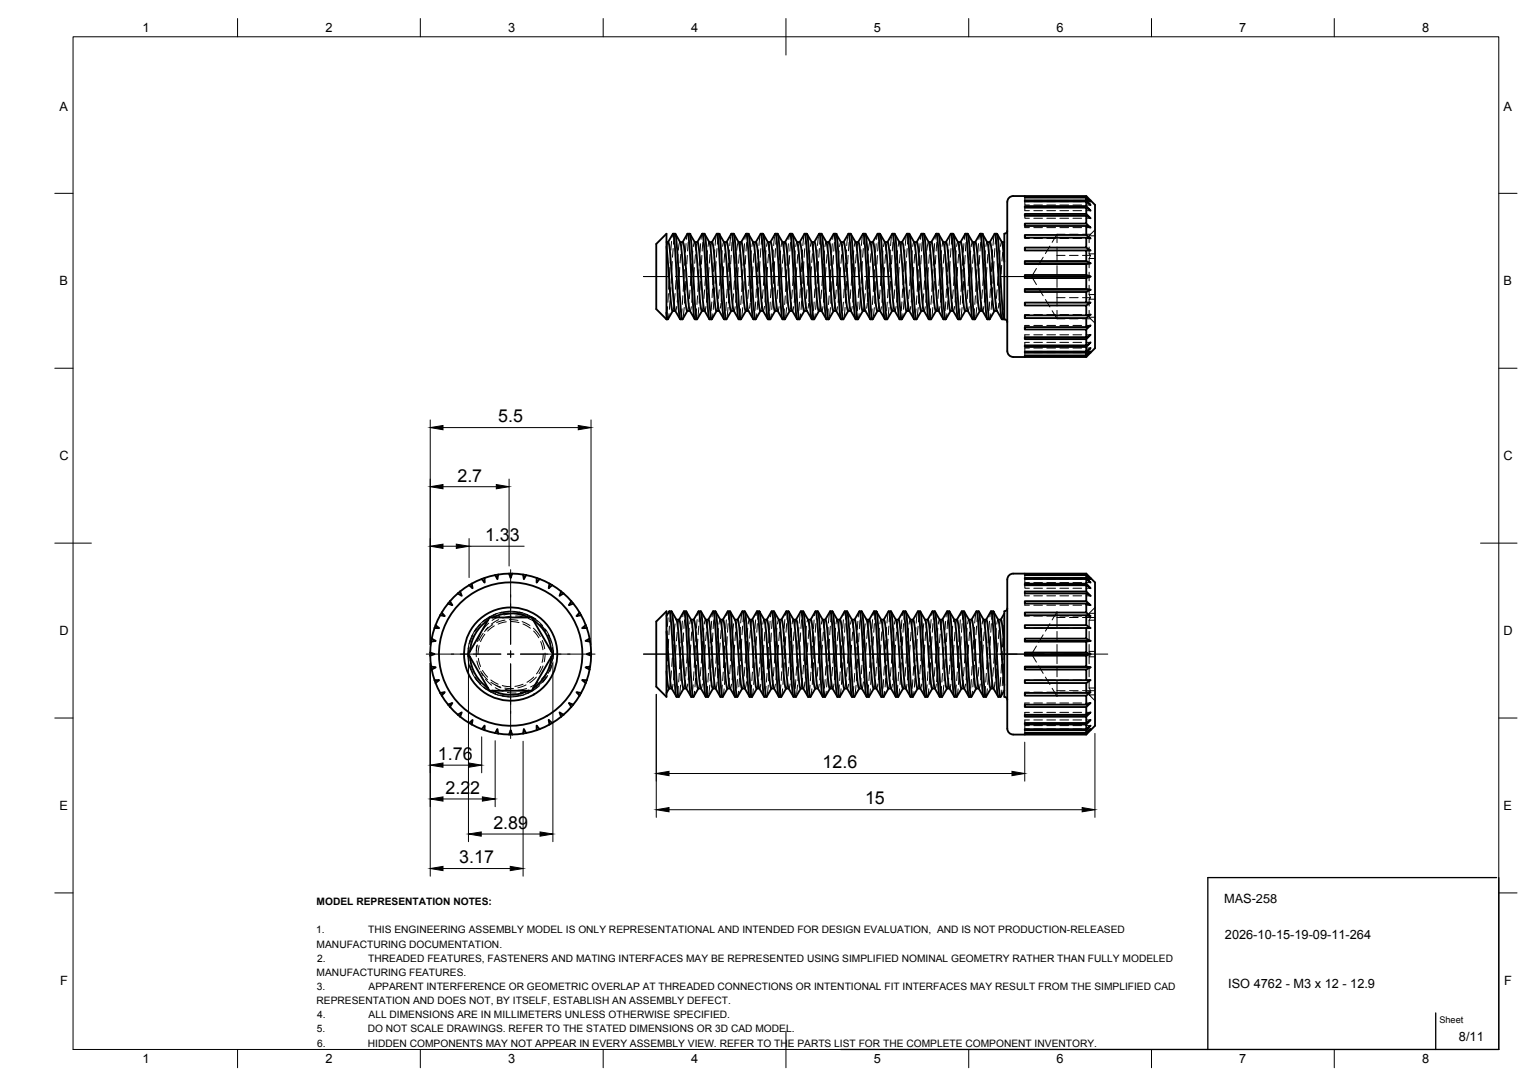
ISO-10303-21;
HEADER;
/* Generated by software containing ST-Developer
 * from STEP Tools, Inc. (www.steptools.com) 
 */

FILE_DESCRIPTION(
/* description */ (''),
/* implementation_level */ '2;1');

FILE_NAME(
/* name */ 'ISO 4762 - M3 x 12 - 12.9.step',
/* time_stamp */ '2026-10-15T12:29:06-07:00',
/* author */ (''),
/* organization */ (''),
/* preprocessor_version */ 'ST-DEVELOPER v20.2',
/* originating_system */ 'Autodesk Translation Framework v15.15.0.0',
/* authorisation */ '');

FILE_SCHEMA (('AUTOMOTIVE_DESIGN { 1 0 10303 214 3 1 1 }'));
ENDSEC;

DATA;
#10=MECHANICAL_DESIGN_GEOMETRIC_PRESENTATION_REPRESENTATION('',(#1749),#135282);
#95=TOROIDAL_SURFACE('',#33614,1.5635,0.1);
#96=TOROIDAL_SURFACE('',#33808,2.55,0.2);
#116=(
BOUNDED_CURVE()
B_SPLINE_CURVE(2,(#106679,#106680,#106681),.UNSPECIFIED.,.F.,.F.)
B_SPLINE_CURVE_WITH_KNOTS((3,3),(0.,0.0211644268265385),.UNSPECIFIED.)
CURVE()
GEOMETRIC_REPRESENTATION_ITEM()
RATIONAL_B_SPLINE_CURVE((1.,1.0009097917251,1.00093939181347))
REPRESENTATION_ITEM('')
);
#117=(
BOUNDED_CURVE()
B_SPLINE_CURVE(2,(#106685,#106686,#106687),.UNSPECIFIED.,.F.,.F.)
B_SPLINE_CURVE_WITH_KNOTS((3,3),(0.022587909800554,0.0437523366271111),
 .UNSPECIFIED.)
CURVE()
GEOMETRIC_REPRESENTATION_ITEM()
RATIONAL_B_SPLINE_CURVE((1.00093939181258,1.00090979172423,1.))
REPRESENTATION_ITEM('')
);
#118=(
BOUNDED_CURVE()
B_SPLINE_CURVE(2,(#106982,#106983,#106984),.UNSPECIFIED.,.F.,.F.)
B_SPLINE_CURVE_WITH_KNOTS((3,3),(0.,0.0211644268265826),.UNSPECIFIED.)
CURVE()
GEOMETRIC_REPRESENTATION_ITEM()
RATIONAL_B_SPLINE_CURVE((1.,1.00090979172134,1.00093939180958))
REPRESENTATION_ITEM('')
);
#119=(
BOUNDED_CURVE()
B_SPLINE_CURVE(2,(#106986,#106987,#106988),.UNSPECIFIED.,.F.,.F.)
B_SPLINE_CURVE_WITH_KNOTS((3,3),(0.0225879098005743,0.043752336627111),
 .UNSPECIFIED.)
CURVE()
GEOMETRIC_REPRESENTATION_ITEM()
RATIONAL_B_SPLINE_CURVE((1.00093939181478,1.00090979172637,1.))
REPRESENTATION_ITEM('')
);
#120=(
BOUNDED_CURVE()
B_SPLINE_CURVE(2,(#106993,#106994,#106995),.UNSPECIFIED.,.F.,.F.)
B_SPLINE_CURVE_WITH_KNOTS((3,3),(0.0225879098005881,0.043752336627111),
 .UNSPECIFIED.)
CURVE()
GEOMETRIC_REPRESENTATION_ITEM()
RATIONAL_B_SPLINE_CURVE((1.00093939180782,1.00090979171963,1.))
REPRESENTATION_ITEM('')
);
#121=(
BOUNDED_CURVE()
B_SPLINE_CURVE(2,(#106997,#106998,#106999),.UNSPECIFIED.,.F.,.F.)
B_SPLINE_CURVE_WITH_KNOTS((3,3),(0.,0.021164426826593),.UNSPECIFIED.)
CURVE()
GEOMETRIC_REPRESENTATION_ITEM()
RATIONAL_B_SPLINE_CURVE((1.,1.0009097917242,1.00093939181253))
REPRESENTATION_ITEM('')
);
#122=(
BOUNDED_CURVE()
B_SPLINE_CURVE(2,(#107000,#107001,#107002),.UNSPECIFIED.,.F.,.F.)
B_SPLINE_CURVE_WITH_KNOTS((3,3),(0.0225879098005839,0.0437523366271112),
 .UNSPECIFIED.)
CURVE()
GEOMETRIC_REPRESENTATION_ITEM()
RATIONAL_B_SPLINE_CURVE((1.00093939180822,1.00090979172002,1.))
REPRESENTATION_ITEM('')
);
#123=(
BOUNDED_CURVE()
B_SPLINE_CURVE(2,(#107004,#107005,#107006),.UNSPECIFIED.,.F.,.F.)
B_SPLINE_CURVE_WITH_KNOTS((3,3),(0.,0.0211644268265428),.UNSPECIFIED.)
CURVE()
GEOMETRIC_REPRESENTATION_ITEM()
RATIONAL_B_SPLINE_CURVE((1.,1.00090979172612,1.00093939181452))
REPRESENTATION_ITEM('')
);
#124=(
BOUNDED_CURVE()
B_SPLINE_CURVE(2,(#107007,#107008,#107009),.UNSPECIFIED.,.F.,.F.)
B_SPLINE_CURVE_WITH_KNOTS((3,3),(0.0225879098005574,0.0437523366271111),
 .UNSPECIFIED.)
CURVE()
GEOMETRIC_REPRESENTATION_ITEM()
RATIONAL_B_SPLINE_CURVE((1.00093939181255,1.00090979172421,1.))
REPRESENTATION_ITEM('')
);
#125=(
BOUNDED_CURVE()
B_SPLINE_CURVE(2,(#107011,#107012,#107013),.UNSPECIFIED.,.F.,.F.)
B_SPLINE_CURVE_WITH_KNOTS((3,3),(0.,0.0211644268266003),.UNSPECIFIED.)
CURVE()
GEOMETRIC_REPRESENTATION_ITEM()
RATIONAL_B_SPLINE_CURVE((1.,1.0009097917207,1.00093939180893))
REPRESENTATION_ITEM('')
);
#126=(
BOUNDED_CURVE()
B_SPLINE_CURVE(2,(#107014,#107015,#107016),.UNSPECIFIED.,.F.,.F.)
B_SPLINE_CURVE_WITH_KNOTS((3,3),(0.022587909800539,0.0437523366271111),
 .UNSPECIFIED.)
CURVE()
GEOMETRIC_REPRESENTATION_ITEM()
RATIONAL_B_SPLINE_CURVE((1.00093939181091,1.00090979172262,1.))
REPRESENTATION_ITEM('')
);
#127=(
BOUNDED_CURVE()
B_SPLINE_CURVE(2,(#107018,#107019,#107020),.UNSPECIFIED.,.F.,.F.)
B_SPLINE_CURVE_WITH_KNOTS((3,3),(0.,0.0211644268266019),.UNSPECIFIED.)
CURVE()
GEOMETRIC_REPRESENTATION_ITEM()
RATIONAL_B_SPLINE_CURVE((1.,1.0009097917251,1.00093939181347))
REPRESENTATION_ITEM('')
);
#128=(
BOUNDED_CURVE()
B_SPLINE_CURVE(2,(#107021,#107022,#107023),.UNSPECIFIED.,.F.,.F.)
B_SPLINE_CURVE_WITH_KNOTS((3,3),(0.0225879098005394,0.0437523366271111),
 .UNSPECIFIED.)
CURVE()
GEOMETRIC_REPRESENTATION_ITEM()
RATIONAL_B_SPLINE_CURVE((1.00093939181174,1.00090979172342,1.))
REPRESENTATION_ITEM('')
);
#129=(
BOUNDED_CURVE()
B_SPLINE_CURVE(2,(#107025,#107026,#107027),.UNSPECIFIED.,.F.,.F.)
B_SPLINE_CURVE_WITH_KNOTS((3,3),(0.,0.0211644268265645),.UNSPECIFIED.)
CURVE()
GEOMETRIC_REPRESENTATION_ITEM()
RATIONAL_B_SPLINE_CURVE((1.,1.00090979172128,1.00093939180953))
REPRESENTATION_ITEM('')
);
#130=(
BOUNDED_CURVE()
B_SPLINE_CURVE(2,(#107028,#107029,#107030),.UNSPECIFIED.,.F.,.F.)
B_SPLINE_CURVE_WITH_KNOTS((3,3),(0.0225879098005151,0.0437523366271111),
 .UNSPECIFIED.)
CURVE()
GEOMETRIC_REPRESENTATION_ITEM()
RATIONAL_B_SPLINE_CURVE((1.00093939181449,1.00090979172609,1.))
REPRESENTATION_ITEM('')
);
#131=(
BOUNDED_CURVE()
B_SPLINE_CURVE(2,(#107032,#107033,#107034),.UNSPECIFIED.,.F.,.F.)
B_SPLINE_CURVE_WITH_KNOTS((3,3),(0.,0.0211644268266015),.UNSPECIFIED.)
CURVE()
GEOMETRIC_REPRESENTATION_ITEM()
RATIONAL_B_SPLINE_CURVE((1.,1.00090979172521,1.00093939181358))
REPRESENTATION_ITEM('')
);
#132=(
BOUNDED_CURVE()
B_SPLINE_CURVE(2,(#107035,#107036,#107037),.UNSPECIFIED.,.F.,.F.)
B_SPLINE_CURVE_WITH_KNOTS((3,3),(0.0225879098005801,0.043752336627111),
 .UNSPECIFIED.)
CURVE()
GEOMETRIC_REPRESENTATION_ITEM()
RATIONAL_B_SPLINE_CURVE((1.00093939181248,1.00090979172414,1.))
REPRESENTATION_ITEM('')
);
#133=(
BOUNDED_CURVE()
B_SPLINE_CURVE(2,(#107039,#107040,#107041),.UNSPECIFIED.,.F.,.F.)
B_SPLINE_CURVE_WITH_KNOTS((3,3),(0.,0.0211644268265639),.UNSPECIFIED.)
CURVE()
GEOMETRIC_REPRESENTATION_ITEM()
RATIONAL_B_SPLINE_CURVE((1.,1.0009097917241,1.00093939181243))
REPRESENTATION_ITEM('')
);
#134=(
BOUNDED_CURVE()
B_SPLINE_CURVE(2,(#107042,#107043,#107044),.UNSPECIFIED.,.F.,.F.)
B_SPLINE_CURVE_WITH_KNOTS((3,3),(0.0225879098005415,0.043752336627111),
 .UNSPECIFIED.)
CURVE()
GEOMETRIC_REPRESENTATION_ITEM()
RATIONAL_B_SPLINE_CURVE((1.00093939181382,1.00090979172544,1.))
REPRESENTATION_ITEM('')
);
#135=(
BOUNDED_CURVE()
B_SPLINE_CURVE(2,(#107046,#107047,#107048),.UNSPECIFIED.,.F.,.F.)
B_SPLINE_CURVE_WITH_KNOTS((3,3),(0.,0.0211644268265226),.UNSPECIFIED.)
CURVE()
GEOMETRIC_REPRESENTATION_ITEM()
RATIONAL_B_SPLINE_CURVE((1.,1.00090979172353,1.00093939181185))
REPRESENTATION_ITEM('')
);
#136=(
BOUNDED_CURVE()
B_SPLINE_CURVE(2,(#107049,#107050,#107051),.UNSPECIFIED.,.F.,.F.)
B_SPLINE_CURVE_WITH_KNOTS((3,3),(0.0225879098005697,0.0437523366271111),
 .UNSPECIFIED.)
CURVE()
GEOMETRIC_REPRESENTATION_ITEM()
RATIONAL_B_SPLINE_CURVE((1.00093939181054,1.00090979172226,1.))
REPRESENTATION_ITEM('')
);
#137=(
BOUNDED_CURVE()
B_SPLINE_CURVE(2,(#107053,#107054,#107055),.UNSPECIFIED.,.F.,.F.)
B_SPLINE_CURVE_WITH_KNOTS((3,3),(0.,0.0211644268265259),.UNSPECIFIED.)
CURVE()
GEOMETRIC_REPRESENTATION_ITEM()
RATIONAL_B_SPLINE_CURVE((1.,1.00090979172262,1.00093939181091))
REPRESENTATION_ITEM('')
);
#138=(
BOUNDED_CURVE()
B_SPLINE_CURVE(2,(#107056,#107057,#107058),.UNSPECIFIED.,.F.,.F.)
B_SPLINE_CURVE_WITH_KNOTS((3,3),(0.0225879098005805,0.0437523366271111),
 .UNSPECIFIED.)
CURVE()
GEOMETRIC_REPRESENTATION_ITEM()
RATIONAL_B_SPLINE_CURVE((1.00093939181205,1.00090979172372,1.))
REPRESENTATION_ITEM('')
);
#139=(
BOUNDED_CURVE()
B_SPLINE_CURVE(2,(#107060,#107061,#107062),.UNSPECIFIED.,.F.,.F.)
B_SPLINE_CURVE_WITH_KNOTS((3,3),(0.,0.0211644268265664),.UNSPECIFIED.)
CURVE()
GEOMETRIC_REPRESENTATION_ITEM()
RATIONAL_B_SPLINE_CURVE((1.,1.0009097917218,1.00093939181006))
REPRESENTATION_ITEM('')
);
#140=(
BOUNDED_CURVE()
B_SPLINE_CURVE(2,(#107063,#107064,#107065),.UNSPECIFIED.,.F.,.F.)
B_SPLINE_CURVE_WITH_KNOTS((3,3),(0.0225879098005396,0.0437523366271112),
 .UNSPECIFIED.)
CURVE()
GEOMETRIC_REPRESENTATION_ITEM()
RATIONAL_B_SPLINE_CURVE((1.00093939181164,1.00090979172332,1.))
REPRESENTATION_ITEM('')
);
#141=(
BOUNDED_CURVE()
B_SPLINE_CURVE(2,(#107067,#107068,#107069),.UNSPECIFIED.,.F.,.F.)
B_SPLINE_CURVE_WITH_KNOTS((3,3),(0.,0.0211644268266089),.UNSPECIFIED.)
CURVE()
GEOMETRIC_REPRESENTATION_ITEM()
RATIONAL_B_SPLINE_CURVE((1.,1.0009097917234,1.00093939181171))
REPRESENTATION_ITEM('')
);
#142=(
BOUNDED_CURVE()
B_SPLINE_CURVE(2,(#107070,#107071,#107072),.UNSPECIFIED.,.F.,.F.)
B_SPLINE_CURVE_WITH_KNOTS((3,3),(0.0225879098005792,0.0437523366271112),
 .UNSPECIFIED.)
CURVE()
GEOMETRIC_REPRESENTATION_ITEM()
RATIONAL_B_SPLINE_CURVE((1.00093939181186,1.00090979172354,1.))
REPRESENTATION_ITEM('')
);
#143=(
BOUNDED_CURVE()
B_SPLINE_CURVE(2,(#107074,#107075,#107076),.UNSPECIFIED.,.F.,.F.)
B_SPLINE_CURVE_WITH_KNOTS((3,3),(0.,0.0211644268265289),.UNSPECIFIED.)
CURVE()
GEOMETRIC_REPRESENTATION_ITEM()
RATIONAL_B_SPLINE_CURVE((1.,1.00090979172507,1.00093939181344))
REPRESENTATION_ITEM('')
);
#144=(
BOUNDED_CURVE()
B_SPLINE_CURVE(2,(#107077,#107078,#107079),.UNSPECIFIED.,.F.,.F.)
B_SPLINE_CURVE_WITH_KNOTS((3,3),(0.0225879098005381,0.0437523366271112),
 .UNSPECIFIED.)
CURVE()
GEOMETRIC_REPRESENTATION_ITEM()
RATIONAL_B_SPLINE_CURVE((1.00093939181048,1.0009097917222,1.))
REPRESENTATION_ITEM('')
);
#145=(
BOUNDED_CURVE()
B_SPLINE_CURVE(2,(#107081,#107082,#107083),.UNSPECIFIED.,.F.,.F.)
B_SPLINE_CURVE_WITH_KNOTS((3,3),(0.,0.0211644268266039),.UNSPECIFIED.)
CURVE()
GEOMETRIC_REPRESENTATION_ITEM()
RATIONAL_B_SPLINE_CURVE((1.,1.00090979172139,1.00093939180963))
REPRESENTATION_ITEM('')
);
#146=(
BOUNDED_CURVE()
B_SPLINE_CURVE(2,(#107084,#107085,#107086),.UNSPECIFIED.,.F.,.F.)
B_SPLINE_CURVE_WITH_KNOTS((3,3),(0.0225879098005447,0.043752336627111),
 .UNSPECIFIED.)
CURVE()
GEOMETRIC_REPRESENTATION_ITEM()
RATIONAL_B_SPLINE_CURVE((1.00093939180967,1.00090979172142,1.))
REPRESENTATION_ITEM('')
);
#147=(
BOUNDED_CURVE()
B_SPLINE_CURVE(2,(#107088,#107089,#107090),.UNSPECIFIED.,.F.,.F.)
B_SPLINE_CURVE_WITH_KNOTS((3,3),(0.,0.021164426826594),.UNSPECIFIED.)
CURVE()
GEOMETRIC_REPRESENTATION_ITEM()
RATIONAL_B_SPLINE_CURVE((1.,1.00090979172174,1.00093939181))
REPRESENTATION_ITEM('')
);
#148=(
BOUNDED_CURVE()
B_SPLINE_CURVE(2,(#107091,#107092,#107093),.UNSPECIFIED.,.F.,.F.)
B_SPLINE_CURVE_WITH_KNOTS((3,3),(0.0225879098005432,0.043752336627111),
 .UNSPECIFIED.)
CURVE()
GEOMETRIC_REPRESENTATION_ITEM()
RATIONAL_B_SPLINE_CURVE((1.00093939180984,1.00090979172158,1.))
REPRESENTATION_ITEM('')
);
#149=(
BOUNDED_CURVE()
B_SPLINE_CURVE(2,(#107095,#107096,#107097),.UNSPECIFIED.,.F.,.F.)
B_SPLINE_CURVE_WITH_KNOTS((3,3),(0.,0.0211644268265628),.UNSPECIFIED.)
CURVE()
GEOMETRIC_REPRESENTATION_ITEM()
RATIONAL_B_SPLINE_CURVE((1.,1.00090979172392,1.00093939181225))
REPRESENTATION_ITEM('')
);
#150=(
BOUNDED_CURVE()
B_SPLINE_CURVE(2,(#107098,#107099,#107100),.UNSPECIFIED.,.F.,.F.)
B_SPLINE_CURVE_WITH_KNOTS((3,3),(0.0225879098005512,0.043752336627111),
 .UNSPECIFIED.)
CURVE()
GEOMETRIC_REPRESENTATION_ITEM()
RATIONAL_B_SPLINE_CURVE((1.00093939181024,1.00090979172197,1.))
REPRESENTATION_ITEM('')
);
#151=(
BOUNDED_CURVE()
B_SPLINE_CURVE(2,(#107102,#107103,#107104),.UNSPECIFIED.,.F.,.F.)
B_SPLINE_CURVE_WITH_KNOTS((3,3),(0.,0.0211644268265179),.UNSPECIFIED.)
CURVE()
GEOMETRIC_REPRESENTATION_ITEM()
RATIONAL_B_SPLINE_CURVE((1.,1.00090979172158,1.00093939180984))
REPRESENTATION_ITEM('')
);
#152=(
BOUNDED_CURVE()
B_SPLINE_CURVE(2,(#107105,#107106,#107107),.UNSPECIFIED.,.F.,.F.)
B_SPLINE_CURVE_WITH_KNOTS((3,3),(0.0225879098005361,0.043752336627111),
 .UNSPECIFIED.)
CURVE()
GEOMETRIC_REPRESENTATION_ITEM()
RATIONAL_B_SPLINE_CURVE((1.00093939181327,1.00090979172491,1.))
REPRESENTATION_ITEM('')
);
#153=(
BOUNDED_CURVE()
B_SPLINE_CURVE(2,(#107109,#107110,#107111),.UNSPECIFIED.,.F.,.F.)
B_SPLINE_CURVE_WITH_KNOTS((3,3),(0.,0.0211644268265286),.UNSPECIFIED.)
CURVE()
GEOMETRIC_REPRESENTATION_ITEM()
RATIONAL_B_SPLINE_CURVE((1.,1.00090979172298,1.00093939181129))
REPRESENTATION_ITEM('')
);
#154=(
BOUNDED_CURVE()
B_SPLINE_CURVE(2,(#107112,#107113,#107114),.UNSPECIFIED.,.F.,.F.)
B_SPLINE_CURVE_WITH_KNOTS((3,3),(0.0225879098005504,0.043752336627111),
 .UNSPECIFIED.)
CURVE()
GEOMETRIC_REPRESENTATION_ITEM()
RATIONAL_B_SPLINE_CURVE((1.00093939181167,1.00090979172335,1.))
REPRESENTATION_ITEM('')
);
#155=(
BOUNDED_CURVE()
B_SPLINE_CURVE(2,(#107116,#107117,#107118),.UNSPECIFIED.,.F.,.F.)
B_SPLINE_CURVE_WITH_KNOTS((3,3),(0.,0.0211644268266161),.UNSPECIFIED.)
CURVE()
GEOMETRIC_REPRESENTATION_ITEM()
RATIONAL_B_SPLINE_CURVE((1.,1.00090979172455,1.0009393918129))
REPRESENTATION_ITEM('')
);
#156=(
BOUNDED_CURVE()
B_SPLINE_CURVE(2,(#107119,#107120,#107121),.UNSPECIFIED.,.F.,.F.)
B_SPLINE_CURVE_WITH_KNOTS((3,3),(0.0225879098004947,0.0437523366271108),
 .UNSPECIFIED.)
CURVE()
GEOMETRIC_REPRESENTATION_ITEM()
RATIONAL_B_SPLINE_CURVE((1.0009393918129,1.00090979172455,1.))
REPRESENTATION_ITEM('')
);
#157=(
BOUNDED_CURVE()
B_SPLINE_CURVE(2,(#107123,#107124,#107125),.UNSPECIFIED.,.F.,.F.)
B_SPLINE_CURVE_WITH_KNOTS((3,3),(0.,0.0211644268265652),.UNSPECIFIED.)
CURVE()
GEOMETRIC_REPRESENTATION_ITEM()
RATIONAL_B_SPLINE_CURVE((1.,1.00090979172294,1.00093939181124))
REPRESENTATION_ITEM('')
);
#158=(
BOUNDED_CURVE()
B_SPLINE_CURVE(2,(#107126,#107127,#107128),.UNSPECIFIED.,.F.,.F.)
B_SPLINE_CURVE_WITH_KNOTS((3,3),(0.0225879098005252,0.043752336627111),
 .UNSPECIFIED.)
CURVE()
GEOMETRIC_REPRESENTATION_ITEM()
RATIONAL_B_SPLINE_CURVE((1.00093939181149,1.00090979172318,1.))
REPRESENTATION_ITEM('')
);
#159=(
BOUNDED_CURVE()
B_SPLINE_CURVE(2,(#107130,#107131,#107132),.UNSPECIFIED.,.F.,.F.)
B_SPLINE_CURVE_WITH_KNOTS((3,3),(0.,0.0211644268265705),.UNSPECIFIED.)
CURVE()
GEOMETRIC_REPRESENTATION_ITEM()
RATIONAL_B_SPLINE_CURVE((1.,1.00090979172216,1.00093939181044))
REPRESENTATION_ITEM('')
);
#160=(
BOUNDED_CURVE()
B_SPLINE_CURVE(2,(#107133,#107134,#107135),.UNSPECIFIED.,.F.,.F.)
B_SPLINE_CURVE_WITH_KNOTS((3,3),(0.0225879098005481,0.043752336627111),
 .UNSPECIFIED.)
CURVE()
GEOMETRIC_REPRESENTATION_ITEM()
RATIONAL_B_SPLINE_CURVE((1.00093939181285,1.0009097917245,1.))
REPRESENTATION_ITEM('')
);
#161=(
BOUNDED_CURVE()
B_SPLINE_CURVE(2,(#107137,#107138,#107139),.UNSPECIFIED.,.F.,.F.)
B_SPLINE_CURVE_WITH_KNOTS((3,3),(0.,0.0211644268265925),.UNSPECIFIED.)
CURVE()
GEOMETRIC_REPRESENTATION_ITEM()
RATIONAL_B_SPLINE_CURVE((1.,1.0009097917218,1.00093939181007))
REPRESENTATION_ITEM('')
);
#162=(
BOUNDED_CURVE()
B_SPLINE_CURVE(2,(#107140,#107141,#107142),.UNSPECIFIED.,.F.,.F.)
B_SPLINE_CURVE_WITH_KNOTS((3,3),(0.0225879098005822,0.0437523366271111),
 .UNSPECIFIED.)
CURVE()
GEOMETRIC_REPRESENTATION_ITEM()
RATIONAL_B_SPLINE_CURVE((1.00093939181221,1.00090979172388,1.))
REPRESENTATION_ITEM('')
);
#163=(
BOUNDED_CURVE()
B_SPLINE_CURVE(2,(#107144,#107145,#107146),.UNSPECIFIED.,.F.,.F.)
B_SPLINE_CURVE_WITH_KNOTS((3,3),(0.,0.0211644268265208),.UNSPECIFIED.)
CURVE()
GEOMETRIC_REPRESENTATION_ITEM()
RATIONAL_B_SPLINE_CURVE((1.,1.00090979172231,1.00093939181059))
REPRESENTATION_ITEM('')
);
#164=(
BOUNDED_CURVE()
B_SPLINE_CURVE(2,(#107147,#107148,#107149),.UNSPECIFIED.,.F.,.F.)
B_SPLINE_CURVE_WITH_KNOTS((3,3),(0.0225879098005163,0.043752336627111),
 .UNSPECIFIED.)
CURVE()
GEOMETRIC_REPRESENTATION_ITEM()
RATIONAL_B_SPLINE_CURVE((1.00093939181029,1.00090979172202,1.))
REPRESENTATION_ITEM('')
);
#165=(
BOUNDED_CURVE()
B_SPLINE_CURVE(2,(#107151,#107152,#107153),.UNSPECIFIED.,.F.,.F.)
B_SPLINE_CURVE_WITH_KNOTS((3,3),(0.,0.0211644268265845),.UNSPECIFIED.)
CURVE()
GEOMETRIC_REPRESENTATION_ITEM()
RATIONAL_B_SPLINE_CURVE((1.,1.00090979172432,1.00093939181266))
REPRESENTATION_ITEM('')
);
#166=(
BOUNDED_CURVE()
B_SPLINE_CURVE(2,(#107154,#107155,#107156),.UNSPECIFIED.,.F.,.F.)
B_SPLINE_CURVE_WITH_KNOTS((3,3),(0.0225879098005664,0.043752336627111),
 .UNSPECIFIED.)
CURVE()
GEOMETRIC_REPRESENTATION_ITEM()
RATIONAL_B_SPLINE_CURVE((1.0009393918107,1.00090979172242,1.))
REPRESENTATION_ITEM('')
);
#167=(
BOUNDED_CURVE()
B_SPLINE_CURVE(2,(#107158,#107159,#107160),.UNSPECIFIED.,.F.,.F.)
B_SPLINE_CURVE_WITH_KNOTS((3,3),(0.,0.0211644268265342),.UNSPECIFIED.)
CURVE()
GEOMETRIC_REPRESENTATION_ITEM()
RATIONAL_B_SPLINE_CURVE((1.,1.00090979172415,1.00093939181249))
REPRESENTATION_ITEM('')
);
#168=(
BOUNDED_CURVE()
B_SPLINE_CURVE(2,(#107161,#107162,#107163),.UNSPECIFIED.,.F.,.F.)
B_SPLINE_CURVE_WITH_KNOTS((3,3),(0.0225879098005407,0.043752336627111),
 .UNSPECIFIED.)
CURVE()
GEOMETRIC_REPRESENTATION_ITEM()
RATIONAL_B_SPLINE_CURVE((1.00093939181109,1.0009097917228,1.))
REPRESENTATION_ITEM('')
);
#169=(
BOUNDED_CURVE()
B_SPLINE_CURVE(2,(#107165,#107166,#107167),.UNSPECIFIED.,.F.,.F.)
B_SPLINE_CURVE_WITH_KNOTS((3,3),(0.,0.0211644268265271),.UNSPECIFIED.)
CURVE()
GEOMETRIC_REPRESENTATION_ITEM()
RATIONAL_B_SPLINE_CURVE((1.,1.00090979172368,1.00093939181201))
REPRESENTATION_ITEM('')
);
#170=(
BOUNDED_CURVE()
B_SPLINE_CURVE(2,(#107168,#107169,#107170),.UNSPECIFIED.,.F.,.F.)
B_SPLINE_CURVE_WITH_KNOTS((3,3),(0.0225879098005404,0.0437523366271111),
 .UNSPECIFIED.)
CURVE()
GEOMETRIC_REPRESENTATION_ITEM()
RATIONAL_B_SPLINE_CURVE((1.00093939181205,1.00090979172373,1.))
REPRESENTATION_ITEM('')
);
#171=(
BOUNDED_CURVE()
B_SPLINE_CURVE(2,(#107172,#107173,#107174),.UNSPECIFIED.,.F.,.F.)
B_SPLINE_CURVE_WITH_KNOTS((3,3),(0.,0.0211644268265742),.UNSPECIFIED.)
CURVE()
GEOMETRIC_REPRESENTATION_ITEM()
RATIONAL_B_SPLINE_CURVE((1.,1.00090979172235,1.00093939181063))
REPRESENTATION_ITEM('')
);
#172=(
BOUNDED_CURVE()
B_SPLINE_CURVE(2,(#107175,#107176,#107177),.UNSPECIFIED.,.F.,.F.)
B_SPLINE_CURVE_WITH_KNOTS((3,3),(0.0225879098005505,0.0437523366271111),
 .UNSPECIFIED.)
CURVE()
GEOMETRIC_REPRESENTATION_ITEM()
RATIONAL_B_SPLINE_CURVE((1.00093939181362,1.00090979172525,1.))
REPRESENTATION_ITEM('')
);
#173=(
BOUNDED_CURVE()
B_SPLINE_CURVE(2,(#107179,#107180,#107181),.UNSPECIFIED.,.F.,.F.)
B_SPLINE_CURVE_WITH_KNOTS((3,3),(0.,0.0211644268265471),.UNSPECIFIED.)
CURVE()
GEOMETRIC_REPRESENTATION_ITEM()
RATIONAL_B_SPLINE_CURVE((1.,1.00090979172441,1.00093939181276))
REPRESENTATION_ITEM('')
);
#174=(
BOUNDED_CURVE()
B_SPLINE_CURVE(2,(#107182,#107183,#107184),.UNSPECIFIED.,.F.,.F.)
B_SPLINE_CURVE_WITH_KNOTS((3,3),(0.0225879098005329,0.0437523366271112),
 .UNSPECIFIED.)
CURVE()
GEOMETRIC_REPRESENTATION_ITEM()
RATIONAL_B_SPLINE_CURVE((1.00093939181116,1.00090979172287,1.))
REPRESENTATION_ITEM('')
);
#175=(
BOUNDED_CURVE()
B_SPLINE_CURVE(2,(#107186,#107187,#107188),.UNSPECIFIED.,.F.,.F.)
B_SPLINE_CURVE_WITH_KNOTS((3,3),(0.,0.021164426826566),.UNSPECIFIED.)
CURVE()
GEOMETRIC_REPRESENTATION_ITEM()
RATIONAL_B_SPLINE_CURVE((1.,1.00090979172296,1.00093939181126))
REPRESENTATION_ITEM('')
);
#176=(
BOUNDED_CURVE()
B_SPLINE_CURVE(2,(#107189,#107190,#107191),.UNSPECIFIED.,.F.,.F.)
B_SPLINE_CURVE_WITH_KNOTS((3,3),(0.0225879098005499,0.0437523366271111),
 .UNSPECIFIED.)
CURVE()
GEOMETRIC_REPRESENTATION_ITEM()
RATIONAL_B_SPLINE_CURVE((1.0009393918127,1.00090979172436,1.))
REPRESENTATION_ITEM('')
);
#177=(
BOUNDED_CURVE()
B_SPLINE_CURVE(2,(#107193,#107194,#107195),.UNSPECIFIED.,.F.,.F.)
B_SPLINE_CURVE_WITH_KNOTS((3,3),(0.,0.0211644268265843),.UNSPECIFIED.)
CURVE()
GEOMETRIC_REPRESENTATION_ITEM()
RATIONAL_B_SPLINE_CURVE((1.,1.00090979172607,1.00093939181447))
REPRESENTATION_ITEM('')
);
#178=(
BOUNDED_CURVE()
B_SPLINE_CURVE(2,(#107196,#107197,#107198),.UNSPECIFIED.,.F.,.F.)
B_SPLINE_CURVE_WITH_KNOTS((3,3),(0.0225879098005132,0.0437523366271111),
 .UNSPECIFIED.)
CURVE()
GEOMETRIC_REPRESENTATION_ITEM()
RATIONAL_B_SPLINE_CURVE((1.00093939181137,1.00090979172306,1.))
REPRESENTATION_ITEM('')
);
#179=(
BOUNDED_CURVE()
B_SPLINE_CURVE(2,(#107200,#107201,#107202),.UNSPECIFIED.,.F.,.F.)
B_SPLINE_CURVE_WITH_KNOTS((3,3),(0.,0.0211644268266212),.UNSPECIFIED.)
CURVE()
GEOMETRIC_REPRESENTATION_ITEM()
RATIONAL_B_SPLINE_CURVE((1.,1.00090979172711,1.00093939181555))
REPRESENTATION_ITEM('')
);
#180=(
BOUNDED_CURVE()
B_SPLINE_CURVE(2,(#107203,#107204,#107205),.UNSPECIFIED.,.F.,.F.)
B_SPLINE_CURVE_WITH_KNOTS((3,3),(0.0225879098005048,0.0437523366271112),
 .UNSPECIFIED.)
CURVE()
GEOMETRIC_REPRESENTATION_ITEM()
RATIONAL_B_SPLINE_CURVE((1.00093939181225,1.00090979172392,1.))
REPRESENTATION_ITEM('')
);
#181=(
BOUNDED_CURVE()
B_SPLINE_CURVE(2,(#107207,#107208,#107209),.UNSPECIFIED.,.F.,.F.)
B_SPLINE_CURVE_WITH_KNOTS((3,3),(0.,0.0211644268265508),.UNSPECIFIED.)
CURVE()
GEOMETRIC_REPRESENTATION_ITEM()
RATIONAL_B_SPLINE_CURVE((1.,1.0009097917239,1.00093939181223))
REPRESENTATION_ITEM('')
);
#182=(
BOUNDED_CURVE()
B_SPLINE_CURVE(2,(#107210,#107211,#107212),.UNSPECIFIED.,.F.,.F.)
B_SPLINE_CURVE_WITH_KNOTS((3,3),(0.0225879098005375,0.0437523366271112),
 .UNSPECIFIED.)
CURVE()
GEOMETRIC_REPRESENTATION_ITEM()
RATIONAL_B_SPLINE_CURVE((1.00093939181233,1.000909791724,1.))
REPRESENTATION_ITEM('')
);
#183=(
BOUNDED_CURVE()
B_SPLINE_CURVE(2,(#107214,#107215,#107216),.UNSPECIFIED.,.F.,.F.)
B_SPLINE_CURVE_WITH_KNOTS((3,3),(0.,0.0211644268265515),.UNSPECIFIED.)
CURVE()
GEOMETRIC_REPRESENTATION_ITEM()
RATIONAL_B_SPLINE_CURVE((1.,1.00090979172704,1.00093939181547))
REPRESENTATION_ITEM('')
);
#184=(
BOUNDED_CURVE()
B_SPLINE_CURVE(2,(#107217,#107218,#107219),.UNSPECIFIED.,.F.,.F.)
B_SPLINE_CURVE_WITH_KNOTS((3,3),(0.022587909800513,0.043752336627111),
 .UNSPECIFIED.)
CURVE()
GEOMETRIC_REPRESENTATION_ITEM()
RATIONAL_B_SPLINE_CURVE((1.00093939181505,1.00090979172663,1.))
REPRESENTATION_ITEM('')
);
#185=(
BOUNDED_CURVE()
B_SPLINE_CURVE(2,(#107221,#107222,#107223),.UNSPECIFIED.,.F.,.F.)
B_SPLINE_CURVE_WITH_KNOTS((3,3),(0.,0.0211644268265743),.UNSPECIFIED.)
CURVE()
GEOMETRIC_REPRESENTATION_ITEM()
RATIONAL_B_SPLINE_CURVE((1.,1.00090979171876,1.00093939180693))
REPRESENTATION_ITEM('')
);
#186=(
BOUNDED_CURVE()
B_SPLINE_CURVE(2,(#107224,#107225,#107226),.UNSPECIFIED.,.F.,.F.)
B_SPLINE_CURVE_WITH_KNOTS((3,3),(0.0225879098005165,0.0437523366271111),
 .UNSPECIFIED.)
CURVE()
GEOMETRIC_REPRESENTATION_ITEM()
RATIONAL_B_SPLINE_CURVE((1.00093939181478,1.00090979172637,1.))
REPRESENTATION_ITEM('')
);
#187=(
BOUNDED_CURVE()
B_SPLINE_CURVE(2,(#107227,#107228,#107229),.UNSPECIFIED.,.F.,.F.)
B_SPLINE_CURVE_WITH_KNOTS((3,3),(0.,0.0211644268265909),.UNSPECIFIED.)
CURVE()
GEOMETRIC_REPRESENTATION_ITEM()
RATIONAL_B_SPLINE_CURVE((1.,1.00090979172334,1.00093939181166))
REPRESENTATION_ITEM('')
);
#188=(
BOUNDED_CURVE()
B_SPLINE_CURVE(2,(#107479,#107480,#107481),.UNSPECIFIED.,.F.,.F.)
B_SPLINE_CURVE_WITH_KNOTS((3,3),(0.,0.0126130588257607),.UNSPECIFIED.)
CURVE()
GEOMETRIC_REPRESENTATION_ITEM()
RATIONAL_B_SPLINE_CURVE((1.,1.00234596681281,1.00329298027609))
REPRESENTATION_ITEM('')
);
#189=(
BOUNDED_CURVE()
B_SPLINE_CURVE(2,(#107485,#107486,#107487),.UNSPECIFIED.,.F.,.F.)
B_SPLINE_CURVE_WITH_KNOTS((3,3),(0.0296897347922136,0.0423027936179772),
 .UNSPECIFIED.)
CURVE()
GEOMETRIC_REPRESENTATION_ITEM()
RATIONAL_B_SPLINE_CURVE((1.00329298027575,1.00234596681257,1.))
REPRESENTATION_ITEM('')
);
#190=(
BOUNDED_CURVE()
B_SPLINE_CURVE(2,(#107489,#107490,#107491),.UNSPECIFIED.,.F.,.F.)
B_SPLINE_CURVE_WITH_KNOTS((3,3),(0.,0.0126130588257611),.UNSPECIFIED.)
CURVE()
GEOMETRIC_REPRESENTATION_ITEM()
RATIONAL_B_SPLINE_CURVE((1.,1.00234596681276,1.00329298027602))
REPRESENTATION_ITEM('')
);
#191=(
BOUNDED_CURVE()
B_SPLINE_CURVE(2,(#107495,#107496,#107497),.UNSPECIFIED.,.F.,.F.)
B_SPLINE_CURVE_WITH_KNOTS((3,3),(0.0296897347922145,0.0423027936179771),
 .UNSPECIFIED.)
CURVE()
GEOMETRIC_REPRESENTATION_ITEM()
RATIONAL_B_SPLINE_CURVE((1.00329298027584,1.00234596681264,1.))
REPRESENTATION_ITEM('')
);
#192=(
BOUNDED_CURVE()
B_SPLINE_CURVE(2,(#107499,#107500,#107501),.UNSPECIFIED.,.F.,.F.)
B_SPLINE_CURVE_WITH_KNOTS((3,3),(0.,0.0126130588257613),.UNSPECIFIED.)
CURVE()
GEOMETRIC_REPRESENTATION_ITEM()
RATIONAL_B_SPLINE_CURVE((1.,1.00234596681274,1.00329298027598))
REPRESENTATION_ITEM('')
);
#193=(
BOUNDED_CURVE()
B_SPLINE_CURVE(2,(#107505,#107506,#107507),.UNSPECIFIED.,.F.,.F.)
B_SPLINE_CURVE_WITH_KNOTS((3,3),(0.0296897347922162,0.0423027936179772),
 .UNSPECIFIED.)
CURVE()
GEOMETRIC_REPRESENTATION_ITEM()
RATIONAL_B_SPLINE_CURVE((1.00329298027606,1.00234596681279,1.))
REPRESENTATION_ITEM('')
);
#194=(
BOUNDED_CURVE()
B_SPLINE_CURVE(2,(#107509,#107510,#107511),.UNSPECIFIED.,.F.,.F.)
B_SPLINE_CURVE_WITH_KNOTS((3,3),(0.,0.0126130588257623),.UNSPECIFIED.)
CURVE()
GEOMETRIC_REPRESENTATION_ITEM()
RATIONAL_B_SPLINE_CURVE((1.,1.00234596681267,1.00329298027589))
REPRESENTATION_ITEM('')
);
#195=(
BOUNDED_CURVE()
B_SPLINE_CURVE(2,(#107515,#107516,#107517),.UNSPECIFIED.,.F.,.F.)
B_SPLINE_CURVE_WITH_KNOTS((3,3),(0.0296897347922159,0.0423027936179772),
 .UNSPECIFIED.)
CURVE()
GEOMETRIC_REPRESENTATION_ITEM()
RATIONAL_B_SPLINE_CURVE((1.00329298027606,1.00234596681279,1.))
REPRESENTATION_ITEM('')
);
#196=(
BOUNDED_CURVE()
B_SPLINE_CURVE(2,(#107519,#107520,#107521),.UNSPECIFIED.,.F.,.F.)
B_SPLINE_CURVE_WITH_KNOTS((3,3),(0.,0.0126130588257623),.UNSPECIFIED.)
CURVE()
GEOMETRIC_REPRESENTATION_ITEM()
RATIONAL_B_SPLINE_CURVE((1.,1.00234596681271,1.00329298027594))
REPRESENTATION_ITEM('')
);
#197=(
BOUNDED_CURVE()
B_SPLINE_CURVE(2,(#107525,#107526,#107527),.UNSPECIFIED.,.F.,.F.)
B_SPLINE_CURVE_WITH_KNOTS((3,3),(0.0296897347922137,0.0423027936179772),
 .UNSPECIFIED.)
CURVE()
GEOMETRIC_REPRESENTATION_ITEM()
RATIONAL_B_SPLINE_CURVE((1.00329298027579,1.0023459668126,1.))
REPRESENTATION_ITEM('')
);
#198=(
BOUNDED_CURVE()
B_SPLINE_CURVE(2,(#107529,#107530,#107531),.UNSPECIFIED.,.F.,.F.)
B_SPLINE_CURVE_WITH_KNOTS((3,3),(0.,0.0126130588257624),.UNSPECIFIED.)
CURVE()
GEOMETRIC_REPRESENTATION_ITEM()
RATIONAL_B_SPLINE_CURVE((1.,1.00234596681265,1.00329298027586))
REPRESENTATION_ITEM('')
);
#199=(
BOUNDED_CURVE()
B_SPLINE_CURVE(2,(#107534,#107535,#107536),.UNSPECIFIED.,.F.,.F.)
B_SPLINE_CURVE_WITH_KNOTS((3,3),(0.0296897347922151,0.0423027936179771),
 .UNSPECIFIED.)
CURVE()
GEOMETRIC_REPRESENTATION_ITEM()
RATIONAL_B_SPLINE_CURVE((1.00329298027587,1.00234596681266,1.))
REPRESENTATION_ITEM('')
);
#611=B_SPLINE_SURFACE_WITH_KNOTS('',3,3,((#105337,#105338,#105339,#105340,
#105341,#105342,#105343,#105344,#105345,#105346,#105347,#105348,#105349,
#105350,#105351,#105352,#105353,#105354,#105355,#105356,#105357,#105358,
#105359,#105360,#105361,#105362,#105363,#105364,#105365,#105366,#105367,
#105368,#105369,#105370,#105371,#105372,#105373,#105374,#105375,#105376,
#105377,#105378,#105379,#105380,#105381,#105382,#105383,#105384,#105385,
#105386,#105387,#105388,#105389,#105390,#105391,#105392,#105393,#105394,
#105395,#105396,#105397,#105398,#105399,#105400,#105401,#105402,#105403,
#105404,#105405,#105406,#105407,#105408,#105409,#105410,#105411,#105412,
#105413,#105414,#105415,#105416,#105417,#105418,#105419,#105420,#105421,
#105422,#105423,#105424,#105425,#105426,#105427,#105428,#105429,#105430,
#105431,#105432,#105433,#105434,#105435,#105436,#105437,#105438,#105439,
#105440,#105441,#105442,#105443,#105444,#105445,#105446,#105447,#105448,
#105449,#105450,#105451,#105452,#105453,#105454,#105455,#105456,#105457,
#105458,#105459,#105460,#105461,#105462,#105463,#105464,#105465,#105466,
#105467,#105468,#105469,#105470,#105471,#105472,#105473,#105474,#105475,
#105476,#105477,#105478,#105479,#105480,#105481,#105482,#105483,#105484,
#105485,#105486,#105487),(#105488,#105489,#105490,#105491,#105492,#105493,
#105494,#105495,#105496,#105497,#105498,#105499,#105500,#105501,#105502,
#105503,#105504,#105505,#105506,#105507,#105508,#105509,#105510,#105511,
#105512,#105513,#105514,#105515,#105516,#105517,#105518,#105519,#105520,
#105521,#105522,#105523,#105524,#105525,#105526,#105527,#105528,#105529,
#105530,#105531,#105532,#105533,#105534,#105535,#105536,#105537,#105538,
#105539,#105540,#105541,#105542,#105543,#105544,#105545,#105546,#105547,
#105548,#105549,#105550,#105551,#105552,#105553,#105554,#105555,#105556,
#105557,#105558,#105559,#105560,#105561,#105562,#105563,#105564,#105565,
#105566,#105567,#105568,#105569,#105570,#105571,#105572,#105573,#105574,
#105575,#105576,#105577,#105578,#105579,#105580,#105581,#105582,#105583,
#105584,#105585,#105586,#105587,#105588,#105589,#105590,#105591,#105592,
#105593,#105594,#105595,#105596,#105597,#105598,#105599,#105600,#105601,
#105602,#105603,#105604,#105605,#105606,#105607,#105608,#105609,#105610,
#105611,#105612,#105613,#105614,#105615,#105616,#105617,#105618,#105619,
#105620,#105621,#105622,#105623,#105624,#105625,#105626,#105627,#105628,
#105629,#105630,#105631,#105632,#105633,#105634,#105635,#105636,#105637,
#105638),(#105639,#105640,#105641,#105642,#105643,#105644,#105645,#105646,
#105647,#105648,#105649,#105650,#105651,#105652,#105653,#105654,#105655,
#105656,#105657,#105658,#105659,#105660,#105661,#105662,#105663,#105664,
#105665,#105666,#105667,#105668,#105669,#105670,#105671,#105672,#105673,
#105674,#105675,#105676,#105677,#105678,#105679,#105680,#105681,#105682,
#105683,#105684,#105685,#105686,#105687,#105688,#105689,#105690,#105691,
#105692,#105693,#105694,#105695,#105696,#105697,#105698,#105699,#105700,
#105701,#105702,#105703,#105704,#105705,#105706,#105707,#105708,#105709,
#105710,#105711,#105712,#105713,#105714,#105715,#105716,#105717,#105718,
#105719,#105720,#105721,#105722,#105723,#105724,#105725,#105726,#105727,
#105728,#105729,#105730,#105731,#105732,#105733,#105734,#105735,#105736,
#105737,#105738,#105739,#105740,#105741,#105742,#105743,#105744,#105745,
#105746,#105747,#105748,#105749,#105750,#105751,#105752,#105753,#105754,
#105755,#105756,#105757,#105758,#105759,#105760,#105761,#105762,#105763,
#105764,#105765,#105766,#105767,#105768,#105769,#105770,#105771,#105772,
#105773,#105774,#105775,#105776,#105777,#105778,#105779,#105780,#105781,
#105782,#105783,#105784,#105785,#105786,#105787,#105788,#105789),(#105790,
#105791,#105792,#105793,#105794,#105795,#105796,#105797,#105798,#105799,
#105800,#105801,#105802,#105803,#105804,#105805,#105806,#105807,#105808,
#105809,#105810,#105811,#105812,#105813,#105814,#105815,#105816,#105817,
#105818,#105819,#105820,#105821,#105822,#105823,#105824,#105825,#105826,
#105827,#105828,#105829,#105830,#105831,#105832,#105833,#105834,#105835,
#105836,#105837,#105838,#105839,#105840,#105841,#105842,#105843,#105844,
#105845,#105846,#105847,#105848,#105849,#105850,#105851,#105852,#105853,
#105854,#105855,#105856,#105857,#105858,#105859,#105860,#105861,#105862,
#105863,#105864,#105865,#105866,#105867,#105868,#105869,#105870,#105871,
#105872,#105873,#105874,#105875,#105876,#105877,#105878,#105879,#105880,
#105881,#105882,#105883,#105884,#105885,#105886,#105887,#105888,#105889,
#105890,#105891,#105892,#105893,#105894,#105895,#105896,#105897,#105898,
#105899,#105900,#105901,#105902,#105903,#105904,#105905,#105906,#105907,
#105908,#105909,#105910,#105911,#105912,#105913,#105914,#105915,#105916,
#105917,#105918,#105919,#105920,#105921,#105922,#105923,#105924,#105925,
#105926,#105927,#105928,#105929,#105930,#105931,#105932,#105933,#105934,
#105935,#105936,#105937,#105938,#105939,#105940)),.UNSPECIFIED.,.F.,.F.,
 .F.,(4,4),(4,1,1,1,1,1,1,1,1,1,1,1,1,1,1,1,1,1,1,1,1,1,1,1,1,1,1,1,1,1,
1,1,1,1,1,1,1,1,1,1,1,1,1,1,1,1,1,1,1,1,1,1,1,1,1,1,1,1,1,1,1,1,1,1,1,1,
1,1,1,1,1,1,1,1,1,1,1,1,1,1,1,1,1,1,1,1,1,1,1,1,1,1,1,1,1,1,1,1,1,1,1,1,
1,1,1,1,1,1,1,1,1,1,1,1,1,1,1,1,1,1,1,1,1,1,1,1,1,1,1,1,1,1,1,1,1,1,1,1,
1,1,1,1,1,1,1,1,1,1,4),(-0.000239926289433817,0.0336233065451596),(8.30175083273572,
9.2967304331541,10.2914247119998,11.2861189908456,12.2808132696913,13.275507548537,
14.2702018273828,15.2648961062285,16.2595903850742,17.2542846639199,18.2489789427657,
19.2436732216114,20.2383675004571,21.2330617793029,22.2277560581486,23.2224503369943,
24.2171446158401,25.2118388946858,26.2065331735315,27.2012274523773,28.195921731223,
29.1906160100687,30.1853102889144,31.1800045677602,32.1746988466059,33.1693931254516,
34.1640874042974,35.1587816831431,36.1534759619888,37.1481702408346,38.1428645196803,
39.137558798526,40.1322530773718,41.1269473562175,42.1216416350632,43.1163359139089,
44.1110301927547,45.1057244716004,46.1004187504461,47.0951130292919,48.0898073081376,
49.0845015869833,50.0791958658291,51.0738901446748,52.0685844235205,53.0632787023663,
54.057972981212,55.0526672600577,56.0473615389035,57.0420558177492,58.0367500965949,
59.0314443754406,60.0261386542864,61.0208329331321,62.0155272119778,63.0102214908236,
64.0049157696693,64.999610048515,65.9943043273608,66.9889986062065,67.9836928850522,
68.978387163898,69.9730814427437,70.9677757215894,71.9624700004351,72.9571642792809,
73.9518585581266,74.9465528369723,75.9412471158181,76.9359413946638,77.9306356735095,
78.9253299523553,79.920024231201,80.9147185100467,81.9094127888925,82.9041070677382,
83.8988013465839,84.8934956254297,85.8881899042754,86.8828841831211,87.8775784619668,
88.8722727408126,89.8669670196583,90.861661298504,91.8563555773498,92.8510498561955,
93.8457441350412,94.840438413887,95.8351326927327,96.8298269715784,97.8245212504242,
98.8192155292699,99.8139098081156,100.808604086961,101.803298365807,102.797992644653,
103.792686923499,104.787381202344,105.78207548119,106.776769760036,107.771464038881,
108.766158317727,109.760852596573,110.755546875419,111.750241154264,112.74493543311,
113.739629711956,114.734323990802,115.729018269647,116.723712548493,117.718406827339,
118.713101106184,119.70779538503,120.702489663876,121.697183942722,122.691878221567,
123.686572500413,124.681266779259,125.675961058105,126.67065533695,127.665349615796,
128.660043894642,129.654738173488,130.649432452333,131.644126731179,132.638821010025,
133.63351528887,134.628209567716,135.622903846562,136.617598125408,137.612292404253,
138.606986683099,139.601680961945,140.596375240791,141.591069519636,142.585763798482,
143.580458077328,144.575152356173,145.569846635019,146.564540913865,147.559235192711,
148.553929471556,149.548623750402,150.543318029248,151.538012308094,152.532706586939,
153.527400865785,154.522095144631,155.517029349766),.UNSPECIFIED.);
#612=B_SPLINE_SURFACE_WITH_KNOTS('',3,3,((#106045,#106046,#106047,#106048,
#106049,#106050,#106051,#106052,#106053,#106054,#106055,#106056,#106057,
#106058,#106059,#106060,#106061,#106062,#106063,#106064,#106065,#106066,
#106067,#106068,#106069,#106070,#106071,#106072,#106073,#106074,#106075,
#106076,#106077,#106078,#106079,#106080,#106081,#106082,#106083,#106084,
#106085,#106086,#106087,#106088,#106089,#106090,#106091,#106092,#106093,
#106094,#106095,#106096,#106097,#106098,#106099,#106100,#106101,#106102,
#106103,#106104,#106105,#106106,#106107,#106108,#106109,#106110,#106111,
#106112,#106113,#106114,#106115,#106116,#106117,#106118,#106119,#106120,
#106121,#106122,#106123,#106124,#106125,#106126,#106127,#106128,#106129,
#106130,#106131,#106132,#106133,#106134,#106135,#106136,#106137,#106138,
#106139,#106140,#106141,#106142,#106143,#106144,#106145,#106146,#106147,
#106148,#106149,#106150,#106151,#106152,#106153,#106154,#106155,#106156,
#106157,#106158,#106159,#106160,#106161,#106162,#106163,#106164,#106165,
#106166,#106167,#106168,#106169,#106170,#106171,#106172,#106173,#106174,
#106175,#106176,#106177,#106178,#106179,#106180,#106181,#106182,#106183,
#106184,#106185,#106186,#106187,#106188,#106189,#106190,#106191,#106192,
#106193,#106194,#106195),(#106196,#106197,#106198,#106199,#106200,#106201,
#106202,#106203,#106204,#106205,#106206,#106207,#106208,#106209,#106210,
#106211,#106212,#106213,#106214,#106215,#106216,#106217,#106218,#106219,
#106220,#106221,#106222,#106223,#106224,#106225,#106226,#106227,#106228,
#106229,#106230,#106231,#106232,#106233,#106234,#106235,#106236,#106237,
#106238,#106239,#106240,#106241,#106242,#106243,#106244,#106245,#106246,
#106247,#106248,#106249,#106250,#106251,#106252,#106253,#106254,#106255,
#106256,#106257,#106258,#106259,#106260,#106261,#106262,#106263,#106264,
#106265,#106266,#106267,#106268,#106269,#106270,#106271,#106272,#106273,
#106274,#106275,#106276,#106277,#106278,#106279,#106280,#106281,#106282,
#106283,#106284,#106285,#106286,#106287,#106288,#106289,#106290,#106291,
#106292,#106293,#106294,#106295,#106296,#106297,#106298,#106299,#106300,
#106301,#106302,#106303,#106304,#106305,#106306,#106307,#106308,#106309,
#106310,#106311,#106312,#106313,#106314,#106315,#106316,#106317,#106318,
#106319,#106320,#106321,#106322,#106323,#106324,#106325,#106326,#106327,
#106328,#106329,#106330,#106331,#106332,#106333,#106334,#106335,#106336,
#106337,#106338,#106339,#106340,#106341,#106342,#106343,#106344,#106345,
#106346),(#106347,#106348,#106349,#106350,#106351,#106352,#106353,#106354,
#106355,#106356,#106357,#106358,#106359,#106360,#106361,#106362,#106363,
#106364,#106365,#106366,#106367,#106368,#106369,#106370,#106371,#106372,
#106373,#106374,#106375,#106376,#106377,#106378,#106379,#106380,#106381,
#106382,#106383,#106384,#106385,#106386,#106387,#106388,#106389,#106390,
#106391,#106392,#106393,#106394,#106395,#106396,#106397,#106398,#106399,
#106400,#106401,#106402,#106403,#106404,#106405,#106406,#106407,#106408,
#106409,#106410,#106411,#106412,#106413,#106414,#106415,#106416,#106417,
#106418,#106419,#106420,#106421,#106422,#106423,#106424,#106425,#106426,
#106427,#106428,#106429,#106430,#106431,#106432,#106433,#106434,#106435,
#106436,#106437,#106438,#106439,#106440,#106441,#106442,#106443,#106444,
#106445,#106446,#106447,#106448,#106449,#106450,#106451,#106452,#106453,
#106454,#106455,#106456,#106457,#106458,#106459,#106460,#106461,#106462,
#106463,#106464,#106465,#106466,#106467,#106468,#106469,#106470,#106471,
#106472,#106473,#106474,#106475,#106476,#106477,#106478,#106479,#106480,
#106481,#106482,#106483,#106484,#106485,#106486,#106487,#106488,#106489,
#106490,#106491,#106492,#106493,#106494,#106495,#106496,#106497),(#106498,
#106499,#106500,#106501,#106502,#106503,#106504,#106505,#106506,#106507,
#106508,#106509,#106510,#106511,#106512,#106513,#106514,#106515,#106516,
#106517,#106518,#106519,#106520,#106521,#106522,#106523,#106524,#106525,
#106526,#106527,#106528,#106529,#106530,#106531,#106532,#106533,#106534,
#106535,#106536,#106537,#106538,#106539,#106540,#106541,#106542,#106543,
#106544,#106545,#106546,#106547,#106548,#106549,#106550,#106551,#106552,
#106553,#106554,#106555,#106556,#106557,#106558,#106559,#106560,#106561,
#106562,#106563,#106564,#106565,#106566,#106567,#106568,#106569,#106570,
#106571,#106572,#106573,#106574,#106575,#106576,#106577,#106578,#106579,
#106580,#106581,#106582,#106583,#106584,#106585,#106586,#106587,#106588,
#106589,#106590,#106591,#106592,#106593,#106594,#106595,#106596,#106597,
#106598,#106599,#106600,#106601,#106602,#106603,#106604,#106605,#106606,
#106607,#106608,#106609,#106610,#106611,#106612,#106613,#106614,#106615,
#106616,#106617,#106618,#106619,#106620,#106621,#106622,#106623,#106624,
#106625,#106626,#106627,#106628,#106629,#106630,#106631,#106632,#106633,
#106634,#106635,#106636,#106637,#106638,#106639,#106640,#106641,#106642,
#106643,#106644,#106645,#106646,#106647,#106648)),.UNSPECIFIED.,.F.,.F.,
 .F.,(4,4),(4,1,1,1,1,1,1,1,1,1,1,1,1,1,1,1,1,1,1,1,1,1,1,1,1,1,1,1,1,1,
1,1,1,1,1,1,1,1,1,1,1,1,1,1,1,1,1,1,1,1,1,1,1,1,1,1,1,1,1,1,1,1,1,1,1,1,
1,1,1,1,1,1,1,1,1,1,1,1,1,1,1,1,1,1,1,1,1,1,1,1,1,1,1,1,1,1,1,1,1,1,1,1,
1,1,1,1,1,1,1,1,1,1,1,1,1,1,1,1,1,1,1,1,1,1,1,1,1,1,1,1,1,1,1,1,1,1,1,1,
1,1,1,1,1,1,1,1,1,1,4),(-0.000616092092482018,0.0332354813107788),(11.6156998340738,
12.6106340263461,13.6053283051919,14.6000225840376,15.5947168628833,16.589411141729,
17.5841054205748,18.5787996994205,19.5734939782662,20.568188257112,21.5628825359577,
22.5575768148034,23.5522710936492,24.5469653724949,25.5416596513406,26.5363539301864,
27.5310482090321,28.5257424878778,29.5204367667235,30.5151310455693,31.509825324415,
32.5045196032607,33.4992138821065,34.4939081609522,35.4886024397979,36.4832967186437,
37.4779909974894,38.4726852763351,39.4673795551809,40.4620738340266,41.4567681128723,
42.4514623917181,43.4461566705638,44.4408509494095,45.4355452282552,46.430239507101,
47.4249337859467,48.4196280647924,49.4143223436382,50.4090166224839,51.4037109013296,
52.3984051801754,53.3930994590211,54.3877937378668,55.3824880167126,56.3771822955583,
57.371876574404,58.3665708532497,59.3612651320955,60.3559594109412,61.3506536897869,
62.3453479686327,63.3400422474784,64.3347365263241,65.3294308051699,66.3241250840156,
67.3188193628613,68.3135136417071,69.3082079205528,70.3029021993985,71.2975964782443,
72.29229075709,73.2869850359357,74.2816793147815,75.2763735936272,76.2710678724729,
77.2657621513186,78.2604564301644,79.2551507090101,80.2498449878558,81.2445392667016,
82.2392335455473,83.233927824393,84.2286221032388,85.2233163820845,86.2180106609302,
87.2127049397759,88.2073992186217,89.2020934974674,90.1967877763131,91.1914820551589,
92.1861763340046,93.1808706128503,94.1755648916961,95.1702591705418,96.1649534493875,
97.1596477282333,98.154342007079,99.1490362859247,100.14373056477,101.138424843616,
102.133119122462,103.127813401308,104.122507680153,105.117201958999,106.111896237845,
107.106590516691,108.101284795536,109.095979074382,110.090673353228,111.085367632073,
112.080061910919,113.074756189765,114.069450468611,115.064144747456,116.058839026302,
117.053533305148,118.048227583994,119.042921862839,120.037616141685,121.032310420531,
122.027004699377,123.021698978222,124.016393257068,125.011087535914,126.005781814759,
127.000476093605,127.995170372451,128.989864651297,129.984558930142,130.979253208988,
131.973947487834,132.96864176668,133.963336045525,134.958030324371,135.952724603217,
136.947418882062,137.942113160908,138.936807439754,139.9315017186,140.926195997445,
141.920890276291,142.915584555137,143.910278833983,144.904973112828,145.899667391674,
146.89436167052,147.889055949366,148.883750228211,149.878444507057,150.873138785903,
151.867833064748,152.862527343594,153.85722162244,154.851915901286,155.846610180131,
156.841304458977,157.835998737823,158.831090341195),.UNSPECIFIED.);
#1429=B_SPLINE_CURVE_WITH_KNOTS('',3,(#84340,#84341,#84342,#84343,#84344,
#84345,#84346,#84347,#84348,#84349,#84350,#84351,#84352,#84353,#84354,#84355,
#84356,#84357,#84358,#84359,#84360,#84361,#84362,#84363,#84364,#84365,#84366,
#84367,#84368,#84369,#84370,#84371,#84372,#84373,#84374,#84375,#84376,#84377,
#84378,#84379,#84380,#84381,#84382,#84383,#84384,#84385,#84386,#84387,#84388,
#84389,#84390,#84391,#84392,#84393,#84394,#84395,#84396,#84397,#84398,#84399,
#84400,#84401,#84402,#84403,#84404,#84405,#84406,#84407,#84408,#84409),
 .UNSPECIFIED.,.F.,.F.,(4,2,2,2,2,2,2,2,2,2,2,2,2,2,2,2,2,2,2,2,2,2,2,2,
2,2,2,2,2,2,2,2,2,2,4),(2.76421125033917,2.77723201547172,2.77936414641811,
2.78041526769368,2.78124968604004,2.78223337735643,2.78402129528137,2.79321622328922,
2.83823089709693,2.84905302946592,2.85195012161635,2.85366978347659,2.85517171837985,
2.85702938956112,2.86065133867415,2.89285528030678,2.92143673575942,2.92472338498418,
2.92600594046501,2.92688020515189,2.92776295475109,2.92867181547554,2.9312066033969,
2.93465924463195,2.94366503037432,2.96357410075447,2.99173096918496,2.99493755243625,
2.99689366405073,2.99842510750741,3.00010057231402,3.0028156070367,3.01237607072373,
3.02909331213562,3.06016904789425),.UNSPECIFIED.);
#1430=B_SPLINE_CURVE_WITH_KNOTS('',3,(#84412,#84413,#84414,#84415,#84416,
#84417,#84418,#84419,#84420,#84421,#84422,#84423,#84424,#84425,#84426,#84427,
#84428,#84429,#84430,#84431,#84432,#84433,#84434,#84435,#84436,#84437,#84438,
#84439,#84440,#84441,#84442),.UNSPECIFIED.,.F.,.F.,(4,3,3,3,3,3,3,3,3,3,
4),(0.,0.116076982094954,0.232097056693097,0.348088955573432,0.464088864439995,
0.580132969108435,0.696353414548085,0.812667965282534,0.929223837127315,
0.994694278845732,1.12274180646094),.UNSPECIFIED.);
#1431=B_SPLINE_CURVE_WITH_KNOTS('',3,(#84447,#84448,#84449,#84450,#84451,
#84452,#84453,#84454,#84455,#84456,#84457,#84458,#84459,#84460,#84461,#84462,
#84463,#84464,#84465,#84466,#84467,#84468,#84469,#84470,#84471,#84472,#84473,
#84474,#84475,#84476,#84477,#84478,#84479,#84480,#84481,#84482,#84483,#84484,
#84485,#84486,#84487,#84488,#84489,#84490,#84491,#84492,#84493,#84494,#84495,
#84496,#84497,#84498,#84499,#84500,#84501,#84502,#84503,#84504,#84505,#84506,
#84507,#84508,#84509,#84510,#84511,#84512,#84513,#84514,#84515,#84516,#84517,
#84518,#84519,#84520,#84521,#84522,#84523,#84524,#84525,#84526,#84527,#84528,
#84529,#84530,#84531,#84532,#84533,#84534,#84535,#84536,#84537,#84538,#84539,
#84540,#84541,#84542,#84543,#84544,#84545,#84546,#84547,#84548,#84549,#84550,
#84551,#84552,#84553,#84554,#84555,#84556,#84557,#84558,#84559,#84560,#84561,
#84562,#84563,#84564,#84565,#84566,#84567,#84568,#84569,#84570,#84571,#84572,
#84573,#84574,#84575,#84576,#84577,#84578,#84579,#84580,#84581,#84582,#84583,
#84584,#84585,#84586,#84587,#84588,#84589,#84590,#84591,#84592,#84593,#84594,
#84595,#84596,#84597,#84598,#84599,#84600,#84601,#84602,#84603,#84604,#84605,
#84606,#84607,#84608,#84609,#84610,#84611,#84612,#84613,#84614,#84615,#84616,
#84617,#84618,#84619,#84620,#84621,#84622,#84623,#84624,#84625,#84626,#84627,
#84628,#84629,#84630,#84631,#84632,#84633,#84634,#84635,#84636,#84637,#84638,
#84639,#84640,#84641,#84642,#84643,#84644,#84645,#84646,#84647,#84648,#84649,
#84650,#84651,#84652,#84653,#84654,#84655,#84656,#84657,#84658,#84659,#84660),
 .UNSPECIFIED.,.F.,.F.,(4,2,2,2,2,2,2,2,2,2,2,2,2,2,2,2,2,2,2,2,2,2,2,2,
2,2,2,2,2,2,2,2,2,2,2,2,2,2,2,2,2,2,2,2,2,2,2,2,2,2,2,2,2,2,2,2,2,2,2,2,
2,2,2,2,2,2,2,2,2,2,2,2,2,2,2,2,2,2,2,2,2,2,2,2,2,2,2,2,2,2,2,2,2,2,2,2,
2,2,2,2,2,2,2,2,2,2,4),(1.84293212233226,1.84972675322102,1.89363004897352,
1.90253426724827,1.90421589751822,1.90527580132308,1.9061130180743,1.9070948894541,
1.90887607843526,1.91796374894772,1.96157588217745,1.9734275382624,1.97640543895408,
1.97813895591688,1.97963236349955,1.98145336963407,1.98492176112329,2.01127384547126,
2.03291890050351,2.03832564164711,2.048326749289,2.0500660438755,2.0511434476079,
2.05198233428802,2.05295244920587,2.05467801496651,2.06279629205082,2.08110985780627,
2.11599054523974,2.12097348378096,2.12292408285825,2.12434187368452,2.12586235332593,
2.12790854361059,2.13254366392763,2.15218614503713,2.17780798049297,2.19379892891233,
2.19594487901795,2.19700277548369,2.1978394715261,2.19882168401008,2.20060773195666,
2.20981355884135,2.25541638217924,2.26546442898909,2.26831135435854,2.26999727050283,
2.2713438929194,2.27315473618654,2.27658094594453,2.30095979807754,2.32755419651397,
2.33987540445844,2.34188814996879,2.34293155802555,2.34376710176236,2.34476042910123,
2.34659636222363,2.35679143941954,2.38524668656633,2.41008306395605,2.41330020671868,
2.41524359566025,2.41675309473676,2.418392185887,2.42102039518425,2.42997986942142,
2.4452871348725,2.47210216811407,2.47541844504838,2.48584383743905,2.48760480136674,
2.48868922252973,2.48953029356983,2.49050003240097,2.49221452784788,2.50009751299538,
2.51750384842348,2.5534564041636,2.5583405689607,2.56027666589274,2.56169249343251,
2.56321902214452,2.56528780056284,2.57003814006713,2.59059509311346,2.61634377357414,
2.62069829041445,2.6314517094385,2.63322921971431,2.63430640465496,2.635145025162,
2.63609429682987,2.63774973012023,2.64496969787454,2.66005364578665,2.69826158559999,
2.70411087848331,2.7064138930993,2.70781844494032,2.70932809953151,2.71136549642641,
2.71600495017063,2.73580471338088,2.7612174323221,2.76421125033917),
 .UNSPECIFIED.);
#1432=B_SPLINE_CURVE_WITH_KNOTS('',3,(#84661,#84662,#84663,#84664,#84665,
#84666,#84667,#84668,#84669,#84670,#84671,#84672,#84673,#84674,#84675,#84676,
#84677,#84678,#84679,#84680,#84681,#84682,#84683,#84684,#84685,#84686,#84687,
#84688,#84689,#84690,#84691,#84692,#84693,#84694,#84695,#84696,#84697,#84698,
#84699,#84700,#84701,#84702,#84703,#84704,#84705,#84706,#84707,#84708,#84709,
#84710,#84711,#84712,#84713,#84714,#84715,#84716,#84717,#84718,#84719,#84720,
#84721,#84722,#84723,#84724,#84725,#84726,#84727,#84728,#84729,#84730,#84731,
#84732,#84733,#84734,#84735,#84736,#84737,#84738,#84739,#84740,#84741,#84742,
#84743,#84744,#84745,#84746,#84747,#84748,#84749,#84750,#84751,#84752,#84753,
#84754,#84755,#84756,#84757,#84758,#84759,#84760,#84761,#84762,#84763,#84764,
#84765,#84766,#84767,#84768,#84769,#84770,#84771,#84772,#84773,#84774,#84775,
#84776,#84777,#84778,#84779,#84780,#84781,#84782,#84783,#84784,#84785,#84786,
#84787,#84788,#84789,#84790,#84791,#84792,#84793,#84794,#84795,#84796,#84797,
#84798,#84799,#84800,#84801,#84802,#84803,#84804,#84805,#84806,#84807,#84808,
#84809,#84810,#84811,#84812,#84813,#84814,#84815,#84816,#84817,#84818,#84819,
#84820,#84821,#84822,#84823,#84824,#84825,#84826,#84827,#84828,#84829,#84830,
#84831,#84832,#84833,#84834,#84835,#84836,#84837,#84838,#84839,#84840,#84841,
#84842,#84843,#84844,#84845,#84846,#84847,#84848,#84849,#84850,#84851,#84852,
#84853,#84854,#84855,#84856,#84857,#84858,#84859,#84860,#84861,#84862,#84863,
#84864,#84865,#84866,#84867,#84868),.UNSPECIFIED.,.F.,.F.,(4,3,3,3,3,3,
3,3,3,3,3,3,3,3,3,3,3,3,3,3,3,3,3,3,3,3,3,3,3,3,3,3,3,3,3,3,3,3,3,3,3,3,
3,3,3,3,3,3,3,3,3,3,3,3,3,3,3,3,3,3,3,3,3,3,3,3,3,3,3,4),(1.12274180646094,
1.23344303714648,1.34400474281886,1.45447521756778,1.5649025668582,1.675415346116,
1.78596714841024,1.89673028703231,1.98934601636245,1.98938855769146,2.09290450097165,
2.10300342145843,2.21641547630216,2.32971463245747,2.44294544481904,2.55615236718893,
2.66946071373613,2.78281897934694,2.89638843688897,2.98404626656238,2.98408283653719,
3.08824929947587,3.09772634541184,3.21117354665859,3.32451180574917,3.43778560999423,
3.5510393504477,3.66440012200753,3.77781400505187,3.89144367555841,3.9787386776113,
3.97877711538292,4.08250992410144,4.09207993213216,4.2051770493851,4.31815974498299,
4.43107315443572,4.5439623100504,4.6569549041463,4.76999804301306,4.88325740232231,
4.97343231611545,4.97347139422865,5.07727163318845,5.08695471027319,5.20023564231666,
5.31340404657688,5.42650472777391,5.53958238998565,5.65276390933596,5.76599650655475,
5.87944381868563,5.96812747436669,5.96816567307438,6.0720443952783,6.08163892013194,
6.19491039730512,6.30806973027035,6.42116174058675,6.53423114964273,6.64740513625744,
6.76063058862048,6.87407149018942,6.96282142730057,6.96285995192011,7.07055002716601,
7.08522649739166,7.20726927241575,7.32882665127003,7.40592683901607),
 .UNSPECIFIED.);
#1433=B_SPLINE_CURVE_WITH_KNOTS('',3,(#84873,#84874,#84875,#84876,#84877,
#84878,#84879,#84880,#84881,#84882,#84883,#84884,#84885,#84886,#84887,#84888,
#84889,#84890,#84891,#84892,#84893,#84894,#84895,#84896,#84897,#84898,#84899,
#84900,#84901,#84902,#84903,#84904,#84905,#84906,#84907,#84908,#84909,#84910,
#84911,#84912,#84913,#84914,#84915,#84916,#84917,#84918,#84919,#84920,#84921,
#84922,#84923,#84924,#84925,#84926,#84927,#84928,#84929,#84930,#84931,#84932,
#84933,#84934,#84935,#84936,#84937,#84938,#84939,#84940,#84941,#84942,#84943,
#84944,#84945,#84946,#84947,#84948,#84949,#84950,#84951,#84952,#84953,#84954,
#84955,#84956,#84957,#84958,#84959,#84960,#84961,#84962,#84963,#84964,#84965,
#84966,#84967,#84968,#84969,#84970,#84971,#84972,#84973,#84974,#84975,#84976,
#84977,#84978,#84979,#84980,#84981,#84982,#84983,#84984,#84985,#84986,#84987,
#84988,#84989,#84990,#84991,#84992,#84993,#84994,#84995,#84996,#84997,#84998,
#84999,#85000,#85001,#85002,#85003,#85004,#85005,#85006,#85007,#85008,#85009,
#85010,#85011,#85012,#85013,#85014,#85015,#85016,#85017,#85018,#85019,#85020,
#85021,#85022,#85023,#85024,#85025,#85026,#85027,#85028,#85029,#85030,#85031,
#85032,#85033,#85034,#85035,#85036,#85037,#85038,#85039,#85040,#85041,#85042,
#85043,#85044,#85045,#85046,#85047,#85048,#85049,#85050,#85051,#85052,#85053,
#85054,#85055,#85056,#85057,#85058,#85059,#85060,#85061,#85062,#85063,#85064,
#85065,#85066,#85067,#85068,#85069,#85070,#85071,#85072,#85073,#85074,#85075,
#85076,#85077,#85078,#85079,#85080,#85081,#85082,#85083,#85084,#85085,#85086,
#85087,#85088,#85089,#85090,#85091,#85092,#85093,#85094,#85095,#85096,#85097,
#85098),.UNSPECIFIED.,.F.,.F.,(4,2,2,2,2,2,2,2,2,2,2,2,2,2,2,2,2,2,2,2,
2,2,2,2,2,2,2,2,2,2,2,2,2,2,2,2,2,2,2,2,2,2,2,2,2,2,2,2,2,2,2,2,2,2,2,2,
2,2,2,2,2,2,2,2,2,2,2,2,2,2,2,2,2,2,2,2,2,2,2,2,2,2,2,2,2,2,2,2,2,2,2,2,
2,2,2,2,2,2,2,2,2,2,2,2,2,2,2,2,2,2,2,2,4),(0.921387803811605,0.926936758225414,
0.951373435828612,0.954804129395882,0.956617246048519,0.958110270005632,
0.959850259882243,0.962856479766152,0.975079366926509,0.979298190100335,
1.00936617713551,1.02525132937347,1.02835895414191,1.02958776700503,1.03044937020407,
1.03124081678934,1.03255472306991,1.03595728245377,1.05898895715911,1.07817757773221,
1.09572983648825,1.10009857587304,1.10209620322965,1.10360857411728,1.10523801182131,
1.10782317757969,1.1155528309422,1.16382109239489,1.17316224137613,1.17495699305652,
1.17594186589962,1.17677894771174,1.17783525422895,1.17997284248409,1.20478848107481,
1.22082347451628,1.2411536123937,1.24587177542103,1.24793238674917,1.24945505889899,
1.2508688142991,1.25280436776222,1.25769863891246,1.29382767544972,1.31129686844298,
1.31919614341598,1.32090736093341,1.3218740905318,1.32271329120114,1.32379516492506,
1.3255492457444,1.33585272962387,1.36377732188093,1.38901927785068,1.39246754258527,
1.39428454541659,1.39577801246737,1.39751538686612,1.40050929998135,1.41256425465499,
1.41678080299792,1.44711181859249,1.46294864718872,1.46605180321614,1.46728005483372,
1.46814167197881,1.46893344949856,1.47024853535171,1.47365750653068,1.49781380886419,
1.51969966924817,1.53009515824971,1.53676229020505,1.53920193144259,1.54064011778627,
1.54214955195102,1.54412539444957,1.54837552616952,1.56503137066043,1.5956648933522,
1.59975803175512,1.61049786588383,1.61227542886662,1.61335274298968,1.61419339272617,
1.61515160916936,1.61682389224284,1.62414366865277,1.63953154623754,1.6788830119811,
1.68346257349327,1.68534439024082,1.68674465313799,1.68827785157124,1.69039828910737,
1.69546656522473,1.70251767402919,1.73728983718405,1.75607952096858,1.7582557449891,
1.75931975099058,1.76015732887981,1.76113625723186,1.7629039629578,1.77174743009627,
1.81195911880053,1.82704847853715,1.82996837258339,1.83184298204354,1.83334004767241,
1.83503409198855,1.83791243905998,1.84293212233226),.UNSPECIFIED.);
#1434=B_SPLINE_CURVE_WITH_KNOTS('',3,(#85099,#85100,#85101,#85102,#85103,
#85104,#85105,#85106,#85107,#85108,#85109,#85110,#85111,#85112,#85113,#85114,
#85115,#85116,#85117,#85118,#85119,#85120,#85121,#85122,#85123,#85124,#85125,
#85126,#85127,#85128,#85129,#85130,#85131,#85132,#85133,#85134,#85135,#85136,
#85137,#85138,#85139,#85140,#85141,#85142,#85143,#85144,#85145,#85146,#85147,
#85148,#85149,#85150,#85151,#85152,#85153,#85154,#85155,#85156,#85157,#85158,
#85159,#85160,#85161,#85162,#85163,#85164,#85165,#85166,#85167,#85168,#85169,
#85170,#85171,#85172,#85173,#85174,#85175,#85176,#85177,#85178,#85179,#85180,
#85181,#85182,#85183,#85184,#85185,#85186,#85187,#85188,#85189,#85190,#85191,
#85192,#85193,#85194,#85195,#85196,#85197,#85198,#85199,#85200,#85201,#85202,
#85203,#85204,#85205,#85206,#85207,#85208,#85209,#85210,#85211,#85212,#85213,
#85214,#85215,#85216,#85217,#85218,#85219,#85220,#85221,#85222,#85223,#85224,
#85225,#85226,#85227,#85228,#85229,#85230,#85231,#85232,#85233,#85234,#85235,
#85236,#85237,#85238,#85239,#85240,#85241,#85242,#85243,#85244,#85245,#85246,
#85247,#85248,#85249,#85250,#85251,#85252,#85253,#85254,#85255,#85256,#85257,
#85258,#85259,#85260,#85261,#85262,#85263,#85264,#85265,#85266,#85267,#85268,
#85269,#85270,#85271,#85272,#85273,#85274,#85275,#85276,#85277,#85278,#85279,
#85280,#85281,#85282,#85283,#85284,#85285,#85286,#85287,#85288,#85289,#85290,
#85291,#85292,#85293,#85294,#85295,#85296,#85297,#85298,#85299,#85300,#85301,
#85302,#85303,#85304,#85305,#85306,#85307,#85308,#85309,#85310,#85311,#85312,
#85313,#85314,#85315,#85316,#85317,#85318,#85319,#85320,#85321,#85322,#85323,
#85324,#85325,#85326,#85327,#85328),.UNSPECIFIED.,.F.,.F.,(4,2,2,2,2,2,
2,2,2,2,2,2,2,2,2,2,2,2,2,2,2,2,2,2,2,2,2,2,2,2,2,2,2,2,2,2,2,2,2,2,2,2,
2,2,2,2,2,2,2,2,2,2,2,2,2,2,2,2,2,2,2,2,2,2,2,2,2,2,2,2,2,2,2,2,2,2,2,2,
2,2,2,2,2,2,2,2,2,2,2,2,2,2,2,2,2,2,2,2,2,2,2,2,2,2,2,2,2,2,2,2,2,2,2,2,
4),(0.000426663060224215,0.00334372776168892,0.00580548779923299,0.00727670778860057,
0.00871198391145891,0.0103315383843915,0.0128741686173557,0.0203085926939853,
0.0570868697109929,0.0714978925426921,0.0785257927530299,0.0801760904562657,
0.0811289542299877,0.0819704945671239,0.0830555745788977,0.0848588062267121,
0.0962351159769923,0.124063785064045,0.144501615681988,0.148544548354182,
0.150879174383388,0.152958208756853,0.154465811855288,0.155862769167813,
0.157728227317054,0.162314579956924,0.201686626305909,0.217047735981436,
0.224361138723218,0.226033975478501,0.226992862053752,0.227834109826924,
0.228912417961401,0.230692415220932,0.241510509066355,0.244482135005218,
0.271276682493469,0.29205639712943,0.296828998085613,0.298899590976447,
0.300424423771155,0.301836496266812,0.303764032652648,0.308608390476885,
0.345338042413753,0.362412884989664,0.370207396717381,0.371912159294307,
0.372877647242888,0.37371731505439,0.374801833290118,0.376564235549385,
0.387031484103116,0.40087227956388,0.438028661835564,0.44277751871448,0.444843806690825,
0.446367740496281,0.447780588628643,0.449711675069913,0.454577974334288,
0.491047669072744,0.50829002406265,0.51612937759542,0.517837022891107,0.518803123761574,
0.519642776758211,0.52072649754364,0.522485930166044,0.532888793509432,
0.537685758523827,0.565364551675045,0.584238306850816,0.588778130912684,
0.590807702261349,0.592325859451261,0.593748738852321,0.595717826580927,
0.600812133804884,0.633552216646864,0.65343742337661,0.661944835688176,
0.663694087838166,0.664669428112848,0.665507959022381,0.666578467197476,
0.668293955913746,0.677810385494339,0.681259025973914,0.708955282841503,
0.724322315414994,0.733307540591152,0.735939228265369,0.737579590421914,
0.739089652993197,0.741032922774273,0.744248044375697,0.768803454566392,
0.787489297391622,0.805480861800272,0.808788876760162,0.810048993630402,
0.810917125895629,0.811702758296273,0.812984199204998,0.816186915099057,
0.847096413183407,0.873857696524386,0.879947728043436,0.882227479436006,
0.883792101937034,0.88532504005613,0.887523684488924,0.892682153255465,
0.922069490131181),.UNSPECIFIED.);
#1435=B_SPLINE_CURVE_WITH_KNOTS('',3,(#85334,#85335,#85336,#85337),
 .UNSPECIFIED.,.F.,.F.,(4,4),(1.84334373110974,1.8434049874987),
 .UNSPECIFIED.);
#1436=B_SPLINE_CURVE_WITH_KNOTS('',3,(#85338,#85339,#85340,#85341,#85342,
#85343,#85344,#85345,#85346,#85347,#85348,#85349,#85350,#85351,#85352,#85353,
#85354,#85355,#85356,#85357,#85358,#85359,#85360,#85361,#85362,#85363,#85364,
#85365,#85366,#85367,#85368,#85369,#85370,#85371,#85372,#85373,#85374,#85375,
#85376,#85377,#85378,#85379,#85380,#85381,#85382,#85383,#85384,#85385,#85386,
#85387,#85388,#85389,#85390,#85391,#85392,#85393,#85394,#85395,#85396,#85397,
#85398,#85399,#85400,#85401,#85402,#85403,#85404,#85405,#85406,#85407,#85408,
#85409,#85410,#85411,#85412,#85413,#85414,#85415,#85416,#85417,#85418,#85419,
#85420,#85421,#85422,#85423,#85424,#85425,#85426,#85427,#85428,#85429,#85430,
#85431,#85432,#85433,#85434,#85435,#85436,#85437,#85438,#85439,#85440,#85441,
#85442,#85443,#85444,#85445,#85446,#85447,#85448,#85449,#85450,#85451,#85452,
#85453,#85454,#85455,#85456,#85457,#85458,#85459,#85460,#85461,#85462,#85463,
#85464,#85465,#85466,#85467,#85468,#85469,#85470,#85471,#85472,#85473,#85474,
#85475,#85476,#85477,#85478,#85479,#85480,#85481,#85482,#85483,#85484,#85485,
#85486,#85487,#85488,#85489,#85490,#85491,#85492,#85493,#85494,#85495,#85496,
#85497,#85498,#85499,#85500,#85501,#85502,#85503,#85504,#85505,#85506,#85507,
#85508,#85509,#85510,#85511,#85512,#85513,#85514,#85515,#85516,#85517,#85518,
#85519,#85520,#85521,#85522,#85523,#85524,#85525,#85526,#85527,#85528,#85529,
#85530,#85531,#85532,#85533,#85534,#85535,#85536,#85537,#85538,#85539,#85540,
#85541,#85542,#85543,#85544,#85545,#85546,#85547,#85548,#85549,#85550,#85551,
#85552,#85553,#85554,#85555,#85556,#85557,#85558,#85559,#85560,#85561,#85562,
#85563),.UNSPECIFIED.,.F.,.F.,(4,2,2,2,2,2,2,2,2,2,2,2,2,2,2,2,2,2,2,2,
2,2,2,2,2,2,2,2,2,2,2,2,2,2,2,2,2,2,2,2,2,2,2,2,2,2,2,2,2,2,2,2,2,2,2,2,
2,2,2,2,2,2,2,2,2,2,2,2,2,2,2,2,2,2,2,2,2,2,2,2,2,2,2,2,2,2,2,2,2,2,2,2,
2,2,2,2,2,2,2,2,2,2,2,2,2,2,2,2,2,2,2,2,4),(4.54905144340028E-6,0.0041094722612925,
0.00657049432095091,0.00771703352774657,0.00856563552563301,0.00935905819477919,
0.0101513018477034,0.0112525102515206,0.0140957116269979,0.0202980545450212,
0.0571463629281216,0.0746692716473391,0.0790340547558608,0.0810308935860163,
0.0825430852926223,0.0841727321326731,0.0867590920214259,0.0944986618932328,
0.130569489967454,0.145182799602654,0.149899830617738,0.152085823271165,
0.15335599822209,0.154482544528838,0.155315474323859,0.156238600428662,
0.157753602802971,0.162619840773681,0.210861806819959,0.222996281103226,
0.225898028138964,0.227597040939179,0.229093154496347,0.230959537339959,
0.233853109776184,0.248458457689565,0.289122425916873,0.297998275161044,
0.299767493740607,0.300746630223574,0.301583914535132,0.302646990995203,
0.304819680187474,0.322878272352124,0.324540037977519,0.358531980468752,
0.36909426516359,0.371871770213025,0.37354343423058,0.37504400973174,0.376954647423715,
0.379993338243799,0.397512267815056,0.425638329177515,0.441759870436782,
0.444890375655771,0.446122625691342,0.446984755870316,0.447775216055932,
0.449084579933711,0.452460116085028,0.478883733400005,0.509681405675604,
0.515906323967581,0.518204308451354,0.519771780931139,0.521300044481074,
0.523138237493501,0.527755482070769,0.567363111941259,0.582588715178668,
0.58986023005568,0.591528517627079,0.592485562766307,0.593325964847073,
0.594403933394872,0.59618451519723,0.606963369452004,0.611006890031077,
0.641645532284795,0.658301289750189,0.662550377430304,0.664525545119753,
0.6660343825478,0.667673146911211,0.670301678615058,0.678378247575453,0.726218018928619,
0.735537722002927,0.737331071839674,0.738315513007524,0.73915242755395,
0.740208778752125,0.742347299492102,0.757929978258259,0.782837246365346,
0.798045982360694,0.80696640652479,0.809590353565831,0.811228301061834,
0.812737764605744,0.814682524675043,0.817905007259305,0.844149739035602,
0.879397424834421,0.882512753585785,0.883742791169759,0.884604639141543,
0.885395829428673,0.886708359948769,0.890102331529588,0.915669479233778,
0.921387803811605),.UNSPECIFIED.);
#1437=B_SPLINE_CURVE_WITH_KNOTS('',3,(#85565,#85566,#85567,#85568,#85569,
#85570,#85571,#85572,#85573,#85574,#85575,#85576,#85577,#85578,#85579,#85580,
#85581,#85582,#85583,#85584,#85585,#85586,#85587,#85588,#85589,#85590,#85591,
#85592,#85593,#85594,#85595,#85596,#85597,#85598,#85599,#85600,#85601,#85602,
#85603,#85604,#85605,#85606,#85607,#85608,#85609,#85610,#85611,#85612,#85613,
#85614,#85615,#85616,#85617,#85618,#85619,#85620,#85621,#85622,#85623,#85624,
#85625,#85626,#85627,#85628,#85629,#85630,#85631,#85632,#85633,#85634,#85635,
#85636,#85637,#85638,#85639,#85640,#85641,#85642,#85643,#85644,#85645,#85646,
#85647,#85648,#85649,#85650,#85651,#85652,#85653,#85654,#85655,#85656,#85657,
#85658,#85659,#85660,#85661,#85662,#85663,#85664,#85665,#85666,#85667,#85668,
#85669,#85670,#85671,#85672,#85673,#85674,#85675,#85676,#85677,#85678,#85679,
#85680,#85681,#85682,#85683,#85684,#85685,#85686,#85687,#85688,#85689,#85690,
#85691,#85692,#85693,#85694,#85695,#85696,#85697,#85698,#85699,#85700,#85701,
#85702,#85703,#85704,#85705,#85706,#85707,#85708,#85709,#85710,#85711,#85712,
#85713,#85714,#85715,#85716,#85717,#85718,#85719,#85720,#85721,#85722,#85723,
#85724,#85725,#85726,#85727,#85728,#85729,#85730,#85731,#85732,#85733,#85734,
#85735,#85736,#85737,#85738,#85739,#85740,#85741,#85742,#85743,#85744,#85745,
#85746,#85747,#85748,#85749,#85750,#85751,#85752,#85753,#85754,#85755,#85756,
#85757,#85758,#85759,#85760,#85761,#85762,#85763,#85764,#85765,#85766,#85767,
#85768,#85769,#85770,#85771,#85772,#85773,#85774,#85775,#85776,#85777,#85778,
#85779,#85780,#85781,#85782,#85783,#85784,#85785,#85786,#85787,#85788,#85789,
#85790,#85791,#85792,#85793,#85794,#85795,#85796,#85797,#85798,#85799,#85800,
#85801,#85802,#85803,#85804,#85805,#85806,#85807,#85808,#85809,#85810,#85811,
#85812,#85813,#85814),.UNSPECIFIED.,.F.,.F.,(4,2,2,2,2,2,2,2,2,2,2,2,2,
2,2,2,2,2,2,2,2,2,2,2,2,2,2,2,2,2,2,2,2,2,2,2,2,2,2,2,2,2,2,2,2,2,2,2,2,
2,2,2,2,2,2,2,2,2,2,2,2,2,2,2,2,2,2,2,2,2,2,2,2,2,2,2,2,2,2,2,2,2,2,2,2,
2,2,2,2,2,2,2,2,2,2,2,2,2,2,2,2,2,2,2,2,2,2,2,2,2,2,2,2,2,2,2,2,2,2,2,2,
2,2,2,4),(0.922069490131181,0.92220125174563,0.951353304736987,0.954625118117278,
0.955918284162328,0.956706101202181,0.957571992931478,0.958820890154348,
0.962054932510227,0.979247484172206,1.00036945292123,1.02345131949731,1.02664415263097,
1.0285808536907,1.03008993408803,1.03173338397707,1.03437917454588,1.04350453637844,
1.05922352184658,1.08007867971714,1.09888348680942,1.10106046688351,1.10212487690641,
1.10296284130973,1.1039423551793,1.10571125425586,1.11456408315627,1.15488282919892,
1.16986590015639,1.17278119368915,1.17465492521696,1.17615263670132,1.17784886041334,
1.18073449162112,1.19263221391073,1.23748888475154,1.24545914765856,1.24708532537392,
1.24812860072792,1.24896527332474,1.24996139839117,1.25180738041548,1.26219220371598,
1.29185987101013,1.31527353737618,1.31847267636831,1.32041115918665,1.32192041053508,
1.32356281958281,1.32620423043858,1.33528718868746,1.35089906839215,1.38267770403834,
1.3912721222959,1.39293640903918,1.39399132599825,1.39482861099182,1.3958152612933,
1.39761719545511,1.40708742309575,1.45851884214338,1.46378698568197,1.46600360995306,
1.46740011670142,1.46893709676678,1.47107743577679,1.47626536388673,1.48353248270139,
1.50458633090199,1.53510174824096,1.53830950661935,1.53959157107798,1.5403771548807,
1.54124482781781,1.5425035857501,1.54580408246349,1.5637206453313,1.58310976211004,
1.60706307088978,1.61027039268239,1.61221104274299,1.61372032223805,1.61536109321222,
1.61799620218171,1.62702076197512,1.64248692143862,1.67446271177295,1.68306009096076,
1.68472427982311,1.6857790387771,1.68656908530414,1.68657222812386,1.68657530886022,
1.68657812929896,1.68658093692676,1.68658373179912,1.68658651403093,1.68658928366336,
1.6865920407385,1.68659478537549,1.68659751764687,1.68755659423814,1.68925853591206,
1.69138130109429,1.69590718357968,1.70958926057312,1.72872751629385,1.75289560636979,
1.75610588003528,1.75804742952256,1.75955688190076,1.76119731173892,1.76383071174866,
1.77283784978246,1.78825994119835,1.81850986985775,1.82477561214273,1.82952459293217,
1.8310257783573,1.83194604873785,1.83274910090807,1.83358616232252,1.83470060027602,
1.83785306587972,1.84354018446068),.UNSPECIFIED.);
#1438=B_SPLINE_CURVE_WITH_KNOTS('',3,(#85815,#85816,#85817,#85818),
 .UNSPECIFIED.,.F.,.F.,(4,4),(0.000539378737039987,0.000599447974599068),
 .UNSPECIFIED.);
#1439=B_SPLINE_CURVE_WITH_KNOTS('',3,(#85823,#85824,#85825,#85826,#85827,
#85828,#85829,#85830,#85831,#85832,#85833,#85834,#85835,#85836,#85837,#85838,
#85839,#85840,#85841,#85842,#85843,#85844,#85845,#85846,#85847,#85848,#85849,
#85850,#85851,#85852,#85853,#85854,#85855,#85856,#85857,#85858,#85859,#85860,
#85861,#85862,#85863,#85864,#85865,#85866,#85867,#85868,#85869,#85870,#85871,
#85872,#85873,#85874,#85875,#85876,#85877,#85878,#85879,#85880,#85881,#85882,
#85883,#85884,#85885,#85886,#85887,#85888,#85889,#85890,#85891,#85892,#85893,
#85894,#85895,#85896,#85897,#85898,#85899,#85900,#85901,#85902,#85903,#85904,
#85905,#85906,#85907,#85908,#85909,#85910,#85911,#85912,#85913,#85914,#85915,
#85916,#85917,#85918,#85919,#85920,#85921,#85922,#85923,#85924,#85925,#85926,
#85927,#85928,#85929,#85930,#85931,#85932,#85933,#85934,#85935,#85936,#85937,
#85938,#85939,#85940,#85941,#85942,#85943,#85944,#85945,#85946,#85947,#85948,
#85949,#85950,#85951,#85952,#85953,#85954,#85955,#85956,#85957,#85958,#85959,
#85960,#85961,#85962,#85963,#85964,#85965,#85966,#85967,#85968,#85969,#85970,
#85971,#85972,#85973,#85974,#85975,#85976,#85977,#85978,#85979,#85980,#85981,
#85982,#85983,#85984,#85985,#85986,#85987,#85988,#85989,#85990,#85991,#85992,
#85993,#85994,#85995,#85996,#85997,#85998,#85999,#86000,#86001,#86002,#86003,
#86004,#86005,#86006,#86007,#86008,#86009,#86010,#86011,#86012,#86013,#86014,
#86015,#86016,#86017,#86018,#86019,#86020,#86021,#86022,#86023,#86024,#86025,
#86026,#86027,#86028,#86029,#86030,#86031,#86032,#86033,#86034,#86035,#86036,
#86037,#86038,#86039,#86040,#86041,#86042,#86043,#86044,#86045,#86046,#86047,
#86048,#86049,#86050,#86051,#86052,#86053,#86054,#86055,#86056,#86057,#86058,
#86059,#86060,#86061,#86062),.UNSPECIFIED.,.F.,.F.,(4,2,2,2,2,2,2,2,2,2,
2,2,2,2,2,2,2,2,2,2,2,2,2,2,2,2,2,2,2,2,2,2,2,2,2,2,2,2,2,2,2,2,2,2,2,2,
2,2,2,2,2,2,2,2,2,2,2,2,2,2,2,2,2,2,2,2,2,2,2,2,2,2,2,2,2,2,2,2,2,2,2,2,
2,2,2,2,2,2,2,2,2,2,2,2,2,2,2,2,2,2,2,2,2,2,2,2,2,2,2,2,2,2,2,2,2,2,2,2,
2,4),(0.921708299814284,0.921789731266711,0.94590707435828,0.971652614281142,
0.975043877985191,0.976356194554188,0.977147502257003,0.978009700204245,
0.979240615055326,0.982360138460563,0.998362981766927,1.02774351448395,
1.0333326511807,1.04487915695327,1.04783400141833,1.0495625129385,1.05105668939971,
1.05288503461159,1.05638726784014,1.08491818002176,1.11813826540223,1.12111213088128,
1.12223220538517,1.12302961781011,1.12388701080135,1.1250921851985,1.1280509299624,
1.14246814861644,1.16168854550644,1.16954298334344,1.18994376038308,1.19307220768716,
1.19501045022373,1.19651505779055,1.19817327328402,1.20088713256837,1.2107232720813,
1.22831520302462,1.25335771752399,1.26550016535475,1.26733204145147,1.26842534373202,
1.26926803438747,1.27021676249985,1.27184596911428,1.27858159303533,1.29205337294686,
1.3129678169058,1.33571659974108,1.33890185416102,1.34083606715715,1.34234446318853,
1.34398843099019,1.34663783660143,1.35580368006252,1.37162666360741,1.40328457701521,
1.4117186746368,1.41337326519574,1.41442511900194,1.41526206444115,1.41625074633227,
1.41806265135896,1.42773493086101,1.45155602192279,1.48159686249775,1.48479702192268,
1.48673559873559,1.4882446057992,1.48988642553663,1.49252616713353,1.50159589293146,
1.5171748457098,1.54873879091301,1.55757950899064,1.559257930194,1.56031703561855,
1.56115443131396,1.56213745575501,1.56392319429677,1.5730889512963,1.61795557119905,
1.62865978357502,1.63157197593149,1.63327374429509,1.63475600232024,1.63661328644093,
1.6402569547735,1.67010809551642,1.68559854168956,1.70302311104751,1.70518502925304,
1.7062461782991,1.7070578572778,1.707062235329,1.70706655878106,1.70707082867284,
1.70707504605706,1.70707921191129,1.70708332714614,1.70708739269483,1.70709140946424,
1.7070953783664,1.7070993002579,1.70710317601657,1.7071070064775,1.70807797953287,
1.70912532094375,1.71076424036142,1.71390999278722,1.72183028100631,1.76418609796086,
1.7746137816538,1.77749980448296,1.77919566084649,1.78054296907062,1.7823454420134,
1.78572527668427,1.80810802194668,1.84334373110974),.UNSPECIFIED.);
#1440=B_SPLINE_CURVE_WITH_KNOTS('',3,(#86063,#86064,#86065,#86066,#86067,
#86068,#86069,#86070,#86071,#86072,#86073,#86074,#86075,#86076,#86077,#86078,
#86079,#86080,#86081,#86082,#86083,#86084,#86085,#86086,#86087,#86088,#86089,
#86090,#86091,#86092,#86093,#86094,#86095,#86096,#86097,#86098,#86099,#86100,
#86101,#86102,#86103,#86104,#86105,#86106,#86107,#86108,#86109,#86110,#86111,
#86112,#86113,#86114,#86115,#86116,#86117,#86118,#86119,#86120,#86121,#86122,
#86123,#86124,#86125,#86126,#86127,#86128,#86129,#86130,#86131,#86132,#86133,
#86134,#86135,#86136,#86137,#86138,#86139,#86140,#86141,#86142,#86143,#86144,
#86145,#86146,#86147,#86148,#86149,#86150,#86151,#86152,#86153,#86154,#86155,
#86156,#86157,#86158,#86159,#86160,#86161,#86162,#86163,#86164,#86165,#86166,
#86167,#86168,#86169,#86170,#86171,#86172,#86173,#86174,#86175,#86176,#86177,
#86178,#86179,#86180,#86181,#86182,#86183,#86184,#86185,#86186,#86187,#86188,
#86189,#86190,#86191,#86192,#86193,#86194,#86195,#86196,#86197,#86198,#86199,
#86200,#86201,#86202,#86203,#86204,#86205,#86206,#86207,#86208,#86209,#86210,
#86211,#86212,#86213,#86214,#86215,#86216,#86217,#86218,#86219,#86220,#86221,
#86222,#86223,#86224,#86225,#86226,#86227,#86228,#86229,#86230,#86231,#86232,
#86233,#86234,#86235,#86236,#86237,#86238,#86239,#86240,#86241,#86242,#86243,
#86244,#86245,#86246,#86247,#86248,#86249,#86250,#86251,#86252,#86253,#86254,
#86255,#86256,#86257,#86258,#86259,#86260,#86261,#86262,#86263,#86264,#86265,
#86266,#86267,#86268,#86269,#86270,#86271,#86272,#86273,#86274,#86275,#86276,
#86277,#86278,#86279,#86280,#86281,#86282,#86283,#86284),.UNSPECIFIED.,
 .F.,.F.,(4,2,2,2,2,2,2,2,2,2,2,2,2,2,2,2,2,2,2,2,2,2,2,2,2,2,2,2,2,2,2,
2,2,2,2,2,2,2,2,2,2,2,2,2,2,2,2,2,2,2,2,2,2,2,2,2,2,2,2,2,2,2,2,2,2,2,2,
2,2,2,2,2,2,2,2,2,2,2,2,2,2,2,2,2,2,2,2,2,2,2,2,2,2,2,2,2,2,2,2,2,2,2,2,
2,2,2,2,2,2,2,4),(0.000599447974599068,0.0316058343624691,0.0559765062106575,
0.0594065575766221,0.0612199114777653,0.0627134313290408,0.0644543456907345,
0.0674630407632168,0.0797103299225923,0.0838689340102289,0.113979531472804,
0.1259644542748,0.130121023356855,0.132119106774741,0.133722103550208,0.134667972504823,
0.135460246533888,0.136519301770196,0.138600674711707,0.153014955338879,
0.179757526025723,0.199859918933514,0.204550761093584,0.20660675735005,
0.208128831328901,0.209544038389503,0.211484713821694,0.216408393520337,
0.252154743076204,0.269874841602856,0.27784025270698,0.279555874845522,
0.280523658843792,0.281362871268922,0.282443592499416,0.284193516071882,
0.294407151238243,0.324622262655388,0.340095833821893,0.349122682942974,
0.351758123255411,0.353399020355675,0.35490836131806,0.356849013692629,
0.360056151691328,0.388757790755906,0.413625845140476,0.423508107512758,
0.425330280655839,0.426321179919503,0.427157984637327,0.428207136025029,
0.42985287271923,0.438140159811396,0.470089785829843,0.485828253098796,
0.494959683161271,0.497605616320123,0.49924880392347,0.500757407702729,
0.502693169520043,0.505883727193834,0.528897271108723,0.549423171677817,
0.562938892862379,0.569688593767652,0.57131884102101,0.572267789937073,
0.573110413999905,0.574203320701592,0.576033893173099,0.588140420692956,
0.618338736506903,0.637574875924401,0.642159239819632,0.644196328871069,
0.645715244828897,0.647135319990179,0.64909496239278,0.654133365625509,
0.688076099415013,0.713905071715865,0.716564481614196,0.717718906419336,
0.718567639260335,0.719379581544169,0.720797048959808,0.724900360469889,
0.732708270428822,0.735733864282571,0.760472217420362,0.777105431807572,
0.786582605608628,0.789262494582738,0.790913177848279,0.792419661684219,
0.794340356414039,0.797479780449177,0.818310957521071,0.825597637369747,
0.844690401519224,0.859273284321613,0.862249334135628,0.863457303400389,
0.864315189735906,0.865111883286627,0.866229333326279,0.869183841100843,
0.902580934070594,0.921827501307929,0.921911067911426),.UNSPECIFIED.);
#1441=B_SPLINE_CURVE_WITH_KNOTS('',3,(#86289,#86290,#86291,#86292,#86293,
#86294,#86295,#86296,#86297,#86298,#86299,#86300,#86301,#86302,#86303,#86304,
#86305,#86306,#86307,#86308,#86309,#86310,#86311,#86312,#86313,#86314,#86315,
#86316,#86317,#86318,#86319,#86320,#86321,#86322,#86323,#86324,#86325,#86326,
#86327,#86328,#86329,#86330,#86331,#86332,#86333,#86334,#86335,#86336,#86337,
#86338,#86339,#86340,#86341,#86342,#86343,#86344,#86345,#86346,#86347,#86348,
#86349,#86350,#86351,#86352,#86353,#86354,#86355,#86356,#86357,#86358,#86359,
#86360,#86361,#86362,#86363,#86364,#86365,#86366,#86367,#86368,#86369,#86370,
#86371,#86372,#86373,#86374,#86375,#86376,#86377,#86378,#86379,#86380,#86381,
#86382,#86383,#86384,#86385,#86386,#86387,#86388,#86389,#86390,#86391,#86392,
#86393,#86394,#86395,#86396,#86397,#86398,#86399,#86400,#86401,#86402,#86403,
#86404,#86405,#86406,#86407,#86408,#86409,#86410,#86411,#86412,#86413,#86414,
#86415,#86416,#86417,#86418,#86419,#86420,#86421,#86422,#86423,#86424,#86425,
#86426,#86427,#86428,#86429,#86430,#86431,#86432,#86433,#86434,#86435,#86436,
#86437,#86438,#86439,#86440,#86441,#86442,#86443,#86444,#86445,#86446,#86447,
#86448,#86449,#86450,#86451,#86452,#86453,#86454,#86455,#86456,#86457,#86458,
#86459,#86460,#86461,#86462,#86463,#86464,#86465,#86466,#86467,#86468,#86469,
#86470,#86471,#86472,#86473,#86474,#86475,#86476,#86477,#86478,#86479,#86480,
#86481,#86482,#86483,#86484,#86485,#86486,#86487,#86488,#86489,#86490,#86491,
#86492,#86493,#86494,#86495,#86496,#86497,#86498,#86499,#86500,#86501,#86502,
#86503,#86504,#86505,#86506,#86507,#86508,#86509,#86510,#86511,#86512,#86513,
#86514,#86515,#86516,#86517,#86518),.UNSPECIFIED.,.F.,.F.,(4,2,2,2,2,2,
2,2,2,2,2,2,2,2,2,2,2,2,2,2,2,2,2,2,2,2,2,2,2,2,2,2,2,2,2,2,2,2,2,2,2,2,
2,2,2,2,2,2,2,2,2,2,2,2,2,2,2,2,2,2,2,2,2,2,2,2,2,2,2,2,2,2,2,2,2,2,2,2,
2,2,2,2,2,2,2,2,2,2,2,2,2,2,2,2,2,2,2,2,2,2,2,2,2,2,2,2,2,2,2,2,2,2,2,2,
4),(0.000214697203212984,0.0160514925799108,0.0231282367207183,0.0254863851464672,
0.0271276107098235,0.0285295300915837,0.0300305745001698,0.0319418376304527,
0.0349815799780459,0.0525094072768143,0.064162534249541,0.0763414403195431,
0.0916808737339768,0.0989864539099635,0.100657443960427,0.101615233837524,
0.102455755710174,0.103533196016409,0.105311507480465,0.116063282985645,
0.116526333666239,0.144585197536107,0.16498866789945,0.169029260291844,
0.172259618593857,0.174023050365629,0.175501559721651,0.177248191605193,
0.18028319852455,0.192878898492621,0.224836677878989,0.242416819340641,
0.245686354163779,0.246940251979115,0.247806806685877,0.248593076365453,
0.24987951232973,0.253114206518393,0.283318632878354,0.290213340483236,
0.314615176939245,0.31804518230156,0.319858186682743,0.321351247099808,
0.323091426357392,0.326098340072308,0.338329663363518,0.34252944998083,
0.381802540076032,0.390568592898111,0.392331988507076,0.393310021502913,
0.394147673939351,0.395212904663296,0.397395599149604,0.41846926761471,
0.447989135166039,0.461283953489719,0.464266384567512,0.465983461799876,
0.467478195262668,0.469320549325389,0.472134979459764,0.485496686589406,
0.527479398662504,0.536454924390792,0.53823010447395,0.539210742250717,
0.540048203858205,0.541110087276293,0.543275660348879,0.560994786650693,
0.58180503566487,0.60408392751185,0.609030074556835,0.611129977332169,0.612659468916105,
0.614064059631685,0.616326109056425,0.621873214146587,0.660201877032794,
0.675306612768332,0.682543764088235,0.684210122161386,0.685167005928949,
0.686007895483813,0.687087293549919,0.688871888851967,0.699809609921197,
0.703508054607814,0.730498545966056,0.750391612974393,0.75505695456852,
0.757108358999092,0.758629564388107,0.76004577000708,0.762370145589266,
0.768289401515878,0.806216899890256,0.821239691086843,0.828452754316401,
0.830117461666343,0.831074018203979,0.831915033711835,0.832995122419306,
0.834781948020924,0.845770141194436,0.873154912323348,0.898203379129927,
0.901648020116273,0.903464388228047,0.904957984613752,0.906696248962834,
0.909693533631725,0.921708299814284),.UNSPECIFIED.);
#1442=B_SPLINE_CURVE_WITH_KNOTS('',3,(#86519,#86520,#86521,#86522,#86523,
#86524,#86525,#86526,#86527,#86528,#86529,#86530,#86531,#86532,#86533,#86534,
#86535,#86536,#86537,#86538,#86539,#86540,#86541,#86542,#86543,#86544,#86545,
#86546,#86547,#86548,#86549,#86550,#86551,#86552,#86553,#86554,#86555,#86556,
#86557,#86558,#86559,#86560,#86561,#86562,#86563,#86564,#86565,#86566,#86567,
#86568,#86569,#86570,#86571,#86572,#86573,#86574,#86575,#86576,#86577,#86578,
#86579,#86580,#86581,#86582,#86583,#86584,#86585,#86586,#86587,#86588,#86589,
#86590,#86591,#86592,#86593,#86594,#86595,#86596,#86597,#86598,#86599,#86600,
#86601,#86602,#86603,#86604,#86605,#86606,#86607,#86608,#86609,#86610,#86611,
#86612,#86613,#86614,#86615,#86616,#86617,#86618,#86619,#86620,#86621,#86622,
#86623,#86624,#86625,#86626,#86627,#86628,#86629,#86630,#86631,#86632,#86633,
#86634,#86635,#86636,#86637,#86638,#86639,#86640,#86641,#86642,#86643,#86644,
#86645,#86646,#86647,#86648,#86649,#86650,#86651,#86652,#86653,#86654,#86655,
#86656,#86657,#86658,#86659,#86660,#86661,#86662,#86663,#86664,#86665,#86666,
#86667,#86668,#86669,#86670,#86671,#86672,#86673,#86674,#86675,#86676,#86677,
#86678,#86679,#86680,#86681,#86682,#86683,#86684,#86685,#86686,#86687,#86688,
#86689,#86690,#86691,#86692,#86693,#86694,#86695,#86696,#86697,#86698,#86699,
#86700,#86701,#86702,#86703,#86704,#86705,#86706,#86707,#86708,#86709,#86710,
#86711,#86712,#86713,#86714,#86715,#86716,#86717,#86718,#86719,#86720,#86721,
#86722,#86723,#86724,#86725,#86726,#86727,#86728,#86729,#86730,#86731,#86732,
#86733,#86734,#86735,#86736,#86737,#86738,#86739,#86740,#86741,#86742,#86743,
#86744),.UNSPECIFIED.,.F.,.F.,(4,2,2,2,2,2,2,2,2,2,2,2,2,2,2,2,2,2,2,2,
2,2,2,2,2,2,2,2,2,2,2,2,2,2,2,2,2,2,2,2,2,2,2,2,2,2,2,2,2,2,2,2,2,2,2,2,
2,2,2,2,2,2,2,2,2,2,2,2,2,2,2,2,2,2,2,2,2,2,2,2,2,2,2,2,2,2,2,2,2,2,2,2,
2,2,2,2,2,2,2,2,2,2,2,2,2,2,2,2,2,2,2,2,4),(0.921911067911426,0.932057510574157,
0.934924512857622,0.936616411754293,0.937964562576898,0.939773288637249,
0.943181744868466,0.966647054738132,0.998596004945917,1.00688034467127,
1.00852574948545,1.0095747433567,1.01041145525951,1.01140227903129,1.01322441113245,
1.02310817570771,1.04798556341299,1.07669719648176,1.07990303696367,1.08184318333282,
1.08335230447239,1.08499313794199,1.08762886268935,1.09666067905984,1.11214562213073,
1.14268795106139,1.15255376393477,1.15428648229455,1.15536195955285,1.15620058621139,
1.15717166785449,1.15890274818593,1.1671175206504,1.18581259318349,1.22018566656015,
1.22520160674482,1.22715746888381,1.22857647307731,1.23009580462306,1.23213617402151,
1.23673963255853,1.2561292339163,1.28634040710973,1.29823263753587,1.30005521174384,
1.30114572279265,1.3019879577464,1.30293810587292,1.30457408750186,1.31140002537676,
1.32515913252836,1.34334903434381,1.3683395239452,1.37155708646108,1.3735006468175,
1.37501024103969,1.37664939910462,1.37927763419326,1.38823614880114,1.40353720091919,
1.42981948241854,1.4330803026184,1.44410327821361,1.44589133026969,1.44697171891923,
1.44781269366585,1.44876889839803,1.45043232239574,1.45762926841595,1.47260173335774,
1.51026920629644,1.51642618574486,1.51878717278402,1.52021018406596,1.52172698162709,
1.52375215328918,1.52827124515601,1.54698800140676,1.57234872007764,1.58965236270196,
1.59181295230498,1.59287380777954,1.59371115701819,1.59469248550477,1.59647101296352,
1.60550892465014,1.64840323755668,1.66089378565031,1.66392101937986,1.66566578872729,
1.66714425530211,1.66890948400089,1.67214302644645,1.67619197921456,1.69777064272047,
1.7179331817276,1.73547837295413,1.73764117613713,1.73870236080801,1.73953959930982,
1.74052036834784,1.74229679957767,1.75130046012535,1.76796782335889,1.78455164984034,
1.80590713024781,1.8090588792184,1.81098283232641,1.81248929892418,1.81413734079802,
1.81583126495222,1.81831832708071,1.84303969707496),.UNSPECIFIED.);
#1443=B_SPLINE_CURVE_WITH_KNOTS('',3,(#86750,#86751,#86752,#86753,#86754,
#86755,#86756,#86757,#86758,#86759,#86760,#86761,#86762,#86763,#86764,#86765,
#86766,#86767,#86768,#86769,#86770,#86771,#86772,#86773,#86774,#86775,#86776,
#86777,#86778,#86779,#86780,#86781,#86782,#86783,#86784,#86785,#86786,#86787,
#86788,#86789,#86790,#86791,#86792,#86793,#86794,#86795,#86796,#86797,#86798,
#86799,#86800,#86801,#86802,#86803,#86804,#86805,#86806,#86807,#86808,#86809,
#86810,#86811,#86812,#86813,#86814,#86815,#86816,#86817,#86818,#86819,#86820,
#86821,#86822,#86823,#86824,#86825,#86826,#86827,#86828,#86829,#86830,#86831,
#86832,#86833,#86834,#86835,#86836,#86837,#86838,#86839,#86840,#86841,#86842,
#86843,#86844,#86845,#86846,#86847,#86848,#86849,#86850,#86851,#86852,#86853,
#86854,#86855,#86856,#86857,#86858,#86859,#86860,#86861,#86862,#86863,#86864,
#86865,#86866,#86867,#86868,#86869,#86870,#86871,#86872,#86873,#86874,#86875,
#86876,#86877,#86878,#86879,#86880,#86881,#86882,#86883,#86884,#86885,#86886,
#86887,#86888,#86889,#86890,#86891,#86892,#86893,#86894,#86895,#86896,#86897,
#86898,#86899,#86900,#86901,#86902,#86903,#86904,#86905,#86906,#86907,#86908,
#86909,#86910,#86911,#86912,#86913,#86914,#86915,#86916,#86917,#86918,#86919,
#86920,#86921,#86922,#86923,#86924,#86925,#86926,#86927,#86928,#86929,#86930,
#86931,#86932,#86933,#86934,#86935,#86936,#86937,#86938,#86939,#86940,#86941,
#86942,#86943,#86944,#86945,#86946,#86947,#86948,#86949,#86950,#86951,#86952,
#86953,#86954,#86955,#86956,#86957,#86958,#86959,#86960,#86961,#86962,#86963,
#86964,#86965,#86966,#86967,#86968,#86969,#86970,#86971,#86972,#86973,#86974,
#86975,#86976,#86977,#86978,#86979),.UNSPECIFIED.,.F.,.F.,(4,2,2,2,2,2,
2,2,2,2,2,2,2,2,2,2,2,2,2,2,2,2,2,2,2,2,2,2,2,2,2,2,2,2,2,2,2,2,2,2,2,2,
2,2,2,2,2,2,2,2,2,2,2,2,2,2,2,2,2,2,2,2,2,2,2,2,2,2,2,2,2,2,2,2,2,2,2,2,
2,2,2,2,2,2,2,2,2,2,2,2,2,2,2,2,2,2,2,2,2,2,2,2,2,2,2,2,2,2,2,2,2,2,2,2,
4),(0.92195427717175,0.921973901496767,0.923091497504975,0.923888218207204,
0.924746030748282,0.925953709841547,0.928928085237592,0.943495821713098,
0.96262116175145,0.969950594700634,0.990774739088636,0.993914235461341,
0.995834912646202,0.997341347758119,0.998991938783069,1.00167158252704,
1.01114675507128,1.02777167317095,1.05232768032855,1.05543805573243,1.06642651098004,
1.06821325573149,1.06929330504395,1.0701342941729,1.07109081623147,1.07275546648672,
1.07996804917874,1.09499104306598,1.13290083688255,1.13885008560609,1.14117885649958,
1.14259585033082,1.1441164503858,1.14616449979271,1.15081115516655,1.1705500189747,
1.195821202368,1.19825117016901,1.20134648902897,1.21232065881903,1.21410668320771,
1.21518647274568,1.21602736955049,1.21698391217889,1.2186488865979,1.22586738079979,
1.24091111672634,1.27892362046886,1.28477171132582,1.28708490083993,1.28849888763765,
1.2900212475605,1.2920804506833,1.29679103739043,1.33300383179863,1.35607978761377,
1.35948236172438,1.36079641428702,1.36158799010225,1.36244976945527,1.36367889757174,
1.36678763657845,1.39641612445705,1.42578529984481,1.43094638411129,1.43314494150014,
1.4346773998433,1.4362411789582,1.43851904872315,1.44460008363608,1.47098728591634,
1.50229890416152,1.50546721600175,1.50674255959211,1.5075268164188,1.50839565409672,
1.50966062213922,1.51300325793552,1.53138701768706,1.5436707350812,1.57426990749613,
1.57745531446596,1.57938937668403,1.58089750971279,1.58254104393215,1.5851894259368,
1.59434841896075,1.61015540781746,1.64187006155175,1.65026317490606,1.65191508158618,
1.65296600885864,1.65380274865187,1.65479181097718,1.6566060277151,1.66633014598367,
1.69203812347397,1.72010097718476,1.72331179390172,1.72525330143445,1.72676249593133,
1.72816194572898,1.73041863275592,1.73677961569699,1.74635009680969,1.76338637087314,
1.79398356736075,1.79719820347499,1.79848131010894,1.79926700081203,1.80013428333466,
1.80139158082396,1.80468316854952,1.82250352462013,1.84334958263878),
 .UNSPECIFIED.);
#1444=B_SPLINE_CURVE_WITH_KNOTS('',3,(#86980,#86981,#86982,#86983),
 .UNSPECIFIED.,.F.,.F.,(4,4),(8.78772022666079E-5,0.000214697203212984),
 .UNSPECIFIED.);
#1445=B_SPLINE_CURVE_WITH_KNOTS('',3,(#86985,#86986,#86987,#86988),
 .UNSPECIFIED.,.F.,.F.,(4,4),(1.84303969707496,1.84316407965133),
 .UNSPECIFIED.);
#1446=B_SPLINE_CURVE_WITH_KNOTS('',3,(#86989,#86990,#86991,#86992,#86993,
#86994,#86995,#86996,#86997,#86998,#86999,#87000,#87001,#87002,#87003,#87004,
#87005,#87006,#87007,#87008,#87009,#87010,#87011,#87012,#87013,#87014,#87015,
#87016,#87017,#87018,#87019,#87020,#87021,#87022,#87023,#87024,#87025,#87026,
#87027,#87028,#87029,#87030,#87031,#87032,#87033,#87034,#87035,#87036,#87037,
#87038,#87039,#87040,#87041,#87042,#87043,#87044,#87045,#87046,#87047,#87048,
#87049,#87050,#87051,#87052,#87053,#87054,#87055,#87056,#87057,#87058,#87059,
#87060,#87061,#87062,#87063,#87064,#87065,#87066,#87067,#87068,#87069,#87070,
#87071,#87072,#87073,#87074,#87075,#87076,#87077,#87078,#87079,#87080,#87081,
#87082,#87083,#87084,#87085,#87086,#87087,#87088,#87089,#87090,#87091,#87092,
#87093,#87094,#87095,#87096,#87097,#87098,#87099,#87100,#87101,#87102,#87103,
#87104,#87105,#87106,#87107,#87108,#87109,#87110,#87111,#87112,#87113,#87114,
#87115,#87116,#87117,#87118,#87119,#87120,#87121,#87122,#87123,#87124,#87125,
#87126,#87127,#87128,#87129,#87130,#87131,#87132,#87133,#87134,#87135,#87136,
#87137,#87138,#87139,#87140,#87141,#87142,#87143,#87144,#87145,#87146,#87147,
#87148,#87149,#87150,#87151,#87152,#87153,#87154,#87155,#87156,#87157,#87158,
#87159,#87160,#87161,#87162,#87163,#87164,#87165,#87166,#87167,#87168,#87169,
#87170,#87171,#87172,#87173,#87174,#87175,#87176,#87177,#87178,#87179,#87180,
#87181,#87182,#87183,#87184,#87185,#87186,#87187,#87188,#87189,#87190,#87191,
#87192,#87193,#87194,#87195,#87196,#87197,#87198,#87199,#87200,#87201,#87202,
#87203,#87204,#87205,#87206,#87207,#87208,#87209,#87210,#87211,#87212,#87213,
#87214),.UNSPECIFIED.,.F.,.F.,(4,2,2,2,2,2,2,2,2,2,2,2,2,2,2,2,2,2,2,2,
2,2,2,2,2,2,2,2,2,2,2,2,2,2,2,2,2,2,2,2,2,2,2,2,2,2,2,2,2,2,2,2,2,2,2,2,
2,2,2,2,2,2,2,2,2,2,2,2,2,2,2,2,2,2,2,2,2,2,2,2,2,2,2,2,2,2,2,2,2,2,2,2,
2,2,2,2,2,2,2,2,2,2,2,2,2,2,2,2,2,2,2,2,4),(0.000470462646023128,0.0204922171035094,
0.0370988817818748,0.0402772102298867,0.0415173749253083,0.0423814292663502,
0.0431708564645063,0.0444730420352634,0.0478015357351266,0.0757274614132303,
0.0893807207704344,0.10267208687341,0.11076690917383,0.11324041277449,0.114880368170131,
0.116390052885393,0.118332831842172,0.121547132606634,0.149085445589273,
0.175197506194649,0.184994531675472,0.186812592023987,0.187802622633527,
0.188639510290839,0.189689798286327,0.191339207447399,0.199686462941816,
0.234798670915509,0.253357209902113,0.257856429728947,0.259878262423531,
0.261394773566892,0.262819126115341,0.265186139976812,0.271377543846967,
0.308997034944195,0.323961046158831,0.331156460148119,0.332819980688512,
0.33377632313522,0.334617468782666,0.335698151298732,0.337486847122686,
0.348517862090443,0.351878685779993,0.376163572466532,0.400891499282885,
0.404329534038799,0.406144629339743,0.407638314561696,0.409377977551032,
0.412380910472977,0.424549830877153,0.428668744361367,0.468081357076615,
0.476859626329267,0.478624173040981,0.479602680976926,0.480440644346913,
0.481506166891304,0.483689129389093,0.504980698994866,0.534325484471477,
0.547582551545762,0.550563270894803,0.552280375998838,0.553775735554607,
0.555619637621047,0.55843789193154,0.571848538021873,0.613779639160073,
0.622752158449686,0.62452763778718,0.625508565615243,0.626346357012073,
0.627408783422206,0.629575889756567,0.647381669012106,0.683023674088682,
0.690162597246958,0.695279564426719,0.697408478077412,0.698943578004517,
0.700342686913735,0.702572751506658,0.707922497214126,0.746463142660987,
0.761610871730347,0.768861159300485,0.770528798321554,0.771486147849491,
0.772327273494162,0.773406772434223,0.775191127926812,0.786069031016917,
0.789906217462343,0.815990244085093,0.83117387298874,0.840085558060999,
0.842709618298333,0.844348231087091,0.845858713681023,0.847805358567995,
0.851032222503032,0.878548247163884,0.912515951173339,0.915643813755194,
0.916876263137658,0.917738951430209,0.918530260935449,0.919626819211096,
0.921853710912926,0.921871960720837),.UNSPECIFIED.);
#1447=B_SPLINE_CURVE_WITH_KNOTS('',3,(#87220,#87221,#87222,#87223),
 .UNSPECIFIED.,.F.,.F.,(4,4),(1.84335924581655,1.84346799293763),
 .UNSPECIFIED.);
#1448=B_SPLINE_CURVE_WITH_KNOTS('',3,(#87224,#87225,#87226,#87227,#87228,
#87229,#87230,#87231,#87232,#87233,#87234,#87235,#87236,#87237,#87238,#87239,
#87240,#87241,#87242,#87243,#87244,#87245,#87246,#87247,#87248,#87249,#87250,
#87251,#87252,#87253,#87254,#87255,#87256,#87257,#87258,#87259,#87260,#87261,
#87262,#87263,#87264,#87265,#87266,#87267,#87268,#87269,#87270,#87271,#87272,
#87273,#87274,#87275,#87276,#87277,#87278,#87279,#87280,#87281,#87282,#87283,
#87284,#87285,#87286,#87287,#87288,#87289,#87290,#87291,#87292,#87293,#87294,
#87295,#87296,#87297,#87298,#87299,#87300,#87301,#87302,#87303,#87304,#87305,
#87306,#87307,#87308,#87309,#87310,#87311,#87312,#87313,#87314,#87315,#87316,
#87317,#87318,#87319,#87320,#87321,#87322,#87323,#87324,#87325,#87326,#87327,
#87328,#87329,#87330,#87331,#87332,#87333,#87334,#87335,#87336,#87337,#87338,
#87339,#87340,#87341,#87342,#87343,#87344,#87345,#87346,#87347,#87348,#87349,
#87350,#87351,#87352,#87353,#87354,#87355,#87356,#87357,#87358,#87359,#87360,
#87361,#87362,#87363,#87364,#87365,#87366,#87367,#87368,#87369,#87370,#87371,
#87372,#87373,#87374,#87375,#87376,#87377,#87378,#87379,#87380,#87381,#87382,
#87383,#87384,#87385,#87386,#87387,#87388,#87389,#87390,#87391,#87392,#87393,
#87394,#87395,#87396,#87397,#87398,#87399,#87400,#87401,#87402,#87403,#87404,
#87405,#87406,#87407,#87408,#87409,#87410,#87411,#87412,#87413,#87414,#87415,
#87416,#87417,#87418,#87419,#87420,#87421,#87422,#87423,#87424,#87425,#87426,
#87427,#87428,#87429,#87430,#87431,#87432,#87433,#87434,#87435,#87436,#87437,
#87438,#87439,#87440,#87441),.UNSPECIFIED.,.F.,.F.,(4,2,2,2,2,2,2,2,2,2,
2,2,2,2,2,2,2,2,2,2,2,2,2,2,2,2,2,2,2,2,2,2,2,2,2,2,2,2,2,2,2,2,2,2,2,2,
2,2,2,2,2,2,2,2,2,2,2,2,2,2,2,2,2,2,2,2,2,2,2,2,2,2,2,2,2,2,2,2,2,2,2,2,
2,2,2,2,2,2,2,2,2,2,2,2,2,2,2,2,2,2,2,2,2,2,2,2,2,2,4),(0.000501094062160151,
0.020376313225356,0.0377674182519577,0.0456454330718914,0.0473550889202536,
0.0483213823981442,0.0491605029236977,0.050242657749981,0.0519979328477672,
0.0623297296595978,0.0924281345294714,0.107896468141753,0.113871172024639,
0.118286036310736,0.120253520557417,0.121776926225932,0.123189123313575,
0.125119067206428,0.1299811675561,0.171020918051707,0.184829815969152,0.191672049711161,
0.193309194057752,0.194259561477828,0.195101668241075,0.196191588880556,
0.19801227919406,0.209853275385144,0.240238608264144,0.259566931752169,
0.264162484858407,0.266201349363525,0.267720332761023,0.269139562432046,
0.271480685232317,0.27751393626361,0.315309858531276,0.330310639796793,
0.337516802809565,0.339180862070359,0.340137196844317,0.340978117791995,
0.342058213536103,0.343845315306817,0.354844194203893,0.358356964904617,
0.384456646491752,0.405205415292156,0.409973673381514,0.41204302346883,
0.413567176170371,0.414978782742025,0.416905932910184,0.42175060921958,
0.458455869168049,0.475538961250223,0.483334938168772,0.485039458283113,
0.4860047231396,0.486844161090152,0.487928313168206,0.489689949193669,0.500147319720073,
0.530125159039801,0.551073509620668,0.555865492522148,0.55793899498697,
0.559463891338942,0.56087455297108,0.562797889452789,0.567619720314074,
0.604576424633933,0.621494178976928,0.629245445338757,0.630947065048312,
0.631911710767307,0.632751273135275,0.633836456256942,0.635601482843632,
0.646127313574301,0.676036838083129,0.691497983676949,0.700519949852961,
0.703154720605649,0.704795347685613,0.706304535108436,0.708245117099112,
0.71145239864302,0.740886310212513,0.765166140901391,0.774931614962136,
0.776747964858226,0.777737544172118,0.778574332254882,0.779624832536468,
0.781275183543627,0.78964021433028,0.821619046844376,0.842828702128301,
0.847651473401638,0.849730310823131,0.851256137888875,0.852665554840647,
0.8545839515487,0.85937647157219,0.896641722775173,0.902130835318364,0.918790577694836,
0.92195427717175),.UNSPECIFIED.);
#1449=B_SPLINE_CURVE_WITH_KNOTS('',3,(#87443,#87444,#87445,#87446,#87447,
#87448,#87449,#87450,#87451,#87452,#87453,#87454,#87455,#87456,#87457,#87458,
#87459,#87460,#87461,#87462,#87463,#87464,#87465,#87466,#87467,#87468,#87469,
#87470,#87471,#87472,#87473,#87474,#87475,#87476,#87477,#87478,#87479,#87480,
#87481,#87482,#87483,#87484,#87485,#87486,#87487,#87488,#87489,#87490,#87491,
#87492,#87493,#87494,#87495,#87496,#87497,#87498,#87499,#87500,#87501,#87502,
#87503,#87504,#87505,#87506,#87507,#87508,#87509,#87510,#87511,#87512,#87513,
#87514,#87515,#87516,#87517,#87518,#87519,#87520,#87521,#87522,#87523,#87524,
#87525,#87526,#87527,#87528,#87529,#87530,#87531,#87532,#87533,#87534,#87535,
#87536,#87537,#87538,#87539,#87540,#87541,#87542,#87543,#87544,#87545,#87546,
#87547,#87548,#87549,#87550,#87551,#87552,#87553,#87554,#87555,#87556,#87557,
#87558,#87559,#87560,#87561,#87562,#87563,#87564,#87565,#87566,#87567,#87568,
#87569,#87570,#87571,#87572,#87573,#87574,#87575,#87576,#87577,#87578,#87579,
#87580,#87581,#87582,#87583,#87584,#87585,#87586,#87587,#87588,#87589,#87590,
#87591,#87592,#87593,#87594,#87595,#87596,#87597,#87598,#87599,#87600,#87601,
#87602,#87603,#87604,#87605,#87606,#87607,#87608,#87609,#87610,#87611,#87612,
#87613,#87614,#87615,#87616,#87617,#87618,#87619,#87620,#87621,#87622,#87623,
#87624,#87625,#87626,#87627,#87628,#87629,#87630,#87631,#87632,#87633,#87634,
#87635,#87636,#87637,#87638,#87639,#87640,#87641,#87642,#87643,#87644,#87645,
#87646,#87647,#87648,#87649,#87650,#87651,#87652,#87653,#87654,#87655,#87656,
#87657,#87658,#87659,#87660,#87661,#87662,#87663,#87664,#87665,#87666,#87667,
#87668,#87669,#87670,#87671,#87672,#87673,#87674,#87675,#87676,#87677,#87678,
#87679,#87680,#87681,#87682,#87683,#87684,#87685,#87686,#87687,#87688,#87689,
#87690,#87691,#87692,#87693,#87694),.UNSPECIFIED.,.F.,.F.,(4,2,2,2,2,2,
2,2,2,2,2,2,2,2,2,2,2,2,2,2,2,2,2,2,2,2,2,2,2,2,2,2,2,2,2,2,2,2,2,2,2,2,
2,2,2,2,2,2,2,2,2,2,2,2,2,2,2,2,2,2,2,2,2,2,2,2,2,2,2,2,2,2,2,2,2,2,2,2,
2,2,2,2,2,2,2,2,2,2,2,2,2,2,2,2,2,2,2,2,2,2,2,2,2,2,2,2,2,2,2,2,2,2,2,2,
2,2,2,2,2,2,2,2,2,2,2,4),(0.921871960720837,0.949440270215207,0.981844760548665,
0.986952506252835,0.988923574561786,0.990346843202346,0.991864447701091,
0.99389161486827,0.998419030815228,1.0171946820494,1.04409920487034,1.0598501517797,
1.0619912342064,1.06304845733733,1.06388587399885,1.06487069916664,1.06666424384185,
1.07597318287055,1.12350908662567,1.13186598618005,1.13452943703573,1.13617647319092,
1.13768392914491,1.13964435589459,1.14381186007085,1.14930204889285,1.1629327539329,
1.18867677082547,1.19390841509642,1.20593926726569,1.20776703180699,1.20885910858364,
1.20970160953145,1.21065099282944,1.21228327831922,1.2190596204163,1.23266092093696,
1.25258459123235,1.27609284374246,1.2792930387934,1.28123159514816,1.2827405666013,
1.28438233156231,1.28702195934497,1.29609127492545,1.31167038566065,1.34326420112935,
1.35205414982,1.35372962784688,1.3547878219802,1.35562513678774,1.35660882851573,
1.35839773028544,1.36762397273887,1.41358743585898,1.4232923439455,1.42610590256454,
1.42778589124642,1.42913556913536,1.43096070576421,1.43444835877218,1.46197712635463,
1.49247184353942,1.49836368556698,1.49999114651512,1.50093938084243,1.50169750912244,
1.50276260327295,1.50494440575319,1.50781261548173,1.51723526435086,1.53831388440014,
1.56783276627006,1.57102968516615,1.57296712753593,1.57447575041889,1.57611765854942,
1.57875866690053,1.58784430150739,1.60346583626812,1.63530263667441,1.64380952792065,
1.64546820210787,1.64652119473949,1.64735805998754,1.64834551100934,1.65015224444485,
1.65972700100909,1.68463737325803,1.71364856568915,1.71685250923932,1.71879199860814,
1.72030090068092,1.72036734817925,1.72041439853904,1.72044803799979,1.72047225569849,
1.72050602193721,1.72053758851671,1.72056713939904,1.72059483925627,1.72062083588314,
1.72064526226447,1.72066823833742,1.72068987253635,1.72071026311724,1.72072949932219,
1.72074766235311,1.72076482625617,1.72078105871009,1.72079642165799,1.72081097189782,
1.72260456772777,1.7259599289535,1.73020406300406,1.73960705086323,1.75614464028749,
1.78758271474888,1.79073419597156,1.79200670526168,1.79279043246386,1.79365984490964,
1.7949276802637,1.79828966621556,1.81689221546138,1.84313766613365),
 .UNSPECIFIED.);
#1450=B_SPLINE_CURVE_WITH_KNOTS('',3,(#87695,#87696,#87697,#87698),
 .UNSPECIFIED.,.F.,.F.,(4,4),(0.000510341810198537,0.000621055971545034),
 .UNSPECIFIED.);
#1451=B_SPLINE_CURVE_WITH_KNOTS('',3,(#87703,#87704,#87705,#87706,#87707,
#87708,#87709,#87710,#87711,#87712,#87713,#87714,#87715,#87716,#87717,#87718,
#87719,#87720,#87721,#87722,#87723,#87724,#87725,#87726,#87727,#87728,#87729,
#87730,#87731,#87732,#87733,#87734,#87735,#87736,#87737,#87738,#87739,#87740,
#87741,#87742,#87743,#87744,#87745,#87746,#87747,#87748,#87749,#87750,#87751,
#87752,#87753,#87754,#87755,#87756,#87757,#87758,#87759,#87760,#87761,#87762,
#87763,#87764,#87765,#87766,#87767,#87768,#87769,#87770,#87771,#87772,#87773,
#87774,#87775,#87776,#87777,#87778,#87779,#87780,#87781,#87782,#87783,#87784,
#87785,#87786,#87787,#87788,#87789,#87790,#87791,#87792,#87793,#87794,#87795,
#87796,#87797,#87798,#87799,#87800,#87801,#87802,#87803,#87804,#87805,#87806,
#87807,#87808,#87809,#87810,#87811,#87812,#87813,#87814,#87815,#87816,#87817,
#87818,#87819,#87820,#87821,#87822,#87823,#87824,#87825,#87826,#87827,#87828,
#87829,#87830,#87831,#87832,#87833,#87834,#87835,#87836,#87837,#87838,#87839,
#87840,#87841,#87842,#87843,#87844,#87845,#87846,#87847,#87848,#87849,#87850,
#87851,#87852,#87853,#87854,#87855,#87856,#87857,#87858,#87859,#87860,#87861,
#87862,#87863,#87864,#87865,#87866,#87867,#87868,#87869,#87870,#87871,#87872,
#87873,#87874,#87875,#87876,#87877,#87878,#87879,#87880,#87881,#87882,#87883,
#87884,#87885,#87886,#87887,#87888,#87889,#87890,#87891,#87892,#87893,#87894,
#87895,#87896,#87897,#87898,#87899,#87900,#87901,#87902,#87903,#87904,#87905,
#87906,#87907,#87908,#87909,#87910,#87911,#87912,#87913,#87914,#87915,#87916,
#87917,#87918,#87919,#87920,#87921,#87922,#87923,#87924,#87925,#87926),
 .UNSPECIFIED.,.F.,.F.,(4,2,2,2,2,2,2,2,2,2,2,2,2,2,2,2,2,2,2,2,2,2,2,2,
2,2,2,2,2,2,2,2,2,2,2,2,2,2,2,2,2,2,2,2,2,2,2,2,2,2,2,2,2,2,2,2,2,2,2,2,
2,2,2,2,2,2,2,2,2,2,2,2,2,2,2,2,2,2,2,2,2,2,2,2,2,2,2,2,2,2,2,2,2,2,2,2,
2,2,2,2,2,2,2,2,2,2,2,2,2,2,2,4),(0.922109850357463,0.926364499330458,0.938252071945183,
0.941232922345019,0.942967199885786,0.944460690111436,0.946281080107383,
0.949746090750819,0.975891065241991,1.00038381370429,1.00451588356627,1.01329126410738,
1.01496793366453,1.01602636640117,1.01686352074859,1.01784659973918,1.01963329440533,
1.02882316078698,1.0741321101012,1.08442447138741,1.08729761044652,1.08899050727524,
1.09033800296037,1.09214398295239,1.09554109250375,1.11858613723642,1.14790794619228,
1.15898242127555,1.16077230856695,1.16185307932804,1.1626938941529,1.16364937824045,
1.16531029777561,1.17247680882564,1.18734837429602,1.22455924321813,1.23116209350491,
1.23359177536206,1.2350276994089,1.2365373818014,1.23851791453039,1.24279532185581,
1.25965907199514,1.28736898559233,1.30454171988466,1.30670444512319,1.30776555292121,
1.30860270835493,1.30958333616694,1.3113593851968,1.32035799399458,1.36267955028518,
1.37571905933657,1.37878488047906,1.38053817785746,1.38188102092444,1.38361697088017,
1.38668774526506,1.4014515929009,1.43929878506412,1.45067941081909,1.45248164966096,
1.45356595729397,1.45440708781459,1.45536016104177,1.45701058580612,1.464035749906,
1.47844050833185,1.50814651004822,1.52150880430896,1.52432265127615,1.52616449079028,
1.5276587262965,1.52937514250395,1.53235619951655,1.5456414545098,1.57512959381509,
1.59619729556426,1.59837898581387,1.59944379248093,1.60028114570728,1.60125886290403,
1.60302178303157,1.6117869241105,1.65106156349731,1.65523784576473,1.66748879079407,
1.67049639363684,1.67223631714902,1.67372877006225,1.67550444632073,1.67880087165689,
1.6829393562013,1.71244647747798,1.74029634877152,1.74362522015739,1.74492690475812,
1.74571583350044,1.74657915177492,1.74781792265938,1.75099081611581,1.76755352926108,
1.79100855696042,1.80084762855678,1.81326033949228,1.8162813771251,1.81802442210205,
1.81950250627412,1.8209278109473,1.82269097878976,1.82534575354189,1.84335924581655),
 .UNSPECIFIED.);
#1452=B_SPLINE_CURVE_WITH_KNOTS('',3,(#87927,#87928,#87929,#87930,#87931,
#87932,#87933,#87934,#87935,#87936,#87937,#87938,#87939,#87940,#87941,#87942,
#87943,#87944,#87945,#87946,#87947,#87948,#87949,#87950,#87951,#87952,#87953,
#87954,#87955,#87956,#87957,#87958,#87959,#87960,#87961,#87962,#87963,#87964,
#87965,#87966,#87967,#87968,#87969,#87970,#87971,#87972,#87973,#87974,#87975,
#87976,#87977,#87978,#87979,#87980,#87981,#87982,#87983,#87984,#87985,#87986,
#87987,#87988,#87989,#87990,#87991,#87992,#87993,#87994,#87995,#87996,#87997,
#87998,#87999,#88000,#88001,#88002,#88003,#88004,#88005,#88006,#88007,#88008,
#88009,#88010,#88011,#88012,#88013,#88014,#88015,#88016,#88017,#88018,#88019,
#88020,#88021,#88022,#88023,#88024,#88025,#88026,#88027,#88028,#88029,#88030,
#88031,#88032,#88033,#88034,#88035,#88036,#88037,#88038,#88039,#88040,#88041,
#88042,#88043,#88044,#88045,#88046,#88047,#88048,#88049,#88050,#88051,#88052,
#88053,#88054,#88055,#88056,#88057,#88058,#88059,#88060,#88061,#88062,#88063,
#88064,#88065,#88066,#88067,#88068,#88069,#88070,#88071,#88072,#88073,#88074,
#88075,#88076,#88077,#88078,#88079,#88080,#88081,#88082,#88083,#88084,#88085,
#88086,#88087,#88088,#88089,#88090,#88091,#88092,#88093,#88094,#88095,#88096,
#88097,#88098,#88099,#88100,#88101,#88102,#88103,#88104,#88105,#88106,#88107,
#88108,#88109,#88110,#88111,#88112,#88113,#88114,#88115,#88116,#88117,#88118,
#88119,#88120,#88121,#88122,#88123,#88124,#88125,#88126,#88127,#88128,#88129,
#88130,#88131,#88132,#88133,#88134,#88135,#88136,#88137,#88138,#88139,#88140,
#88141,#88142,#88143,#88144,#88145,#88146,#88147,#88148,#88149,#88150,#88151,
#88152,#88153,#88154,#88155,#88156,#88157,#88158,#88159,#88160,#88161,#88162),
 .UNSPECIFIED.,.F.,.F.,(4,2,2,2,2,2,2,2,2,2,2,2,2,2,2,2,2,2,2,2,2,2,2,2,
2,2,2,2,2,2,2,2,2,2,2,2,2,2,2,2,2,2,2,2,2,2,2,2,2,2,2,2,2,2,2,2,2,2,2,2,
2,2,2,2,2,2,2,2,2,2,2,2,2,2,2,2,2,2,2,2,2,2,2,2,2,2,2,2,2,2,2,2,2,2,2,2,
2,2,2,2,2,2,2,2,2,2,2,2,2,2,2,2,2,2,2,2,2,4),(0.000621055971545034,0.0164926796293739,
0.0191424794876196,0.0209040757166634,0.0223297365801582,0.0236773254295353,
0.0253762575001516,0.028274252475158,0.0388233649085059,0.0485458344049959,
0.0682550157821357,0.0852865890181955,0.0930686791312674,0.0947724834768994,
0.0957376949138948,0.0965773200645051,0.0976620404053763,0.0994252519311364,
0.109911090360743,0.114550976110018,0.126268455762736,0.148564967824195,
0.158404387555766,0.162786493138197,0.166240426924207,0.168049692651747,
0.169545187720327,0.17126067029907,0.174158237475727,0.18506807987538,0.191760653128429,
0.220146080575321,0.236670583682186,0.239841072468563,0.241080045847406,
0.241943888771945,0.242733603456548,0.244037204297219,0.247374245808302,
0.275159674935999,0.308505692472417,0.31208412791158,0.313928290823128,
0.315423554641253,0.317140210663372,0.320043200985554,0.331013388873103,
0.337597127611375,0.376013997553858,0.384707558979374,0.386467235801051,
0.387444661494943,0.388282703239985,0.389349619916852,0.391053647525328,
0.400357966284453,0.403997720132482,0.440250011500114,0.455242174118239,
0.45832721935937,0.46006698553238,0.461410802087836,0.463162567746466,0.466218578314965,
0.479100405068117,0.521582509197995,0.530593251180539,0.532370726160038,
0.533352040023926,0.534189720984912,0.535251443584593,0.536938258905477,
0.545927337685542,0.577357008136213,0.592922943615645,0.601986644574306,
0.604625954600122,0.606267793831014,0.607777015550761,0.609716145240351,
0.612917808843082,0.636497281597006,0.641289614579291,0.666172962314351,
0.676350172627506,0.678186413933024,0.679180370145092,0.680017039023202,
0.681062599921189,0.683080837211674,0.6954891002435,0.720222841308283,0.737839819218355,
0.747684069007246,0.750398810713735,0.752057305106886,0.753561999645563,
0.75550012606168,0.758627908359886,0.779009524883296,0.786951119708183,
0.806264450903208,0.820500464269846,0.82344031351037,0.824642442175337,
0.825499329162049,0.8262976042475,0.827420764790109,0.830416803026016,0.863430040095334,
0.882915239736762,0.893418385440269,0.896191831735704,0.897863197372455,
0.899364872648781,0.901278793526907,0.904326494053748,0.921990538769251),
 .UNSPECIFIED.);
#1453=B_SPLINE_CURVE_WITH_KNOTS('',3,(#88167,#88168,#88169,#88170,#88171,
#88172,#88173,#88174,#88175,#88176,#88177,#88178,#88179,#88180,#88181,#88182,
#88183,#88184,#88185,#88186,#88187,#88188,#88189,#88190,#88191,#88192,#88193,
#88194,#88195,#88196,#88197,#88198,#88199,#88200,#88201,#88202,#88203,#88204,
#88205,#88206,#88207,#88208,#88209,#88210,#88211,#88212,#88213,#88214,#88215,
#88216,#88217,#88218,#88219,#88220,#88221,#88222,#88223,#88224,#88225,#88226,
#88227,#88228,#88229,#88230,#88231,#88232,#88233,#88234,#88235,#88236,#88237,
#88238,#88239,#88240,#88241,#88242,#88243,#88244,#88245,#88246,#88247,#88248,
#88249,#88250,#88251,#88252,#88253,#88254,#88255,#88256,#88257,#88258,#88259,
#88260,#88261,#88262,#88263,#88264,#88265,#88266,#88267,#88268,#88269,#88270,
#88271,#88272,#88273,#88274,#88275,#88276,#88277,#88278,#88279,#88280,#88281,
#88282,#88283,#88284,#88285,#88286,#88287,#88288,#88289,#88290,#88291,#88292,
#88293,#88294,#88295,#88296,#88297,#88298,#88299,#88300,#88301,#88302,#88303,
#88304,#88305,#88306,#88307,#88308,#88309,#88310,#88311,#88312,#88313,#88314,
#88315,#88316,#88317,#88318,#88319,#88320,#88321,#88322,#88323,#88324,#88325,
#88326,#88327,#88328,#88329,#88330,#88331,#88332,#88333,#88334,#88335,#88336,
#88337,#88338,#88339,#88340,#88341,#88342,#88343,#88344,#88345,#88346,#88347,
#88348,#88349,#88350,#88351,#88352,#88353,#88354,#88355,#88356,#88357,#88358,
#88359,#88360,#88361,#88362,#88363,#88364,#88365,#88366,#88367,#88368,#88369,
#88370,#88371,#88372,#88373,#88374,#88375,#88376,#88377,#88378,#88379,#88380,
#88381,#88382,#88383,#88384,#88385,#88386,#88387,#88388,#88389,#88390,#88391,
#88392,#88393,#88394,#88395,#88396,#88397,#88398,#88399,#88400,#88401,#88402,
#88403,#88404,#88405,#88406,#88407,#88408,#88409,#88410,#88411,#88412,#88413,
#88414,#88415,#88416,#88417,#88418,#88419,#88420,#88421,#88422,#88423,#88424),
 .UNSPECIFIED.,.F.,.F.,(4,2,2,2,2,2,2,2,2,2,2,2,2,2,2,2,2,2,2,2,2,2,2,2,
2,2,2,2,2,2,2,2,2,2,2,2,2,2,2,2,2,2,2,2,2,2,2,2,2,2,2,2,2,2,2,2,2,2,2,2,
2,2,2,2,2,2,2,2,2,2,2,2,2,2,2,2,2,2,2,2,2,2,2,2,2,2,2,2,2,2,2,2,2,2,2,2,
2,2,2,2,2,2,2,2,2,2,2,2,2,2,2,2,2,2,2,2,2,2,2,2,2,2,2,2,2,2,2,2,4),(0.000580235344661419,
0.0225432725559789,0.0395195756805615,0.0547395813179001,0.0636647592289831,
0.0662893339773771,0.0679275068706122,0.0694370656605665,0.071381791396974,
0.0746038758623836,0.100692516496477,0.134022921254523,0.137186221434361,
0.138831619142547,0.139881618525447,0.140854475675506,0.14085845504871,
0.140862475382216,0.14086653747776,0.140870642194567,0.140874790346985,
0.140878982754138,0.140883220351244,0.140887504057328,0.140891834753636,
0.140896213392345,0.140900640982074,0.140905118533105,0.140909647062502,
0.140914227611597,0.140918861284402,0.140923549246386,0.14092829263095,
0.140933092597562,0.140937950393802,0.140942867296467,0.14094784458359,
0.141762958628665,0.142847246558218,0.144609616366993,0.155049145550168,
0.196770974110713,0.209027001387201,0.211938011948635,0.213639297782944,
0.21513550833927,0.216999514246637,0.219884630711234,0.234360152636289,
0.275172747046177,0.284061267213561,0.285831476204802,0.286810960669843,
0.287648418956745,0.288711557736351,0.290403810357839,0.299499540448613,
0.330229923266626,0.351800758571081,0.356665191279316,0.358750943959766,
0.360277740098149,0.361685174891756,0.363596460974486,0.368348380697992,
0.406003952948499,0.422457822563985,0.430081001629044,0.431773878741676,
0.432736493932439,0.433576193984735,0.434664063183912,0.436438424621314,
0.447137735160929,0.447666166110834,0.488570899497871,0.500829523502527,
0.503740726563205,0.505442057516021,0.506938267048643,0.508802218339132,
0.511687148474593,0.526159803908707,0.56697554561199,0.575864321203696,
0.577634547798976,0.578614037668986,0.579451497902992,0.580514635722414,
0.582686914796312,0.60106129134795,0.627512104316833,0.644443987980966,
0.648730689246205,0.650713189823178,0.652223398067841,0.653659090162944,
0.656086602020193,0.662672843991754,0.699893670327183,0.714764785291494,
0.721932128303132,0.723593308505528,0.724548963585063,0.725389937841757,
0.72647093567088,0.728261248933046,0.739338752603396,0.741691332518053,
0.768807938975371,0.791741189702345,0.795136080787728,0.796941804215888,
0.798420636620535,0.800161852764312,0.80317294626838,0.815457920507041,
0.819529757589767,0.849700462084764,0.865568663206356,0.868674777175894,
0.869903430230972,0.870765069343073,0.871556665839067,0.872871051160187,
0.876276076178247,0.899766057275845,0.922002574267844,0.922109850357463),
 .UNSPECIFIED.);
#1454=B_SPLINE_CURVE_WITH_KNOTS('',3,(#88425,#88426,#88427,#88428,#88429,
#88430,#88431,#88432,#88433,#88434,#88435,#88436,#88437,#88438,#88439,#88440,
#88441,#88442,#88443,#88444,#88445,#88446,#88447,#88448,#88449,#88450,#88451,
#88452,#88453,#88454,#88455,#88456,#88457,#88458,#88459,#88460,#88461,#88462,
#88463,#88464,#88465,#88466,#88467,#88468,#88469,#88470,#88471,#88472,#88473,
#88474,#88475,#88476,#88477,#88478,#88479,#88480,#88481,#88482,#88483,#88484,
#88485,#88486,#88487,#88488,#88489,#88490,#88491,#88492,#88493,#88494,#88495,
#88496,#88497,#88498,#88499,#88500,#88501,#88502,#88503,#88504,#88505,#88506,
#88507,#88508,#88509,#88510,#88511,#88512,#88513,#88514,#88515,#88516,#88517,
#88518,#88519,#88520,#88521,#88522,#88523,#88524,#88525,#88526,#88527,#88528,
#88529,#88530,#88531,#88532,#88533,#88534,#88535,#88536,#88537,#88538,#88539,
#88540,#88541,#88542,#88543,#88544,#88545,#88546,#88547,#88548,#88549,#88550,
#88551,#88552,#88553,#88554,#88555,#88556,#88557,#88558,#88559,#88560,#88561,
#88562,#88563,#88564,#88565,#88566,#88567,#88568,#88569,#88570,#88571,#88572,
#88573,#88574,#88575,#88576,#88577,#88578,#88579,#88580,#88581,#88582,#88583,
#88584,#88585,#88586,#88587,#88588,#88589,#88590,#88591,#88592,#88593,#88594,
#88595,#88596,#88597,#88598,#88599,#88600,#88601,#88602,#88603,#88604,#88605,
#88606,#88607,#88608,#88609,#88610,#88611,#88612,#88613,#88614,#88615,#88616,
#88617,#88618,#88619,#88620,#88621,#88622,#88623,#88624,#88625,#88626,#88627,
#88628,#88629,#88630,#88631,#88632,#88633,#88634,#88635,#88636),
 .UNSPECIFIED.,.F.,.F.,(4,2,2,2,2,2,2,2,2,2,2,2,2,2,2,2,2,2,2,2,2,2,2,2,
2,2,2,2,2,2,2,2,2,2,2,2,2,2,2,2,2,2,2,2,2,2,2,2,2,2,2,2,2,2,2,2,2,2,2,2,
2,2,2,2,2,2,2,2,2,2,2,2,2,2,2,2,2,2,2,2,2,2,2,2,2,2,2,2,2,2,2,2,2,2,2,2,
2,2,2,2,2,2,2,2,2,4),(0.921990538769251,0.922095714747312,0.954066959065241,
0.956951359949483,0.967811963590554,0.969592959807857,0.970671362648303,
0.971512220070758,0.972469925098997,0.974139718874511,0.981423336962385,
0.996687786089568,1.03626819204048,1.04089393363255,1.04273409733647,1.04426345407392,
1.04583149900183,1.0481293137838,1.05434765110521,1.08523431900078,1.11156122215719,
1.11493993802917,1.11625022294177,1.11704114865964,1.1179037117141,1.11913647685773,
1.12226774003668,1.138391386666,1.16660570962418,1.18407355713843,1.1871119728053,
1.18902303553471,1.19052433179077,1.19219720289691,1.1949776762486,1.20556384066999,
1.23969399347116,1.25922201751933,1.26140358689794,1.26246874595402,1.26330657907497,
1.26428510865692,1.2660501378811,1.2748395746389,1.31438580228374,1.31890257055696,
1.33060486333009,1.33357315738072,1.3353046884915,1.33679855930986,1.33862286541939,
1.34210601138453,1.36931958415441,1.39901068159224,1.40586936074096,1.40756671848025,
1.40854049621983,1.4093787857176,1.41045038567129,1.4126648696164,1.41558769301656,
1.42279167537777,1.45471099869009,1.4756146086433,1.47875571621069,1.48067677673975,
1.48218315387718,1.48383331875828,1.48651146728239,1.49597306370812,1.51256421488705,
1.53646255770429,1.55103584297068,1.55311760970949,1.55417665570773,1.55501393149779,
1.55599674841249,1.55778195653453,1.56694195061446,1.61175814102968,1.62248041990789,
1.62535976877521,1.62707059765008,1.62856583555445,1.63041648189668,1.63402848051207,
1.66610736196892,1.6951366279121,1.69840673501729,1.69970258802717,1.70056077746854,
1.70141992685552,1.70268965000434,1.70416224813143,1.7233984861634,1.74484585204786,
1.76723107794458,1.77040721009391,1.77233844050999,1.77384604614888,1.77549071054097,
1.77814469949125,1.78736208417325,1.80332027201119,1.83991647277704,1.84332409142739),
 .UNSPECIFIED.);
#1455=B_SPLINE_CURVE_WITH_KNOTS('',3,(#88642,#88643,#88644,#88645,#88646,
#88647,#88648,#88649,#88650,#88651,#88652,#88653,#88654,#88655,#88656,#88657,
#88658,#88659,#88660,#88661,#88662,#88663,#88664,#88665,#88666,#88667,#88668,
#88669,#88670,#88671,#88672,#88673,#88674,#88675,#88676,#88677,#88678,#88679,
#88680,#88681,#88682,#88683,#88684,#88685,#88686,#88687,#88688,#88689,#88690,
#88691,#88692,#88693,#88694,#88695,#88696,#88697,#88698,#88699,#88700,#88701,
#88702,#88703,#88704,#88705,#88706,#88707,#88708,#88709,#88710,#88711,#88712,
#88713,#88714,#88715,#88716,#88717,#88718,#88719,#88720,#88721,#88722,#88723,
#88724,#88725,#88726,#88727,#88728,#88729,#88730,#88731,#88732,#88733,#88734,
#88735,#88736,#88737,#88738,#88739,#88740,#88741,#88742,#88743,#88744,#88745,
#88746,#88747,#88748,#88749,#88750,#88751,#88752,#88753,#88754,#88755,#88756,
#88757,#88758,#88759,#88760,#88761,#88762,#88763,#88764,#88765,#88766,#88767,
#88768,#88769,#88770,#88771,#88772,#88773,#88774,#88775,#88776,#88777,#88778,
#88779,#88780,#88781,#88782,#88783,#88784,#88785,#88786,#88787,#88788,#88789,
#88790,#88791,#88792,#88793,#88794,#88795,#88796,#88797,#88798,#88799,#88800,
#88801,#88802,#88803,#88804,#88805,#88806,#88807,#88808,#88809,#88810,#88811,
#88812,#88813,#88814,#88815,#88816,#88817,#88818,#88819,#88820,#88821,#88822,
#88823,#88824,#88825,#88826,#88827,#88828,#88829,#88830,#88831,#88832,#88833,
#88834,#88835,#88836,#88837,#88838,#88839,#88840,#88841,#88842,#88843,#88844,
#88845,#88846,#88847,#88848,#88849,#88850,#88851,#88852,#88853,#88854,#88855,
#88856,#88857,#88858,#88859,#88860,#88861,#88862,#88863,#88864,#88865,#88866,
#88867,#88868,#88869),.UNSPECIFIED.,.F.,.F.,(4,2,2,2,2,2,2,2,2,2,2,2,2,
2,2,2,2,2,2,2,2,2,2,2,2,2,2,2,2,2,2,2,2,2,2,2,2,2,2,2,2,2,2,2,2,2,2,2,2,
2,2,2,2,2,2,2,2,2,2,2,2,2,2,2,2,2,2,2,2,2,2,2,2,2,2,2,2,2,2,2,2,2,2,2,2,
2,2,2,2,2,2,2,2,2,2,2,2,2,2,2,2,2,2,2,2,2,2,2,2,2,2,2,2,4),(0.922179861339329,
0.922305856265592,0.948358510328141,0.952471061589414,0.960057621900698,
0.961812599274569,0.962799615103655,0.963636667678953,0.964690587806809,
0.966815796791742,0.990242684552143,1.02785755058805,1.03261781327026,1.03453079875911,
1.03593889508962,1.03746584191979,1.03955078738963,1.04440870119828,1.06591590573847,
1.08588201402429,1.10529634706939,1.10747729341786,1.10854227211977,1.10938001991263,
1.11035849728518,1.11212353476405,1.12091481754642,1.16047210605452,1.16499180419956,
1.17669761125749,1.17966535219894,1.18139666135297,1.18289039691978,1.18471460416134,
1.18819774795401,1.21541593730762,1.2451114789543,1.25197835099754,1.2536763194092,
1.25465018452638,1.25548837095895,1.2565595886586,1.25877241890841,1.26169250881564,
1.26880617547408,1.30007185789791,1.32170910461652,1.32486827489585,1.32679458168917,
1.32830157689105,1.32994885606631,1.33261435486327,1.3419470979786,1.35820130365542,
1.38587320479266,1.39735432297528,1.39916106055838,1.40024688647809,1.40108845891231,
1.40204119731707,1.40368914947989,1.41067542785987,1.42495008116317,1.42943758368689,
1.46528075985601,1.47019886469861,1.47213831365025,1.47355296170009,1.4750747485341,
1.47713091099572,1.48182454587331,1.5019514764184,1.53197077249725,1.53459822760856,
1.54346465885915,1.54514421681024,1.5462035211316,1.54704072643429,1.54802312341557,
1.54980669905122,1.55893855784719,1.60327143654874,1.61444340938124,1.61736501374219,
1.61908547640894,1.62057964540784,1.62241681993276,1.62596378018616,1.6599767204213,
1.68708910933584,1.69044493580093,1.69175123085083,1.69254119999579,1.69338662910514,
1.69458300141436,1.69595131864392,1.69838545976789,1.71975572404526,1.75729822192961,
1.76206257494683,1.76397584026046,1.76538365933871,1.76690984135475,1.7689929087563,
1.77384262506732,1.79528699039251,1.83071308178169,1.83583772328696,1.8373827581069,
1.83831255036784,1.83912037044699,1.83995194488624,1.8410514131662,1.84370654451412),
 .UNSPECIFIED.);
#1456=B_SPLINE_CURVE_WITH_KNOTS('',3,(#88870,#88871,#88872,#88873),
 .UNSPECIFIED.,.F.,.F.,(4,4),(0.000555968474940145,0.000580235344661419),
 .UNSPECIFIED.);
#1457=B_SPLINE_CURVE_WITH_KNOTS('',3,(#88875,#88876,#88877,#88878),
 .UNSPECIFIED.,.F.,.F.,(4,4),(1.84332409142739,1.84334992990566),
 .UNSPECIFIED.);
#1458=B_SPLINE_CURVE_WITH_KNOTS('',3,(#88879,#88880,#88881,#88882,#88883,
#88884,#88885,#88886,#88887,#88888,#88889,#88890,#88891,#88892,#88893,#88894,
#88895,#88896,#88897,#88898,#88899,#88900,#88901,#88902,#88903,#88904,#88905,
#88906,#88907,#88908,#88909,#88910,#88911,#88912,#88913,#88914,#88915,#88916,
#88917,#88918,#88919,#88920,#88921,#88922,#88923,#88924,#88925,#88926,#88927,
#88928,#88929,#88930,#88931,#88932,#88933,#88934,#88935,#88936,#88937,#88938,
#88939,#88940,#88941,#88942,#88943,#88944,#88945,#88946,#88947,#88948,#88949,
#88950,#88951,#88952,#88953,#88954,#88955,#88956,#88957,#88958,#88959,#88960,
#88961,#88962,#88963,#88964,#88965,#88966,#88967,#88968,#88969,#88970,#88971,
#88972,#88973,#88974,#88975,#88976,#88977,#88978,#88979,#88980,#88981,#88982,
#88983,#88984,#88985,#88986,#88987,#88988,#88989,#88990,#88991,#88992,#88993,
#88994,#88995,#88996,#88997,#88998,#88999,#89000,#89001,#89002,#89003,#89004,
#89005,#89006,#89007,#89008,#89009,#89010,#89011,#89012,#89013,#89014,#89015,
#89016,#89017,#89018,#89019,#89020,#89021,#89022,#89023,#89024,#89025,#89026,
#89027,#89028,#89029,#89030,#89031,#89032,#89033,#89034,#89035,#89036,#89037,
#89038,#89039,#89040,#89041,#89042,#89043,#89044,#89045,#89046,#89047,#89048,
#89049,#89050,#89051,#89052,#89053,#89054,#89055,#89056,#89057,#89058,#89059,
#89060,#89061,#89062,#89063,#89064,#89065,#89066,#89067,#89068,#89069,#89070,
#89071,#89072,#89073,#89074,#89075,#89076,#89077,#89078,#89079,#89080,#89081,
#89082,#89083,#89084,#89085,#89086,#89087,#89088,#89089,#89090,#89091,#89092,
#89093,#89094,#89095,#89096,#89097,#89098,#89099,#89100,#89101,#89102,#89103,
#89104),.UNSPECIFIED.,.F.,.F.,(4,2,2,2,2,2,2,2,2,2,2,2,2,2,2,2,2,2,2,2,
2,2,2,2,2,2,2,2,2,2,2,2,2,2,2,2,2,2,2,2,2,2,2,2,2,2,2,2,2,2,2,2,2,2,2,2,
2,2,2,2,2,2,2,2,2,2,2,2,2,2,2,2,2,2,2,2,2,2,2,2,2,2,2,2,2,2,2,2,2,2,2,2,
2,2,2,2,2,2,2,2,2,2,2,2,2,2,2,2,2,2,2,2,4),(0.000558997173511017,0.00118482932324078,
0.00213421037112796,0.00296734761077362,0.00377422552920924,0.00458612664028208,
0.00600328572722705,0.0101047151419729,0.0499071472742641,0.0687509441811788,
0.0732860597346557,0.0753142545984871,0.0768316688740968,0.0782540592719929,
0.0802227984831767,0.0853180886060037,0.117978450357613,0.135225524452579,
0.142596710507808,0.145590045548383,0.147172427392033,0.148196450562901,
0.149149832051276,0.149957577827412,0.151012024863666,0.152675300869839,
0.161257720930523,0.192808992350366,0.216360670874264,0.219771331470604,
0.221580502378189,0.222928673605137,0.224620195985398,0.227485572994004,
0.237699113643811,0.28307311271274,0.292265224587159,0.294052346625034,
0.295035683625365,0.29587307375244,0.296931850412204,0.299011849248387,
0.313228411725894,0.32192560895474,0.339700225554792,0.360195866723772,
0.364934239562936,0.366998639521996,0.368522200395972,0.369935427239762,
0.371868157818852,0.376744432904364,0.413080927379175,0.430403285379708,
0.438263649441004,0.439972597159422,0.440938956990164,0.44177844179225,
0.44286148795803,0.444619045202413,0.454988911676274,0.468911596175963,
0.506079850619068,0.510828502862542,0.512894703262471,0.514418575931632,
0.515831371050421,0.517762392583832,0.522628581453398,0.559083053245657,
0.576326495362742,0.581545280923769,0.5850076798281,0.586290481428787,0.587163146112699,
0.587944538923776,0.589203378250332,0.592272158372798,0.624596620718649,
0.653883098486395,0.657394639692195,0.659225003737515,0.660575529111487,
0.662252712200261,0.665052391168854,0.674622328163887,0.720733300802602,
0.729967378695579,0.731756932043072,0.732740887696176,0.733578366533266,
0.734636696281846,0.736783353185639,0.752769023714274,0.779480604171151,
0.798235249906596,0.802759705631013,0.804786311058138,0.806303795753107,
0.807727167355917,0.80969872078133,0.814809762884154,0.847079575981986,
0.867316992227833,0.875907090064295,0.877660935188146,0.878637156507913,
0.879475434636893,0.880544289616095,0.882254529009274,0.891673459689964,
0.921986581853743,0.922114039327125),.UNSPECIFIED.);
#1459=B_SPLINE_CURVE_WITH_KNOTS('',3,(#89109,#89110,#89111,#89112,#89113,
#89114,#89115,#89116,#89117,#89118,#89119,#89120,#89121,#89122,#89123,#89124,
#89125,#89126,#89127,#89128,#89129,#89130,#89131,#89132,#89133,#89134,#89135,
#89136,#89137,#89138,#89139,#89140,#89141,#89142,#89143,#89144,#89145,#89146,
#89147,#89148,#89149,#89150,#89151,#89152,#89153,#89154,#89155,#89156,#89157,
#89158,#89159,#89160,#89161,#89162,#89163,#89164,#89165,#89166,#89167,#89168,
#89169,#89170,#89171,#89172,#89173,#89174,#89175,#89176,#89177,#89178,#89179,
#89180,#89181,#89182,#89183,#89184,#89185,#89186,#89187,#89188,#89189,#89190,
#89191,#89192,#89193,#89194,#89195,#89196,#89197,#89198,#89199,#89200,#89201,
#89202,#89203,#89204,#89205,#89206,#89207,#89208,#89209,#89210,#89211,#89212,
#89213,#89214,#89215,#89216,#89217,#89218,#89219,#89220,#89221,#89222,#89223,
#89224,#89225,#89226,#89227,#89228,#89229,#89230,#89231,#89232,#89233,#89234,
#89235,#89236,#89237,#89238,#89239,#89240,#89241,#89242,#89243,#89244,#89245,
#89246,#89247,#89248,#89249,#89250,#89251,#89252,#89253,#89254,#89255,#89256,
#89257,#89258,#89259,#89260,#89261,#89262,#89263,#89264,#89265,#89266,#89267,
#89268,#89269,#89270,#89271,#89272,#89273,#89274,#89275,#89276,#89277,#89278,
#89279,#89280,#89281,#89282,#89283,#89284,#89285,#89286,#89287,#89288,#89289,
#89290,#89291,#89292,#89293,#89294,#89295,#89296,#89297,#89298,#89299,#89300,
#89301,#89302,#89303,#89304,#89305,#89306,#89307,#89308,#89309,#89310,#89311,
#89312,#89313,#89314,#89315,#89316,#89317,#89318,#89319,#89320,#89321,#89322,
#89323,#89324,#89325,#89326,#89327,#89328,#89329,#89330,#89331,#89332,#89333,
#89334,#89335,#89336,#89337,#89338),.UNSPECIFIED.,.F.,.F.,(4,2,2,2,2,2,
2,2,2,2,2,2,2,2,2,2,2,2,2,2,2,2,2,2,2,2,2,2,2,2,2,2,2,2,2,2,2,2,2,2,2,2,
2,2,2,2,2,2,2,2,2,2,2,2,2,2,2,2,2,2,2,2,2,2,2,2,2,2,2,2,2,2,2,2,2,2,2,2,
2,2,2,2,2,2,2,2,2,2,2,2,2,2,2,2,2,2,2,2,2,2,2,2,2,2,2,2,2,2,2,2,2,2,2,2,
4),(0.000619400602369933,0.00919608380241888,0.0114757258341164,0.0130852337262251,
0.0144846605649322,0.0159937718795114,0.0179350564357408,0.022114236926196,
0.032031337510015,0.0624021120980362,0.0775989411366287,0.0848628546610285,
0.0865309563306177,0.0874881414695774,0.0883288305791964,0.0894073768571555,
0.0911893428924231,0.10206266955029,0.104991085741233,0.14435892336912,
0.151829607439505,0.155434572654819,0.157591370624042,0.159540601878171,
0.161024931277541,0.162451405275953,0.164831134417604,0.171102925614037,
0.208640876783377,0.223586868379027,0.230776472957122,0.232439230065579,
0.233395219437834,0.2342361054806,0.235316500447613,0.237104806172868,0.248135269445715,
0.251504598009287,0.277703873985716,0.300587409916543,0.303980957542119,
0.305786379850709,0.307265175533071,0.309006593252569,0.312018646113224,
0.324316932097665,0.328354201485825,0.367710139799065,0.376483397917154,
0.378247276673065,0.379225450016874,0.380063143578499,0.381128324899813,
0.383310579784424,0.404976144596082,0.434025501880801,0.447215797656127,
0.450191516252336,0.451907188438811,0.453402150641002,0.455246650255673,
0.458067838523388,0.471532547064675,0.513410537352359,0.522378940464121,
0.524153805453075,0.5251344104456,0.525971930927403,0.527034000333089,0.52920031942802,
0.546975894543856,0.572144314686801,0.590668106169812,0.595162823306987,
0.597183726938314,0.598699971185129,0.600124383781581,0.602100892286698,
0.607245577550293,0.638161720593932,0.647374159833474,0.661533690456628,
0.668485319846315,0.670130821667723,0.671083096507633,0.671924898523636,
0.673011854756539,0.674822217352027,0.686389561780758,0.713977024023634,
0.738224311746537,0.741651456337512,0.743464088741333,0.744812599207838,
0.746501622000406,0.749355633228877,0.759450426431562,0.764306768158382,
0.805280098387922,0.814182389041639,0.815953707955983,0.816933594006844,
0.817771264592479,0.818834504714592,0.821006448222701,0.839293883884213,
0.861414731154785,0.876657580204402,0.885592712470732,0.888218790759248,
0.889857595021026,0.891367528195395,0.893312446747319,0.896534221967008,
0.922179861339329),.UNSPECIFIED.);
#1460=B_SPLINE_CURVE_WITH_KNOTS('',3,(#89339,#89340,#89341,#89342,#89343,
#89344,#89345,#89346,#89347,#89348,#89349,#89350,#89351,#89352,#89353,#89354,
#89355,#89356,#89357,#89358,#89359,#89360,#89361,#89362,#89363,#89364,#89365,
#89366,#89367,#89368,#89369,#89370,#89371,#89372,#89373,#89374,#89375,#89376,
#89377,#89378,#89379,#89380,#89381,#89382,#89383,#89384,#89385,#89386,#89387,
#89388,#89389,#89390,#89391,#89392,#89393,#89394,#89395,#89396,#89397,#89398,
#89399,#89400,#89401,#89402,#89403,#89404,#89405,#89406,#89407,#89408,#89409,
#89410,#89411,#89412,#89413,#89414,#89415,#89416,#89417,#89418,#89419,#89420,
#89421,#89422,#89423,#89424,#89425,#89426,#89427,#89428,#89429,#89430,#89431,
#89432,#89433,#89434,#89435,#89436,#89437,#89438,#89439,#89440,#89441,#89442,
#89443,#89444,#89445,#89446,#89447,#89448,#89449,#89450,#89451,#89452,#89453,
#89454,#89455,#89456,#89457,#89458,#89459,#89460,#89461,#89462,#89463,#89464,
#89465,#89466,#89467,#89468,#89469,#89470,#89471,#89472,#89473,#89474,#89475,
#89476,#89477,#89478,#89479,#89480,#89481,#89482,#89483,#89484,#89485,#89486,
#89487,#89488,#89489,#89490,#89491,#89492,#89493,#89494,#89495,#89496,#89497,
#89498,#89499,#89500,#89501,#89502,#89503,#89504,#89505,#89506,#89507,#89508,
#89509,#89510,#89511,#89512,#89513,#89514,#89515,#89516,#89517,#89518,#89519,
#89520,#89521,#89522,#89523,#89524,#89525,#89526,#89527,#89528,#89529,#89530,
#89531,#89532,#89533,#89534,#89535,#89536,#89537,#89538,#89539,#89540,#89541,
#89542,#89543,#89544,#89545,#89546,#89547,#89548,#89549,#89550,#89551,#89552,
#89553,#89554,#89555,#89556,#89557,#89558,#89559,#89560,#89561,#89562),
 .UNSPECIFIED.,.F.,.F.,(4,2,2,2,2,2,2,2,2,2,2,2,2,2,2,2,2,2,2,2,2,2,2,2,
2,2,2,2,2,2,2,2,2,2,2,2,2,2,2,2,2,2,2,2,2,2,2,2,2,2,2,2,2,2,2,2,2,2,2,2,
2,2,2,2,2,2,2,2,2,2,2,2,2,2,2,2,2,2,2,2,2,2,2,2,2,2,2,2,2,2,2,2,2,2,2,2,
2,2,2,2,2,2,2,2,2,2,2,2,2,2,2,4),(0.922114039327125,0.945624226091696,0.948827213167595,
0.950766787910697,0.95227615166331,0.953917940417018,0.956556719896715,
0.965614224239166,0.98116202678807,1.01246585172647,1.02157084447469,1.02326409805016,
1.02432779940373,1.02516565711389,1.02614557025996,1.02791648355293,1.03680686138869,
1.07761456210416,1.09211817122803,1.09500593533567,1.09687116432286,1.09836805222302,
1.10006978317618,1.10298076015325,1.11522531876594,1.16043282024345,1.16774194722377,
1.16947654246819,1.17045901437327,1.17129662955524,1.17235692037406,1.17451339722148,
1.20075664048657,1.23511087100066,1.24012967632635,1.24208630216522,1.24350574076812,
1.24502542543749,1.24706607401043,1.25166932296381,1.2710526267236,1.30131640882227,
1.31318239624137,1.31500435576094,1.31609483207024,1.31693724471554,1.31788782455129,
1.31952506759398,1.32636376376929,1.34016140203455,1.35787370072324,1.38330156871137,
1.38652234062216,1.38846710080209,1.38997718922515,1.3916164452091,1.39424387758119,
1.4031901839883,1.41845886950231,1.43190817195468,1.45693337690098,1.46033498341433,
1.46164908933463,1.46244082570776,1.46330290638594,1.46453269474231,1.46764433395997,
1.49732463428851,1.52663891927665,1.5317955332396,1.53399368124589,1.53552637060039,
1.53709081954051,1.53937046727338,1.5454611581662,1.57234146806514,1.60308991959664,
1.60629536538627,1.60757714090552,1.60836274426424,1.60923062516734,1.61049000287245,
1.61379392792179,1.63174562065282,1.636085479537,1.67300778850469,1.67783363694066,
1.67975784583906,1.68116889339814,1.68266345697938,1.68466973481214,1.68690709750569,
1.69070946107611,1.71941683777152,1.74891025369856,1.75216760867964,1.7534581787459,
1.75424541769429,1.75511159462619,1.75636249846862,1.75961058599429,1.77695656433478,
1.80811934078148,1.81789037217457,1.82341798093191,1.82567704400571,1.82708129752298,
1.82850450734555,1.82999540875606,1.83196472933021,1.83647854077429,1.84364195192957),
 .UNSPECIFIED.);
#1461=B_SPLINE_CURVE_WITH_KNOTS('',3,(#89568,#89569,#89570,#89571,#89572,
#89573,#89574,#89575,#89576,#89577,#89578,#89579,#89580,#89581,#89582,#89583,
#89584,#89585,#89586,#89587,#89588,#89589,#89590,#89591,#89592,#89593,#89594,
#89595,#89596,#89597,#89598,#89599,#89600,#89601,#89602,#89603,#89604,#89605,
#89606,#89607,#89608,#89609,#89610,#89611,#89612,#89613,#89614,#89615,#89616,
#89617,#89618,#89619,#89620,#89621,#89622,#89623,#89624,#89625,#89626,#89627,
#89628,#89629,#89630,#89631,#89632,#89633,#89634,#89635,#89636,#89637,#89638,
#89639,#89640,#89641,#89642,#89643,#89644,#89645,#89646,#89647,#89648,#89649,
#89650,#89651,#89652,#89653,#89654,#89655,#89656,#89657,#89658,#89659,#89660,
#89661,#89662,#89663,#89664,#89665,#89666,#89667,#89668,#89669,#89670,#89671,
#89672,#89673,#89674,#89675,#89676,#89677,#89678,#89679,#89680,#89681,#89682,
#89683,#89684,#89685,#89686,#89687,#89688,#89689,#89690,#89691,#89692,#89693,
#89694,#89695,#89696,#89697,#89698,#89699,#89700,#89701,#89702,#89703,#89704,
#89705,#89706,#89707,#89708,#89709,#89710,#89711,#89712,#89713,#89714,#89715,
#89716,#89717,#89718,#89719,#89720,#89721,#89722,#89723,#89724,#89725,#89726,
#89727,#89728,#89729,#89730,#89731,#89732,#89733,#89734,#89735,#89736,#89737,
#89738,#89739,#89740,#89741,#89742,#89743,#89744,#89745,#89746,#89747,#89748,
#89749,#89750,#89751,#89752,#89753,#89754,#89755,#89756,#89757,#89758,#89759,
#89760,#89761,#89762,#89763,#89764,#89765,#89766,#89767,#89768,#89769,#89770,
#89771,#89772,#89773,#89774,#89775,#89776,#89777,#89778,#89779,#89780,#89781,
#89782,#89783),.UNSPECIFIED.,.F.,.F.,(4,2,2,2,2,2,2,2,2,2,2,2,2,2,2,2,2,
2,2,2,2,2,2,2,2,2,2,2,2,2,2,2,2,2,2,2,2,2,2,2,2,2,2,2,2,2,2,2,2,2,2,2,2,
2,2,2,2,2,2,2,2,2,2,2,2,2,2,2,2,2,2,2,2,2,2,2,2,2,2,2,2,2,2,2,2,2,2,2,2,
2,2,2,2,2,2,2,2,2,2,2,2,2,2,2,2,2,2,4),(0.921789712209714,0.969516972442617,
0.977663339138593,0.98030092688334,0.981941991943733,0.983450697723574,
0.985422434348305,0.989651431407274,1.00615278638608,1.03785913539119,1.04089646410054,
1.04775715836731,1.05261563440904,1.05412981322882,1.05505282476476,1.05590305395752,
1.0570678273355,1.05978746378977,1.07203033675686,1.10037080861799,1.12195989480259,
1.12511780720191,1.12704370160843,1.12855058745357,1.13019796401356,1.13286410403104,
1.14220414903906,1.15847764038684,1.18594699705429,1.19758809187558,1.19940103590949,
1.20048865537482,1.2013304224424,1.20228202611142,1.20392495737164,1.21084464147499,
1.22490386165016,1.23738994994271,1.26775655083843,1.27094342005437,1.27287782464316,
1.27438589890923,1.27602904006446,1.27867606162792,1.28782295291143,1.30359975283607,
1.33543111750219,1.34375461335686,1.34540221447486,1.34645177873384,1.34728837377195,
1.34827836932085,1.35009716687256,1.35991693227439,1.38447052606481,1.41357562985581,
1.41678799606442,1.41872987235136,1.42023901628632,1.42187854239438,1.42450923567496,
1.43349440273658,1.44886245267503,1.47682714120374,1.48925133127379,1.49126955204612,
1.49231487256587,1.49315122052713,1.49414462176963,1.49597937228689,1.50613467520886,
1.5343491410549,1.55943177379842,1.5626412378287,1.56458222624065,1.56609119464961,
1.56773104676413,1.57036339632274,1.57936548273834,1.59477627473829,1.62381683074958,
1.63517331849145,1.63697493135469,1.63805919866253,1.63890050656631,1.63985401801396,
1.64150574026862,1.64854454731483,1.66299183048334,1.69836402112731,1.70686349647,
1.70954327597369,1.7111935317762,1.71264536435632,1.71452935021861,1.71659050619125,
1.71996237934712,1.72676402910598,1.74567363976231,1.77712948827864,1.78191009300749,
1.78341478036209,1.78433560656666,1.78518656065515,1.78635622180276,1.78910466453662,
1.80160047464782,1.84316778997506),.UNSPECIFIED.);
#1462=B_SPLINE_CURVE_WITH_KNOTS('',3,(#89784,#89785,#89786,#89787),
 .UNSPECIFIED.,.F.,.F.,(4,4),(0.000539904033087321,0.000619400602369933),
 .UNSPECIFIED.);
#1463=B_SPLINE_CURVE_WITH_KNOTS('',3,(#89789,#89790,#89791,#89792),
 .UNSPECIFIED.,.F.,.F.,(4,4),(1.84364195192957,1.84371903373639),
 .UNSPECIFIED.);
#1464=B_SPLINE_CURVE_WITH_KNOTS('',3,(#89793,#89794,#89795,#89796,#89797,
#89798,#89799,#89800,#89801,#89802,#89803,#89804,#89805,#89806,#89807,#89808,
#89809,#89810,#89811,#89812,#89813,#89814,#89815,#89816,#89817,#89818,#89819,
#89820,#89821,#89822,#89823,#89824,#89825,#89826,#89827,#89828,#89829,#89830,
#89831,#89832,#89833,#89834,#89835,#89836,#89837,#89838,#89839,#89840,#89841,
#89842,#89843,#89844,#89845,#89846,#89847,#89848,#89849,#89850,#89851,#89852,
#89853,#89854,#89855,#89856,#89857,#89858,#89859,#89860,#89861,#89862,#89863,
#89864,#89865,#89866,#89867,#89868,#89869,#89870,#89871,#89872,#89873,#89874,
#89875,#89876,#89877,#89878,#89879,#89880,#89881,#89882,#89883,#89884,#89885,
#89886,#89887,#89888,#89889,#89890,#89891,#89892,#89893,#89894,#89895,#89896,
#89897,#89898,#89899,#89900,#89901,#89902,#89903,#89904,#89905,#89906,#89907,
#89908,#89909,#89910,#89911,#89912,#89913,#89914,#89915,#89916,#89917,#89918,
#89919,#89920,#89921,#89922,#89923,#89924,#89925,#89926,#89927,#89928,#89929,
#89930,#89931,#89932,#89933,#89934,#89935,#89936,#89937,#89938,#89939,#89940,
#89941,#89942,#89943,#89944,#89945,#89946,#89947,#89948,#89949,#89950,#89951,
#89952,#89953,#89954,#89955,#89956,#89957,#89958,#89959,#89960,#89961,#89962,
#89963,#89964,#89965,#89966,#89967,#89968,#89969,#89970,#89971,#89972,#89973,
#89974,#89975,#89976,#89977,#89978,#89979,#89980,#89981,#89982,#89983,#89984,
#89985,#89986,#89987,#89988,#89989,#89990,#89991,#89992,#89993,#89994,#89995,
#89996,#89997,#89998,#89999,#90000,#90001,#90002,#90003,#90004),
 .UNSPECIFIED.,.F.,.F.,(4,2,2,2,2,2,2,2,2,2,2,2,2,2,2,2,2,2,2,2,2,2,2,2,
2,2,2,2,2,2,2,2,2,2,2,2,2,2,2,2,2,2,2,2,2,2,2,2,2,2,2,2,2,2,2,2,2,2,2,2,
2,2,2,2,2,2,2,2,2,2,2,2,2,2,2,2,2,2,2,2,2,2,2,2,2,2,2,2,2,2,2,2,2,2,2,2,
2,2,2,2,2,2,2,2,2,4),(0.000533489402586898,0.00397323680534875,0.0450333008082084,
0.0539418411053825,0.0557137595300517,0.056693902620216,0.0575317523610931,
0.0585951874530287,0.0607674367854684,0.0830439982009745,0.111619081738958,
0.120239360693202,0.124230807004118,0.127429296934491,0.129169560833597,
0.130525137239771,0.132226947218926,0.135137666476426,0.145819993136191,
0.19068803890273,0.199852633535366,0.20163865270645,0.202621919678572,0.203459577841137,
0.204519111964732,0.206198411437829,0.215048351287394,0.24661592413807,
0.262200294062169,0.271271785411787,0.273912177051211,0.275554436616223,
0.277063875151419,0.27900304801765,0.282204274750429,0.311416513620761,
0.335887361997227,0.345692028790184,0.347510771624519,0.348501087103721,
0.34933816373541,0.350388623340007,0.352038181978138,0.360383549382576,
0.363199267196655,0.363475251828812,0.393650528935288,0.413775552405436,
0.418469745328183,0.420526662715693,0.422049208562541,0.423464704578996,
0.425783436093726,0.431662420042453,0.469630780813025,0.484662715424888,
0.491879054254956,0.493544390366178,0.494501294783121,0.49534261352143,
0.496423107518798,0.4982106451861,0.509205696583877,0.511730426493795,0.540834664335965,
0.559884502852041,0.564446383613359,0.566479881656849,0.567998637114707,
0.569420382840689,0.57177202267251,0.577868671527939,0.628203211064114,
0.637634008862099,0.639434289901172,0.640420768144195,0.641258348674152,
0.642314204333238,0.643981027453988,0.652612140878818,0.696826390533408,
0.708672631895328,0.711554932428218,0.713250689886008,0.714748899817381,
0.716624459510588,0.719544900341177,0.734616558799752,0.7748370878581,0.783682368437372,
0.785451084588931,0.786430684444065,0.787268828320787,0.788333610964954,
0.790511839375826,0.809397958946926,0.844119637683016,0.851167052438432,
0.856233481611442,0.858354303975419,0.859888198561486,0.861289382925383,
0.863172869886759,0.86775866705016,0.906923387391549,0.922374656735376),
 .UNSPECIFIED.);
#1465=B_SPLINE_CURVE_WITH_KNOTS('',3,(#90010,#90011,#90012,#90013),
 .UNSPECIFIED.,.F.,.F.,(4,4),(1.84368667532253,1.8438184773998),
 .UNSPECIFIED.);
#1466=B_SPLINE_CURVE_WITH_KNOTS('',3,(#90014,#90015,#90016,#90017,#90018,
#90019,#90020,#90021,#90022,#90023,#90024,#90025,#90026,#90027,#90028,#90029,
#90030,#90031,#90032,#90033,#90034,#90035,#90036,#90037,#90038,#90039,#90040,
#90041,#90042,#90043,#90044,#90045,#90046,#90047,#90048,#90049,#90050,#90051,
#90052,#90053,#90054,#90055,#90056,#90057,#90058,#90059,#90060,#90061,#90062,
#90063,#90064,#90065,#90066,#90067,#90068,#90069,#90070,#90071,#90072,#90073,
#90074,#90075,#90076,#90077,#90078,#90079,#90080,#90081,#90082,#90083,#90084,
#90085,#90086,#90087,#90088,#90089,#90090,#90091,#90092,#90093,#90094,#90095,
#90096,#90097,#90098,#90099,#90100,#90101,#90102,#90103,#90104,#90105,#90106,
#90107,#90108,#90109,#90110,#90111,#90112,#90113,#90114,#90115,#90116,#90117,
#90118,#90119,#90120,#90121,#90122,#90123,#90124,#90125,#90126,#90127,#90128,
#90129,#90130,#90131,#90132,#90133,#90134,#90135,#90136,#90137,#90138,#90139,
#90140,#90141,#90142,#90143,#90144,#90145,#90146,#90147,#90148,#90149,#90150,
#90151,#90152,#90153,#90154,#90155,#90156,#90157,#90158,#90159,#90160,#90161,
#90162,#90163,#90164,#90165,#90166,#90167,#90168,#90169,#90170,#90171,#90172,
#90173,#90174,#90175,#90176,#90177,#90178,#90179,#90180,#90181,#90182,#90183,
#90184,#90185,#90186,#90187,#90188,#90189,#90190,#90191,#90192,#90193,#90194,
#90195,#90196,#90197,#90198,#90199,#90200,#90201,#90202,#90203,#90204,#90205,
#90206,#90207,#90208,#90209,#90210,#90211,#90212,#90213,#90214,#90215,#90216,
#90217,#90218,#90219,#90220,#90221,#90222,#90223,#90224,#90225,#90226,#90227,
#90228,#90229,#90230,#90231,#90232,#90233,#90234,#90235,#90236,#90237,#90238,
#90239,#90240,#90241,#90242,#90243,#90244,#90245,#90246,#90247,#90248,#90249),
 .UNSPECIFIED.,.F.,.F.,(4,2,2,2,2,2,2,2,2,2,2,2,2,2,2,2,2,2,2,2,2,2,2,2,
2,2,2,2,2,2,2,2,2,2,2,2,2,2,2,2,2,2,2,2,2,2,2,2,2,2,2,2,2,2,2,2,2,2,2,2,
2,2,2,2,2,2,2,2,2,2,2,2,2,2,2,2,2,2,2,2,2,2,2,2,2,2,2,2,2,2,2,2,2,2,2,2,
2,2,2,2,2,2,2,2,2,2,2,2,2,2,2,2,2,2,2,2,2,4),(0.000428601095637824,0.0290350720482551,
0.0310841819515501,0.0327551988883566,0.0337130083902071,0.0345535502786231,
0.035631019808094,0.0374093868099898,0.0481615772158818,0.052273716103244,
0.0633512603638037,0.0779198501948231,0.0939925952084204,0.102368644220221,
0.104285408891655,0.10609096576465,0.107569831301646,0.109311284196931,
0.112323280422703,0.124619526983771,0.128663680243591,0.151709828378808,
0.168993846101592,0.176832292301315,0.178505195061469,0.179484114210167,
0.180321684728525,0.181385730962344,0.183562411614655,0.202405249323511,
0.237148968204392,0.244197114676824,0.249263233919308,0.251383143293465,
0.252916089687658,0.254316207588198,0.256197956259698,0.260777985643243,
0.299949942379356,0.315453627400328,0.322807234262837,0.324481682479458,
0.325440275484734,0.32628072187121,0.327357070578448,0.329131545820094,
0.339831722679084,0.370663704004278,0.390652070736079,0.395328681362214,
0.397381885791505,0.398903211540054,0.400318661621551,0.402261132942787,
0.407197060087205,0.44278754201314,0.46062088966577,0.468615690863605,0.470332910568821,
0.471300903210197,0.472139846870594,0.473219614828353,0.47496680066878,
0.485129051628043,0.515401408395332,0.5363681559274,0.541162094246406,0.543235818247271,
0.544760642467246,0.54617107159134,0.548093835201716,0.552912888917977,
0.589890950744903,0.606790729815376,0.614536808700958,0.616237974443752,
0.617202464867521,0.618041958229898,0.619127139038517,0.620892333209406,
0.631423872921794,0.634149845871044,0.662979035413663,0.682509765140976,
0.687130445788821,0.689173827656646,0.690693595391687,0.692111701775473,
0.694064267219357,0.699060487314966,0.733771606940388,0.752221611976676,
0.760375272421964,0.762102516929666,0.76307273267756,0.763911419005878,
0.764988011738607,0.76672453738627,0.776666919767031,0.782267392838599,
0.805552082362621,0.830236133881733,0.833672823773881,0.835487424329227,
0.836836098482247,0.838523634673806,0.841371031067518,0.851398146492318,
0.857491623107137,0.897392444028762,0.906210872114216,0.907977458172426,
0.908956294707278,0.909794037565089,0.910858615021977,0.91255519161423,
0.921724077110065,0.921789712209714),.UNSPECIFIED.);
#1467=B_SPLINE_CURVE_WITH_KNOTS('',3,(#90251,#90252,#90253,#90254,#90255,
#90256,#90257,#90258,#90259,#90260,#90261,#90262,#90263,#90264,#90265,#90266,
#90267,#90268,#90269,#90270,#90271,#90272,#90273,#90274,#90275,#90276,#90277,
#90278,#90279,#90280,#90281,#90282,#90283,#90284,#90285,#90286,#90287,#90288,
#90289,#90290,#90291,#90292,#90293,#90294,#90295,#90296,#90297,#90298,#90299,
#90300,#90301,#90302,#90303,#90304,#90305,#90306,#90307,#90308,#90309,#90310,
#90311,#90312,#90313,#90314,#90315,#90316,#90317,#90318,#90319,#90320,#90321,
#90322,#90323,#90324,#90325,#90326,#90327,#90328,#90329,#90330,#90331,#90332,
#90333,#90334,#90335,#90336,#90337,#90338,#90339,#90340,#90341,#90342,#90343,
#90344,#90345,#90346,#90347,#90348,#90349,#90350,#90351,#90352,#90353,#90354,
#90355,#90356,#90357,#90358,#90359,#90360,#90361,#90362,#90363,#90364,#90365,
#90366,#90367,#90368,#90369,#90370,#90371,#90372,#90373,#90374,#90375,#90376,
#90377,#90378,#90379,#90380,#90381,#90382,#90383,#90384,#90385,#90386,#90387,
#90388,#90389,#90390,#90391,#90392,#90393,#90394,#90395,#90396,#90397,#90398,
#90399,#90400,#90401,#90402,#90403,#90404,#90405,#90406,#90407,#90408,#90409,
#90410,#90411,#90412,#90413,#90414,#90415,#90416,#90417,#90418,#90419,#90420,
#90421,#90422,#90423,#90424,#90425,#90426,#90427,#90428,#90429,#90430,#90431,
#90432,#90433,#90434,#90435,#90436,#90437,#90438,#90439,#90440,#90441,#90442,
#90443,#90444,#90445,#90446,#90447,#90448,#90449,#90450,#90451,#90452,#90453,
#90454,#90455,#90456,#90457,#90458,#90459,#90460,#90461,#90462,#90463,#90464,
#90465,#90466,#90467,#90468,#90469,#90470,#90471,#90472,#90473,#90474,#90475,
#90476),.UNSPECIFIED.,.F.,.F.,(4,2,2,2,2,2,2,2,2,2,2,2,2,2,2,2,2,2,2,2,
2,2,2,2,2,2,2,2,2,2,2,2,2,2,2,2,2,2,2,2,2,2,2,2,2,2,2,2,2,2,2,2,2,2,2,2,
2,2,2,2,2,2,2,2,2,2,2,2,2,2,2,2,2,2,2,2,2,2,2,2,2,2,2,2,2,2,2,2,2,2,2,2,
2,2,2,2,2,2,2,2,2,2,2,2,2,2,2,2,2,2,2,2,4),(0.922374656735376,0.922441678336817,
0.929669563352342,0.931398013497983,0.932379245701514,0.933133327485008,
0.934154377021716,0.936117662869169,0.949668511573435,0.978599913803431,
0.99950309319788,1.00264567689765,1.00456774062369,1.00607496506275,1.007726120093,
1.01040601455546,1.01987525904208,1.03648178654763,1.05246817701862,1.07486147229562,
1.07703546006387,1.07809937797505,1.07893743104844,1.07991760135824,1.08168905123686,
1.09058365373482,1.13142881373052,1.14590925157162,1.14879591706687,1.15066103985426,
1.15215823534679,1.15386074058017,1.15677409968098,1.1690450573802,1.2066866730778,
1.21011190129153,1.22111804185858,1.22290600999143,1.22398663716322,1.22482797849294,
1.2257848066074,1.22744978901483,1.23466086729284,1.24967651901599,1.28754670880767,
1.29353421236312,1.29586917817801,1.29728772594104,1.298808304525,1.30085337778138,
1.30548053531504,1.32505477851414,1.35276125107147,1.35599530990382,1.36702217182252,
1.36881091548896,1.36989172870319,1.37073303810518,1.37168962811205,1.37335373326487,
1.3805537965296,1.39553306347069,1.43323279119158,1.43937922786553,1.44173875298288,
1.44316187486993,1.44467953756059,1.44670715268892,1.45123713180544,1.47003328032966,
1.49710674954745,1.51266765250984,1.51480640888025,1.51586315992757,1.51670053763647,
1.51768570748545,1.51948087626994,1.52882112663116,1.57702007751937,1.58482029049405,
1.58741496865909,1.58904682755785,1.590559000198,1.5925527638141,1.59689857919281,
1.61427073157841,1.6503870241433,1.65907731127102,1.66074876059535,1.66180574475427,
1.66264300101881,1.66362767121947,1.66542101950393,1.67462109717352,1.69767869170011,
1.72320023579086,1.73074654846158,1.73330840509739,1.7349330898852,1.73644793990468,
1.73845911607361,1.742703335404,1.76176944885827,1.77710430862767,1.80254111148967,
1.80594173691123,1.80725558217838,1.80804719634072,1.80890917573716,1.81013887279834,
1.81153304103024,1.81688352078661,1.84386758684803),.UNSPECIFIED.);
#1468=B_SPLINE_CURVE_WITH_KNOTS('',3,(#90477,#90478,#90479,#90480),
 .UNSPECIFIED.,.F.,.F.,(4,4),(0.000437250149454394,0.000569891382468709),
 .UNSPECIFIED.);
#1469=B_SPLINE_CURVE_WITH_KNOTS('',3,(#90485,#90486,#90487,#90488,#90489,
#90490,#90491,#90492,#90493,#90494,#90495,#90496,#90497,#90498,#90499,#90500,
#90501,#90502,#90503,#90504,#90505,#90506,#90507,#90508,#90509,#90510,#90511,
#90512,#90513,#90514,#90515,#90516,#90517,#90518,#90519,#90520,#90521,#90522,
#90523,#90524,#90525,#90526,#90527,#90528,#90529,#90530,#90531,#90532,#90533,
#90534,#90535,#90536,#90537,#90538,#90539,#90540,#90541,#90542,#90543,#90544,
#90545,#90546,#90547,#90548,#90549,#90550,#90551,#90552,#90553,#90554,#90555,
#90556,#90557,#90558,#90559,#90560,#90561,#90562,#90563,#90564,#90565,#90566,
#90567,#90568,#90569,#90570,#90571,#90572,#90573,#90574,#90575,#90576,#90577,
#90578,#90579,#90580,#90581,#90582,#90583,#90584,#90585,#90586,#90587,#90588,
#90589,#90590,#90591,#90592,#90593,#90594,#90595,#90596,#90597,#90598,#90599,
#90600,#90601,#90602,#90603,#90604,#90605,#90606,#90607,#90608,#90609,#90610,
#90611,#90612,#90613,#90614,#90615,#90616,#90617,#90618,#90619,#90620,#90621,
#90622,#90623,#90624,#90625,#90626,#90627,#90628,#90629,#90630,#90631,#90632,
#90633,#90634,#90635,#90636,#90637,#90638,#90639,#90640,#90641,#90642,#90643,
#90644,#90645,#90646,#90647,#90648,#90649,#90650,#90651,#90652,#90653,#90654,
#90655,#90656,#90657,#90658,#90659,#90660,#90661,#90662,#90663,#90664,#90665,
#90666,#90667,#90668,#90669,#90670,#90671,#90672,#90673,#90674,#90675,#90676,
#90677,#90678,#90679,#90680,#90681,#90682,#90683,#90684,#90685,#90686,#90687,
#90688,#90689,#90690,#90691,#90692,#90693,#90694,#90695,#90696,#90697,#90698,
#90699,#90700,#90701,#90702,#90703,#90704,#90705,#90706,#90707,#90708,#90709,
#90710,#90711,#90712),.UNSPECIFIED.,.F.,.F.,(4,2,2,2,2,2,2,2,2,2,2,2,2,
2,2,2,2,2,2,2,2,2,2,2,2,2,2,2,2,2,2,2,2,2,2,2,2,2,2,2,2,2,2,2,2,2,2,2,2,
2,2,2,2,2,2,2,2,2,2,2,2,2,2,2,2,2,2,2,2,2,2,2,2,2,2,2,2,2,2,2,2,2,2,2,2,
2,2,2,2,2,2,2,2,2,2,2,2,2,2,2,2,2,2,2,2,2,2,2,2,2,2,2,2,4),(0.922237918268933,
0.926191380517241,0.928119136273235,0.929622265718532,0.931285630671642,
0.934023493063675,0.944125402861637,0.962454933641687,0.991889074968301,
0.999075909855535,1.00080040965521,1.00178039749423,1.00261796873746,1.00368084370519,
1.0058512515426,1.03270699473906,1.06637721632002,1.07143241105219,1.07339463166143,
1.07481525079866,1.0763335103127,1.07836757148888,1.08293592137179,1.10204291116039,
1.1315854070021,1.13445517732235,1.14463158888902,1.14638195575269,1.14746269654295,
1.1483017540574,1.14926914126989,1.15098353319044,1.15893311426642,1.17659485078496,
1.21246334268913,1.21737983272704,1.21931906276357,1.22073369826865,1.22225561069733,
1.22431218795711,1.22900784980099,1.24915062863753,1.27901742982362,1.29041927107787,
1.2922228579389,1.29330776575634,1.29414923112743,1.29510253520903,1.29675302271267,
1.30377338419188,1.31815923966033,1.34839826012403,1.3613316449532,1.36439084658745,
1.36614305909745,1.36748649037184,1.36922488470512,1.37230492781941,1.38721768321407,
1.42297123686884,1.42539232928606,1.43633239314308,1.43811689464082,1.43919620642788,
1.44003700860903,1.44099376058001,1.44265982786119,1.449894473333,1.46499328388894,
1.50325668840128,1.50886886276059,1.51114173453244,1.51254819335221,1.51407588306873,
1.5161663824848,1.52105817626358,1.54286212948439,1.57254396029178,1.58232286539809,
1.58405106567852,1.58512508976432,1.58596345918923,1.5869352271435,1.58866990840903,
1.59694670305082,1.61589018058861,1.64993240861968,1.65496655955894,1.65692521533157,
1.6583447912648,1.6598633719341,1.66190035739807,1.66633367998342,1.67235653071594,
1.68801302370398,1.71216513777381,1.72781247307564,1.72995298528613,1.73100976777579,
1.73184675312409,1.73283095715545,1.73387720794681,1.73794425893755,1.75494459842043,
1.77044323174245,1.77166507438393,1.7981109293864,1.80133484956356,1.80328007860033,
1.80478967806922,1.80642754540642,1.80905086815995,1.81212690020928,1.84368667532253),
 .UNSPECIFIED.);
#1470=B_SPLINE_CURVE_WITH_KNOTS('',3,(#90713,#90714,#90715,#90716,#90717,
#90718,#90719,#90720,#90721,#90722,#90723,#90724,#90725,#90726,#90727,#90728,
#90729,#90730,#90731,#90732,#90733,#90734,#90735,#90736,#90737,#90738,#90739,
#90740,#90741,#90742,#90743,#90744,#90745,#90746,#90747,#90748,#90749,#90750,
#90751,#90752,#90753,#90754,#90755,#90756,#90757,#90758,#90759,#90760,#90761,
#90762,#90763,#90764,#90765,#90766,#90767,#90768,#90769,#90770,#90771,#90772,
#90773,#90774,#90775,#90776,#90777,#90778,#90779,#90780,#90781,#90782,#90783,
#90784,#90785,#90786,#90787,#90788,#90789,#90790,#90791,#90792,#90793,#90794,
#90795,#90796,#90797,#90798,#90799,#90800,#90801,#90802,#90803,#90804,#90805,
#90806,#90807,#90808,#90809,#90810,#90811,#90812,#90813,#90814,#90815,#90816,
#90817,#90818,#90819,#90820,#90821,#90822,#90823,#90824,#90825,#90826,#90827,
#90828,#90829,#90830,#90831,#90832,#90833,#90834,#90835,#90836,#90837,#90838,
#90839,#90840,#90841,#90842,#90843,#90844,#90845,#90846,#90847,#90848,#90849,
#90850,#90851,#90852,#90853,#90854,#90855,#90856,#90857,#90858,#90859,#90860,
#90861,#90862,#90863,#90864,#90865,#90866,#90867,#90868,#90869,#90870,#90871,
#90872,#90873,#90874,#90875,#90876,#90877,#90878,#90879,#90880,#90881,#90882,
#90883,#90884,#90885,#90886,#90887,#90888,#90889,#90890,#90891,#90892,#90893,
#90894,#90895,#90896,#90897,#90898,#90899,#90900,#90901,#90902,#90903,#90904,
#90905,#90906,#90907,#90908,#90909,#90910,#90911,#90912,#90913,#90914,#90915,
#90916,#90917,#90918,#90919,#90920,#90921,#90922,#90923,#90924,#90925,#90926,
#90927,#90928,#90929,#90930,#90931,#90932,#90933,#90934,#90935,#90936,#90937,
#90938,#90939,#90940,#90941,#90942,#90943,#90944),.UNSPECIFIED.,.F.,.F.,
(4,2,2,2,2,2,2,2,2,2,2,2,2,2,2,2,2,2,2,2,2,2,2,2,2,2,2,2,2,2,2,2,2,2,2,
2,2,2,2,2,2,2,2,2,2,2,2,2,2,2,2,2,2,2,2,2,2,2,2,2,2,2,2,2,2,2,2,2,2,2,2,
2,2,2,2,2,2,2,2,2,2,2,2,2,2,2,2,2,2,2,2,2,2,2,2,2,2,2,2,2,2,2,2,2,2,2,2,
2,2,2,2,2,2,2,2,4),(0.000569891382468709,0.0234211215008631,0.0315171806116301,
0.0339709507313322,0.0356514811228152,0.0372904855016129,0.0388005311631058,
0.0407454991466058,0.043967164020376,0.0697359704180957,0.0844820296529836,
0.0988428121560535,0.107481436198876,0.109244982890933,0.110223230805987,
0.11106115406743,0.112126860457267,0.114310981263468,0.134638951409163,
0.164053319859173,0.177676762169647,0.18081673796223,0.182638142610473,
0.184132090598205,0.185866480323286,0.188846498971669,0.200717047092492,
0.233131063805651,0.246781920501471,0.253574678304614,0.255208327210515,
0.256158076276057,0.257000604441232,0.25809234348391,0.259918760145209,
0.271906743243061,0.297193090713906,0.314735376428027,0.324552159824207,
0.32726429947459,0.328922186055001,0.330426968953316,0.332366108330506,
0.335497373125117,0.356011549494214,0.390892671955947,0.399248465929993,
0.400988356283973,0.401961488635483,0.402800056497892,0.403873093279465,
0.405597333071729,0.415288666826581,0.421307420759307,0.448587327955876,
0.46741073454005,0.471943738532229,0.473971810494902,0.475489457928112,
0.476912302909234,0.479270763592592,0.485411497540558,0.523098540317878,
0.538070497887251,0.545268612143073,0.546932467540542,0.547888956264438,
0.54873019972848,0.549810968446364,0.551599725619324,0.562628340190154,
0.566012356347143,0.592202465961849,0.615086289528182,0.618480922763481,
0.620287048494713,0.621766488939377,0.623508750029304,0.62652248439948,
0.638831970114233,0.642841142841366,0.673063236989276,0.688919668413057,
0.692025151299668,0.693254012674242,0.69411595522706,0.694907964105746,
0.696223316119934,0.699632375081228,0.723790847739265,0.745670453589918,
0.75606487262287,0.760619041201492,0.764212010330671,0.766059312856068,
0.767554986933282,0.769269763017668,0.772163961525809,0.783036015483478,
0.786952820842268,0.827943342067928,0.83684703368413,0.838618769265589,
0.839598912949456,0.840436825921643,0.841500421755409,0.843673265471758,
0.862012533910661,0.897195178130637,0.904288691818974,0.909380527776448,
0.911505336825534,0.913039741168961,0.91443976540244,0.916674648209001,
0.922012310475654),.UNSPECIFIED.);
#1471=B_SPLINE_CURVE_WITH_KNOTS('',3,(#90949,#90950,#90951,#90952,#90953,
#90954,#90955,#90956,#90957,#90958,#90959,#90960,#90961,#90962,#90963,#90964,
#90965,#90966,#90967,#90968,#90969,#90970,#90971,#90972,#90973,#90974,#90975,
#90976,#90977,#90978,#90979,#90980,#90981,#90982,#90983,#90984,#90985,#90986,
#90987,#90988,#90989,#90990,#90991,#90992,#90993,#90994,#90995,#90996,#90997,
#90998,#90999,#91000,#91001,#91002,#91003,#91004,#91005,#91006,#91007,#91008,
#91009,#91010,#91011,#91012,#91013,#91014,#91015,#91016,#91017,#91018,#91019,
#91020,#91021,#91022,#91023,#91024,#91025,#91026,#91027,#91028,#91029,#91030,
#91031,#91032,#91033,#91034,#91035,#91036,#91037,#91038,#91039,#91040,#91041,
#91042,#91043,#91044,#91045,#91046,#91047,#91048,#91049,#91050,#91051,#91052,
#91053,#91054,#91055,#91056,#91057,#91058,#91059,#91060,#91061,#91062,#91063,
#91064,#91065,#91066,#91067,#91068,#91069,#91070,#91071,#91072,#91073,#91074,
#91075,#91076,#91077,#91078,#91079,#91080,#91081,#91082,#91083,#91084,#91085,
#91086,#91087,#91088,#91089,#91090,#91091,#91092,#91093,#91094,#91095,#91096,
#91097,#91098,#91099,#91100,#91101,#91102,#91103,#91104,#91105,#91106,#91107,
#91108,#91109,#91110,#91111,#91112,#91113,#91114,#91115,#91116,#91117,#91118,
#91119,#91120,#91121,#91122,#91123,#91124,#91125,#91126,#91127,#91128,#91129,
#91130,#91131,#91132,#91133,#91134,#91135,#91136,#91137,#91138,#91139,#91140,
#91141,#91142,#91143,#91144,#91145,#91146,#91147,#91148,#91149,#91150,#91151,
#91152,#91153,#91154,#91155,#91156,#91157,#91158,#91159,#91160,#91161,#91162,
#91163,#91164,#91165,#91166,#91167,#91168,#91169,#91170,#91171,#91172,#91173,
#91174,#91175,#91176),.UNSPECIFIED.,.F.,.F.,(4,2,2,2,2,2,2,2,2,2,2,2,2,
2,2,2,2,2,2,2,2,2,2,2,2,2,2,2,2,2,2,2,2,2,2,2,2,2,2,2,2,2,2,2,2,2,2,2,2,
2,2,2,2,2,2,2,2,2,2,2,2,2,2,2,2,2,2,2,2,2,2,2,2,2,2,2,2,2,2,2,2,2,2,2,2,
2,2,2,2,2,2,2,2,2,2,2,2,2,2,2,2,2,2,2,2,2,2,2,2,2,2,2,2,4),(0.000603157058436499,
0.0242728015901372,0.0455242222249288,0.0503514875987475,0.0524308860125723,
0.0539566101115037,0.0553655701855657,0.0572827886299263,0.0620694707013623,
0.099379775291639,0.102545358965389,0.116838533857367,0.121490824014618,
0.123655519389192,0.125362449551318,0.126333778083171,0.126337691211615,
0.126341651433116,0.126345659551442,0.126349716391369,0.126353822850078,
0.127190990917063,0.128249684223656,0.1299272293033,0.138757312345306,0.17100292461915,
0.191533483353917,0.196275389841045,0.198339976075251,0.199863153369347,
0.201275652089698,0.203206804707063,0.20807605831657,0.244489499537873,
0.261761562072419,0.269607877709756,0.271315508305104,0.27228137131579,
0.273120578558098,0.274203448618717,0.275961068058469,0.286340350187178,
0.295183586668706,0.319507365454128,0.337806469474444,0.342272235850673,
0.344287741411451,0.345802988305927,0.347228696031453,0.349603969183966,
0.355847514036339,0.393426364216901,0.408374808841762,0.41556538462058,
0.417228312338521,0.418184391169677,0.419025350140752,0.42010583143647,
0.421894264863799,0.432924996460801,0.436108066989557,0.462487116587213,
0.485382382099437,0.488776478899617,0.49058211151842,0.492061037907891,
0.493802561074966,0.496814675384872,0.509111350805791,0.513155866981549,
0.552511676599832,0.56128540280106,0.563049418113686,0.564027672791934,
0.564865439480634,0.565930718254876,0.568113187653535,0.589866027533524,
0.606707473900117,0.631220901665064,0.634654020888471,0.63646792445505,
0.63796134282706,0.639701503609759,0.642707298657573,0.654917462954403,
0.659006768372456,0.698416368541185,0.707194991925221,0.708959386853598,
0.709937772186992,0.710775601288849,0.711840895797125,0.713539763905891,
0.722749965942763,0.76637228426485,0.778163385065766,0.781040511201531,
0.782734564429488,0.784232083904403,0.786107854793001,0.789030688848387,
0.804167326361854,0.844313480092512,0.853151338136041,0.854918979493543,
0.855898028664477,0.85673572349562,0.857799944438683,0.859495394901204,
0.868644171644638,0.899312640430864,0.92219364149957,0.922237918268933),
 .UNSPECIFIED.);
#1472=B_SPLINE_CURVE_WITH_KNOTS('',3,(#91177,#91178,#91179,#91180,#91181,
#91182,#91183,#91184,#91185,#91186,#91187,#91188,#91189,#91190,#91191,#91192,
#91193,#91194,#91195,#91196,#91197,#91198,#91199,#91200,#91201,#91202,#91203,
#91204,#91205,#91206,#91207,#91208,#91209,#91210,#91211,#91212,#91213,#91214,
#91215,#91216,#91217,#91218,#91219,#91220,#91221,#91222,#91223,#91224,#91225,
#91226,#91227,#91228,#91229,#91230,#91231,#91232,#91233,#91234,#91235,#91236,
#91237,#91238,#91239,#91240,#91241,#91242,#91243,#91244,#91245,#91246,#91247,
#91248,#91249,#91250,#91251,#91252,#91253,#91254,#91255,#91256,#91257,#91258,
#91259,#91260,#91261,#91262,#91263,#91264,#91265,#91266,#91267,#91268,#91269,
#91270,#91271,#91272,#91273,#91274,#91275,#91276,#91277,#91278,#91279,#91280,
#91281,#91282,#91283,#91284,#91285,#91286,#91287,#91288,#91289,#91290,#91291,
#91292,#91293,#91294,#91295,#91296,#91297,#91298,#91299,#91300,#91301,#91302,
#91303,#91304,#91305,#91306,#91307,#91308,#91309,#91310,#91311,#91312,#91313,
#91314,#91315,#91316,#91317,#91318,#91319,#91320,#91321,#91322,#91323,#91324,
#91325,#91326,#91327,#91328,#91329,#91330,#91331,#91332,#91333,#91334,#91335,
#91336,#91337,#91338,#91339,#91340,#91341,#91342,#91343,#91344,#91345,#91346,
#91347,#91348,#91349,#91350,#91351,#91352,#91353,#91354,#91355,#91356,#91357,
#91358,#91359,#91360,#91361,#91362,#91363,#91364,#91365,#91366,#91367,#91368,
#91369,#91370,#91371,#91372,#91373,#91374,#91375,#91376,#91377,#91378,#91379,
#91380,#91381,#91382,#91383,#91384,#91385,#91386,#91387,#91388),
 .UNSPECIFIED.,.F.,.F.,(4,2,2,2,2,2,2,2,2,2,2,2,2,2,2,2,2,2,2,2,2,2,2,2,
2,2,2,2,2,2,2,2,2,2,2,2,2,2,2,2,2,2,2,2,2,2,2,2,2,2,2,2,2,2,2,2,2,2,2,2,
2,2,2,2,2,2,2,2,2,2,2,2,2,2,2,2,2,2,2,2,2,2,2,2,2,2,2,2,2,2,2,2,2,2,2,2,
2,2,2,2,2,2,2,2,2,4),(0.922012310475654,0.922053808326363,0.949455824714825,
0.980528444692292,0.983719999894429,0.984999548071363,0.985784813757977,
0.986653290540001,0.987915201678888,0.991235277550237,1.00936229902265,
1.02659807552285,1.05246100582919,1.05568386392365,1.05762934388777,1.05913967148792,
1.06077886681035,1.06340550166928,1.07234219378278,1.08758610019145,1.10790122412403,
1.12793654730576,1.13012047774734,1.13118624408529,1.13202429074506,1.13300276475955,
1.13476693373777,1.14353620666142,1.18282372255295,1.18701135371279,1.19926325525754,
1.20227256744914,1.20401374016723,1.2055074236171,1.20732090411564,1.21075098030214,
1.23511516870443,1.26178250415154,1.27406222930179,1.27589897747276,1.27699375435078,
1.277836710955,1.27878477472938,1.28041071672016,1.2871030386372,1.30043974824966,
1.32188474872857,1.34428388675028,1.34746139161366,1.34939342081783,1.35090162854341,
1.35254692800404,1.35520189353604,1.3644221744581,1.3803847460207,1.41098684208453,
1.42016999933871,1.4218674950582,1.42293244928709,1.42377035632849,1.42474924379045,
1.42651559610713,1.4353258366773,1.47511925967412,1.48066672649061,1.49126351871709,
1.49416583012754,1.49586560599262,1.49721294531379,1.49901153509807,1.50237131992824,
1.52402543071296,1.54909326115857,1.56560408614993,1.56775704018537,1.56881650574999,
1.5696539166194,1.57063666359216,1.57242116588277,1.5815646331395,1.62609006279349,
1.63708222855347,1.63998684703158,1.64170365505979,1.64319855322547,1.64504162642632,
1.64861591268507,1.68205919800277,1.7097092430882,1.71304962887461,1.71435359723089,
1.71514325641996,1.71593506806637,1.71709792995239,1.71978491699447,1.72358547575521,
1.73404962440439,1.77554765578889,1.78356984827116,1.78619213296712,1.78782984969521,
1.78933965012658,1.79131888859957,1.79558781985974,1.8123854668724,1.84347475602747),
 .UNSPECIFIED.);
#1473=B_SPLINE_CURVE_WITH_KNOTS('',3,(#91394,#91395,#91396,#91397,#91398,
#91399,#91400,#91401,#91402,#91403,#91404,#91405,#91406,#91407,#91408,#91409,
#91410,#91411,#91412,#91413,#91414,#91415,#91416,#91417,#91418,#91419,#91420,
#91421,#91422,#91423,#91424,#91425,#91426,#91427,#91428,#91429,#91430,#91431,
#91432,#91433,#91434,#91435,#91436,#91437,#91438,#91439,#91440,#91441,#91442,
#91443,#91444,#91445,#91446,#91447,#91448,#91449,#91450,#91451,#91452,#91453,
#91454,#91455,#91456,#91457,#91458,#91459,#91460,#91461,#91462,#91463,#91464,
#91465,#91466,#91467,#91468,#91469,#91470,#91471,#91472,#91473,#91474,#91475,
#91476,#91477,#91478,#91479,#91480,#91481,#91482,#91483,#91484,#91485,#91486,
#91487,#91488,#91489,#91490,#91491,#91492,#91493,#91494,#91495,#91496,#91497,
#91498,#91499,#91500,#91501,#91502,#91503,#91504,#91505,#91506,#91507,#91508,
#91509,#91510,#91511,#91512,#91513,#91514,#91515,#91516,#91517,#91518,#91519,
#91520,#91521,#91522,#91523,#91524,#91525,#91526,#91527,#91528,#91529,#91530,
#91531,#91532,#91533,#91534,#91535,#91536,#91537,#91538,#91539,#91540,#91541,
#91542,#91543,#91544,#91545,#91546,#91547,#91548,#91549,#91550,#91551,#91552,
#91553,#91554,#91555,#91556,#91557,#91558,#91559,#91560,#91561,#91562,#91563,
#91564,#91565,#91566,#91567,#91568,#91569,#91570,#91571,#91572,#91573,#91574,
#91575,#91576,#91577,#91578,#91579,#91580,#91581,#91582,#91583,#91584,#91585,
#91586,#91587,#91588,#91589,#91590,#91591,#91592,#91593,#91594,#91595,#91596,
#91597,#91598,#91599,#91600,#91601,#91602,#91603,#91604,#91605,#91606,#91607,
#91608,#91609,#91610,#91611,#91612,#91613,#91614,#91615,#91616,#91617,#91618,
#91619,#91620,#91621,#91622,#91623,#91624,#91625),.UNSPECIFIED.,.F.,.F.,
(4,2,2,2,2,2,2,2,2,2,2,2,2,2,2,2,2,2,2,2,2,2,2,2,2,2,2,2,2,2,2,2,2,2,2,
2,2,2,2,2,2,2,2,2,2,2,2,2,2,2,2,2,2,2,2,2,2,2,2,2,2,2,2,2,2,2,2,2,2,2,2,
2,2,2,2,2,2,2,2,2,2,2,2,2,2,2,2,2,2,2,2,2,2,2,2,2,2,2,2,2,2,2,2,2,2,2,2,
2,2,2,2,2,2,2,2,4),(0.92220090061974,0.922325888116382,0.929171380658707,
0.944910417814658,0.947051038261568,0.948108072843558,0.9489453561298,0.949930025013108,
0.951723270745192,0.961029923508041,1.00850138698254,1.01692383708755,1.01959486903211,
1.02124341671153,1.02275014578737,1.02470660615659,1.02885412891554,1.06167680520233,
1.08454191506249,1.09155920700789,1.09326982510087,1.09424661867011,1.09508450525561,
1.09615170321977,1.09834400459525,1.12278401280386,1.15909034657558,1.16397128534812,
1.16590452490943,1.16731764096164,1.16884062117056,1.17090341854495,1.17563445618998,
1.19607034499369,1.22334825821511,1.22615479033711,1.23702743095864,1.23881000275399,
1.23988873981184,1.2407294656659,1.24168655535469,1.2433541876858,1.25061099521239,
1.2657850321197,1.30444229493087,1.30969707579691,1.31191120450844,1.31330702704867,
1.31484397478946,1.31698560842737,1.32218328021569,1.32946848222614,1.35061032612254,
1.38098904106956,1.38421493273134,1.38549987882817,1.38628586935009,1.3871527072722,
1.38840803044897,1.39168695864234,1.40937080414152,1.43029035384477,1.45302481649981,
1.45620900610413,1.45814262711265,1.45965059411416,1.46129412730463,1.46394290542258,
1.47310732126338,1.48892877731242,1.52056293615756,1.52900419925148,1.53065889680903,
1.53171063039138,1.53254735199949,1.53353561931391,1.53534637627702,1.54500308550315,
1.56875537706158,1.59886558841991,1.60206399916757,1.60400178310818,1.60551033163413,
1.60715181224644,1.60979136027428,1.61886395583434,1.63445222451569,1.66213694960228,
1.67451803689323,1.67653467489069,1.67757965379503,1.67841598574851,1.67938969775886,
1.68114884599781,1.68336741545605,1.68818380798208,1.70329560238921,1.74164518418991,
1.7471787445908,1.74943825888756,1.75084218494262,1.75237167034521,1.75447287499963,
1.75942825667814,1.78179040117797,1.80000504732398,1.80787176689765,1.81270722073954,
1.82075949869818,1.82239019564568,1.82343451635495,1.82427074015814,1.82506598874869,
1.8260479410353,1.82752872464318,1.84359018605298),.UNSPECIFIED.);
#1474=B_SPLINE_CURVE_WITH_KNOTS('',3,(#91626,#91627,#91628,#91629),
 .UNSPECIFIED.,.F.,.F.,(4,4),(0.000504233101903366,0.000603157058436499),
 .UNSPECIFIED.);
#1475=B_SPLINE_CURVE_WITH_KNOTS('',3,(#91631,#91632,#91633,#91634),
 .UNSPECIFIED.,.F.,.F.,(4,4),(1.84347475602747,1.84357418596773),
 .UNSPECIFIED.);
#1476=B_SPLINE_CURVE_WITH_KNOTS('',3,(#91635,#91636,#91637,#91638,#91639,
#91640,#91641,#91642,#91643,#91644,#91645,#91646,#91647,#91648,#91649,#91650,
#91651,#91652,#91653,#91654,#91655,#91656,#91657,#91658,#91659,#91660,#91661,
#91662,#91663,#91664,#91665,#91666,#91667,#91668,#91669,#91670,#91671,#91672,
#91673,#91674,#91675,#91676,#91677,#91678,#91679,#91680,#91681,#91682,#91683,
#91684,#91685,#91686,#91687,#91688,#91689,#91690,#91691,#91692,#91693,#91694,
#91695,#91696,#91697,#91698,#91699,#91700,#91701,#91702,#91703,#91704,#91705,
#91706,#91707,#91708,#91709,#91710,#91711,#91712,#91713,#91714,#91715,#91716,
#91717,#91718,#91719,#91720,#91721,#91722,#91723,#91724,#91725,#91726,#91727,
#91728,#91729,#91730,#91731,#91732,#91733,#91734,#91735,#91736,#91737,#91738,
#91739,#91740,#91741,#91742,#91743,#91744,#91745,#91746,#91747,#91748,#91749,
#91750,#91751,#91752,#91753,#91754,#91755,#91756,#91757,#91758,#91759,#91760,
#91761,#91762,#91763,#91764,#91765,#91766,#91767,#91768,#91769,#91770,#91771,
#91772,#91773,#91774,#91775,#91776,#91777,#91778,#91779,#91780,#91781,#91782,
#91783,#91784,#91785,#91786,#91787,#91788,#91789,#91790,#91791,#91792,#91793,
#91794,#91795,#91796,#91797,#91798,#91799,#91800,#91801,#91802,#91803,#91804,
#91805,#91806,#91807,#91808,#91809,#91810,#91811,#91812,#91813,#91814,#91815,
#91816,#91817,#91818,#91819,#91820,#91821,#91822,#91823,#91824,#91825,#91826,
#91827,#91828,#91829,#91830,#91831,#91832,#91833,#91834,#91835,#91836,#91837,
#91838,#91839,#91840,#91841,#91842,#91843,#91844,#91845,#91846,#91847,#91848,
#91849,#91850,#91851,#91852,#91853,#91854,#91855,#91856,#91857,#91858,#91859,
#91860,#91861,#91862,#91863,#91864),.UNSPECIFIED.,.F.,.F.,(4,2,2,2,2,2,
2,2,2,2,2,2,2,2,2,2,2,2,2,2,2,2,2,2,2,2,2,2,2,2,2,2,2,2,2,2,2,2,2,2,2,2,
2,2,2,2,2,2,2,2,2,2,2,2,2,2,2,2,2,2,2,2,2,2,2,2,2,2,2,2,2,2,2,2,2,2,2,2,
2,2,2,2,2,2,2,2,2,2,2,2,2,2,2,2,2,2,2,2,2,2,2,2,2,2,2,2,2,2,2,2,2,2,2,2,
4),(0.000514367078856413,0.0145491834342173,0.0159723333821196,0.0169307456053303,
0.0177208162106002,0.0185598473094828,0.0196386025654595,0.0213819679780018,
0.0314599034020634,0.0384405059200993,0.0640065293208735,0.0831024169649428,
0.0876694908409809,0.0897036020698978,0.0912221463529332,0.0926432104126621,
0.0946063324042943,0.0996655295224006,0.133196328624006,0.139827735978584,
0.154048280886289,0.158686042382176,0.160846107346323,0.162569295973232,
0.163534594088163,0.164371878264975,0.165428474660188,0.167566792227759,
0.192354390306657,0.211287190609083,0.229185364956923,0.233599982327971,
0.235606533211473,0.237120772034357,0.238747545335732,0.241318523352881,
0.248933555089244,0.290869300131118,0.3049240147517,0.307844798036407,0.309043863488256,
0.309900263008358,0.310699438675858,0.311825761227252,0.314843824875668,
0.347587392027096,0.367248803133798,0.377812096025181,0.380590910569084,
0.382263573116883,0.383765182632549,0.385677330502464,0.388718823848285,
0.406280457836509,0.434283339279588,0.450490326151363,0.453630094275619,
0.454864289627471,0.455727214292652,0.456517971226011,0.457826992779143,
0.461197307826611,0.487877340014091,0.518431063279376,0.524668383519615,
0.526969068294142,0.528537832201057,0.530066934633274,0.531905633552078,
0.536521459514119,0.576165623906971,0.591380580461383,0.598650417277672,
0.600319344936863,0.601276926423549,0.602117918338552,0.603196814428242,
0.604979287975413,0.615852269783709,0.61877549619381,0.621522709073118,
0.650263236054138,0.662498474932574,0.667598427435381,0.671529708301216,
0.673444797452557,0.674946765474791,0.676617813094535,0.679389225609711,
0.688693882009756,0.735114611881829,0.74436597440058,0.74615658066323,0.747140827492345,
0.747978378994018,0.749036577115915,0.751182240392891,0.767116820935144,
0.796235179698225,0.813027418718856,0.81729643654,0.819276302815579,0.820786825935832,
0.822425564493073,0.825050006188704,0.83308285832759,0.881000615253691,
0.890327880790218,0.892122683501165,0.893107931706556,0.893945542452374,
0.895002805086352,0.897143294078358,0.921919804481415,0.922044868712354),
 .UNSPECIFIED.);
#1477=B_SPLINE_CURVE_WITH_KNOTS('',3,(#91869,#91870,#91871,#91872,#91873,
#91874,#91875,#91876,#91877,#91878,#91879,#91880,#91881,#91882,#91883,#91884,
#91885,#91886,#91887,#91888,#91889,#91890,#91891,#91892,#91893,#91894,#91895,
#91896,#91897,#91898,#91899,#91900,#91901,#91902,#91903,#91904,#91905,#91906,
#91907,#91908,#91909,#91910,#91911,#91912,#91913,#91914,#91915,#91916,#91917,
#91918,#91919,#91920,#91921,#91922,#91923,#91924,#91925,#91926,#91927,#91928,
#91929,#91930,#91931,#91932,#91933,#91934,#91935,#91936,#91937,#91938,#91939,
#91940,#91941,#91942,#91943,#91944,#91945,#91946,#91947,#91948,#91949,#91950,
#91951,#91952,#91953,#91954,#91955,#91956,#91957,#91958,#91959,#91960,#91961,
#91962,#91963,#91964,#91965,#91966,#91967,#91968,#91969,#91970,#91971,#91972,
#91973,#91974,#91975,#91976,#91977,#91978,#91979,#91980,#91981,#91982,#91983,
#91984,#91985,#91986,#91987,#91988,#91989,#91990,#91991,#91992,#91993,#91994,
#91995,#91996,#91997,#91998,#91999,#92000,#92001,#92002,#92003,#92004,#92005,
#92006,#92007,#92008,#92009,#92010,#92011,#92012,#92013,#92014,#92015,#92016,
#92017,#92018,#92019,#92020,#92021,#92022,#92023,#92024,#92025,#92026,#92027,
#92028,#92029,#92030,#92031,#92032,#92033,#92034,#92035,#92036,#92037,#92038,
#92039,#92040,#92041,#92042,#92043,#92044,#92045,#92046,#92047,#92048,#92049,
#92050,#92051,#92052,#92053,#92054,#92055,#92056,#92057,#92058,#92059,#92060,
#92061,#92062,#92063,#92064,#92065,#92066,#92067,#92068,#92069,#92070,#92071,
#92072,#92073,#92074,#92075,#92076,#92077,#92078,#92079,#92080,#92081,#92082,
#92083,#92084,#92085,#92086,#92087,#92088),.UNSPECIFIED.,.F.,.F.,(4,2,2,
2,2,2,2,2,2,2,2,2,2,2,2,2,2,2,2,2,2,2,2,2,2,2,2,2,2,2,2,2,2,2,2,2,2,2,2,
2,2,2,2,2,2,2,2,2,2,2,2,2,2,2,2,2,2,2,2,2,2,2,2,2,2,2,2,2,2,2,2,2,2,2,2,
2,2,2,2,2,2,2,2,2,2,2,2,2,2,2,2,2,2,2,2,2,2,2,2,2,2,2,2,2,2,2,2,2,2,4),
(0.000560841254929146,0.00122756953817873,0.00267783709836508,0.00567972886798112,
0.0181404681574918,0.0482412476540577,0.0631058226340338,0.0702712299010112,
0.0719322779124441,0.0728879076863163,0.073728893577787,0.074809949783987,
0.0766004493265835,0.0876821930869903,0.0934836507060726,0.118466356148674,
0.132922348118984,0.14153694467225,0.144129266545428,0.14553501432938,0.146922238349318,
0.148684188609048,0.151883422859173,0.16719752434947,0.207148620060003,
0.215970682958397,0.217737382556324,0.218716201272492,0.219553878953511,
0.220618309432577,0.222796599214438,0.241812416348709,0.27641312480095,
0.287075251525013,0.289861973754058,0.291536071740568,0.293036860785837,
0.294945072957918,0.297974518986067,0.315238399591854,0.343693836168037,
0.359788736556918,0.362917222689147,0.364149435902665,0.36501179462008,
0.365802663216913,0.367113095539219,0.370493437868455,0.396815555788648,
0.427749043793531,0.43396315179399,0.436260129516705,0.437827806985887,
0.43935695795578,0.441197049068491,0.445823569974353,0.485390019406719,
0.500655046706769,0.507939190168633,0.509608807644229,0.510566368139009,
0.511407058598387,0.51248518732404,0.514265603325819,0.525039635340057,
0.529105156428922,0.530736963300407,0.557265998364079,0.575997299907815,
0.580518225428479,0.58254380013687,0.584060725004862,0.585679346535489,
0.58821425323658,0.595559647273401,0.644307115618753,0.653671182364416,
0.65546738505493,0.656452688764453,0.657289909113878,0.658346102245061,
0.660014916233895,0.668662787504782,0.700017285642924,0.715901171077016,
0.725090015718347,0.727741707522573,0.729386168383326,0.730894397707321,
0.732827540488198,0.736009171757536,0.758600313644145,0.779718294718379,
0.793139809137975,0.799859817340565,0.801487782092057,0.802436227597114,
0.803278963837292,0.804372721475638,0.80620620218633,0.818393093773607,
0.844663171343837,0.867198441868272,0.872173952201972,0.87427899915139,
0.875809569388275,0.877213302395477,0.879108651497984,0.88376550628148,
0.92220090061974),.UNSPECIFIED.);
#1478=B_SPLINE_CURVE_WITH_KNOTS('',3,(#92089,#92090,#92091,#92092,#92093,
#92094,#92095,#92096,#92097,#92098,#92099,#92100,#92101,#92102,#92103,#92104,
#92105,#92106,#92107,#92108,#92109,#92110,#92111,#92112,#92113,#92114,#92115,
#92116,#92117,#92118,#92119,#92120,#92121,#92122,#92123,#92124,#92125,#92126,
#92127,#92128,#92129,#92130,#92131,#92132,#92133,#92134,#92135,#92136,#92137,
#92138,#92139,#92140,#92141,#92142,#92143,#92144,#92145,#92146,#92147,#92148,
#92149,#92150,#92151,#92152,#92153,#92154,#92155,#92156,#92157,#92158,#92159,
#92160,#92161,#92162,#92163,#92164,#92165,#92166,#92167,#92168,#92169,#92170,
#92171,#92172,#92173,#92174,#92175,#92176,#92177,#92178,#92179,#92180,#92181,
#92182,#92183,#92184,#92185,#92186,#92187,#92188,#92189,#92190,#92191,#92192,
#92193,#92194,#92195,#92196,#92197,#92198,#92199,#92200,#92201,#92202,#92203,
#92204,#92205,#92206,#92207,#92208,#92209,#92210,#92211,#92212,#92213,#92214,
#92215,#92216,#92217,#92218,#92219,#92220,#92221,#92222,#92223,#92224,#92225,
#92226,#92227,#92228,#92229,#92230,#92231,#92232,#92233,#92234,#92235,#92236,
#92237,#92238,#92239,#92240,#92241,#92242,#92243,#92244,#92245,#92246,#92247,
#92248,#92249,#92250,#92251,#92252,#92253,#92254,#92255,#92256,#92257,#92258,
#92259,#92260,#92261,#92262,#92263,#92264,#92265,#92266,#92267,#92268,#92269,
#92270,#92271,#92272,#92273,#92274,#92275,#92276,#92277,#92278,#92279,#92280,
#92281,#92282,#92283,#92284,#92285,#92286,#92287,#92288,#92289,#92290,#92291,
#92292,#92293,#92294,#92295,#92296,#92297,#92298,#92299,#92300,#92301,#92302,
#92303,#92304,#92305,#92306,#92307,#92308),.UNSPECIFIED.,.F.,.F.,(4,2,2,
2,2,2,2,2,2,2,2,2,2,2,2,2,2,2,2,2,2,2,2,2,2,2,2,2,2,2,2,2,2,2,2,2,2,2,2,
2,2,2,2,2,2,2,2,2,2,2,2,2,2,2,2,2,2,2,2,2,2,2,2,2,2,2,2,2,2,2,2,2,2,2,2,
2,2,2,2,2,2,2,2,2,2,2,2,2,2,2,2,2,2,2,2,2,2,2,2,2,2,2,2,2,2,2,2,2,2,4),
(0.922044868712354,0.957951216955999,0.962857132189006,0.964795243308246,
0.966210145180478,0.9677333716962,0.969793542894975,0.974505481536299,1.01033907250438,
1.0338039155043,1.03720987579679,1.03852492584848,1.03931701440143,1.04017928093119,
1.04140900386122,1.04451874111044,1.07372111205207,1.10353715082914,1.1086946534071,
1.11089337087447,1.1124265223922,1.11399149734849,1.11627201105666,1.12236561508084,
1.14930613726452,1.18000634886144,1.18321643011407,1.18449922076051,1.18528518696247,
1.18615322471591,1.18741241065632,1.19071345506026,1.20862773288827,1.22811240673908,
1.25200343314321,1.25521115203296,1.25715237260071,1.2586622920841,1.2603039561618,
1.26294093295913,1.2719762186749,1.28746609780656,1.31797414836967,1.32789531037431,
1.3296314252471,1.33070821458202,1.33154734756932,1.33251842554787,1.3342480693396,
1.34242910861663,1.36098295462764,1.39558537584312,1.40059166365024,1.40254652978157,
1.40396575209104,1.40548619857169,1.40752960195658,1.41214653280481,1.43163573793088,
1.46109093775326,1.46575197942915,1.47398752796917,1.4756304750864,1.47667897077869,
1.47751601842559,1.47850810236714,1.48033480490755,1.49030057773163,1.50465655267378,
1.54179382211166,1.54660189492035,1.5485234289827,1.54993406629443,1.55146017990374,
1.55353756966455,1.55834869626468,1.57944921565393,1.61104710500875,1.61984885719269,
1.6215254494019,1.6225841891728,1.62342182948617,1.62440578001485,1.62619483841352,
1.63541480323601,1.68121846539728,1.69108264970303,1.69385733035515,1.69555583432989,
1.69702341744196,1.69846303747577,1.70150822980826,1.71580014007246,1.75047936255721,
1.75524581448804,1.76564446812615,1.76740352464161,1.76848707458016,1.76932667796977,
1.77029285853423,1.7720007494468,1.77984282979742,1.7970971166788,1.8275937815837,
1.83252639647331,1.83812231186191,1.84034742488907,1.84176042468243,1.84300117335869,
1.84382673505472),.UNSPECIFIED.);
#1479=B_SPLINE_CURVE_WITH_KNOTS('',3,(#92313,#92314,#92315,#92316,#92317,
#92318,#92319,#92320,#92321,#92322,#92323,#92324,#92325,#92326,#92327,#92328,
#92329,#92330,#92331,#92332,#92333,#92334,#92335,#92336,#92337,#92338,#92339,
#92340,#92341,#92342,#92343,#92344,#92345,#92346,#92347,#92348,#92349,#92350,
#92351,#92352,#92353,#92354,#92355,#92356,#92357,#92358,#92359,#92360,#92361,
#92362,#92363,#92364,#92365,#92366,#92367,#92368,#92369,#92370,#92371,#92372,
#92373,#92374,#92375,#92376,#92377,#92378,#92379,#92380,#92381,#92382,#92383,
#92384,#92385,#92386,#92387,#92388,#92389,#92390,#92391,#92392,#92393,#92394,
#92395,#92396,#92397,#92398,#92399,#92400,#92401,#92402,#92403,#92404,#92405,
#92406,#92407,#92408,#92409,#92410,#92411,#92412,#92413,#92414,#92415,#92416,
#92417,#92418,#92419,#92420,#92421,#92422,#92423,#92424,#92425,#92426,#92427,
#92428,#92429,#92430,#92431,#92432,#92433,#92434,#92435,#92436,#92437,#92438,
#92439,#92440,#92441,#92442,#92443,#92444,#92445,#92446,#92447,#92448,#92449,
#92450,#92451,#92452,#92453,#92454,#92455,#92456,#92457,#92458,#92459,#92460,
#92461,#92462,#92463,#92464,#92465,#92466,#92467,#92468,#92469,#92470,#92471,
#92472,#92473,#92474,#92475,#92476,#92477,#92478,#92479,#92480,#92481,#92482,
#92483,#92484,#92485,#92486,#92487,#92488,#92489,#92490,#92491,#92492,#92493,
#92494,#92495,#92496,#92497,#92498,#92499,#92500,#92501,#92502,#92503,#92504,
#92505,#92506,#92507,#92508,#92509,#92510,#92511,#92512,#92513,#92514,#92515,
#92516,#92517,#92518,#92519,#92520,#92521,#92522,#92523,#92524,#92525,#92526,
#92527,#92528,#92529,#92530,#92531,#92532,#92533,#92534),.UNSPECIFIED.,
 .F.,.F.,(4,2,2,2,2,2,2,2,2,2,2,2,2,2,2,2,2,2,2,2,2,2,2,2,2,2,2,2,2,2,2,
2,2,2,2,2,2,2,2,2,2,2,2,2,2,2,2,2,2,2,2,2,2,2,2,2,2,2,2,2,2,2,2,2,2,2,2,
2,2,2,2,2,2,2,2,2,2,2,2,2,2,2,2,2,2,2,2,2,2,2,2,2,2,2,2,2,2,2,2,2,2,2,2,
2,2,2,2,2,2,2,4),(0.92184713791035,0.959502202714741,0.964248452591541,
0.966156811049808,0.967563602013588,0.969091156156367,0.971180574837927,
0.976065701690815,0.997810886587701,1.02713685176618,1.03730234613504,1.03905214723152,
1.04013269185765,1.04097169562458,1.0419391328413,1.04365388153892,1.05160994584751,
1.06929694504387,1.10512553887402,1.11004478453439,1.11198442586174,1.11339912362621,
1.11492087830805,1.11697684646725,1.12166937331292,1.14178715244534,1.17188928515539,
1.17273432237921,1.18316199506977,1.18492196537473,1.18600553516131,1.18684480276664,
1.18781018172543,1.18951565207609,1.1973287366786,1.21447855352106,1.25110000003608,
1.25595276669724,1.25788110008379,1.25929286085876,1.2608165019727,1.26288395880259,
1.2676424961359,1.28831042375301,1.30862340201075,1.32865266040931,1.33083561439304,
1.33190083574309,1.33273841724212,1.33371628803733,1.33547920376982,1.34423845665217,
1.38342544851417,1.38781514310891,1.3999761416561,1.40297752093518,1.4047162932078,
1.40620921539986,1.40802338134246,1.41145963549553,1.43617313975216,1.4603718058285,
1.46384144304377,1.47483184582374,1.47661814597033,1.47769784321836,1.47853850608394,
1.47949459753753,1.48115836177949,1.48836497250983,1.50337154463875,1.54121631636813,
1.54721110253447,1.549546013434,1.55096377325012,1.55248292851237,1.55452507219774,
1.55914117317309,1.57863886211985,1.60781127175613,1.61105675297003,1.62078703102191,
1.62251245465064,1.62358549676229,1.62442358458636,1.6253955811703,1.62713202352675,
1.63544317725256,1.66991338570153,1.69086710689583,1.69428921568218,1.69610054202612,
1.69755590889034,1.69895896290358,1.70150520065044,1.70970187225048,1.72316486819267,
1.74781792230383,1.76618561505148,1.7683570221211,1.76941977827453,1.77025696197296,
1.77123615053114,1.77300589804385,1.78189313395678,1.8226996992311,1.83718485204772,
1.84032456194338,1.8419602229474,1.84280903719847,1.84319664678967),
 .UNSPECIFIED.);
#1480=B_SPLINE_CURVE_WITH_KNOTS('',3,(#92535,#92536,#92537,#92538,#92539,
#92540,#92541,#92542,#92543,#92544,#92545,#92546,#92547,#92548,#92549,#92550,
#92551,#92552,#92553,#92554,#92555,#92556,#92557,#92558,#92559,#92560,#92561,
#92562,#92563,#92564,#92565,#92566,#92567,#92568,#92569,#92570,#92571,#92572,
#92573,#92574,#92575,#92576,#92577,#92578,#92579,#92580,#92581,#92582,#92583,
#92584,#92585,#92586,#92587,#92588,#92589,#92590,#92591,#92592,#92593,#92594,
#92595,#92596,#92597,#92598,#92599,#92600,#92601,#92602,#92603,#92604,#92605,
#92606,#92607,#92608,#92609,#92610,#92611,#92612,#92613,#92614,#92615,#92616,
#92617,#92618,#92619,#92620,#92621,#92622,#92623,#92624,#92625,#92626,#92627,
#92628,#92629,#92630,#92631,#92632,#92633,#92634,#92635,#92636,#92637,#92638,
#92639,#92640,#92641,#92642,#92643,#92644,#92645,#92646,#92647,#92648,#92649,
#92650,#92651,#92652,#92653,#92654,#92655,#92656,#92657,#92658,#92659,#92660,
#92661,#92662,#92663,#92664,#92665,#92666,#92667,#92668,#92669,#92670,#92671,
#92672,#92673,#92674,#92675,#92676,#92677,#92678,#92679,#92680,#92681,#92682,
#92683,#92684,#92685,#92686,#92687,#92688,#92689,#92690,#92691,#92692,#92693,
#92694,#92695,#92696,#92697,#92698,#92699,#92700,#92701,#92702,#92703,#92704,
#92705,#92706,#92707,#92708,#92709,#92710,#92711,#92712,#92713,#92714,#92715,
#92716,#92717,#92718,#92719,#92720,#92721,#92722,#92723,#92724,#92725,#92726,
#92727,#92728,#92729,#92730,#92731,#92732,#92733,#92734,#92735,#92736,#92737,
#92738,#92739,#92740,#92741,#92742,#92743,#92744,#92745,#92746,#92747,#92748,
#92749,#92750,#92751,#92752,#92753,#92754,#92755,#92756,#92757,#92758,#92759,
#92760,#92761,#92762,#92763,#92764,#92765,#92766,#92767,#92768,#92769,#92770,
#92771,#92772,#92773,#92774,#92775,#92776,#92777,#92778,#92779,#92780,#92781,
#92782),.UNSPECIFIED.,.F.,.F.,(4,2,2,2,2,2,2,2,2,2,2,2,2,2,2,2,2,2,2,2,
2,2,2,2,2,2,2,2,2,2,2,2,2,2,2,2,2,2,2,2,2,2,2,2,2,2,2,2,2,2,2,2,2,2,2,2,
2,2,2,2,2,2,2,2,2,2,2,2,2,2,2,2,2,2,2,2,2,2,2,2,2,2,2,2,2,2,2,2,2,2,2,2,
2,2,2,2,2,2,2,2,2,2,2,2,2,2,2,2,2,2,2,2,2,2,2,2,2,2,2,2,2,2,2,4),(0.00012595403202429,
0.00218637696266717,0.00554721496821566,0.0239701111963791,0.0549555024570598,
0.0636516104352712,0.0670061422371314,0.0694733219362498,0.0705931884102283,
0.0714369703945452,0.0723816528101506,0.0739923205577916,0.0797162191741279,
0.110377873674624,0.136998805598095,0.141103587059436,0.142994152621875,
0.143020098183966,0.143046065870231,0.143072140017256,0.143098410197693,
0.143124972852337,0.143151933243671,0.143179407914987,0.143207527730223,
0.143236441781002,0.14326632246758,0.143297372223598,0.143329832604141,
0.143363996858905,0.143400227678008,0.143438983102546,0.143480855440994,
0.143526632169561,0.143577395805891,0.144957057462043,0.146705001471571,
0.14984124782424,0.164210301934727,0.205133245307085,0.214031167616271,
0.21580243835845,0.21678241386525,0.217620237933776,0.218683791331271,0.220856781157315,
0.239233502956004,0.257374347094855,0.275282649333089,0.285233094207398,
0.287957727233648,0.289618476098257,0.291122756979793,0.29305690630218,
0.296171217751287,0.316033489673126,0.35153527606005,0.35995526673488,0.361699123477876,
0.362673179710778,0.363511729196881,0.364583687709302,0.366304170682459,
0.375919616626686,0.382066480279564,0.409311086696754,0.4281318055117,0.432664686170611,
0.434692856912888,0.436210639211135,0.437633654884878,0.439603705195045,
0.444704969762174,0.47725879114568,0.504375707510041,0.507053723176792,
0.50821158373033,0.509061025093207,0.509872153033562,0.511284864792439,
0.515352271524616,0.547470932545512,0.575660180833196,0.579158623129055,
0.580986428030765,0.582336837988072,0.58401614983331,0.586824785491797,
0.596476726083428,0.602933215397876,0.642909884322407,0.651734677152069,
0.653501996700771,0.654481177582231,0.655319182211822,0.656384069648828,
0.658563447040849,0.677644759745462,0.712189363349494,0.722843238208159,
0.725629948181284,0.727304448801835,0.728805862426927,0.730715234046021,
0.733747263033456,0.751009086425224,0.789012703406279,0.797670777485914,
0.799428638215717,0.800405773101758,0.801244012328779,0.802311756290388,
0.804018199210054,0.813363859088499,0.816967421623116,0.846250287691673,
0.865755008074216,0.870373298635367,0.872416782579536,0.873937083934142,
0.87554994869635,0.878056510194058,0.88518976221749,0.921744011977849),
 .UNSPECIFIED.);
#1481=B_SPLINE_CURVE_WITH_KNOTS('',3,(#92788,#92789,#92790,#92791),
 .UNSPECIFIED.,.F.,.F.,(4,4),(1.84328751696407,1.84339250911099),
 .UNSPECIFIED.);
#1482=B_SPLINE_CURVE_WITH_KNOTS('',3,(#92792,#92793,#92794,#92795,#92796,
#92797,#92798,#92799,#92800,#92801,#92802,#92803,#92804,#92805,#92806,#92807,
#92808,#92809,#92810,#92811,#92812,#92813,#92814,#92815,#92816,#92817,#92818,
#92819,#92820,#92821,#92822,#92823,#92824,#92825,#92826,#92827,#92828,#92829,
#92830,#92831,#92832,#92833,#92834,#92835,#92836,#92837,#92838,#92839,#92840,
#92841,#92842,#92843,#92844,#92845,#92846,#92847,#92848,#92849,#92850,#92851,
#92852,#92853,#92854,#92855,#92856,#92857,#92858,#92859,#92860,#92861,#92862,
#92863,#92864,#92865,#92866,#92867,#92868,#92869,#92870,#92871,#92872,#92873,
#92874,#92875,#92876,#92877,#92878,#92879,#92880,#92881,#92882,#92883,#92884,
#92885,#92886,#92887,#92888,#92889,#92890,#92891,#92892,#92893,#92894,#92895,
#92896,#92897,#92898,#92899,#92900,#92901,#92902,#92903,#92904,#92905,#92906,
#92907,#92908,#92909,#92910,#92911,#92912,#92913,#92914,#92915,#92916,#92917,
#92918,#92919,#92920,#92921,#92922,#92923,#92924,#92925,#92926,#92927,#92928,
#92929,#92930,#92931,#92932,#92933,#92934,#92935,#92936,#92937,#92938,#92939,
#92940,#92941,#92942,#92943,#92944,#92945,#92946,#92947,#92948,#92949,#92950,
#92951,#92952,#92953,#92954,#92955,#92956,#92957,#92958,#92959,#92960,#92961,
#92962,#92963,#92964,#92965,#92966,#92967,#92968,#92969,#92970,#92971,#92972,
#92973,#92974,#92975,#92976,#92977,#92978,#92979,#92980,#92981,#92982,#92983,
#92984,#92985,#92986,#92987,#92988,#92989,#92990,#92991,#92992,#92993,#92994,
#92995,#92996,#92997,#92998,#92999,#93000,#93001,#93002,#93003,#93004,#93005,
#93006,#93007,#93008,#93009,#93010,#93011,#93012,#93013,#93014,#93015,#93016,
#93017,#93018,#93019,#93020,#93021,#93022,#93023,#93024,#93025,#93026,#93027,
#93028,#93029,#93030,#93031,#93032,#93033,#93034,#93035,#93036,#93037,#93038,
#93039,#93040,#93041,#93042,#93043),.UNSPECIFIED.,.F.,.F.,(4,2,2,2,2,2,
2,2,2,2,2,2,2,2,2,2,2,2,2,2,2,2,2,2,2,2,2,2,2,2,2,2,2,2,2,2,2,2,2,2,2,2,
2,2,2,2,2,2,2,2,2,2,2,2,2,2,2,2,2,2,2,2,2,2,2,2,2,2,2,2,2,2,2,2,2,2,2,2,
2,2,2,2,2,2,2,2,2,2,2,2,2,2,2,2,2,2,2,2,2,2,2,2,2,2,2,2,2,2,2,2,2,2,2,2,
2,2,2,2,2,2,2,2,2,2,2,4),(0.000507238272519671,0.0115418756662477,0.0161571515980744,
0.0175387459960026,0.0184800213009734,0.0192665950615534,0.0201084096248052,
0.0211965733620706,0.0230114391999691,0.0347020160235591,0.0421510699498056,
0.0629843018573606,0.0786783707889196,0.087791964193193,0.0904356812284005,
0.0920781025212334,0.0935864074751727,0.0955223417032235,0.0987143659005448,
0.121823158328269,0.142229744673646,0.155766161873468,0.16026128371635,
0.162373702648284,0.164065047205974,0.165023582816099,0.165026289481035,
0.16502900841385,0.165031739646659,0.165034483317566,0.165037239494238,
0.165040008196784,0.165042789523719,0.165045583614506,0.165884248018116,
0.166961579432677,0.168700784394348,0.178700731597012,0.184200587396513,
0.211105093774062,0.232350788405546,0.235697760840822,0.237493357017398,
0.238971777810241,0.240721778058453,0.24377141410812,0.256571256187601,
0.299144704642571,0.308161566058544,0.30993901754339,0.310920150949101,
0.311757569683489,0.312818801779902,0.314504531697237,0.323479859128245,
0.354926694790919,0.370495029651168,0.379559213562087,0.38219808772191,
0.383839518327,0.385348268110146,0.387286652872957,0.390486772602777,0.414010639504558,
0.433903873874492,0.447505272164639,0.454282058326798,0.455914194091047,
0.456863450066428,0.457705798384517,0.458797618410472,0.460624823668758,
0.472643209202041,0.501037126350278,0.516429831595371,0.525424242536336,
0.528056017980191,0.529695862242627,0.531205058415621,0.533146666039113,
0.536357838593584,0.56499738458374,0.589917764242636,0.599810258968735,
0.601632640613339,0.60262344653153,0.603460044239458,0.604508754759125,
0.606153459330318,0.614427710277649,0.646412431380139,0.667697184496171,
0.672528479771231,0.674608640766409,0.676134560611962,0.677543445880114,
0.679460169640051,0.684243574775772,0.721592007256339,0.738248490911493,
0.745927941863251,0.74762467943057,0.748588190957836,0.749427827593889,
0.750514502575196,0.752284714430037,0.762912850310487,0.776606589220784,
0.813728503794617,0.818475755710185,0.820541362201342,0.82206479592093,
0.82347718065036,0.825407631681245,0.830272301428554,0.866745356671935,
0.883980439204212,0.891817078929897,0.893524166361651,0.894489952440844,
0.895329241447557,0.896412411779411,0.898170901120078,0.908566028100056,
0.921725293771825,0.92184713791035),.UNSPECIFIED.);
#1483=B_SPLINE_CURVE_WITH_KNOTS('',3,(#93045,#93046,#93047,#93048,#93049,
#93050,#93051,#93052,#93053,#93054,#93055,#93056,#93057,#93058,#93059,#93060,
#93061,#93062,#93063,#93064,#93065,#93066,#93067,#93068,#93069,#93070,#93071,
#93072,#93073,#93074,#93075,#93076,#93077,#93078,#93079,#93080,#93081,#93082,
#93083,#93084,#93085,#93086,#93087,#93088,#93089,#93090,#93091,#93092,#93093,
#93094,#93095,#93096,#93097,#93098,#93099,#93100,#93101,#93102,#93103,#93104,
#93105,#93106,#93107,#93108,#93109,#93110,#93111,#93112,#93113,#93114,#93115,
#93116,#93117,#93118,#93119,#93120,#93121,#93122,#93123,#93124,#93125,#93126,
#93127,#93128,#93129,#93130,#93131,#93132,#93133,#93134,#93135,#93136,#93137,
#93138,#93139,#93140,#93141,#93142,#93143,#93144,#93145,#93146,#93147,#93148,
#93149,#93150,#93151,#93152,#93153,#93154,#93155,#93156,#93157,#93158,#93159,
#93160,#93161,#93162,#93163,#93164,#93165,#93166,#93167,#93168,#93169,#93170,
#93171,#93172,#93173,#93174,#93175,#93176,#93177,#93178,#93179,#93180,#93181,
#93182,#93183,#93184,#93185,#93186,#93187,#93188,#93189,#93190,#93191,#93192,
#93193,#93194,#93195,#93196,#93197,#93198,#93199,#93200,#93201,#93202,#93203,
#93204,#93205,#93206,#93207,#93208,#93209,#93210,#93211,#93212,#93213,#93214,
#93215,#93216,#93217,#93218,#93219,#93220,#93221,#93222,#93223,#93224,#93225,
#93226,#93227,#93228,#93229,#93230,#93231,#93232,#93233,#93234,#93235,#93236,
#93237,#93238,#93239,#93240,#93241,#93242,#93243,#93244,#93245,#93246,#93247,
#93248,#93249,#93250,#93251,#93252,#93253,#93254,#93255,#93256,#93257,#93258,
#93259,#93260,#93261,#93262,#93263,#93264,#93265,#93266,#93267,#93268,#93269,
#93270,#93271,#93272,#93273,#93274,#93275,#93276,#93277,#93278,#93279,#93280,
#93281,#93282,#93283,#93284),.UNSPECIFIED.,.F.,.F.,(4,2,2,2,2,2,2,2,2,2,
2,2,2,2,2,2,2,2,2,2,2,2,2,2,2,2,2,2,2,2,2,2,2,2,2,2,2,2,2,2,2,2,2,2,2,2,
2,2,2,2,2,2,2,2,2,2,2,2,2,2,2,2,2,2,2,2,2,2,2,2,2,2,2,2,2,2,2,2,2,2,2,2,
2,2,2,2,2,2,2,2,2,2,2,2,2,2,2,2,2,2,2,2,2,2,2,2,2,2,2,2,2,2,2,2,2,2,2,2,
2,4),(0.921744011977849,0.921865738458927,0.942875463146245,0.945058987704988,
0.946124727844946,0.946962837126453,0.947941480348613,0.949706193849952,
0.958483171269677,0.997857769285124,1.00187835052179,1.01419853273591,1.01721313057314,
1.01895560251344,1.0204350532745,1.02224098303035,1.02563462099119,1.04848407546454,
1.07493123890233,1.07808623450929,1.08909791407495,1.09088591753303,1.09196647160793,
1.09280769694936,1.09376432570356,1.09542880642761,1.10263529751694,1.11763689221872,
1.15544509611991,1.16148560244784,1.1638283010648,1.16524816107476,1.16676757045501,
1.16880658534114,1.17340071769271,1.19271066898546,1.22306651610329,1.23492716994851,
1.23674892120692,1.23783933268164,1.2386817319795,1.23963233829674,1.24126972005375,
1.24811034418236,1.2619141802092,1.27953506561225,1.30504490179358,1.30826601596226,
1.31021086919364,1.31172096257071,1.31336015649653,1.31598734191935,1.32493135350266,
1.3401943565466,1.35554782663822,1.3786729325822,1.38207577983284,1.38339007796561,
1.38418184574252,1.38504388360563,1.38627348205163,1.3893839636763,1.40529378766577,
1.43527994794866,1.4396329781728,1.45181249929639,1.4548163387311,1.45655624372948,
1.45804996887263,1.45986490392343,1.46330200352542,1.48798919102565,1.51148591021547,
1.51647211320548,1.52674685887107,1.52849974082616,1.52958137564175,1.53042070745019,
1.53138795173193,1.53310100821026,1.54102522776882,1.55858967427563,1.59459275642693,
1.5994982202846,1.60143586669545,1.60285032804622,1.6043729844576,1.60643221539607,
1.61114125540389,1.64630990005493,1.67041592703416,1.67382310313879,1.67513807747604,
1.67592996080104,1.67679185839171,1.67799608307912,1.68096790791604,1.6852713676201,
1.69791597508939,1.70532821100474,1.74038201230939,1.74535752409139,1.74730693232044,
1.74872444459137,1.7502451746662,1.75229265811921,1.75693484534131,1.77663505762934,
1.78935914088988,1.80298014927108,1.80863787201225,1.81852255491565,1.82025634996804,
1.82133221316388,1.82217095734787,1.82296140675861,1.82392165848958,1.825349327827,
1.83023071831389,1.84305473654517),.UNSPECIFIED.);
#1484=B_SPLINE_CURVE_WITH_KNOTS('',3,(#93285,#93286,#93287,#93288),
 .UNSPECIFIED.,.F.,.F.,(4,4),(6.06069286854334E-5,0.000165048526771096),
 .UNSPECIFIED.);
#1485=B_SPLINE_CURVE_WITH_KNOTS('',3,(#93293,#93294,#93295,#93296,#93297,
#93298,#93299,#93300,#93301,#93302,#93303,#93304,#93305,#93306,#93307,#93308,
#93309,#93310,#93311,#93312,#93313,#93314,#93315,#93316,#93317,#93318,#93319,
#93320,#93321,#93322,#93323,#93324,#93325,#93326,#93327,#93328,#93329,#93330,
#93331,#93332,#93333,#93334,#93335,#93336,#93337,#93338,#93339,#93340,#93341,
#93342,#93343,#93344,#93345,#93346,#93347,#93348,#93349,#93350,#93351,#93352,
#93353,#93354,#93355,#93356,#93357,#93358,#93359,#93360,#93361,#93362,#93363,
#93364,#93365,#93366,#93367,#93368,#93369,#93370,#93371,#93372,#93373,#93374,
#93375,#93376,#93377,#93378,#93379,#93380,#93381,#93382,#93383,#93384,#93385,
#93386,#93387,#93388,#93389,#93390,#93391,#93392,#93393,#93394,#93395,#93396,
#93397,#93398,#93399,#93400,#93401,#93402,#93403,#93404,#93405,#93406,#93407,
#93408,#93409,#93410,#93411,#93412,#93413,#93414,#93415,#93416,#93417,#93418,
#93419,#93420,#93421,#93422,#93423,#93424,#93425,#93426,#93427,#93428,#93429,
#93430,#93431,#93432,#93433,#93434,#93435,#93436,#93437,#93438,#93439,#93440,
#93441,#93442,#93443,#93444,#93445,#93446,#93447,#93448,#93449,#93450,#93451,
#93452,#93453,#93454,#93455,#93456,#93457,#93458,#93459,#93460,#93461,#93462,
#93463,#93464,#93465,#93466,#93467,#93468,#93469,#93470,#93471,#93472,#93473,
#93474,#93475,#93476,#93477,#93478,#93479,#93480,#93481,#93482,#93483,#93484,
#93485,#93486,#93487,#93488,#93489,#93490,#93491,#93492,#93493,#93494,#93495,
#93496,#93497,#93498,#93499,#93500,#93501,#93502,#93503,#93504,#93505,#93506,
#93507,#93508,#93509,#93510,#93511,#93512,#93513,#93514,#93515,#93516,#93517,
#93518,#93519,#93520,#93521,#93522,#93523,#93524,#93525,#93526,#93527,#93528,
#93529,#93530,#93531,#93532,#93533,#93534,#93535,#93536,#93537,#93538,#93539,
#93540,#93541,#93542,#93543,#93544,#93545,#93546,#93547,#93548),
 .UNSPECIFIED.,.F.,.F.,(4,2,2,2,2,2,2,2,2,2,2,2,2,2,2,2,2,2,2,2,2,2,2,2,
2,2,2,2,2,2,2,2,2,2,2,2,2,2,2,2,2,2,2,2,2,2,2,2,2,2,2,2,2,2,2,2,2,2,2,2,
2,2,2,2,2,2,2,2,2,2,2,2,2,2,2,2,2,2,2,2,2,2,2,2,2,2,2,2,2,2,2,2,2,2,2,2,
2,2,2,2,2,2,2,2,2,2,2,2,2,2,2,2,2,2,2,2,2,2,2,2,2,2,2,2,2,2,2,4),(0.922053660167366,
0.922087260060697,0.940040360019168,0.958910709984947,0.983671445610604,
0.985810267030443,0.986866773817845,0.987703816919092,0.988688410408651,
0.990482049751448,0.999802918261662,1.04760833158185,1.05573564435285,1.05837060642386,
1.06001090511697,1.06151948947206,1.06349191178263,1.06772567124173,1.08426476345355,
1.11574005942909,1.11885233189373,1.12983902779931,1.13162520391438,1.13270487849394,
1.1335455565126,1.13450170272864,1.13616564787603,1.14337437849144,1.15838785883843,
1.19626480252467,1.20222978917324,1.2045603323842,1.20597729398325,1.20749701025564,
1.20954238349892,1.21417651122442,1.2338200852316,1.25922972009727,1.26100214864451,
1.26482076322953,1.27568689324359,1.27746791799819,1.27854602954697,1.2793864628986,
1.28034344268722,1.28201139689418,1.28927770565495,1.30448693936983,1.34414883568525,
1.3487613483557,1.35059880301895,1.35212688710593,1.35369462407545,1.35599383057863,
1.36222726691849,1.39276552672758,1.41942133833821,1.42278982840368,1.42409804027155,
1.42488827484649,1.42575058815126,1.42698382421619,1.43012066012992,1.44630887783009,
1.47432585394347,1.49190032765189,1.49494096782665,1.49685216649045,1.49835277641904,
1.500024058684,1.50279994461129,1.51334407414068,1.53295260484837,1.56573419028011,
1.56874343108313,1.56986798384359,1.57066632193375,1.57152226232998,1.57272138558515,
1.57564567927515,1.58974377943675,1.60915394397955,1.61679756787017,1.63753339326822,
1.64066930848961,1.64258843731963,1.64409404646603,1.64574412966254,1.64842384050773,
1.65790877083962,1.67456349461645,1.69821351357824,1.70255103019716,1.71317250854167,
1.71494190029434,1.71602812568589,1.71686744654269,1.71687216082131,1.7168768143746,
1.71688140830469,1.71688594376328,1.71689042178191,1.71689484343876,1.71689920972128,
1.71690352167988,1.71690778028904,1.71691198646676,1.71691614111979,1.71692024519425,
1.7169242996355,1.71692830523611,1.71693226285809,1.71693617336732,1.71790696852665,
1.719614421643,1.72177880850698,1.72643098462764,1.74072683873456,1.74383712668433,
1.78121434372384,1.78599374279393,1.78790937635078,1.78931763970165,1.79084305803641,
1.79292284985602,1.79775473667297,1.81904968632349,1.84328751696407),
 .UNSPECIFIED.);
#1486=B_SPLINE_CURVE_WITH_KNOTS('',3,(#93549,#93550,#93551,#93552,#93553,
#93554,#93555,#93556,#93557,#93558,#93559,#93560,#93561,#93562,#93563,#93564,
#93565,#93566,#93567,#93568,#93569,#93570,#93571,#93572,#93573,#93574,#93575,
#93576,#93577,#93578,#93579,#93580,#93581,#93582,#93583,#93584,#93585,#93586,
#93587,#93588,#93589,#93590,#93591,#93592,#93593,#93594,#93595,#93596,#93597,
#93598,#93599,#93600,#93601,#93602,#93603,#93604,#93605,#93606,#93607,#93608,
#93609,#93610,#93611,#93612,#93613,#93614,#93615,#93616,#93617,#93618,#93619,
#93620,#93621,#93622,#93623,#93624,#93625,#93626,#93627,#93628,#93629,#93630,
#93631,#93632,#93633,#93634,#93635,#93636,#93637,#93638,#93639,#93640,#93641,
#93642,#93643,#93644,#93645,#93646,#93647,#93648,#93649,#93650,#93651,#93652,
#93653,#93654,#93655,#93656,#93657,#93658,#93659,#93660,#93661,#93662,#93663,
#93664,#93665,#93666,#93667,#93668,#93669,#93670,#93671,#93672,#93673,#93674,
#93675,#93676,#93677,#93678,#93679,#93680,#93681,#93682,#93683,#93684,#93685,
#93686,#93687,#93688,#93689,#93690,#93691,#93692,#93693,#93694,#93695,#93696,
#93697,#93698,#93699,#93700,#93701,#93702,#93703,#93704,#93705,#93706,#93707,
#93708,#93709,#93710,#93711,#93712,#93713,#93714,#93715,#93716,#93717,#93718,
#93719,#93720,#93721,#93722,#93723,#93724,#93725,#93726,#93727,#93728,#93729,
#93730,#93731,#93732,#93733,#93734,#93735,#93736,#93737,#93738,#93739,#93740,
#93741,#93742,#93743,#93744,#93745,#93746,#93747,#93748,#93749,#93750,#93751,
#93752,#93753,#93754,#93755,#93756,#93757,#93758),.UNSPECIFIED.,.F.,.F.,
(4,2,2,2,2,2,2,2,2,2,2,2,2,2,2,2,2,2,2,2,2,2,2,2,2,2,2,2,2,2,2,2,2,2,2,
2,2,2,2,2,2,2,2,2,2,2,2,2,2,2,2,2,2,2,2,2,2,2,2,2,2,2,2,2,2,2,2,2,2,2,2,
2,2,2,2,2,2,2,2,2,2,2,2,2,2,2,2,2,2,2,2,2,2,2,2,2,2,2,2,2,2,2,2,2,4),(0.000165048526771096,
0.0253293883020531,0.0440233312379338,0.0485398414473035,0.0505648628561064,
0.0520819455305609,0.0535055102898666,0.055478239491361,0.0605976600882879,
0.0925806594593137,0.10915816826352,0.117396232764874,0.120628643687784,
0.122986886223187,0.12409383075386,0.124938905444333,0.12587847551582,0.127466259173235,
0.132972937720969,0.16925234368963,0.191681696135606,0.195063574176281,
0.196866782701579,0.198214489825009,0.199910658158823,0.202796750168318,
0.213220029316128,0.251687139151591,0.265761457742648,0.268684113545649,
0.269883381047268,0.270739721685867,0.271538680130797,0.272664469367232,
0.275679517991829,0.308422014850004,0.336476115064903,0.340539390079268,
0.342479881201168,0.343984674175026,0.345641523504167,0.348349582542018,
0.357088150645222,0.404153698408706,0.413437102129098,0.415229164613122,
0.416213619409496,0.417050987617156,0.418108494810463,0.420251265221457,
0.436076610926745,0.458751781769642,0.48340680028559,0.486843423628163,
0.488658281846636,0.490152031996057,0.491892066490804,0.494896377870751,
0.507082102985869,0.511188035506528,0.550597961678869,0.559376301281374,
0.561140919085653,0.562119473964424,0.562957482177003,0.564023067720846,
0.566206179224661,0.588183613402241,0.596117734484779,0.625354867098855,
0.631497351123744,0.63378463826994,0.63535077359174,0.636882353070066,0.638730141208508,
0.643402166041564,0.682627912157238,0.698100337801896,0.705445750016467,
0.707120145580897,0.708078999657966,0.708919873807517,0.709997043152338,
0.711773438040698,0.722493362893514,0.753298414168122,0.77329564601873,
0.777974224727522,0.780028339488228,0.781550364211679,0.782966484875099,
0.784909912426693,0.789848493038749,0.825420735390588,0.84326989705901,
0.851269806027336,0.85298789305913,0.853956349300999,0.854795684524097,
0.855875962836496,0.857623996064188,0.86779260362386,0.895513888013049,
0.92109500354705,0.921781199990569),.UNSPECIFIED.);
#1487=B_SPLINE_CURVE_WITH_KNOTS('',3,(#93763,#93764,#93765,#93766,#93767,
#93768,#93769,#93770,#93771,#93772,#93773,#93774,#93775,#93776,#93777,#93778,
#93779,#93780,#93781,#93782,#93783,#93784,#93785,#93786,#93787,#93788,#93789,
#93790,#93791,#93792,#93793,#93794,#93795,#93796,#93797,#93798,#93799,#93800,
#93801,#93802,#93803,#93804,#93805,#93806,#93807,#93808,#93809,#93810,#93811,
#93812,#93813,#93814,#93815,#93816,#93817,#93818,#93819,#93820,#93821,#93822,
#93823,#93824,#93825,#93826,#93827,#93828,#93829,#93830,#93831,#93832,#93833,
#93834,#93835,#93836,#93837,#93838,#93839,#93840,#93841,#93842,#93843,#93844,
#93845,#93846,#93847,#93848,#93849,#93850,#93851,#93852,#93853,#93854,#93855,
#93856,#93857,#93858,#93859,#93860,#93861,#93862,#93863,#93864,#93865,#93866,
#93867,#93868,#93869,#93870,#93871,#93872,#93873,#93874,#93875,#93876,#93877,
#93878,#93879,#93880,#93881,#93882,#93883,#93884,#93885,#93886,#93887,#93888,
#93889,#93890,#93891,#93892,#93893,#93894,#93895,#93896,#93897,#93898,#93899,
#93900,#93901,#93902,#93903,#93904,#93905,#93906,#93907,#93908,#93909,#93910,
#93911,#93912,#93913,#93914,#93915,#93916,#93917,#93918,#93919,#93920,#93921,
#93922,#93923,#93924,#93925,#93926,#93927,#93928,#93929,#93930,#93931,#93932,
#93933,#93934,#93935,#93936,#93937,#93938,#93939,#93940,#93941,#93942,#93943,
#93944,#93945,#93946,#93947,#93948,#93949,#93950,#93951,#93952,#93953,#93954,
#93955,#93956,#93957,#93958,#93959,#93960,#93961,#93962,#93963,#93964,#93965,
#93966,#93967,#93968,#93969,#93970,#93971,#93972,#93973,#93974,#93975,#93976,
#93977,#93978,#93979,#93980,#93981,#93982,#93983,#93984,#93985,#93986,#93987,
#93988,#93989,#93990),.UNSPECIFIED.,.F.,.F.,(4,2,2,2,2,2,2,2,2,2,2,2,2,
2,2,2,2,2,2,2,2,2,2,2,2,2,2,2,2,2,2,2,2,2,2,2,2,2,2,2,2,2,2,2,2,2,2,2,2,
2,2,2,2,2,2,2,2,2,2,2,2,2,2,2,2,2,2,2,2,2,2,2,2,2,2,2,2,2,2,2,2,2,2,2,2,
2,2,2,2,2,2,2,2,2,2,2,2,2,2,2,2,2,2,2,2,2,2,2,2,2,2,2,2,4),(0.00056079372868648,
0.0314868325224866,0.0345598635795401,0.0371810842167673,0.0388185847011278,
0.0403284860626301,0.0422749990790293,0.0455029771596276,0.0724134642533599,
0.0872259664856132,0.101947138251465,0.109164320163466,0.110836809300504,
0.111794974413502,0.112635462014109,0.11371242912883,0.115489139215583,
0.126221107362654,0.128816795710397,0.132081318273396,0.156173772407901,
0.171434016811604,0.177355359165885,0.181728724373122,0.183754843511515,
0.185271694282524,0.186694272331117,0.188664405386996,0.193769847522993,
0.226162967187165,0.246306035750068,0.254872941407773,0.256624855220193,
0.257600370626565,0.258438267959618,0.259506906218576,0.261217299757883,
0.27064950507009,0.302044032362892,0.317302963090176,0.326243708766339,
0.328869849463748,0.330508349749237,0.332017771100936,0.333961706768687,
0.337181150505317,0.3662284688738,0.390796876715171,0.400619329131009,0.402438186940812,
0.403428179111341,0.404264756774781,0.405314281688441,0.406961781844157,
0.415283332591889,0.447278012038036,0.468504645774497,0.473328970080421,
0.475407843006287,0.476933459153305,0.47834251479773,0.480260163788278,
0.48504948533156,0.522330013438216,0.53902709121155,0.546717468734998,0.548414854612492,
0.549378469746305,0.550218018268044,0.551304349595943,0.553073556687684,
0.56368495909994,0.564269942653249,0.570558938821339,0.594857189204174,
0.616637607065162,0.620000669124977,0.621799680235413,0.62327823891301,
0.625025257715295,0.628061764484938,0.640677113568726,0.683446680757099,
0.692477058164472,0.694255267817985,0.695236574889481,0.696073992199009,
0.697135030279977,0.698820090335841,0.707783081089864,0.75164721128199,
0.763459359468865,0.766337819828426,0.76803203133338,0.769529307174784,
0.771404264713819,0.774324850434573,0.789423958958945,0.829601299629364,
0.838440914800426,0.840208492969272,0.841187452754502,0.842025038781892,
0.843089079352831,0.84526566082161,0.864091502318696,0.888440640740583,
0.901833252358031,0.909999925860023,0.912543469636756,0.914163927687913,
0.915679995621691,0.917665771636198,0.922053660167366),.UNSPECIFIED.);
#1488=B_SPLINE_CURVE_WITH_KNOTS('',3,(#93991,#93992,#93993,#93994,#93995,
#93996,#93997,#93998,#93999,#94000,#94001,#94002,#94003,#94004,#94005,#94006,
#94007,#94008,#94009,#94010,#94011,#94012,#94013,#94014,#94015,#94016,#94017,
#94018,#94019,#94020,#94021,#94022,#94023,#94024,#94025,#94026,#94027,#94028,
#94029,#94030,#94031,#94032,#94033,#94034,#94035,#94036,#94037,#94038,#94039,
#94040,#94041,#94042,#94043,#94044,#94045,#94046,#94047,#94048,#94049,#94050,
#94051,#94052,#94053,#94054,#94055,#94056,#94057,#94058,#94059,#94060,#94061,
#94062,#94063,#94064,#94065,#94066,#94067,#94068,#94069,#94070,#94071,#94072,
#94073,#94074,#94075,#94076,#94077,#94078,#94079,#94080,#94081,#94082,#94083,
#94084,#94085,#94086,#94087,#94088,#94089,#94090,#94091,#94092,#94093,#94094,
#94095,#94096,#94097,#94098,#94099,#94100,#94101,#94102,#94103,#94104,#94105,
#94106,#94107,#94108,#94109,#94110,#94111,#94112,#94113,#94114,#94115,#94116,
#94117,#94118,#94119,#94120,#94121,#94122,#94123,#94124,#94125,#94126,#94127,
#94128,#94129,#94130,#94131,#94132,#94133,#94134,#94135,#94136,#94137,#94138,
#94139,#94140,#94141,#94142,#94143,#94144,#94145,#94146,#94147,#94148,#94149,
#94150,#94151,#94152,#94153,#94154,#94155,#94156,#94157,#94158,#94159,#94160,
#94161,#94162,#94163,#94164,#94165,#94166,#94167,#94168,#94169,#94170,#94171,
#94172,#94173,#94174,#94175,#94176,#94177,#94178,#94179,#94180,#94181,#94182,
#94183,#94184,#94185,#94186,#94187,#94188,#94189,#94190,#94191,#94192,#94193,
#94194,#94195,#94196,#94197,#94198,#94199,#94200,#94201,#94202,#94203,#94204,
#94205,#94206,#94207,#94208,#94209,#94210,#94211,#94212,#94213,#94214,#94215,
#94216,#94217,#94218,#94219,#94220,#94221,#94222),.UNSPECIFIED.,.F.,.F.,
(4,2,2,2,2,2,2,2,2,2,2,2,2,2,2,2,2,2,2,2,2,2,2,2,2,2,2,2,2,2,2,2,2,2,2,
2,2,2,2,2,2,2,2,2,2,2,2,2,2,2,2,2,2,2,2,2,2,2,2,2,2,2,2,2,2,2,2,2,2,2,2,
2,2,2,2,2,2,2,2,2,2,2,2,2,2,2,2,2,2,2,2,2,2,2,2,2,2,2,2,2,2,2,2,2,2,2,2,
2,2,2,2,2,2,2,2,4),(0.921781199990569,0.92455095130394,0.926369992845057,
0.927864117165824,0.929601106002656,0.932591516343193,0.944590865243596,
0.949293899696131,0.979093267103647,0.995024654573263,0.998137633628146,
0.999367725088923,1.00022994456683,1.00102174896383,1.00233585262656,1.00573684592158,
1.03077341063013,1.06505526322163,1.06976355062009,1.07182283997351,1.07334568558818,
1.07476042344764,1.07669860552441,1.08160625616145,1.11757494442375,1.13515119104018,
1.14307936949195,1.14479283679915,1.14576025985897,1.14659970808534,1.14768145085986,
1.14943443285809,1.15970666592777,1.18987032639148,1.20534364386987,1.21437093478311,
1.21700674299596,1.21864792017993,1.22015755308706,1.22209862854499,1.22530656891669,
1.25473863107226,1.2757464528823,1.28440318015446,1.28774742812013,1.29020875530951,
1.29132760484008,1.2921713194975,1.29311669242011,1.2947302137988,1.3004808435593,
1.30626871977407,1.30930471325302,1.33737951701725,1.35694385064697,1.36156935968951,
1.36361405187422,1.36513448008221,1.36655297988812,1.36850574083191,1.37350061478156,
1.40824376170405,1.43406245578207,1.4362509610709,1.43731764330944,1.43815577309033,
1.4391336086655,1.4408478370578,1.44790386429858,1.44979800263793,1.4814650796046,
1.4970622927606,1.50613861089842,1.50877933953405,1.51042158155929,1.51193085145158,
1.5138695959426,1.51706965847292,1.54054429365722,1.56050029693511,1.57409281112921,
1.58086737186545,1.58249974582887,1.58344927734843,1.5842919696053,1.58538438367816,
1.587212905422,1.59925479608142,1.62565749930631,1.65055185824534,1.65399373811137,
1.65580975672256,1.65730363596076,1.65904288161403,1.66204349298362,1.67417871372211,
1.67859734755346,1.70855105229235,1.72445648647901,1.72756679366189,1.72879641004152,
1.72965849363162,1.73045033591453,1.73176480791234,1.73516837594106,1.75829974816944,
1.7776790180723,1.79499523856027,1.79933387057718,1.80132656348101,1.80283883844358,
1.80447169141039,1.80706983679546,1.81573374903721,1.83030588459926,1.8432544735135),
 .UNSPECIFIED.);
#1489=B_SPLINE_CURVE_WITH_KNOTS('',3,(#94228,#94229,#94230,#94231,#94232,
#94233,#94234,#94235,#94236,#94237,#94238,#94239,#94240,#94241,#94242,#94243,
#94244,#94245,#94246,#94247,#94248,#94249,#94250,#94251,#94252,#94253,#94254,
#94255,#94256,#94257,#94258,#94259,#94260,#94261,#94262,#94263,#94264,#94265,
#94266,#94267,#94268,#94269,#94270,#94271,#94272,#94273,#94274,#94275,#94276,
#94277,#94278,#94279,#94280,#94281,#94282,#94283,#94284,#94285,#94286,#94287,
#94288,#94289,#94290,#94291,#94292,#94293,#94294,#94295,#94296,#94297,#94298,
#94299,#94300,#94301,#94302,#94303,#94304,#94305,#94306,#94307,#94308,#94309,
#94310,#94311,#94312,#94313,#94314,#94315,#94316,#94317,#94318,#94319,#94320,
#94321,#94322,#94323,#94324,#94325,#94326,#94327,#94328,#94329,#94330,#94331,
#94332,#94333,#94334,#94335,#94336,#94337,#94338,#94339,#94340,#94341,#94342,
#94343,#94344,#94345,#94346,#94347,#94348,#94349,#94350,#94351,#94352,#94353,
#94354,#94355,#94356,#94357,#94358,#94359,#94360,#94361,#94362,#94363,#94364,
#94365,#94366,#94367,#94368,#94369,#94370,#94371,#94372,#94373,#94374,#94375,
#94376,#94377,#94378,#94379,#94380,#94381,#94382,#94383,#94384,#94385,#94386,
#94387,#94388,#94389,#94390,#94391,#94392,#94393,#94394,#94395,#94396,#94397,
#94398,#94399,#94400,#94401,#94402,#94403,#94404,#94405,#94406,#94407,#94408,
#94409,#94410,#94411,#94412,#94413,#94414,#94415,#94416,#94417,#94418,#94419,
#94420,#94421,#94422,#94423,#94424,#94425,#94426,#94427,#94428,#94429,#94430,
#94431,#94432,#94433,#94434,#94435,#94436,#94437,#94438,#94439,#94440,#94441,
#94442,#94443,#94444,#94445,#94446,#94447,#94448,#94449,#94450,#94451,#94452,
#94453),.UNSPECIFIED.,.F.,.F.,(4,2,2,2,2,2,2,2,2,2,2,2,2,2,2,2,2,2,2,2,
2,2,2,2,2,2,2,2,2,2,2,2,2,2,2,2,2,2,2,2,2,2,2,2,2,2,2,2,2,2,2,2,2,2,2,2,
2,2,2,2,2,2,2,2,2,2,2,2,2,2,2,2,2,2,2,2,2,2,2,2,2,2,2,2,2,2,2,2,2,2,2,2,
2,2,2,2,2,2,2,2,2,2,2,2,2,2,2,2,2,2,2,2,4),(0.717606620371918,0.724937303735731,
0.72771389595266,0.72888278799588,0.729730165448876,0.730647726823811,0.732136308992316,
0.73678160719935,0.768402239729924,0.796423821392427,0.799925976396239,
0.80175695640325,0.803254677655556,0.804988896032012,0.807957585117534,
0.819622552326261,0.864542031817913,0.872241162803488,0.874009203477053,
0.875001700919868,0.875832872735957,0.876882871898634,0.878984749072429,
0.89957509783129,0.929771591109237,0.942756162588134,0.945819933785195,
0.947573744537744,0.948917873732766,0.950656544863179,0.95373524925088,
0.968601891243069,1.0040053419056,1.00701040447089,1.01785002831095,1.01963014616438,
1.02070808014087,1.02154842329556,1.02250507618966,1.02417287734539,1.03144459367853,
1.04667321819947,1.0863368694704,1.09095248756988,1.09278982277997,1.09431726656705,
1.09588378280359,1.09818012924158,1.10439888502929,1.13531603198701,1.16165487700035,
1.16503396067604,1.16634340607445,1.16713352886259,1.16799583108429,1.16922778679252,
1.17235396922868,1.18842502050758,1.21720898018135,1.2243668936313,1.23501452377013,
1.23792210383151,1.23962329924067,1.24110633894059,1.24296628002408,1.24662074531124,
1.27806483870237,1.30767612503891,1.3109392755739,1.31223116949292,1.31301889491692,
1.31388493343726,1.31513511845046,1.31837872927036,1.33567699042397,1.34803104693547,
1.37716376910126,1.38233104206709,1.38453078151396,1.38606357113137,1.38762727790221,
1.38990429049629,1.39597850367512,1.42192912837342,1.42776626852438,1.45338219518245,
1.45677440129569,1.45808673156896,1.45887794155059,1.45973989963584,1.46097028512708,
1.46395167097746,1.46830742711889,1.48119288853573,1.50699447052287,1.5258449547263,
1.5289267787661,1.53085073164652,1.53235323409534,1.53401829323474,1.53573667617848,
1.54145490323515,1.55968522198252,1.57484523843323,1.59922670856218,1.6026316006263,
1.60394594253714,1.60473751311349,1.6055992434061,1.60682804040949,1.6082209491119,
1.61365131628245,1.63904789497656),.UNSPECIFIED.);
#1490=B_SPLINE_CURVE_WITH_KNOTS('',3,(#94454,#94455,#94456,#94457),
 .UNSPECIFIED.,.F.,.F.,(4,4),(0.000428749880585189,0.00056079372868648),
 .UNSPECIFIED.);
#1491=B_SPLINE_CURVE_WITH_KNOTS('',3,(#94458,#94459,#94460,#94461,#94462,
#94463,#94464,#94465,#94466,#94467,#94468,#94469,#94470,#94471,#94472,#94473,
#94474,#94475,#94476,#94477,#94478,#94479,#94480,#94481,#94482,#94483,#94484,
#94485,#94486,#94487,#94488,#94489,#94490,#94491,#94492,#94493,#94494,#94495,
#94496,#94497,#94498,#94499,#94500,#94501,#94502,#94503,#94504,#94505,#94506,
#94507,#94508,#94509,#94510,#94511,#94512,#94513,#94514,#94515,#94516,#94517,
#94518,#94519,#94520,#94521,#94522,#94523,#94524,#94525,#94526,#94527,#94528,
#94529,#94530,#94531,#94532,#94533,#94534,#94535,#94536,#94537,#94538,#94539,
#94540,#94541,#94542,#94543,#94544,#94545,#94546,#94547,#94548,#94549,#94550,
#94551,#94552,#94553,#94554,#94555,#94556,#94557,#94558,#94559,#94560,#94561,
#94562,#94563,#94564,#94565,#94566,#94567,#94568,#94569,#94570,#94571,#94572,
#94573,#94574,#94575,#94576,#94577,#94578,#94579,#94580,#94581,#94582,#94583,
#94584,#94585,#94586,#94587,#94588,#94589,#94590,#94591,#94592,#94593,#94594,
#94595,#94596,#94597,#94598,#94599,#94600,#94601,#94602,#94603,#94604,#94605,
#94606,#94607,#94608,#94609,#94610,#94611,#94612,#94613,#94614,#94615,#94616,
#94617,#94618,#94619,#94620,#94621,#94622,#94623,#94624,#94625,#94626,#94627,
#94628,#94629,#94630,#94631,#94632,#94633,#94634,#94635,#94636,#94637,#94638,
#94639,#94640,#94641,#94642,#94643,#94644,#94645,#94646,#94647,#94648,#94649,
#94650,#94651,#94652,#94653,#94654,#94655,#94656,#94657,#94658,#94659,#94660,
#94661,#94662,#94663,#94664,#94665,#94666,#94667,#94668,#94669,#94670,#94671,
#94672,#94673,#94674,#94675,#94676,#94677,#94678,#94679,#94680,#94681,#94682,
#94683),.UNSPECIFIED.,.F.,.F.,(4,2,2,2,2,2,2,2,2,2,2,2,2,2,2,2,2,2,2,2,
2,2,2,2,2,2,2,2,2,2,2,2,2,2,2,2,2,2,2,2,2,2,2,2,2,2,2,2,2,2,2,2,2,2,2,2,
2,2,2,2,2,2,2,2,2,2,2,2,2,2,2,2,2,2,2,2,2,2,2,2,2,2,2,2,2,2,2,2,2,2,2,2,
2,2,2,2,2,2,2,2,2,2,2,2,2,2,2,2,2,2,2,2,4),(1.8432544735135,1.8581363739033,
1.86112220837997,1.87199099534198,1.87377297983242,1.87485174794923,1.87569273833946,
1.87665041392195,1.87831976961295,1.88559534826818,1.90083125139594,1.94046777125858,
1.94508724735617,1.9469265328112,1.94845578117905,1.95002434981121,1.95232410921401,
1.95855499105206,1.98926037353949,2.01576739741428,2.01914140474939,2.0204510073231,
2.02124186120728,2.02210465525392,2.02333827005434,2.02647444683507,2.04264654034132,
2.07066897754576,2.08827570540849,2.09131882588206,2.09323143629484,2.09473306762275,
2.09640540121951,2.09918284141753,2.10973086876282,2.12934522951758,2.16212278622311,
2.16514227758109,2.16626877159969,2.16706797513093,2.16792435908762,2.16912325548418,
2.17204283790939,2.18608753455905,2.22793132200851,2.23563790852107,2.23822074099923,
2.23985010818368,2.2413633813349,2.24336364012969,2.24774402244608,2.26537775381782,
2.28448711846242,2.3093890232548,2.3115227903059,2.31257843230654,2.31341554963876,
2.3144011018584,2.31619896006248,2.32559914920328,2.37521258159991,2.38185828637151,
2.38429442281185,2.38573169728544,2.38724101307681,2.38921809666859,2.39347639338184,
2.41019678982574,2.44004992322427,2.44578951561498,2.45563738933412,2.45736886604957,
2.45844380758605,2.45928217985398,2.4602531541547,2.461984427979,2.47020720730987,
2.48893603076886,2.52326417040624,2.52828263426371,2.53023875068998,2.53165769187546,
2.53317672403976,2.53521628682881,2.53981618777728,2.55918022556685,2.58945059709051,
2.60129966026234,2.60312060653294,2.60421064523502,2.60505295477509,2.60600390272237,
2.60764216152916,2.6144911394687,2.62832325001618,2.64523808840187,2.67134918821194,
2.67457170201162,2.67651697086531,2.67802714538887,2.67966619221896,2.68229264239869,
2.69122951398775,2.70647487972667,2.72536440763726,2.74679920447638,2.74898103650369,
2.75004613345169,2.75088344515566,2.75186049662732,2.75362245727572,2.76238681864969,
2.76458849571582),.UNSPECIFIED.);
#1492=B_SPLINE_CURVE_WITH_KNOTS('',3,(#94689,#94690,#94691,#94692,#94693,
#94694,#94695,#94696,#94697,#94698,#94699,#94700,#94701,#94702,#94703,#94704,
#94705,#94706,#94707,#94708,#94709,#94710,#94711,#94712,#94713,#94714,#94715,
#94716,#94717,#94718,#94719,#94720,#94721,#94722,#94723,#94724,#94725,#94726,
#94727,#94728,#94729,#94730,#94731,#94732,#94733,#94734,#94735,#94736,#94737,
#94738,#94739,#94740,#94741,#94742,#94743,#94744,#94745,#94746,#94747,#94748,
#94749,#94750,#94751,#94752,#94753,#94754,#94755,#94756,#94757,#94758,#94759,
#94760,#94761,#94762,#94763,#94764,#94765,#94766,#94767,#94768,#94769,#94770,
#94771,#94772,#94773,#94774,#94775,#94776,#94777,#94778,#94779,#94780,#94781,
#94782,#94783,#94784,#94785,#94786,#94787,#94788,#94789,#94790,#94791,#94792,
#94793,#94794,#94795,#94796,#94797,#94798,#94799,#94800,#94801,#94802),
 .UNSPECIFIED.,.F.,.F.,(4,2,2,2,2,2,2,2,2,2,2,2,2,2,2,2,2,2,2,2,2,2,2,2,
2,2,2,2,2,2,2,2,2,2,2,2,2,2,2,2,2,2,2,2,2,2,2,2,2,2,2,2,2,2,2,2,4),(-0.423911080838966,
-0.405908211040072,-0.402945684174472,-0.401057530385946,-0.399554399235692,
-0.397855357586041,-0.394963617425683,-0.382532843334228,-0.350771365776667,
-0.344155903874234,-0.342492928273389,-0.341527363314198,-0.340772431801499,
-0.339720645055032,-0.337575447171142,-0.318902188176821,-0.289632196839236,
-0.285408451687143,-0.283470616792185,-0.281969865296512,-0.2803418803254,
-0.277727928237807,-0.268593217070172,-0.23944422163428,-0.226992082995754,
-0.225204556914693,-0.224128704593718,-0.223289083878224,-0.222318390100464,
-0.220589885175706,-0.212188939951695,-0.19030078397516,-0.170407573432568,
-0.167425713515098,-0.165529010270916,-0.164021556253698,-0.162320256413333,
-0.159431029504583,-0.147102952224871,-0.115896794955732,-0.108940542391568,
-0.10724034705368,-0.106260105942312,-0.10541646138879,-0.104312932188852,
-0.103083802959583,-0.101020854601744,-0.0966688858107392,-0.0659538254154411,
-0.0539488960812429,-0.0509875805156346,-0.0492411068141357,-0.0477186667861302,
-0.0458353018362169,-0.042144008099143,-0.0181099242452841,-9.99999997863821E-7),
 .UNSPECIFIED.);
#1493=B_SPLINE_CURVE_WITH_KNOTS('',3,(#94805,#94806,#94807,#94808,#94809,
#94810,#94811,#94812,#94813,#94814,#94815,#94816,#94817,#94818,#94819,#94820,
#94821,#94822,#94823,#94824,#94825,#94826,#94827,#94828,#94829,#94830,#94831,
#94832,#94833,#94834,#94835,#94836,#94837,#94838,#94839,#94840,#94841,#94842,
#94843,#94844,#94845,#94846,#94847,#94848,#94849,#94850,#94851,#94852,#94853,
#94854,#94855,#94856,#94857,#94858,#94859,#94860,#94861,#94862,#94863,#94864,
#94865,#94866,#94867,#94868,#94869,#94870,#94871,#94872,#94873,#94874,#94875,
#94876,#94877,#94878,#94879,#94880,#94881,#94882,#94883,#94884,#94885,#94886),
 .UNSPECIFIED.,.F.,.F.,(4,3,3,3,3,3,3,3,3,3,3,3,3,3,3,3,3,3,3,3,3,3,3,3,
3,3,3,4),(11.6159397475004,11.7279534302045,11.7402765323561,11.8627684357717,
11.9852329360532,12.1077126178578,12.2334429699799,12.3561779531201,12.4834059897331,
12.5952366943264,12.6106340263461,12.6106792268383,12.718077365594,12.7349708112018,
12.8532987602863,12.9714916814451,13.0896045359157,13.2076921393023,13.3258929009561,
13.4441598868657,13.5566380093714,13.5626466500754,13.6053283051919,13.6053817568075,
13.7129385955191,13.725252783422,13.8508263858764,13.9763998223961),
 .UNSPECIFIED.);
#1494=B_SPLINE_CURVE_WITH_KNOTS('',3,(#94891,#94892,#94893,#94894,#94895,
#94896,#94897,#94898,#94899,#94900,#94901,#94902,#94903,#94904,#94905,#94906,
#94907,#94908,#94909,#94910,#94911,#94912,#94913,#94914,#94915,#94916,#94917,
#94918,#94919,#94920,#94921,#94922,#94923,#94924,#94925,#94926,#94927,#94928,
#94929,#94930,#94931,#94932,#94933,#94934,#94935,#94936,#94937,#94938,#94939,
#94940,#94941,#94942,#94943,#94944,#94945,#94946,#94947,#94948,#94949,#94950,
#94951,#94952,#94953,#94954,#94955,#94956,#94957,#94958,#94959,#94960,#94961,
#94962,#94963,#94964,#94965,#94966,#94967,#94968,#94969,#94970,#94971,#94972,
#94973,#94974,#94975,#94976,#94977,#94978,#94979,#94980,#94981,#94982,#94983,
#94984,#94985,#94986,#94987,#94988,#94989,#94990,#94991,#94992,#94993,#94994,
#94995,#94996,#94997,#94998,#94999,#95000,#95001,#95002,#95003,#95004,#95005,
#95006,#95007,#95008,#95009,#95010,#95011,#95012,#95013,#95014,#95015,#95016,
#95017,#95018,#95019,#95020,#95021,#95022,#95023,#95024,#95025,#95026,#95027,
#95028,#95029,#95030,#95031,#95032,#95033,#95034,#95035,#95036,#95037,#95038,
#95039,#95040,#95041,#95042,#95043,#95044,#95045,#95046,#95047,#95048,#95049,
#95050,#95051,#95052,#95053,#95054,#95055,#95056,#95057,#95058,#95059,#95060,
#95061,#95062,#95063,#95064,#95065,#95066,#95067,#95068,#95069,#95070,#95071,
#95072,#95073,#95074,#95075,#95076,#95077,#95078,#95079,#95080,#95081,#95082,
#95083,#95084,#95085,#95086,#95087,#95088,#95089,#95090,#95091,#95092,#95093,
#95094,#95095,#95096,#95097,#95098,#95099,#95100,#95101,#95102,#95103,#95104,
#95105,#95106,#95107,#95108),.UNSPECIFIED.,.F.,.F.,(4,2,2,2,2,2,2,2,2,2,
2,2,2,2,2,2,2,2,2,2,2,2,2,2,2,2,2,2,2,2,2,2,2,2,2,2,2,2,2,2,2,2,2,2,2,2,
2,2,2,2,2,2,2,2,2,2,2,2,2,2,2,2,2,2,2,2,2,2,2,2,2,2,2,2,2,2,2,2,2,2,2,2,
2,2,2,2,2,2,2,2,2,2,2,2,2,2,2,2,2,2,2,2,2,2,2,2,2,2,4),(-1.16578625258722,
-1.16495654187368,-1.16387501348904,-1.16303297303707,-1.1620629866672,
-1.16033394485289,-1.15188727820847,-1.12963412033475,-1.1104469835436,
-1.10748738777761,-1.10560281206173,-1.10410373135837,-1.10241061282265,
-1.09953244228331,-1.0872267352026,-1.05637041394269,-1.04889684686108,
-1.04716995475504,-1.0461901107729,-1.04534952929034,-1.04426464835453,
-1.04197498292351,-1.03889883285415,-1.03104273656382,-1.0063481291354,
-0.992640476299625,-0.9895944166997,-0.987846825113856,-0.98636714294917,
-0.984562623157298,-0.981162977683459,-0.976890565698702,-0.967198668382222,
-0.951556633460711,-0.933393821295391,-0.930455067393325,-0.929341844000728,
-0.928546592610655,-0.927681699048231,-0.926436143859374,-0.92320457470987,
-0.918368552294689,-0.902034378221544,-0.877501261995395,-0.872984035893418,
-0.870985689089877,-0.869467053799717,-0.867847658102225,-0.865306839995702,
-0.85700970951092,-0.827093006994181,-0.820444421276279,-0.813894183147314,
-0.812237116229529,-0.811273136987149,-0.810514063718278,-0.809450436543141,
-0.807272889010454,-0.789683323536542,-0.759416520850773,-0.755328828738471,
-0.753386932804677,-0.75188091242938,-0.750219519245063,-0.747488586636999,
-0.73717713213949,-0.71748982862789,-0.698511044436333,-0.695567413783529,
-0.694453463778226,-0.693657870737538,-0.692793767140101,-0.691549919168422,
-0.688325103285038,-0.683501581693507,-0.667239799232136,-0.642592123635406,
-0.638078649210613,-0.636082078756564,-0.634564871758043,-0.632947093886349,
-0.630409058292278,-0.62212431160859,-0.592230577070229,-0.585590872619476,
-0.578989339942265,-0.577329024853092,-0.576364892165802,-0.575606739190672,
-0.574545905558548,-0.572379782936935,-0.552910823499936,-0.524785970609621,
-0.520458360306892,-0.518493129209306,-0.516979169580948,-0.51534463755178,
-0.512736781622201,-0.503789355310463,-0.47429073229228,-0.462011770044367,
-0.460223268836459,-0.459143190738879,-0.458299202617069,-0.457322322059325,
-0.45557387726905,-0.446865573376514,-0.429016188564468,-0.423911080838966),
 .UNSPECIFIED.);
#1495=B_SPLINE_CURVE_WITH_KNOTS('',3,(#95109,#95110,#95111,#95112,#95113,
#95114,#95115,#95116,#95117,#95118,#95119,#95120,#95121,#95122,#95123,#95124,
#95125,#95126,#95127,#95128,#95129,#95130,#95131,#95132,#95133,#95134,#95135,
#95136,#95137,#95138,#95139,#95140,#95141,#95142,#95143,#95144,#95145,#95146,
#95147,#95148,#95149,#95150,#95151,#95152,#95153,#95154,#95155,#95156,#95157,
#95158,#95159,#95160,#95161,#95162,#95163,#95164,#95165,#95166,#95167,#95168,
#95169,#95170,#95171,#95172,#95173,#95174,#95175,#95176,#95177,#95178,#95179,
#95180,#95181,#95182,#95183,#95184,#95185,#95186,#95187,#95188,#95189,#95190,
#95191,#95192,#95193,#95194,#95195,#95196,#95197,#95198,#95199,#95200,#95201,
#95202,#95203,#95204,#95205,#95206,#95207,#95208,#95209,#95210,#95211,#95212,
#95213,#95214,#95215,#95216,#95217,#95218,#95219,#95220,#95221,#95222,#95223,
#95224,#95225,#95226,#95227,#95228,#95229,#95230,#95231,#95232,#95233,#95234,
#95235,#95236,#95237,#95238,#95239,#95240,#95241,#95242,#95243,#95244,#95245,
#95246,#95247,#95248,#95249,#95250,#95251,#95252,#95253,#95254,#95255,#95256,
#95257,#95258,#95259,#95260,#95261,#95262,#95263,#95264,#95265,#95266,#95267,
#95268,#95269,#95270,#95271,#95272,#95273,#95274,#95275,#95276,#95277,#95278,
#95279,#95280,#95281,#95282,#95283,#95284,#95285,#95286,#95287,#95288,#95289,
#95290,#95291,#95292,#95293,#95294,#95295,#95296,#95297,#95298,#95299,#95300,
#95301,#95302,#95303,#95304,#95305,#95306,#95307,#95308,#95309,#95310,#95311,
#95312,#95313,#95314,#95315,#95316,#95317,#95318,#95319,#95320,#95321,#95322,
#95323,#95324,#95325,#95326,#95327,#95328,#95329,#95330,#95331,#95332,#95333,
#95334,#95335,#95336,#95337,#95338,#95339,#95340,#95341,#95342,#95343,#95344,
#95345,#95346,#95347,#95348,#95349,#95350,#95351,#95352,#95353,#95354,#95355,
#95356,#95357,#95358,#95359,#95360),.UNSPECIFIED.,.F.,.F.,(4,2,2,2,2,2,
2,2,2,2,2,2,2,2,2,2,2,2,2,2,2,2,2,2,2,2,2,2,2,2,2,2,2,2,2,2,2,2,2,2,2,2,
2,2,2,2,2,2,2,2,2,2,2,2,2,2,2,2,2,2,2,2,2,2,2,2,2,2,2,2,2,2,2,2,2,2,2,2,
2,2,2,2,2,2,2,2,2,2,2,2,2,2,2,2,2,2,2,2,2,2,2,2,2,2,2,2,2,2,2,2,2,2,2,2,
2,2,2,2,2,2,2,2,2,2,2,4),(-3.17187947594733,-3.16473921561708,-3.16044316022415,
-3.15846517394355,-3.15695858374128,-3.15550482049477,-3.15406538677774,
-3.15208883016073,-3.14702675590512,-3.13661888044744,-3.11307841034839,
-3.10170138613847,-3.09980716171223,-3.09878428835165,-3.09801338455359,
-3.09697594603795,-3.09501861920091,-3.08313200236917,-3.06093000735926,
-3.05061394924129,-3.04615428213288,-3.04266380028948,-3.04084529016682,
-3.04082970367069,-3.04081308834817,-3.04079537316206,-3.04077648185846,
-3.04075633252447,-3.04073483719827,-3.04071190137564,-3.0406874234969,
-3.04066129445413,-3.04063339698503,-3.04060360512891,-3.04057178360287,
-3.04053778717087,-3.04051430308288,-3.04048217521517,-3.04043825415266,
-3.04037827706347,-3.04021217474066,-3.03868567534402,-3.03667384093241,
-3.03211184985238,-3.0077630940736,-2.99109257182972,-2.98619608800655,
-2.98293338566112,-2.98168248022944,-2.98081636090251,-2.98002687645685,
-2.97892473992055,-2.97604294642776,-2.95505059765632,-2.92818487901805,
-2.92479986426057,-2.92300643314673,-2.92166802083699,-2.91998339613827,
-2.91710777801048,-2.90622305090127,-2.88241214551628,-2.86803096211046,
-2.86515617296928,-2.86397305226884,-2.86312331737095,-2.86231496670698,
-2.86091410110994,-2.85689131048492,-2.82232135423191,-2.80962358938941,
-2.80671604439528,-2.80501425651505,-2.80351265896253,-2.80163169890575,
-2.79869077066792,-2.78059942225208,-2.75753930416373,-2.74896173234075,
-2.74722111813196,-2.74624631948059,-2.74540265460367,-2.74432113162423,
-2.74252649138957,-2.73005240772113,-2.70030937760648,-2.69176898761776,
-2.68920302699147,-2.68757829101405,-2.6860620585469,-2.6840775962008,-2.67963839706581,
-2.65309963755078,-2.63219491261709,-2.63003427031576,-2.62897490286081,
-2.62821730997577,-2.6272532254352,-2.62559159585125,-2.61896608146239,
-2.61234247874397,-2.58246684431845,-2.57420731415295,-2.57167292818137,
-2.57005657166638,-2.56854006816777,-2.56654351167923,-2.5620261450634,
-2.53753545536722,-2.52114250077137,-2.51629823951272,-2.51306381837714,
-2.51181894868876,-2.51095501667289,-2.51016029464169,-2.50904853637329,
-2.50611857824521,-2.48765980805246,-2.46759729142429,-2.457178204582,-2.45443942572901,
-2.45277690884135,-2.45127222392516,-2.44933536282734,-2.44527082756646,
-2.43011734130913),.UNSPECIFIED.);
#1496=B_SPLINE_CURVE_WITH_KNOTS('',3,(#95365,#95366,#95367,#95368,#95369,
#95370,#95371,#95372,#95373,#95374,#95375,#95376,#95377,#95378,#95379,#95380,
#95381,#95382,#95383,#95384,#95385,#95386,#95387,#95388,#95389,#95390,#95391,
#95392,#95393,#95394,#95395,#95396,#95397,#95398,#95399,#95400,#95401,#95402,
#95403,#95404,#95405,#95406,#95407,#95408,#95409,#95410,#95411,#95412,#95413,
#95414,#95415,#95416,#95417,#95418,#95419,#95420,#95421,#95422,#95423,#95424,
#95425,#95426,#95427,#95428,#95429,#95430,#95431,#95432,#95433,#95434,#95435,
#95436,#95437,#95438,#95439,#95440,#95441,#95442,#95443,#95444,#95445,#95446,
#95447,#95448,#95449,#95450,#95451,#95452,#95453,#95454,#95455,#95456,#95457,
#95458,#95459,#95460,#95461,#95462,#95463,#95464,#95465,#95466,#95467,#95468,
#95469,#95470,#95471,#95472,#95473,#95474,#95475,#95476,#95477,#95478,#95479,
#95480,#95481,#95482,#95483,#95484,#95485,#95486,#95487,#95488,#95489,#95490,
#95491,#95492,#95493,#95494,#95495,#95496,#95497,#95498,#95499,#95500,#95501,
#95502,#95503,#95504,#95505,#95506,#95507,#95508,#95509,#95510,#95511,#95512,
#95513,#95514,#95515,#95516,#95517,#95518,#95519,#95520,#95521,#95522,#95523,
#95524,#95525,#95526,#95527,#95528,#95529,#95530,#95531,#95532,#95533,#95534,
#95535,#95536,#95537,#95538,#95539,#95540,#95541,#95542,#95543,#95544,#95545,
#95546,#95547,#95548,#95549,#95550,#95551,#95552,#95553,#95554,#95555,#95556,
#95557,#95558,#95559,#95560,#95561,#95562,#95563,#95564,#95565,#95566,#95567,
#95568),.UNSPECIFIED.,.F.,.F.,(4,2,2,2,2,2,2,2,2,2,2,2,2,2,2,2,2,2,2,2,
2,2,2,2,2,2,2,2,2,2,2,2,2,2,2,2,2,2,2,2,2,2,2,2,2,2,2,2,2,2,2,2,2,2,2,2,
2,2,2,2,2,2,2,2,2,2,2,2,2,2,2,2,2,2,2,2,2,2,2,2,2,2,2,2,2,2,2,2,2,2,2,2,
2,2,2,2,2,2,2,2,2,4),(-1.90752595100115,-1.88362007859244,-1.87112823595947,
-1.86923240311331,-1.86822682861868,-1.86738863321829,-1.86633766927285,
-1.86468173537945,-1.8557597745918,-1.83061280324773,-1.82000118008745,
-1.81545898028867,-1.81189055818152,-1.81005141379379,-1.80855615675114,
-1.80683182606532,-1.80388768999709,-1.79176290704775,-1.76603521218253,
-1.75475694109299,-1.75219701800133,-1.75106212471271,-1.75021593980457,
-1.74926644958552,-1.74763045583421,-1.74153093645605,-1.70930448767715,
-1.69684311878572,-1.69395531811923,-1.69226035765088,-1.69076196957358,
-1.68888136103131,-1.68593406072472,-1.66747583626637,-1.64456837248137,
-1.63601254258091,-1.63427770759079,-1.63330661495954,-1.63246496521011,
-1.63138569179719,-1.62959662607504,-1.61723848958478,-1.58779912984415,
-1.57887860735567,-1.57627473302151,-1.57464193181266,-1.57312906146327,
-1.57116451827422,-1.56786265759568,-1.54203959778174,-1.52568792496754,
-1.52084946018167,-1.51761716182718,-1.51637162997539,-1.51550684957953,
-1.51471173461568,-1.51359879543186,-1.51066130463228,-1.49252208165286,
-1.47691089020177,-1.46721161593233,-1.46085672556273,-1.45855022034882,
-1.45698086817229,-1.45545090116724,-1.45360756069512,-1.449118910736,-1.42706666905852,
-1.40284243785337,-1.40011138653267,-1.3990297660391,-1.39824275966789,
-1.39736994698105,-1.39608427528726,-1.39257836425615,-1.37040107937369,
-1.34728885334641,-1.34274930355675,-1.34074733930023,-1.33922838715297,
-1.3376109883521,-1.33507819770006,-1.32685280826892,-1.29689557226867,
-1.29025670941099,-1.28366196973957,-1.28200159105016,-1.28103707627179,
-1.28027871311056,-1.27921745288886,-1.27704907926542,-1.2560123952169,
-1.22970667905637,-1.22526151599802,-1.22327608557229,-1.22175977128464,
-1.22013558524442,-1.21757185672893,-1.20905283779287,-1.179309962143,-1.16675301095494,
-1.16578625258722),.UNSPECIFIED.);
#1497=B_SPLINE_CURVE_WITH_KNOTS('',3,(#95569,#95570,#95571,#95572,#95573,
#95574,#95575,#95576,#95577,#95578,#95579,#95580,#95581,#95582,#95583,#95584,
#95585,#95586,#95587,#95588,#95589,#95590,#95591,#95592,#95593,#95594,#95595,
#95596,#95597,#95598,#95599,#95600,#95601,#95602,#95603,#95604,#95605,#95606,
#95607,#95608,#95609,#95610,#95611,#95612,#95613,#95614,#95615,#95616,#95617,
#95618,#95619,#95620,#95621,#95622,#95623,#95624,#95625,#95626,#95627,#95628,
#95629,#95630,#95631,#95632,#95633,#95634,#95635,#95636,#95637,#95638,#95639,
#95640,#95641,#95642,#95643,#95644,#95645,#95646,#95647,#95648,#95649,#95650,
#95651,#95652,#95653,#95654,#95655,#95656,#95657,#95658,#95659,#95660,#95661,
#95662,#95663,#95664,#95665,#95666,#95667,#95668,#95669,#95670,#95671,#95672,
#95673,#95674,#95675,#95676,#95677,#95678,#95679,#95680,#95681,#95682,#95683,
#95684,#95685,#95686,#95687,#95688,#95689,#95690,#95691,#95692,#95693,#95694,
#95695,#95696,#95697,#95698,#95699,#95700,#95701,#95702,#95703,#95704,#95705,
#95706,#95707,#95708,#95709,#95710,#95711,#95712,#95713,#95714,#95715,#95716,
#95717,#95718,#95719,#95720,#95721,#95722,#95723,#95724,#95725,#95726,#95727,
#95728,#95729,#95730,#95731,#95732,#95733,#95734,#95735,#95736,#95737,#95738,
#95739,#95740,#95741,#95742,#95743,#95744,#95745,#95746,#95747,#95748,#95749,
#95750,#95751,#95752,#95753,#95754,#95755,#95756,#95757,#95758,#95759,#95760,
#95761,#95762,#95763,#95764,#95765,#95766,#95767,#95768,#95769,#95770,#95771,
#95772,#95773,#95774,#95775,#95776,#95777,#95778,#95779,#95780,#95781,#95782,
#95783,#95784,#95785,#95786,#95787,#95788,#95789,#95790),.UNSPECIFIED.,
 .F.,.F.,(4,2,2,2,2,2,2,2,2,2,2,2,2,2,2,2,2,2,2,2,2,2,2,2,2,2,2,2,2,2,2,
2,2,2,2,2,2,2,2,2,2,2,2,2,2,2,2,2,2,2,2,2,2,2,2,2,2,2,2,2,2,2,2,2,2,2,2,
2,2,2,2,2,2,2,2,2,2,2,2,2,2,2,2,2,2,2,2,2,2,2,2,2,2,2,2,2,2,2,2,2,2,2,2,
2,2,2,2,2,2,2,4),(-2.43011734130913,-2.41481597979633,-2.39735880329152,
-2.3951857239436,-2.39412332080614,-2.39336474106553,-2.39240087403877,
-2.39074293165702,-2.38417507960966,-2.37754099977846,-2.34765118013879,
-2.33936461579502,-2.33682578563583,-2.33520738364571,-2.33368949355389,
-2.33169186189631,-2.32717517701453,-2.30262989511402,-2.28628960318989,
-2.2814530635049,-2.27822188698461,-2.27697677552855,-2.27611229495503,
-2.27531751752274,-2.27420510798581,-2.27126957426423,-2.25308987489998,
-2.23741153811376,-2.22777208390113,-2.22144585230775,-2.21914379736487,
-2.21757578345002,-2.21604583130719,-2.21385756719043,-2.2098303906548,
-2.18405653985788,-2.16250179614377,-2.16033255818783,-2.15927139526951,
-2.15851328196107,-2.15754930103005,-2.15589057139364,-2.14931192937181,
-2.14267957413884,-2.11279472797624,-2.10450682264593,-2.10196773305272,
-2.10034919926566,-2.09883120778007,-2.09683347215035,-2.09231665468224,
-2.06780511780435,-2.0514485793426,-2.04660938853951,-2.04337679968161,
-2.04213131911732,-2.04126663773164,-2.0404717332308,-2.0393591730667,-2.0364234808381,
-2.01824308175593,-2.00256287380938,-1.99292551321565,-1.98660010744146,
-1.98429796104629,-1.98272976567177,-1.9811995425484,-1.97901072271622,
-1.97498207079746,-1.94923880548864,-1.92765532393432,-1.9254858153486,
-1.92442451582824,-1.92366634347788,-1.92270237944221,-1.92104366308279,
-1.91446490803787,-1.90783238510119,-1.87794963104795,-1.86965969423404,
-1.86712048027951,-1.86550198325893,-1.86398410929363,-1.86198665203645,
-1.85747102856351,-1.83290660094356,-1.81658592119984,-1.81175256170352,
-1.8085229096544,-1.80727793881097,-1.80641340280718,-1.80561840504782,
-1.80450551193352,-1.80156717702645,-1.78343911347554,-1.76785126220425,
-1.75812539288814,-1.75384296291085,-1.75043697141373,-1.74863147700218,
-1.74715220089815,-1.74540650430903,-1.74236735281841,-1.72878470509405,
-1.70397250207422,-1.69608978396245,-1.69300705029047,-1.69071388327278,
-1.68962851881294,-1.68879575725663,-1.68837727951077),.UNSPECIFIED.);
#1498=B_SPLINE_CURVE_WITH_KNOTS('',3,(#95795,#95796,#95797,#95798,#95799,
#95800,#95801,#95802,#95803,#95804,#95805,#95806,#95807,#95808,#95809,#95810,
#95811,#95812,#95813,#95814,#95815,#95816,#95817,#95818,#95819,#95820,#95821,
#95822,#95823,#95824,#95825,#95826,#95827,#95828,#95829,#95830,#95831,#95832,
#95833,#95834,#95835,#95836,#95837,#95838,#95839,#95840,#95841,#95842,#95843,
#95844,#95845,#95846,#95847,#95848,#95849,#95850,#95851,#95852,#95853,#95854,
#95855,#95856,#95857,#95858,#95859,#95860,#95861,#95862,#95863,#95864,#95865,
#95866,#95867,#95868,#95869,#95870,#95871,#95872,#95873,#95874,#95875,#95876,
#95877,#95878,#95879,#95880,#95881,#95882,#95883,#95884,#95885,#95886,#95887,
#95888,#95889,#95890,#95891,#95892,#95893,#95894,#95895,#95896,#95897,#95898,
#95899,#95900,#95901,#95902,#95903,#95904,#95905,#95906,#95907,#95908,#95909,
#95910,#95911,#95912,#95913,#95914,#95915,#95916,#95917,#95918,#95919,#95920,
#95921,#95922,#95923,#95924,#95925,#95926,#95927,#95928,#95929,#95930,#95931,
#95932,#95933,#95934,#95935,#95936,#95937,#95938,#95939,#95940,#95941,#95942,
#95943,#95944,#95945,#95946,#95947,#95948,#95949,#95950,#95951,#95952,#95953,
#95954,#95955,#95956,#95957,#95958,#95959,#95960,#95961,#95962,#95963,#95964,
#95965,#95966,#95967,#95968,#95969,#95970,#95971,#95972,#95973,#95974,#95975,
#95976,#95977,#95978,#95979,#95980,#95981,#95982,#95983,#95984,#95985,#95986,
#95987,#95988,#95989,#95990,#95991,#95992,#95993,#95994,#95995,#95996,#95997,
#95998,#95999,#96000,#96001,#96002,#96003,#96004,#96005,#96006,#96007,#96008,
#96009,#96010),.UNSPECIFIED.,.F.,.F.,(4,2,2,2,2,2,2,2,2,2,2,2,2,2,2,2,2,
2,2,2,2,2,2,2,2,2,2,2,2,2,2,2,2,2,2,2,2,2,2,2,2,2,2,2,2,2,2,2,2,2,2,2,2,
2,2,2,2,2,2,2,2,2,2,2,2,2,2,2,2,2,2,2,2,2,2,2,2,2,2,2,2,2,2,2,2,2,2,2,2,
2,2,2,2,2,2,2,2,2,2,2,2,2,2,2,2,2,2,4),(-2.64925299467486,-2.64439351024018,
-2.63565889459159,-2.63307331472224,-2.63144440576356,-2.62992995093017,
-2.62795594218273,-2.62357474183728,-2.59619746795857,-2.57586934090486,
-2.57385329507439,-2.57282268699081,-2.57206719318075,-2.57107948403193,
-2.56931753007274,-2.56131765817323,-2.53100239768952,-2.51876962769625,
-2.51589668789644,-2.51420488438948,-2.51270589196559,-2.51081999124654,
-2.50785545885685,-2.48503067071668,-2.46864116774041,-2.46155619862553,
-2.45868673852026,-2.45651796612064,-2.45545665759374,-2.45469832475683,
-2.45373392202227,-2.45207391558962,-2.44548261860415,-2.43885340813565,
-2.40892171742417,-2.40068743612303,-2.39815377975433,-2.39653623048402,
-2.3950174179726,-2.39301604707854,-2.38847968822856,-2.36676311390131,
-2.34820482573476,-2.34302860948065,-2.33963065150869,-2.33836052006936,
-2.3374908864139,-2.33670096754575,-2.33560785923745,-2.33280833504335,
-2.30996599499759,-2.28482659429243,-2.2814493210076,-2.27964963938307,
-2.27817035326332,-2.27641902530293,-2.27335569285477,-2.25930627414214,
-2.22659252383275,-2.22377608093784,-2.22163863865929,-2.22058351565617,
-2.21982582960366,-2.21885704792273,-2.21717808546918,-2.21035518688709,
-2.17887351667309,-2.16649564916164,-2.163613189024,-2.16191934049744,-2.16042070496863,
-2.15853814660727,-2.15558456668745,-2.13680309970434,-2.1141775387529,
-2.10847936773302,-2.10483354671467,-2.1035283383505,-2.1026514869268,-2.10186792572786,
-2.1008000089707,-2.09814943393302,-2.0730549085317,-2.05289726207563,-2.04756503052882,
-2.0454086436735,-2.04386887570229,-2.0424735113764,-2.04026180869694,-2.03614825122908,
-2.01376601227614,-2.00366217768058,-1.98994878542966,-1.98713101531951,
-1.98595149737698,-1.98509858985585,-1.98417003067989,-1.98262854204101,
-1.97746256902453,-1.9543775990238,-1.93298772212286,-1.92934500580595,
-1.92749086290136,-1.92599465069147,-1.92428157668236,-1.92138652203456,
-1.90998773984318,-1.90752595100115),.UNSPECIFIED.);
#1499=B_SPLINE_CURVE_WITH_KNOTS('',3,(#96011,#96012,#96013,#96014,#96015,
#96016,#96017,#96018,#96019,#96020,#96021,#96022,#96023,#96024,#96025,#96026,
#96027,#96028,#96029,#96030,#96031,#96032,#96033,#96034,#96035,#96036,#96037,
#96038,#96039,#96040,#96041,#96042,#96043,#96044,#96045,#96046,#96047,#96048,
#96049,#96050,#96051,#96052,#96053,#96054,#96055,#96056,#96057,#96058,#96059,
#96060,#96061,#96062,#96063,#96064,#96065,#96066,#96067,#96068,#96069,#96070,
#96071,#96072,#96073,#96074,#96075,#96076,#96077,#96078,#96079,#96080,#96081,
#96082,#96083,#96084,#96085,#96086,#96087,#96088,#96089,#96090,#96091,#96092,
#96093,#96094,#96095,#96096,#96097,#96098,#96099,#96100,#96101,#96102,#96103,
#96104,#96105,#96106,#96107,#96108,#96109,#96110,#96111,#96112,#96113,#96114,
#96115,#96116,#96117,#96118,#96119,#96120,#96121,#96122,#96123,#96124,#96125,
#96126,#96127,#96128,#96129,#96130,#96131,#96132,#96133,#96134,#96135,#96136,
#96137,#96138,#96139,#96140,#96141,#96142,#96143,#96144,#96145,#96146,#96147,
#96148,#96149,#96150,#96151,#96152,#96153,#96154,#96155,#96156,#96157,#96158,
#96159,#96160,#96161,#96162,#96163,#96164,#96165,#96166,#96167,#96168,#96169,
#96170,#96171,#96172,#96173,#96174,#96175,#96176,#96177,#96178,#96179,#96180,
#96181,#96182,#96183,#96184,#96185,#96186,#96187,#96188,#96189,#96190,#96191,
#96192,#96193,#96194,#96195,#96196,#96197,#96198,#96199,#96200,#96201,#96202,
#96203,#96204,#96205,#96206,#96207,#96208,#96209,#96210,#96211,#96212,#96213,
#96214,#96215,#96216,#96217,#96218),.UNSPECIFIED.,.F.,.F.,(4,2,2,2,2,2,
2,2,2,2,2,2,2,2,2,2,2,2,2,2,2,2,2,2,2,2,2,2,2,2,2,2,2,2,2,2,2,2,2,2,2,2,
2,2,2,2,2,2,2,2,2,2,2,2,2,2,2,2,2,2,2,2,2,2,2,2,2,2,2,2,2,2,2,2,2,2,2,2,
2,2,2,2,2,2,2,2,2,2,2,2,2,2,2,2,2,2,2,2,2,2,2,2,2,4),(-1.68837727951077,
-1.68781998827758,-1.68610979525433,-1.67886635089715,-1.64780264548136,
-1.63547486615305,-1.63259618872471,-1.63090345529188,-1.62940513817301,
-1.62752209583028,-1.62456603543931,-1.60208463247758,-1.58604837104348,
-1.58328776244323,-1.57479403079398,-1.57300287084039,-1.57200878358889,
-1.57117010413174,-1.57010575287063,-1.56792058347704,-1.54999750431417,
-1.5201389670866,-1.51600081545764,-1.5140714746315,-1.51256409693759,-1.51091542116062,
-1.50823770536098,-1.49852389736165,-1.48002805574701,-1.45910579318059,
-1.45621523972934,-1.45510858376549,-1.45431526753437,-1.45344932519703,
-1.45219699867077,-1.44891827769304,-1.44398634083731,-1.42704748350368,
-1.40332169062381,-1.39878941643496,-1.39678907942413,-1.39527075619288,
-1.39365345110996,-1.39111961347584,-1.38288005792432,-1.35294259185594,
-1.34630432348075,-1.33970486856746,-1.3380444022016,-1.3370800401523,-1.33632193093201,
-1.33526121958634,-1.33309467692154,-1.3127563740379,-1.28568157624691,
-1.28128131800398,-1.27930424410242,-1.27778965052923,-1.27616276355083,
-1.27358506945204,-1.26492447566055,-1.23529328123922,-1.22278897324005,
-1.22099485422695,-1.21991420100556,-1.21907253005077,-1.2181026569478,
-1.21637298908872,-1.20790641209283,-1.18553319150925,-1.1664777146516,
-1.16352049009428,-1.16163701279139,-1.16013855537909,-1.15844588210301,
-1.15556785209376,-1.14325333290793,-1.11232117755965,-1.10492188802842,
-1.10320050946234,-1.10222212669995,-1.10138161656133,-1.10029535559583,
-1.09799783477396,-1.09490794205804,-1.0869986496557,-1.06205865171597,
-1.04864715763952,-1.04561679310036,-1.04387296233757,-1.04239341535756,
-1.04058530574585,-1.03716735423768,-1.0121242096119,-0.989206628751375,
-0.986409617298101,-0.98531692822558,-0.984527124500201,-0.983657402301642,
-0.982386808912438,-0.978985619553725,-0.973803504429689,-0.955204122596725,
-0.946563016930913),.UNSPECIFIED.);
#1500=B_SPLINE_CURVE_WITH_KNOTS('',3,(#96224,#96225,#96226,#96227,#96228,
#96229,#96230,#96231,#96232,#96233,#96234,#96235,#96236,#96237,#96238,#96239,
#96240,#96241,#96242,#96243,#96244,#96245,#96246,#96247,#96248,#96249,#96250,
#96251,#96252,#96253,#96254,#96255,#96256,#96257,#96258,#96259,#96260,#96261,
#96262,#96263,#96264,#96265,#96266,#96267,#96268,#96269,#96270,#96271,#96272,
#96273,#96274,#96275,#96276,#96277,#96278,#96279,#96280,#96281,#96282,#96283,
#96284,#96285,#96286,#96287,#96288,#96289,#96290,#96291,#96292,#96293,#96294,
#96295,#96296,#96297,#96298,#96299,#96300,#96301,#96302,#96303,#96304,#96305,
#96306,#96307,#96308,#96309,#96310,#96311,#96312,#96313,#96314,#96315,#96316,
#96317,#96318,#96319,#96320,#96321,#96322,#96323,#96324,#96325,#96326,#96327,
#96328,#96329,#96330,#96331,#96332,#96333,#96334,#96335,#96336,#96337,#96338,
#96339,#96340,#96341,#96342,#96343,#96344,#96345,#96346,#96347,#96348,#96349,
#96350,#96351,#96352,#96353,#96354,#96355,#96356,#96357,#96358,#96359,#96360,
#96361,#96362,#96363,#96364,#96365,#96366,#96367,#96368,#96369,#96370,#96371,
#96372,#96373,#96374,#96375,#96376,#96377,#96378,#96379,#96380,#96381,#96382,
#96383,#96384,#96385,#96386,#96387,#96388,#96389),.UNSPECIFIED.,.F.,.F.,
(4,2,2,2,2,2,2,2,2,2,2,2,2,2,2,2,2,2,2,2,2,2,2,2,2,2,2,2,2,2,2,2,2,2,2,
2,2,2,2,2,2,2,2,2,2,2,2,2,2,2,2,2,2,2,2,2,2,2,2,2,2,2,2,2,2,2,2,2,2,2,2,
2,2,2,2,2,2,2,2,2,2,2,4),(-0.537654944100775,-0.535789434415299,-0.530947381133612,
-0.514580167551101,-0.490084584660939,-0.485565321528231,-0.483566236081426,
-0.482047101143448,-0.480427231448254,-0.477885793525669,-0.469587853842892,
-0.439665187161532,-0.433016535679776,-0.426451903678453,-0.424793424927305,
-0.423829021551239,-0.423070125063847,-0.422007310375762,-0.419832860044324,
-0.402343849447898,-0.371897899064157,-0.367826861984351,-0.365888215743501,
-0.364382717444537,-0.362719887114946,-0.35998196007451,-0.349584623386473,
-0.32960290970421,-0.310991294368649,-0.308059469310665,-0.306946758269144,
-0.306151391360009,-0.305285841775843,-0.304038405518085,-0.300796693331405,
-0.29594092366606,-0.279489546469263,-0.255103847963886,-0.250581519354464,
-0.248581854820801,-0.247062582934163,-0.245442858781237,-0.242902261654239,
-0.234612787780911,-0.204682516993568,-0.198034421772961,-0.191465316403598,
-0.189806424106082,-0.188841905400883,-0.188082996306437,-0.187020265440863,
-0.184846351190446,-0.167378181365044,-0.136903367542583,-0.132835647464107,
-0.130897590697415,-0.129445614808312,-0.129398584673514,-0.129342416684613,
-0.129302777728965,-0.129274889351391,-0.129240549353893,-0.12756818050583,
-0.124705725681973,-0.12122400083898,-0.114021254191121,-0.0911078939858096,
-0.0745667805052817,-0.0725599365381608,-0.0715177521615853,-0.0706793631632185,
-0.0696648629221745,-0.0677282820327141,-0.0537098029930007,-0.0275392113435695,
-0.0171711065967806,-0.0144304378264026,-0.0127669742247786,-0.0113088240864444,
-0.0098533766463521,-0.00798939879024556,-0.00478412906894591,-9.99999999917733E-7),
 .UNSPECIFIED.);
#1501=B_SPLINE_CURVE_WITH_KNOTS('',3,(#96390,#96391,#96392,#96393,#96394,
#96395,#96396,#96397,#96398,#96399,#96400,#96401,#96402,#96403,#96404,#96405,
#96406,#96407,#96408,#96409,#96410,#96411,#96412,#96413,#96414,#96415,#96416,
#96417,#96418,#96419,#96420,#96421,#96422,#96423,#96424,#96425,#96426,#96427,
#96428,#96429,#96430,#96431,#96432,#96433,#96434,#96435,#96436,#96437,#96438,
#96439,#96440,#96441,#96442,#96443),.UNSPECIFIED.,.F.,.F.,(4,2,2,2,2,2,
2,2,2,2,2,2,2,2,2,2,2,2,2,2,2,2,2,2,2,2,4),(-2.85368559544924,-2.81938608199108,
-2.81030961351792,-2.80854721642627,-2.80757009001122,-2.80672923804291,
-2.80564065848723,-2.80385950953547,-2.79173942507301,-2.7625979824271,
-2.75637958199243,-2.75323833338059,-2.75061443207407,-2.74900757992761,
-2.74758466130194,-2.74570140373577,-2.74274564548966,-2.7239293707165,
-2.70133497900864,-2.69283039418367,-2.69109827123299,-2.69012771407087,
-2.68928588651286,-2.68820557349282,-2.68641312434399,-2.67396368254774,
-2.64925299467486),.UNSPECIFIED.);
#1502=B_SPLINE_CURVE_WITH_KNOTS('',3,(#96444,#96445,#96446,#96447,#96448,
#96449,#96450,#96451,#96452,#96453,#96454,#96455,#96456,#96457,#96458,#96459,
#96460,#96461,#96462,#96463,#96464,#96465,#96466,#96467,#96468,#96469,#96470,
#96471,#96472,#96473,#96474,#96475,#96476,#96477,#96478,#96479,#96480,#96481,
#96482,#96483,#96484,#96485,#96486,#96487,#96488,#96489,#96490,#96491,#96492,
#96493,#96494,#96495,#96496,#96497,#96498,#96499,#96500,#96501,#96502,#96503,
#96504,#96505,#96506,#96507,#96508,#96509,#96510,#96511,#96512,#96513,#96514,
#96515,#96516,#96517,#96518,#96519,#96520,#96521,#96522,#96523,#96524,#96525,
#96526,#96527,#96528,#96529,#96530,#96531,#96532,#96533,#96534,#96535,#96536,
#96537,#96538,#96539,#96540,#96541,#96542,#96543,#96544,#96545,#96546,#96547,
#96548,#96549,#96550,#96551,#96552,#96553,#96554,#96555,#96556,#96557,#96558,
#96559,#96560,#96561,#96562,#96563,#96564,#96565,#96566,#96567,#96568,#96569,
#96570,#96571,#96572,#96573,#96574,#96575,#96576,#96577,#96578,#96579,#96580,
#96581,#96582,#96583,#96584,#96585,#96586,#96587,#96588,#96589,#96590,#96591,
#96592,#96593,#96594,#96595,#96596,#96597,#96598,#96599,#96600,#96601,#96602,
#96603,#96604,#96605,#96606,#96607,#96608,#96609,#96610,#96611,#96612,#96613,
#96614,#96615,#96616,#96617,#96618,#96619,#96620,#96621,#96622,#96623,#96624,
#96625,#96626,#96627,#96628,#96629,#96630,#96631,#96632,#96633,#96634,#96635,
#96636,#96637,#96638,#96639,#96640,#96641,#96642,#96643,#96644,#96645,#96646,
#96647,#96648,#96649,#96650,#96651,#96652,#96653,#96654,#96655,#96656,#96657,
#96658,#96659,#96660,#96661),.UNSPECIFIED.,.F.,.F.,(4,2,2,2,2,2,2,2,2,2,
2,2,2,2,2,2,2,2,2,2,2,2,2,2,2,2,2,2,2,2,2,2,2,2,2,2,2,2,2,2,2,2,2,2,2,2,
2,2,2,2,2,2,2,2,2,2,2,2,2,2,2,2,2,2,2,2,2,2,2,2,2,2,2,2,2,2,2,2,2,2,2,2,
2,2,2,2,2,2,2,2,2,2,2,2,2,2,2,2,2,2,2,2,2,2,2,2,2,2,4),(-0.946563016930913,
-0.933543375261107,-0.929009140367105,-0.927008139137741,-0.925489390025472,
-0.923871706480782,-0.921337433505994,-0.913097924492891,-0.883150834223557,
-0.876511016857133,-0.869908544931653,-0.868247532108279,-0.867282889721922,
-0.86652458230784,-0.865463623065431,-0.863296681852881,-0.843047106167405,
-0.815859994076131,-0.811465573806204,-0.809489222871741,-0.807974422528057,
-0.806346569401789,-0.803765748407679,-0.795078739523885,-0.765456565894513,
-0.752960370416633,-0.751166189901932,-0.750085369736987,-0.749243486889604,
-0.748273273917912,-0.746542772802078,-0.738067268495438,-0.71564853254054,
-0.69663361684836,-0.69367624316458,-0.691792456537885,-0.690293617109017,
-0.688600367667036,-0.685721000716398,-0.673394577760545,-0.642384729066529,
-0.635053489863898,-0.633336554734155,-0.632359027962573,-0.631526147626519,
-0.630442426595042,-0.628159064392551,-0.625093902727327,-0.617280252282636,
-0.592803719098889,-0.578825766515184,-0.57576553179727,-0.574014653615267,
-0.572534992457822,-0.570733936579166,-0.56735132820757,-0.563106045903372,
-0.553505071266121,-0.537759260907421,-0.519534548142031,-0.516597706164644,
-0.515484669052243,-0.514689428041729,-0.513824441598386,-0.512578544540572,
-0.509344914334808,-0.50450484478626,-0.48814701270472,-0.463638893578981,
-0.459120691590664,-0.457122255418734,-0.455603693883614,-0.453984518406383,
-0.451444357169866,-0.443152646648182,-0.413237651196606,-0.406592022840417,
-0.40001261636984,-0.398353305966229,-0.397388938362001,-0.396630401853502,
-0.395568544255559,-0.393397696789795,-0.376015086200967,-0.345430838764617,
-0.341378160289219,-0.339443452728329,-0.337938936622103,-0.336275088590443,
-0.333530621562447,-0.323045066780609,-0.302752436624759,-0.284564297864742,
-0.281625701240686,-0.280512417965607,-0.279717095485449,-0.278852129075036,
-0.277606440116836,-0.274374345786027,-0.269537420335027,-0.253199354551679,
-0.228663201841218,-0.224145795664896,-0.222147460249137,-0.220628877206173,
-0.219009584431811,-0.21646904090926,-0.208174229584812,-0.204517382372539),
 .UNSPECIFIED.);
#1503=B_SPLINE_CURVE_WITH_KNOTS('',3,(#96666,#96667,#96668,#96669,#96670,
#96671,#96672,#96673,#96674,#96675,#96676,#96677,#96678,#96679,#96680,#96681,
#96682,#96683,#96684,#96685,#96686,#96687,#96688,#96689,#96690,#96691,#96692,
#96693,#96694,#96695,#96696,#96697,#96698,#96699,#96700,#96701,#96702,#96703,
#96704,#96705,#96706,#96707,#96708,#96709,#96710,#96711,#96712,#96713,#96714,
#96715,#96716,#96717,#96718,#96719,#96720,#96721,#96722,#96723,#96724,#96725,
#96726,#96727,#96728,#96729,#96730,#96731,#96732,#96733,#96734,#96735,#96736,
#96737,#96738,#96739,#96740,#96741,#96742,#96743,#96744,#96745,#96746,#96747,
#96748,#96749,#96750,#96751,#96752,#96753,#96754,#96755,#96756,#96757,#96758,
#96759,#96760,#96761,#96762,#96763,#96764,#96765,#96766,#96767,#96768,#96769,
#96770,#96771,#96772,#96773,#96774,#96775,#96776,#96777,#96778,#96779,#96780,
#96781,#96782,#96783,#96784,#96785,#96786,#96787,#96788,#96789,#96790,#96791,
#96792,#96793,#96794,#96795,#96796,#96797,#96798,#96799,#96800,#96801,#96802,
#96803,#96804,#96805,#96806,#96807,#96808,#96809,#96810,#96811,#96812,#96813,
#96814,#96815,#96816,#96817,#96818,#96819,#96820,#96821,#96822,#96823,#96824,
#96825,#96826,#96827,#96828,#96829,#96830,#96831,#96832,#96833,#96834,#96835,
#96836,#96837,#96838,#96839,#96840,#96841,#96842,#96843,#96844,#96845,#96846,
#96847,#96848,#96849,#96850,#96851,#96852,#96853,#96854,#96855,#96856,#96857,
#96858,#96859,#96860,#96861,#96862,#96863,#96864,#96865,#96866,#96867,#96868,
#96869,#96870,#96871,#96872,#96873,#96874,#96875,#96876,#96877,#96878,#96879,
#96880,#96881,#96882,#96883,#96884,#96885),.UNSPECIFIED.,.F.,.F.,(4,2,2,
2,2,2,2,2,2,2,2,2,2,2,2,2,2,2,2,2,2,2,2,2,2,2,2,2,2,2,2,2,2,2,2,2,2,2,2,
2,2,2,2,2,2,2,2,2,2,2,2,2,2,2,2,2,2,2,2,2,2,2,2,2,2,2,2,2,2,2,2,2,2,2,2,
2,2,2,2,2,2,2,2,2,2,2,2,2,2,2,2,2,2,2,2,2,2,2,2,2,2,2,2,2,2,2,2,2,2,4),
(-1.27975427727725,-1.25199137047719,-1.2493861684092,-1.24795605413082,
-1.24670473500885,-1.24583850733499,-1.24504412631629,-1.24393492438005,
-1.24102936833812,-1.22046684545241,-1.20604336971845,-1.19705571217952,
-1.19107438868889,-1.18890711482678,-1.18750659945926,-1.18598938184144,
-1.1840015550619,-1.1795458133282,-1.15278914018882,-1.13808430320792,-1.13352500983649,
-1.13048617808367,-1.1292388225823,-1.12837334061542,-1.1275780416231,-1.12646544340642,
-1.12353385323737,-1.10513420448383,-1.08501620582852,-1.07457982324743,
-1.0718388463062,-1.07017541104046,-1.06867016562359,-1.06673296820058,
-1.06266921959483,-1.03214972768199,-1.01469977961972,-1.01252640859014,
-1.0114638338231,-1.01070499668163,-1.00974050140096,-1.00808152619519,
-1.00151007460853,-0.994872770029299,-0.964961008133719,-0.956673173050825,
-0.95413287521227,-0.952513280162439,-0.950994084821972,-0.948994454910477,
-0.944471949744033,-0.920058519159929,-0.903610202969209,-0.898754773236036,
-0.895513561965845,-0.894266237093875,-0.893400744325761,-0.892605409700215,
-0.891492727669283,-0.888560634559187,-0.869868832058371,-0.849969375697545,
-0.839595815676233,-0.836859956359817,-0.835197614040961,-0.833692061380742,
-0.831752648806168,-0.827677395399033,-0.797246780094766,-0.779727540466477,
-0.777552150100562,-0.776489160180354,-0.77573025909539,-0.774766001104869,
-0.773108124239889,-0.766550115246269,-0.759910112492467,-0.730018557154092,
-0.721702483369917,-0.719159148492118,-0.717538865773099,-0.716019899224641,
-0.714021844164187,-0.709508502666446,-0.684765956089572,-0.676101493216078,
-0.661861018297902,-0.659919396433078,-0.658903881336649,-0.658065571402876,
-0.65702462922252,-0.655023386087201,-0.639862526826004,-0.633171124375001,
-0.607483957067017,-0.603451721784349,-0.601261030727202,-0.599729540785908,
-0.598160074139939,-0.595856103905065,-0.589525912707429,-0.579879704757375,
-0.564181223881447,-0.545983606284509,-0.543045109004461,-0.541931575654508,
-0.541136007376822,-0.540270683575712,-0.539024306948506,-0.537654944100775),
 .UNSPECIFIED.);
#1504=B_SPLINE_CURVE_WITH_KNOTS('',3,(#96887,#96888,#96889,#96890,#96891,
#96892,#96893,#96894,#96895,#96896,#96897,#96898,#96899,#96900,#96901,#96902,
#96903,#96904,#96905,#96906,#96907,#96908,#96909,#96910,#96911,#96912,#96913,
#96914,#96915,#96916,#96917,#96918,#96919,#96920,#96921,#96922,#96923,#96924,
#96925,#96926,#96927,#96928,#96929,#96930,#96931,#96932,#96933,#96934,#96935,
#96936,#96937,#96938,#96939,#96940,#96941,#96942),.UNSPECIFIED.,.F.,.F.,
(4,2,2,2,2,2,2,2,2,2,2,2,2,2,2,2,2,2,2,2,2,2,2,2,2,2,2,4),(-0.204517382372539,
-0.178260528710531,-0.171614465939901,-0.165036253785904,-0.163377013093062,
-0.162412645657632,-0.161654084114003,-0.160592158797679,-0.158421055664157,
-0.141031124508097,-0.110454985546614,-0.106401055436445,-0.104466078025292,
-0.102961494387479,-0.101362134321586,-0.0987650910074259,-0.0956616331105435,
-0.0895499348259312,-0.0726251376513031,-0.0493628884496759,-0.0465823321335659,
-0.0454922521321131,-0.0447029763573064,-0.0438322353545825,-0.0425574477223321,
-0.0391288503697206,-0.018101941217382,-9.99999999334866E-7),
 .UNSPECIFIED.);
#1505=B_SPLINE_CURVE_WITH_KNOTS('',3,(#96943,#96944,#96945,#96946,#96947,
#96948,#96949,#96950,#96951,#96952,#96953,#96954,#96955,#96956,#96957,#96958,
#96959,#96960,#96961,#96962,#96963,#96964,#96965,#96966,#96967,#96968,#96969,
#96970,#96971,#96972,#96973,#96974,#96975,#96976,#96977,#96978,#96979,#96980,
#96981,#96982,#96983,#96984,#96985,#96986,#96987,#96988,#96989,#96990,#96991,
#96992,#96993,#96994,#96995,#96996,#96997,#96998,#96999,#97000,#97001,#97002,
#97003,#97004,#97005,#97006,#97007,#97008,#97009,#97010,#97011,#97012,#97013,
#97014,#97015,#97016,#97017,#97018,#97019,#97020,#97021,#97022,#97023,#97024,
#97025,#97026,#97027,#97028,#97029,#97030,#97031,#97032,#97033,#97034,#97035,
#97036,#97037,#97038,#97039,#97040,#97041,#97042,#97043,#97044,#97045,#97046,
#97047,#97048,#97049,#97050,#97051,#97052,#97053,#97054,#97055,#97056,#97057,
#97058,#97059,#97060,#97061,#97062,#97063,#97064,#97065,#97066,#97067,#97068,
#97069,#97070,#97071,#97072,#97073,#97074,#97075,#97076,#97077,#97078,#97079,
#97080,#97081,#97082,#97083,#97084,#97085,#97086,#97087,#97088,#97089,#97090,
#97091,#97092,#97093,#97094,#97095,#97096,#97097,#97098,#97099,#97100,#97101,
#97102),.UNSPECIFIED.,.F.,.F.,(4,2,2,2,2,2,2,2,2,2,2,2,2,2,2,2,2,2,2,2,
2,2,2,2,2,2,2,2,2,2,2,2,2,2,2,2,2,2,2,2,2,2,2,2,2,2,2,2,2,2,2,2,2,2,2,2,
2,2,2,2,2,2,2,2,2,2,2,2,2,2,2,2,2,2,2,2,2,2,2,4),(-3.48624385780003,-3.47968930691364,
-3.47573880689191,-3.4740821909817,-3.47267806908479,-3.47117870449806,
-3.46928641528836,-3.46557720932842,-3.45535784924294,-3.4246234335228,
-3.41638808331368,-3.41467132645148,-3.41370418633071,-3.41286191236619,
-3.41177672076385,-3.40996730853489,-3.39662162732591,-3.37656970251867,
-3.36570710000715,-3.36109315356723,-3.35854379436467,-3.35631853704546,
-3.35478161598719,-3.35325072097044,-3.35105967957976,-3.34702365578681,
-3.32127602239909,-3.29969866281412,-3.29752868554427,-3.29646714030711,
-3.29570878577414,-3.29474457929997,-3.29308541795997,-3.28650451149845,
-3.27987065043401,-3.24997831033339,-3.24168967859122,-3.23915020974154,
-3.23753140328845,-3.23601313587224,-3.23401500982554,-3.22949720661632,
-3.20496895368156,-3.18861347599592,-3.18377395732304,-3.18054105197065,
-3.17929540993799,-3.17843059850735,-3.17763551326552,-3.176522697548,-3.17358625468488,
-3.15540160246922,-3.13971816419939,-3.13007749621605,-3.12375007188259,
-3.12144729179094,-3.119878693829,-3.11834810009179,-3.11615878867429,-3.11212932872914,
-3.08637810083257,-3.0647923385948,-3.06262229172352,-3.06156071783781,
-3.06080234503758,-3.05983811835208,-3.05817892877509,-3.05159799690581,
-3.04496395578766,-3.01507111257892,-3.00678201838198,-3.00424246137772,
-3.00262361065234,-3.00110531006374,-2.99910715253951,-2.99458933177557,
-2.9700572810668,-2.95370384307095,-2.94886460473741,-2.94874919963959),
 .UNSPECIFIED.);
#1506=B_SPLINE_CURVE_WITH_KNOTS('',3,(#97107,#97108,#97109,#97110,#97111,
#97112,#97113,#97114,#97115,#97116,#97117,#97118,#97119,#97120,#97121,#97122,
#97123,#97124,#97125,#97126,#97127,#97128,#97129,#97130,#97131,#97132,#97133,
#97134,#97135,#97136,#97137,#97138,#97139,#97140,#97141,#97142,#97143,#97144,
#97145,#97146,#97147,#97148,#97149,#97150,#97151,#97152,#97153,#97154,#97155,
#97156,#97157,#97158,#97159,#97160,#97161,#97162,#97163,#97164,#97165,#97166,
#97167,#97168,#97169,#97170,#97171,#97172,#97173,#97174,#97175,#97176,#97177,
#97178,#97179,#97180,#97181,#97182,#97183,#97184,#97185,#97186,#97187,#97188,
#97189,#97190,#97191,#97192,#97193,#97194,#97195,#97196,#97197,#97198,#97199,
#97200,#97201,#97202,#97203,#97204,#97205,#97206,#97207,#97208,#97209,#97210,
#97211,#97212,#97213,#97214,#97215,#97216,#97217,#97218,#97219,#97220,#97221,
#97222,#97223,#97224,#97225,#97226,#97227,#97228,#97229,#97230,#97231,#97232,
#97233,#97234,#97235,#97236,#97237,#97238,#97239,#97240,#97241,#97242,#97243,
#97244,#97245,#97246,#97247,#97248,#97249,#97250,#97251,#97252,#97253,#97254,
#97255,#97256,#97257,#97258,#97259,#97260,#97261,#97262,#97263,#97264,#97265,
#97266,#97267,#97268,#97269,#97270,#97271,#97272,#97273,#97274,#97275,#97276,
#97277,#97278,#97279,#97280,#97281,#97282,#97283,#97284,#97285,#97286,#97287,
#97288,#97289,#97290,#97291,#97292,#97293,#97294,#97295,#97296,#97297,#97298,
#97299,#97300,#97301,#97302,#97303,#97304,#97305,#97306,#97307,#97308,#97309,
#97310,#97311,#97312,#97313,#97314,#97315,#97316,#97317,#97318,#97319,#97320,
#97321,#97322,#97323,#97324,#97325,#97326),.UNSPECIFIED.,.F.,.F.,(4,2,2,
2,2,2,2,2,2,2,2,2,2,2,2,2,2,2,2,2,2,2,2,2,2,2,2,2,2,2,2,2,2,2,2,2,2,2,2,
2,2,2,2,2,2,2,2,2,2,2,2,2,2,2,2,2,2,2,2,2,2,2,2,2,2,2,2,2,2,2,2,2,2,2,2,
2,2,2,2,2,2,2,2,2,2,2,2,2,2,2,2,2,2,2,2,2,2,2,2,2,2,2,2,2,2,2,2,2,2,4),
(-0.742062510194801,-0.736873225342865,-0.732806069602463,-0.730868275943952,
-0.729363008565338,-0.727699996180712,-0.72496075667552,-0.714545192383826,
-0.694498614772829,-0.675978223068981,-0.67304653797817,-0.671933918317771,
-0.671138625410848,-0.6702731663647,-0.669025877113159,-0.665784639025209,
-0.660929657847286,-0.644481805877878,-0.620096036935879,-0.615574221659552,
-0.613574767187254,-0.612055648296152,-0.610436080905066,-0.607895716329152,
-0.599606876740267,-0.569679726799791,-0.563032275923686,-0.556463916494297,
-0.554805196987647,-0.553840776026411,-0.553081942139507,-0.552019314382996,
-0.549845603126137,-0.532378705361215,-0.501907393605616,-0.497840090088558,
-0.495902228388823,-0.494396909181205,-0.492733840575492,-0.489994510873881,
-0.479578635159875,-0.459531529393454,-0.441010289384183,-0.438078503971869,
-0.436965846175701,-0.436170525995552,-0.435305037253762,-0.434057705178371,
-0.430816355657519,-0.425961207439399,-0.409512788179206,-0.385126186769233,
-0.380604216274537,-0.378604693195326,-0.37708552218971,-0.37546589924846,
-0.372925447561444,-0.364636323943848,-0.334708147158132,-0.32806046827743,
-0.321491883378753,-0.319833106959273,-0.318868652911839,-0.318109792994398,
-0.317047128789903,-0.314873342988328,-0.297405846798249,-0.266933488780481,
-0.262866045864875,-0.260928117713057,-0.25942274687041,-0.257759621202867,
-0.255020197475023,-0.244603963763567,-0.224556167892638,-0.206034295759932,
-0.203102409772794,-0.201989713807829,-0.201194366344894,-0.200328847913545,
-0.199081473050705,-0.195840012343133,-0.190984697582693,-0.174535714125226,
-0.150164769065553,-0.145631444051202,-0.143629891320126,-0.142110342886935,
-0.140709614980209,-0.138492924912212,-0.132397383291039,-0.123186729675139,
-0.100865008703675,-0.0870939715360433,-0.0852858201090558,-0.0842006554811097,
-0.0833579376182,-0.0823897113833211,-0.0806696712496977,-0.072470763153566,
-0.0593359563225871,-0.045059337371504,-0.030476726664995,-0.027659988660972,
-0.0258184925403211,-0.0243222753918401,-0.0229115649271589,-0.0212193354767052,
-0.0187333837042564,-1.00000008385059E-6),.UNSPECIFIED.);
#1507=B_SPLINE_CURVE_WITH_KNOTS('',3,(#97327,#97328,#97329,#97330,#97331,
#97332,#97333,#97334,#97335,#97336,#97337,#97338,#97339,#97340,#97341,#97342,
#97343,#97344,#97345,#97346,#97347,#97348,#97349,#97350,#97351,#97352,#97353,
#97354,#97355,#97356,#97357,#97358,#97359,#97360,#97361,#97362,#97363,#97364,
#97365,#97366,#97367,#97368,#97369,#97370,#97371,#97372,#97373,#97374,#97375,
#97376,#97377,#97378,#97379,#97380,#97381,#97382,#97383,#97384,#97385,#97386,
#97387,#97388,#97389,#97390,#97391,#97392,#97393,#97394,#97395,#97396,#97397,
#97398,#97399,#97400,#97401,#97402,#97403,#97404,#97405,#97406,#97407,#97408,
#97409,#97410,#97411,#97412,#97413,#97414,#97415,#97416,#97417,#97418,#97419,
#97420,#97421,#97422,#97423,#97424,#97425,#97426,#97427,#97428,#97429,#97430,
#97431,#97432,#97433,#97434,#97435,#97436,#97437,#97438,#97439,#97440,#97441,
#97442,#97443,#97444,#97445,#97446,#97447,#97448,#97449,#97450,#97451,#97452,
#97453,#97454,#97455,#97456,#97457,#97458,#97459,#97460,#97461,#97462,#97463,
#97464,#97465,#97466,#97467,#97468,#97469,#97470,#97471,#97472,#97473,#97474,
#97475,#97476,#97477,#97478,#97479,#97480,#97481,#97482,#97483,#97484,#97485,
#97486,#97487,#97488,#97489,#97490,#97491,#97492,#97493,#97494,#97495,#97496,
#97497,#97498,#97499,#97500,#97501,#97502,#97503,#97504,#97505,#97506,#97507,
#97508,#97509,#97510,#97511,#97512,#97513,#97514,#97515,#97516,#97517,#97518,
#97519,#97520,#97521,#97522,#97523,#97524,#97525,#97526,#97527,#97528,#97529,
#97530,#97531,#97532,#97533,#97534,#97535,#97536,#97537,#97538,#97539,#97540,
#97541,#97542,#97543,#97544),.UNSPECIFIED.,.F.,.F.,(4,2,2,2,2,2,2,2,2,2,
2,2,2,2,2,2,2,2,2,2,2,2,2,2,2,2,2,2,2,2,2,2,2,2,2,2,2,2,2,2,2,2,2,2,2,2,
2,2,2,2,2,2,2,2,2,2,2,2,2,2,2,2,2,2,2,2,2,2,2,2,2,2,2,2,2,2,2,2,2,2,2,2,
2,2,2,2,2,2,2,2,2,2,2,2,2,2,2,2,2,2,2,2,2,2,2,2,2,2,4),(-2.94874919963959,
-2.94563181336272,-2.94438616932686,-2.94352134164249,-2.9427262295307,
-2.94161336042909,-2.93867664477627,-2.92049594125669,-2.90481990378337,
-2.8951716182036,-2.88884054412347,-2.88653722719753,-2.88496849127357,
-2.8834379379217,-2.88124899019365,-2.8772209945663,-2.85142959079008,-2.82988005621161,
-2.82771003991804,-2.82664845594012,-2.82589006572939,-2.82492580292341,
-2.82326652084327,-2.81668482031881,-2.81005072088468,-2.78015618473745,
-2.77186811969537,-2.76932862961244,-2.76770976621996,-2.76619141500019,
-2.76419313432092,-2.75967478626329,-2.7351571068768,-2.71879195802694,
-2.71395076033784,-2.71071698023472,-2.70947116876784,-2.70860629404098,
-2.70781119420487,-2.70669841572578,-2.70376255310536,-2.68556030021428,
-2.66984655242859,-2.66023340089687,-2.65391892335074,-2.65161784995547,
-2.65004954813491,-2.64851857685317,-2.64632755916661,-2.64229192481368,
-2.61669401127094,-2.60337869593432,-2.59429832090056,-2.59253570780119,
-2.59155854160376,-2.59071771446621,-2.58962926936559,-2.58784855611947,
-2.57574356815116,-2.54663867354052,-2.53719187527053,-2.53453776874591,
-2.53289389135039,-2.53138442810734,-2.5294434367491,-2.52524438228764,
-2.49587639680752,-2.4775309312382,-2.47533358817698,-2.47426661449917,
-2.47342748751495,-2.47243476984707,-2.47065065363171,-2.46228457510869,
-2.43230743330612,-2.42011777321775,-2.41724763451464,-2.41555643801239,
-2.41405735272636,-2.41217049850482,-2.40920283352659,-2.3891901890282,
-2.38724898164711,-2.36747259894213,-2.35926444946408,-2.35754914363084,
-2.35658225927113,-2.35573983681129,-2.35465398220687,-2.35284248740325,
-2.33878654230967,-2.31807641461105,-2.30807480991439,-2.30371001763489,
-2.30025208759365,-2.29843551985566,-2.29708617175595,-2.29539590635686,
-2.29253021073826,-2.28195198318271,-2.2580260494147,-2.24363463152286,
-2.24075042566623,-2.23955979022528,-2.23870495394633,-2.2377807981689,
-2.23625942108317,-2.23127379633466,-2.20677820015193),.UNSPECIFIED.);
#1508=B_SPLINE_CURVE_WITH_KNOTS('',3,(#97549,#97550,#97551,#97552,#97553,
#97554,#97555,#97556,#97557,#97558,#97559,#97560,#97561,#97562,#97563,#97564,
#97565,#97566,#97567,#97568,#97569,#97570,#97571,#97572,#97573,#97574,#97575,
#97576,#97577,#97578,#97579,#97580,#97581,#97582,#97583,#97584,#97585,#97586,
#97587,#97588,#97589,#97590,#97591,#97592,#97593,#97594,#97595,#97596,#97597,
#97598,#97599,#97600,#97601,#97602,#97603,#97604,#97605,#97606,#97607,#97608,
#97609,#97610,#97611,#97612,#97613,#97614,#97615,#97616,#97617,#97618,#97619,
#97620,#97621,#97622,#97623,#97624,#97625,#97626,#97627,#97628,#97629,#97630,
#97631,#97632,#97633,#97634,#97635,#97636,#97637,#97638,#97639,#97640,#97641,
#97642,#97643,#97644,#97645,#97646,#97647,#97648,#97649,#97650,#97651,#97652,
#97653,#97654,#97655,#97656,#97657,#97658,#97659,#97660,#97661,#97662,#97663,
#97664,#97665,#97666,#97667,#97668,#97669,#97670,#97671,#97672,#97673,#97674,
#97675,#97676,#97677,#97678,#97679,#97680,#97681,#97682,#97683,#97684,#97685,
#97686,#97687,#97688,#97689,#97690,#97691,#97692,#97693,#97694,#97695,#97696,
#97697,#97698,#97699,#97700,#97701,#97702,#97703,#97704,#97705,#97706,#97707,
#97708,#97709,#97710,#97711,#97712,#97713,#97714,#97715,#97716,#97717,#97718,
#97719,#97720,#97721,#97722,#97723,#97724,#97725,#97726,#97727,#97728,#97729,
#97730,#97731,#97732,#97733,#97734,#97735,#97736,#97737,#97738,#97739,#97740,
#97741,#97742,#97743,#97744,#97745,#97746,#97747,#97748,#97749,#97750,#97751,
#97752,#97753,#97754,#97755,#97756),.UNSPECIFIED.,.F.,.F.,(4,2,2,2,2,2,
2,2,2,2,2,2,2,2,2,2,2,2,2,2,2,2,2,2,2,2,2,2,2,2,2,2,2,2,2,2,2,2,2,2,2,2,
2,2,2,2,2,2,2,2,2,2,2,2,2,2,2,2,2,2,2,2,2,2,2,2,2,2,2,2,2,2,2,2,2,2,2,2,
2,2,2,2,2,2,2,2,2,2,2,2,2,2,2,2,2,2,2,2,2,2,2,2,2,4),(-1.48411343733603,
-1.48391937310299,-1.46979791345893,-1.44217094315329,-1.43824144942646,
-1.43629458071536,-1.43487784313069,-1.43335459476186,-1.43129367620594,
-1.42654436271121,-1.41998565202743,-1.40083602324541,-1.38081805978295,
-1.37789894277997,-1.37678800916947,-1.37599321408102,-1.37512748052567,
-1.37387844619672,-1.37062513018299,-1.36574562215395,-1.34914406759509,
-1.32496541931158,-1.32043920508221,-1.31843910199311,-1.31691999566555,
-1.31530092751719,-1.31276236584729,-1.30448891516698,-1.27455384889865,
-1.26790837164263,-1.26133363315694,-1.25967449115301,-1.25871003186337,
-1.25795129722163,-1.25688897645381,-1.25471649648369,-1.23728677584488,
-1.20677233317044,-1.2027113325222,-1.20077478610655,-1.19926975686926,
-1.19760626616624,-1.19486451918617,-1.18441684133425,-1.16425711219195,
-1.14589196910587,-1.14295934986015,-1.14184666105141,-1.14105138342591,
-1.14018601556656,-1.13893898082861,-1.13569908990507,-1.13084670990019,
-1.11441402372758,-1.09001130270313,-1.08549026710628,-1.08349103051009,
-1.08197202765248,-1.08035253635164,-1.0778121911182,-1.06952248093534,
-1.03959841782298,-1.03295128618048,-1.0263840613134,-1.02472551151036,
-1.02376116882008,-1.02300238378214,-1.02193980789052,-1.01976614330796,
-1.00229692844627,-0.97183222092432,-0.96776461244867,-0.965826771272516,
-0.96432153981366,-0.96265864095223,-0.959919759536341,-0.94950779657122,
-0.929473205906618,-0.910938302271087,-0.908006730024431,-0.906894149096673,
-0.906098882946798,-0.905233451947954,-0.903986201350591,-0.900745053860764,
-0.895890200008261,-0.879442688064493,-0.855057989796824,-0.850536316746511,
-0.848536926975115,-0.847017857948266,-0.845398344398416,-0.842858065702801,
-0.834569519654809,-0.804643340629272,-0.797996110643673,-0.791427957786785,
-0.789769292113311,-0.788804902743149,-0.788046093894874,-0.786983501437117,
-0.784809863235326,-0.767343590916143,-0.742062510194801),.UNSPECIFIED.);
#1509=B_SPLINE_CURVE_WITH_KNOTS('',3,(#97757,#97758,#97759,#97760,#97761,
#97762,#97763,#97764,#97765,#97766,#97767,#97768,#97769,#97770,#97771,#97772,
#97773,#97774,#97775,#97776,#97777,#97778,#97779,#97780,#97781,#97782,#97783,
#97784,#97785,#97786,#97787,#97788,#97789,#97790,#97791,#97792,#97793,#97794,
#97795,#97796,#97797,#97798,#97799,#97800,#97801,#97802,#97803,#97804,#97805,
#97806,#97807,#97808,#97809,#97810,#97811,#97812,#97813,#97814,#97815,#97816,
#97817,#97818,#97819,#97820,#97821,#97822,#97823,#97824,#97825,#97826,#97827,
#97828,#97829,#97830,#97831,#97832,#97833,#97834,#97835,#97836,#97837,#97838,
#97839,#97840,#97841,#97842,#97843,#97844,#97845,#97846,#97847,#97848,#97849,
#97850,#97851,#97852,#97853,#97854,#97855,#97856,#97857,#97858,#97859,#97860,
#97861,#97862,#97863,#97864,#97865,#97866,#97867,#97868,#97869,#97870,#97871,
#97872,#97873,#97874,#97875,#97876,#97877,#97878,#97879,#97880,#97881,#97882,
#97883,#97884,#97885,#97886,#97887,#97888,#97889,#97890,#97891,#97892,#97893,
#97894,#97895,#97896,#97897,#97898,#97899,#97900,#97901,#97902,#97903,#97904,
#97905,#97906,#97907,#97908,#97909,#97910,#97911,#97912,#97913,#97914,#97915,
#97916,#97917,#97918,#97919,#97920,#97921,#97922,#97923,#97924,#97925,#97926,
#97927,#97928,#97929,#97930,#97931,#97932,#97933,#97934,#97935,#97936,#97937,
#97938,#97939,#97940,#97941,#97942,#97943,#97944,#97945,#97946,#97947,#97948,
#97949,#97950,#97951,#97952,#97953,#97954,#97955,#97956,#97957,#97958,#97959,
#97960,#97961,#97962,#97963,#97964,#97965,#97966,#97967,#97968),
 .UNSPECIFIED.,.F.,.F.,(4,2,2,2,2,2,2,2,2,2,2,2,2,2,2,2,2,2,2,2,2,2,2,2,
2,2,2,2,2,2,2,2,2,2,2,2,2,2,2,2,2,2,2,2,2,2,2,2,2,2,2,2,2,2,2,2,2,2,2,2,
2,2,2,2,2,2,2,2,2,2,2,2,2,2,2,2,2,2,2,2,2,2,2,2,2,2,2,2,2,2,2,2,2,2,2,2,
2,2,2,2,2,2,2,2,2,4),(-2.20677820015193,-2.19782960546998,-2.18524257551801,
-2.18234651604768,-2.18064970785602,-2.17915151037252,-2.1772735701919,
-2.17433523092769,-2.15626959839353,-2.13299626968107,-2.12437999180744,
-2.12264176548573,-2.12166990949715,-2.12082834350583,-2.11975014283919,
-2.11796483893494,-2.10571925429444,-2.07644693946391,-2.06726843738073,
-2.06463952170548,-2.06300120198874,-2.06149009575149,-2.05953753985984,
-2.05527495910282,-2.02651360467143,-2.0076813778414,-2.00547137576711,
-2.00440195344056,-2.00356269726017,-2.00257193829803,-2.0007963755545,
-1.99256516272289,-1.96245945135483,-1.95025275853269,-1.94738158187449,
-1.94569021112711,-1.94419123868638,-1.94230488414745,-1.93933871169091,
-1.91671034502803,-1.9003870691124,-1.8896125997876,-1.88777499095322,-1.88678176369205,
-1.88594276825481,-1.88487668670315,-1.88317070003192,-1.87323412624796,
-1.84907194678992,-1.83852824763725,-1.83400544482355,-1.83044903042786,
-1.82861233948987,-1.82711724836727,-1.82539107742984,-1.82243883097819,
-1.81019451494527,-1.78444278643403,-1.77328369346748,-1.7707372182407,
-1.76960473894355,-1.76875888820371,-1.7678081649945,-1.76616655703857,
-1.7600062831576,-1.73329216150789,-1.71601076727462,-1.71309609345232,
-1.71122532129363,-1.70972775310294,-1.70802618401248,-1.70510829538191,
-1.69217465206501,-1.67521802115282,-1.65647819344893,-1.65354327201266,
-1.6524306079394,-1.65163555335253,-1.65077067747817,-1.64952478748937,
-1.64629032950031,-1.64144830223028,-1.62507606895734,-1.60059514261638,
-1.59607710796654,-1.59407891202565,-1.59256059790068,-1.59094174862975,
-1.58840223023976,-1.58011384269552,-1.55020267036847,-1.54355837122753,
-1.53697920676373,-1.53532011047188,-1.5343558939778,-1.5335974929654,-1.53253584664277,
-1.53036550857978,-1.51299046027206,-1.48240563647643,-1.47835443034983,
-1.47642020637837,-1.47491597105228,-1.47325233670926,-1.47050799711252,
-1.46482421780974),.UNSPECIFIED.);
#1510=B_SPLINE_CURVE_WITH_KNOTS('',3,(#97973,#97974,#97975,#97976,#97977,
#97978,#97979,#97980,#97981,#97982,#97983,#97984,#97985,#97986,#97987,#97988,
#97989,#97990,#97991,#97992,#97993,#97994,#97995,#97996,#97997,#97998,#97999,
#98000,#98001,#98002,#98003,#98004,#98005,#98006,#98007,#98008,#98009,#98010,
#98011,#98012,#98013,#98014,#98015,#98016,#98017,#98018,#98019,#98020,#98021,
#98022,#98023,#98024,#98025,#98026,#98027,#98028,#98029,#98030,#98031,#98032,
#98033,#98034,#98035,#98036,#98037,#98038,#98039,#98040,#98041,#98042,#98043,
#98044,#98045,#98046,#98047,#98048,#98049,#98050,#98051,#98052,#98053,#98054,
#98055,#98056,#98057,#98058,#98059,#98060,#98061,#98062,#98063,#98064,#98065,
#98066,#98067,#98068,#98069,#98070,#98071,#98072,#98073,#98074,#98075,#98076,
#98077,#98078,#98079,#98080,#98081,#98082,#98083,#98084,#98085,#98086,#98087,
#98088,#98089,#98090,#98091,#98092,#98093,#98094,#98095,#98096,#98097,#98098,
#98099,#98100,#98101,#98102,#98103,#98104,#98105,#98106,#98107,#98108,#98109,
#98110,#98111,#98112,#98113,#98114,#98115,#98116,#98117,#98118,#98119,#98120,
#98121,#98122,#98123,#98124,#98125,#98126,#98127,#98128,#98129,#98130,#98131,
#98132,#98133,#98134,#98135,#98136,#98137,#98138,#98139,#98140,#98141,#98142,
#98143,#98144,#98145,#98146,#98147,#98148,#98149,#98150,#98151,#98152,#98153,
#98154,#98155,#98156,#98157,#98158,#98159,#98160,#98161,#98162,#98163,#98164,
#98165,#98166,#98167,#98168,#98169,#98170,#98171,#98172,#98173,#98174,#98175,
#98176,#98177,#98178,#98179,#98180,#98181,#98182,#98183,#98184,#98185,#98186,
#98187,#98188),.UNSPECIFIED.,.F.,.F.,(4,2,2,2,2,2,2,2,2,2,2,2,2,2,2,2,2,
2,2,2,2,2,2,2,2,2,2,2,2,2,2,2,2,2,2,2,2,2,2,2,2,2,2,2,2,2,2,2,2,2,2,2,2,
2,2,2,2,2,2,2,2,2,2,2,2,2,2,2,2,2,2,2,2,2,2,2,2,2,2,2,2,2,2,2,2,2,2,2,2,
2,2,2,2,2,2,2,2,2,2,2,2,2,2,2,2,2,2,4),(-2.22607311897124,-2.21929097350467,
-2.20184663678831,-2.1996738642096,-2.19861157330789,-2.19785293534124,
-2.19688868835388,-2.19523012968417,-2.18866018895975,-2.18202465914146,
-2.1521203992696,-2.14383516185461,-2.14129557415982,-2.13967641268918,
-2.13815761061215,-2.13615847872499,-2.13163701355976,-2.10723555996063,
-2.09078731868563,-2.08593247508836,-2.08269177223932,-2.08144472237794,
-2.08057944611062,-2.07978433102873,-2.07867198334757,-2.07574099727257,
-2.05735400750317,-2.03723455461772,-2.02679885505298,-2.02405837689652,
-2.02239530050497,-2.02089041594831,-2.01895373356547,-2.01489125575152,
-1.98437637370039,-1.96693249704206,-1.96475969277226,-1.96369737864859,
-1.96293872095436,-1.96197444458483,-1.96031582603649,-1.95374552485027,
-1.94710985140665,-1.91720450455584,-1.90891942598523,-1.90637981070113,
-1.90476061464001,-1.90324176820599,-1.90124256055587,-1.89672084748269,
-1.87232371251244,-1.85587126976998,-1.85101568780574,-1.84777459627112,
-1.84652746740652,-1.84566215915344,-1.84486703298962,-1.84375469399392,
-1.84082393163144,-1.82239978557885,-1.80230702524183,-1.79187884229759,
-1.78913892990292,-1.78747594903847,-1.78597099157341,-1.78403399194874,
-1.77997000837532,-1.74946525645529,-1.73201252422919,-1.72983942216229,
-1.72877703233859,-1.72801834901254,-1.72705407902309,-1.72539555590722,
-1.71882674723765,-1.71219058801633,-1.68228702651055,-1.6739982848203,
-1.67145823626562,-1.66983891760047,-1.66832006378673,-1.66632100343427,
-1.66180031506509,-1.63735816753994,-1.62093881526335,-1.616088531535,-1.61285004753217,
-1.61160329242204,-1.61073803966324,-1.60994280098531,-1.60883008851428,
-1.60589654520782,-1.58711761841533,-1.5672924211645,-1.55694138896825,
-1.55420778264581,-1.55254615509739,-1.5510408280934,-1.5491011136097,-1.54502298822946,
-1.51462822507784,-1.49708992145263,-1.49491433881309,-1.49385144290656,
-1.49309268530451,-1.4921287142232,-1.49047155714957,-1.48411343733603),
 .UNSPECIFIED.);
#1511=B_SPLINE_CURVE_WITH_KNOTS('',3,(#98189,#98190,#98191,#98192,#98193,
#98194,#98195,#98196,#98197,#98198,#98199,#98200,#98201,#98202,#98203,#98204,
#98205,#98206,#98207,#98208,#98209,#98210,#98211,#98212,#98213,#98214,#98215,
#98216,#98217,#98218,#98219,#98220,#98221,#98222,#98223,#98224,#98225,#98226,
#98227,#98228,#98229,#98230,#98231,#98232,#98233,#98234,#98235,#98236,#98237,
#98238,#98239,#98240,#98241,#98242,#98243,#98244,#98245,#98246,#98247,#98248,
#98249,#98250,#98251,#98252,#98253,#98254,#98255,#98256,#98257,#98258,#98259,
#98260,#98261,#98262,#98263,#98264,#98265,#98266,#98267,#98268,#98269,#98270,
#98271,#98272,#98273,#98274,#98275,#98276,#98277,#98278,#98279,#98280,#98281,
#98282,#98283,#98284,#98285,#98286,#98287,#98288,#98289,#98290,#98291,#98292,
#98293,#98294,#98295,#98296,#98297,#98298,#98299,#98300,#98301,#98302,#98303,
#98304,#98305,#98306,#98307,#98308,#98309,#98310,#98311,#98312,#98313,#98314,
#98315,#98316,#98317,#98318,#98319,#98320,#98321,#98322,#98323,#98324,#98325,
#98326,#98327,#98328,#98329,#98330,#98331,#98332,#98333,#98334,#98335,#98336,
#98337,#98338,#98339,#98340,#98341,#98342,#98343,#98344,#98345,#98346,#98347,
#98348,#98349,#98350,#98351,#98352,#98353,#98354,#98355,#98356,#98357,#98358,
#98359,#98360,#98361,#98362,#98363,#98364,#98365,#98366,#98367,#98368,#98369,
#98370,#98371,#98372,#98373,#98374,#98375,#98376,#98377,#98378,#98379,#98380,
#98381,#98382,#98383,#98384,#98385,#98386,#98387,#98388,#98389,#98390,#98391,
#98392,#98393,#98394),.UNSPECIFIED.,.F.,.F.,(4,2,2,2,2,2,2,2,2,2,2,2,2,
2,2,2,2,2,2,2,2,2,2,2,2,2,2,2,2,2,2,2,2,2,2,2,2,2,2,2,2,2,2,2,2,2,2,2,2,
2,2,2,2,2,2,2,2,2,2,2,2,2,2,2,2,2,2,2,2,2,2,2,2,2,2,2,2,2,2,2,2,2,2,2,2,
2,2,2,2,2,2,2,2,2,2,2,2,2,2,2,2,2,4),(-1.46482421780974,-1.46001994932202,
-1.43971559363077,-1.42155231735944,-1.41861317870521,-1.41749995646963,
-1.41670473759329,-1.41583995287812,-1.41459463946323,-1.41136415181476,
-1.40653016733953,-1.39020783042935,-1.36565915175576,-1.36114281590523,
-1.35914487918438,-1.35762656992739,-1.35600754100542,-1.3534673524203,
-1.3451731481688,-1.31526518534176,-1.30862017719824,-1.30204349333684,
-1.30038456908071,-1.29942037352597,-1.29866193967416,-1.2976001833691,
-1.2954293908031,-1.27804037321172,-1.24747212951246,-1.2434185308706,-1.24148381441753,
-1.2399794783136,-1.23831601924344,-1.23557263500235,-1.22509705304821,
-1.20483720260103,-1.18660948706426,-1.18367317733575,-1.18256028950037,
-1.18176514331254,-1.18090024639802,-1.17965445581982,-1.17642097704914,
-1.1715810280829,-1.15522245515856,-1.13072042524661,-1.12620262984951,
-1.12420439819367,-1.12268600169625,-1.12106701145758,-1.11852716029011,
-1.11023664378171,-1.08032474361402,-1.07367987417458,-1.06710105922155,
-1.0654419207791,-1.0644776570861,-1.06371920478855,-1.06265746829177,-1.06048687993743,
-1.04310686284157,-1.01252511141035,-1.0084729942557,-1.00653852202217,
-1.00503417473672,-1.00337049899509,-1.00062628266808,-0.990141242459935,
-0.969848582487102,-0.951665671743487,-0.948727246683078,-0.947614067007472,
-0.946818827236084,-0.945953960780812,-0.944708432285455,-0.941476846000052,
-0.936640758685802,-0.920306364980012,-0.895770732472425,-0.891253696576016,
-0.889255559335028,-0.887737140308702,-0.886118035340222,-0.883577813600781,
-0.875284306475449,-0.845373490488388,-0.83872816404903,-0.832150458556475,
-0.830491377321681,-0.82952710808295,-0.828768627223265,-0.827706819327287,
-0.825535972292219,-0.808148813821095,-0.777574698039789,-0.773521340243112,
-0.77158659457866,-0.770082173149268,-0.768418556118181,-0.765674763579876,
-0.755195668359902,-0.734924512360489,-0.722776382337732),.UNSPECIFIED.);
#1512=B_SPLINE_CURVE_WITH_KNOTS('',3,(#98399,#98400,#98401,#98402,#98403,
#98404,#98405,#98406,#98407,#98408,#98409,#98410,#98411,#98412,#98413,#98414,
#98415,#98416,#98417,#98418,#98419,#98420,#98421,#98422,#98423,#98424,#98425,
#98426,#98427,#98428,#98429,#98430,#98431,#98432,#98433,#98434,#98435,#98436,
#98437,#98438,#98439,#98440,#98441,#98442,#98443,#98444,#98445,#98446,#98447,
#98448,#98449,#98450,#98451,#98452,#98453,#98454,#98455,#98456,#98457,#98458,
#98459,#98460,#98461,#98462,#98463,#98464,#98465,#98466,#98467,#98468,#98469,
#98470,#98471,#98472,#98473,#98474,#98475,#98476,#98477,#98478,#98479,#98480,
#98481,#98482,#98483,#98484,#98485,#98486,#98487,#98488,#98489,#98490,#98491,
#98492,#98493,#98494,#98495,#98496,#98497,#98498,#98499,#98500,#98501,#98502,
#98503,#98504,#98505,#98506,#98507,#98508,#98509,#98510,#98511,#98512,#98513,
#98514,#98515,#98516,#98517,#98518,#98519,#98520,#98521,#98522,#98523,#98524,
#98525,#98526,#98527,#98528,#98529,#98530,#98531,#98532,#98533,#98534,#98535,
#98536,#98537,#98538,#98539,#98540,#98541,#98542,#98543,#98544,#98545,#98546,
#98547,#98548,#98549,#98550,#98551,#98552,#98553,#98554,#98555,#98556,#98557,
#98558,#98559,#98560,#98561,#98562,#98563,#98564,#98565,#98566,#98567,#98568,
#98569,#98570,#98571,#98572,#98573,#98574,#98575,#98576,#98577,#98578,#98579,
#98580,#98581,#98582,#98583,#98584,#98585,#98586,#98587,#98588,#98589,#98590,
#98591,#98592,#98593,#98594,#98595,#98596,#98597,#98598,#98599,#98600,#98601,
#98602,#98603,#98604,#98605,#98606,#98607,#98608,#98609,#98610,#98611,#98612,
#98613,#98614,#98615,#98616,#98617,#98618),.UNSPECIFIED.,.F.,.F.,(4,2,2,
2,2,2,2,2,2,2,2,2,2,2,2,2,2,2,2,2,2,2,2,2,2,2,2,2,2,2,2,2,2,2,2,2,2,2,2,
2,2,2,2,2,2,2,2,2,2,2,2,2,2,2,2,2,2,2,2,2,2,2,2,2,2,2,2,2,2,2,2,2,2,2,2,
2,2,2,2,2,2,2,2,2,2,2,2,2,2,2,2,2,2,2,2,2,2,2,2,2,2,2,2,2,2,2,2,2,2,4),
(-2.96795039865844,-2.96582312178668,-2.96411238401058,-2.96264615200535,
-2.96120232953042,-2.95976648285695,-2.95733638411068,-2.95061343729543,
-2.91678081521481,-2.90596739345903,-2.90412810799626,-2.90313443010285,
-2.90229532205603,-2.90122941424266,-2.899524286847,-2.88961158757631,-2.88031750535324,
-2.86580509013092,-2.85503624381333,-2.85044878485478,-2.84790946403175,
-2.84568861099755,-2.84415331235272,-2.84262041423798,-2.8407665656986,
-2.83632531186626,-2.81194750279753,-2.79550013957811,-2.79064561722568,
-2.78740514170684,-2.78615818805693,-2.78529298137241,-2.78449793249726,
-2.78338568043151,-2.78045497116021,-2.7620659038308,-2.74195074538013,
-2.73151665661648,-2.7287764644494,-2.72711353751422,-2.72560877270466,
-2.72367222270958,-2.71960994093126,-2.68909861461352,-2.67165534807906,
-2.66948269800173,-2.66842046605485,-2.66766186980976,-2.66669767532902,
-2.66503920584079,-2.65846960343412,-2.6518344420474,-2.62193178925201,
-2.61364705288247,-2.61110760951643,-2.60948853800343,-2.60796981886377,
-2.60597079403584,-2.60144956172376,-2.57705004995336,-2.56060225625885,
-2.55574760552114,-2.55250704402705,-2.55126005710661,-2.55039482727659,
-2.5495997570843,-2.54848747513251,-2.5455566865813,-2.52716720531476,-2.50705145006173,
-2.49661706525348,-2.49387679834531,-2.49221382658099,-2.49070902154583,
-2.4887724202592,-2.48471003267899,-2.45419786599084,-2.43675415023053,
-2.43458144248419,-2.43351918219339,-2.43276056564562,-2.43179634527647,
-2.43013783107876,-2.4235680491917,-2.41693271078169,-2.38702925172266,
-2.37874430083671,-2.37620479024701,-2.37458567554674,-2.37306691566721,
-2.37106783688021,-2.36654648105286,-2.34214641160455,-2.32569810507832,
-2.32084331263122,-2.31760265854901,-2.31635563735819,-2.31549038418914,
-2.3146952929029,-2.31358298190684,-2.31065212069231,-2.29226157465932,
-2.27214570480497,-2.26171116191006,-2.25897083156582,-2.25730781744919,
-2.25580297161136,-2.25386631433926,-2.24980379625315,-2.22607311897124),
 .UNSPECIFIED.);
#1513=B_SPLINE_CURVE_WITH_KNOTS('',3,(#98619,#98620,#98621,#98622,#98623,
#98624,#98625,#98626,#98627,#98628,#98629,#98630,#98631,#98632,#98633,#98634,
#98635,#98636,#98637,#98638,#98639,#98640,#98641,#98642,#98643,#98644,#98645,
#98646,#98647,#98648,#98649,#98650,#98651,#98652,#98653,#98654,#98655,#98656,
#98657,#98658,#98659,#98660,#98661,#98662,#98663,#98664,#98665,#98666,#98667,
#98668,#98669,#98670,#98671,#98672,#98673,#98674,#98675,#98676,#98677,#98678,
#98679,#98680,#98681,#98682,#98683,#98684,#98685,#98686,#98687,#98688,#98689,
#98690,#98691,#98692,#98693,#98694,#98695,#98696,#98697,#98698,#98699,#98700,
#98701,#98702,#98703,#98704,#98705,#98706,#98707,#98708,#98709,#98710,#98711,
#98712,#98713,#98714,#98715,#98716,#98717,#98718,#98719,#98720,#98721,#98722,
#98723,#98724,#98725,#98726,#98727,#98728,#98729,#98730,#98731,#98732,#98733,
#98734,#98735,#98736,#98737,#98738,#98739,#98740,#98741,#98742,#98743,#98744,
#98745,#98746,#98747,#98748,#98749,#98750,#98751,#98752,#98753,#98754,#98755,
#98756,#98757,#98758,#98759,#98760,#98761,#98762,#98763,#98764,#98765,#98766,
#98767,#98768,#98769,#98770,#98771,#98772,#98773,#98774,#98775,#98776,#98777,
#98778,#98779,#98780,#98781,#98782,#98783,#98784,#98785,#98786,#98787,#98788,
#98789,#98790,#98791,#98792,#98793,#98794,#98795,#98796,#98797,#98798,#98799,
#98800,#98801,#98802,#98803,#98804,#98805,#98806,#98807,#98808,#98809,#98810,
#98811,#98812,#98813,#98814,#98815,#98816,#98817,#98818,#98819,#98820,#98821,
#98822,#98823,#98824,#98825,#98826,#98827,#98828,#98829,#98830,#98831,#98832,
#98833,#98834,#98835,#98836,#98837,#98838,#98839,#98840,#98841,#98842),
 .UNSPECIFIED.,.F.,.F.,(4,2,2,2,2,2,2,2,2,2,2,2,2,2,2,2,2,2,2,2,2,2,2,2,
2,2,2,2,2,2,2,2,2,2,2,2,2,2,2,2,2,2,2,2,2,2,2,2,2,2,2,2,2,2,2,2,2,2,2,2,
2,2,2,2,2,2,2,2,2,2,2,2,2,2,2,2,2,2,2,2,2,2,2,2,2,2,2,2,2,2,2,2,2,2,2,2,
2,2,2,2,2,2,2,2,2,2,2,2,2,2,2,4),(-0.722776382337732,-0.71670969380575,
-0.713772601598928,-0.712659566861819,-0.711864349472997,-0.710999413964259,
-0.709753631907668,-0.706520531551523,-0.701681451522177,-0.685329089473591,
-0.660815835596637,-0.65629801331289,-0.654299699248656,-0.652781212609362,
-0.651162099776851,-0.648622000653125,-0.640330154988522,-0.610416925061539,
-0.603771556543183,-0.59719270324614,-0.595533490176064,-0.594569171791328,
-0.593810669414327,-0.592748853646526,-0.590578070347913,-0.573195013440525,
-0.542613806318726,-0.538561104060447,-0.536626445552064,-0.535121993832293,
-0.533458243669305,-0.530714000034983,-0.520230118854494,-0.499942624720985,
-0.481749372222675,-0.478811190096316,-0.477697993422082,-0.476902716937715,
-0.476037782284897,-0.474792108930055,-0.471559887721116,-0.466722630334772,
-0.450381907936951,-0.425851704769859,-0.42133418297843,-0.419335882791448,
-0.417817360234243,-0.416198164397421,-0.41365784112425,-0.405364385979259,
-0.37545120158245,-0.368805499226406,-0.362227085257113,-0.360567873271435,
-0.359603536395724,-0.358845007546557,-0.357783139236549,-0.355612192965832,
-0.33822533204436,-0.307647388778757,-0.303594008818171,-0.301659183930078,
-0.300154671082593,-0.298490922667605,-0.295746843055298,-0.28526572048483,
-0.264988492305487,-0.246779220897407,-0.243841645118142,-0.242728501367635,
-0.241933222833659,-0.241068240084413,-0.23982242177642,-0.236589403977412,
-0.231750597476462,-0.215400782040919,-0.190881167420983,-0.18636318553894,
-0.184364765777982,-0.182846185120308,-0.181226958856382,-0.178686654082288,
-0.170393878298478,-0.140479018320842,-0.133833186267082,-0.127254101028983,
-0.125594797115679,-0.12463042029666,-0.123871868440924,-0.122809978843987,
-0.120794313396195,-0.118085898298531,-0.11157921046003,-0.0847788066827937,
-0.0710930379762348,-0.0680476788053426,-0.0663000920922622,-0.0648201876150918,
-0.0630151221594017,-0.059840848056003,-0.0424085710450419,-0.0284568101529183,
-0.0241031573718179,-0.0103445925008922,-0.00853705100009869,-0.00745225982743724,
-0.00660984167598957,-0.00564199331628065,-0.00461671524486754,-0.0030282692782334,
0.,0.0193343403549321),.UNSPECIFIED.);
#1514=B_SPLINE_CURVE_WITH_KNOTS('',3,(#98847,#98848,#98849,#98850,#98851,
#98852,#98853,#98854,#98855,#98856,#98857,#98858,#98859,#98860,#98861,#98862,
#98863,#98864,#98865,#98866,#98867,#98868,#98869,#98870,#98871,#98872,#98873,
#98874,#98875,#98876,#98877,#98878,#98879,#98880,#98881,#98882,#98883,#98884,
#98885,#98886,#98887,#98888,#98889,#98890,#98891,#98892,#98893,#98894,#98895,
#98896,#98897,#98898,#98899,#98900,#98901,#98902,#98903,#98904,#98905,#98906,
#98907,#98908,#98909,#98910,#98911,#98912,#98913,#98914,#98915,#98916,#98917,
#98918,#98919,#98920,#98921,#98922,#98923,#98924,#98925,#98926,#98927,#98928,
#98929,#98930,#98931,#98932,#98933,#98934,#98935,#98936,#98937,#98938,#98939,
#98940,#98941,#98942,#98943,#98944,#98945,#98946,#98947,#98948,#98949,#98950,
#98951,#98952,#98953,#98954,#98955,#98956,#98957,#98958,#98959,#98960,#98961,
#98962,#98963,#98964,#98965,#98966,#98967,#98968,#98969,#98970,#98971,#98972,
#98973,#98974,#98975,#98976,#98977,#98978,#98979,#98980,#98981,#98982,#98983,
#98984,#98985,#98986,#98987,#98988,#98989,#98990,#98991,#98992,#98993,#98994,
#98995,#98996,#98997,#98998,#98999,#99000,#99001,#99002,#99003,#99004,#99005,
#99006,#99007,#99008,#99009,#99010,#99011,#99012,#99013,#99014,#99015,#99016,
#99017,#99018,#99019,#99020,#99021,#99022,#99023,#99024,#99025,#99026,#99027,
#99028,#99029,#99030,#99031,#99032,#99033,#99034,#99035,#99036,#99037,#99038,
#99039,#99040,#99041,#99042,#99043,#99044,#99045,#99046,#99047,#99048,#99049,
#99050,#99051,#99052,#99053,#99054,#99055,#99056,#99057,#99058,#99059,#99060,
#99061,#99062,#99063,#99064,#99065,#99066,#99067,#99068,#99069,#99070,#99071,
#99072,#99073,#99074,#99075,#99076,#99077,#99078,#99079,#99080,#99081,#99082,
#99083,#99084),.UNSPECIFIED.,.F.,.F.,(4,2,2,2,2,2,2,2,2,2,2,2,2,2,2,2,2,
2,2,2,2,2,2,2,2,2,2,2,2,2,2,2,2,2,2,2,2,2,2,2,2,2,2,2,2,2,2,2,2,2,2,2,2,
2,2,2,2,2,2,2,2,2,2,2,2,2,2,2,2,2,2,2,2,2,2,2,2,2,2,2,2,2,2,2,2,2,2,2,2,
2,2,2,2,2,2,2,2,2,2,2,2,2,2,2,2,2,2,2,2,2,2,2,2,2,2,2,2,2,4),(-0.742146480711913,
-0.730686365730827,-0.706301136079038,-0.701779365981078,-0.699779933249417,
-0.698260831564137,-0.69664128317838,-0.6941009498033,-0.685812224992619,
-0.655885402884276,-0.649238029918415,-0.642669736091088,-0.641011034774147,
-0.640046624672213,-0.63928779950678,-0.638225184193244,-0.636051499215259,
-0.618584850007295,-0.588113823977103,-0.584046575082922,-0.582108737104111,
-0.580603435324913,-0.578940384962293,-0.576201082965369,-0.565785281894072,
-0.545738250448365,-0.527217429904185,-0.524285677830778,-0.523173032747767,
-0.522377721668476,-0.521512242846235,-0.520264925092833,-0.517023612934832,
-0.512168520805433,-0.495720292912289,-0.471333966863692,-0.46681204825984,
-0.464812548098975,-0.463293394495491,-0.461673790097061,-0.459133367474245,
-0.450844338492267,-0.420916504703379,-0.414268901932379,-0.407700392410164,
-0.406041635001019,-0.405077192002399,-0.404318340776084,-0.403255688738652,
-0.401081927813235,-0.383614630955482,-0.353142622895265,-0.34907522644454,
-0.347137320465424,-0.345631966861323,-0.34396886025404,-0.341229467956718,
-0.330813354215518,-0.310765790287895,-0.292244127181168,-0.289312274777373,
-0.2881995915571,-0.287404253203741,-0.28653874468529,-0.28529138410809,
-0.282049960521632,-0.277194701361948,-0.260745906248171,-0.236358747608618,
-0.23183667378618,-0.229837105017573,-0.228317899298664,-0.226698239348884,
-0.224157729612459,-0.215868416588593,-0.185939555941578,-0.179291725161071,
-0.172722990169445,-0.171064175846755,-0.170099699761621,-0.169340822504424,
-0.168278134018156,-0.166104298545297,-0.148636403226273,-0.118163502966416,
-0.11417942824114,-0.112232673618163,-0.110758944782324,-0.110533163732709,
-0.1104708700406,-0.110417800358241,-0.110372121652461,-0.110332466450366,
-0.110297790673932,-0.110267281365393,-0.110240294786231,-0.110216313703445,
-0.110194917173601,-0.110175758736259,-0.110158550351455,-0.110123961628251,
-0.110090036369164,-0.110056716115043,-0.110023946513459,-0.109991676869477,
-0.108068324725186,-0.105966805335979,-0.102485666467731,-0.0769792213491306,
-0.0572382317910659,-0.0543144065797727,-0.053202700784251,-0.0524075883548014,
-0.0515417804150689,-0.0502930872286179,-0.0470431689749201,-0.0421708969525724,
-0.0256175127124944,-9.99999999140577E-7),.UNSPECIFIED.);
#1515=B_SPLINE_CURVE_WITH_KNOTS('',3,(#99085,#99086,#99087,#99088,#99089,
#99090,#99091,#99092,#99093,#99094,#99095,#99096,#99097,#99098,#99099,#99100,
#99101,#99102,#99103,#99104,#99105,#99106,#99107,#99108,#99109,#99110,#99111,
#99112,#99113,#99114,#99115,#99116,#99117,#99118,#99119,#99120,#99121,#99122,
#99123,#99124,#99125,#99126,#99127,#99128,#99129,#99130,#99131,#99132,#99133,
#99134,#99135,#99136,#99137,#99138,#99139,#99140,#99141,#99142,#99143,#99144,
#99145,#99146,#99147,#99148,#99149,#99150,#99151,#99152,#99153,#99154,#99155,
#99156,#99157,#99158,#99159,#99160,#99161,#99162,#99163,#99164,#99165,#99166,
#99167,#99168,#99169,#99170,#99171,#99172,#99173,#99174,#99175,#99176,#99177,
#99178,#99179,#99180,#99181,#99182,#99183,#99184,#99185,#99186,#99187,#99188,
#99189,#99190,#99191,#99192,#99193,#99194,#99195,#99196,#99197,#99198,#99199,
#99200,#99201,#99202,#99203,#99204,#99205,#99206,#99207,#99208,#99209,#99210,
#99211,#99212,#99213,#99214,#99215,#99216,#99217,#99218,#99219,#99220,#99221,
#99222,#99223,#99224,#99225,#99226,#99227,#99228,#99229,#99230,#99231,#99232,
#99233,#99234,#99235,#99236,#99237,#99238,#99239,#99240,#99241,#99242,#99243,
#99244,#99245,#99246,#99247,#99248,#99249,#99250,#99251,#99252,#99253,#99254,
#99255,#99256,#99257,#99258,#99259,#99260,#99261,#99262,#99263,#99264,#99265,
#99266,#99267,#99268,#99269,#99270,#99271,#99272,#99273,#99274,#99275,#99276,
#99277,#99278,#99279,#99280,#99281,#99282,#99283,#99284,#99285,#99286,#99287,
#99288,#99289,#99290,#99291,#99292,#99293,#99294,#99295,#99296,#99297,#99298,
#99299,#99300),.UNSPECIFIED.,.F.,.F.,(4,2,2,2,2,2,2,2,2,2,2,2,2,2,2,2,2,
2,2,2,2,2,2,2,2,2,2,2,2,2,2,2,2,2,2,2,2,2,2,2,2,2,2,2,2,2,2,2,2,2,2,2,2,
2,2,2,2,2,2,2,2,2,2,2,2,2,2,2,2,2,2,2,2,2,2,2,2,2,2,2,2,2,2,2,2,2,2,2,2,
2,2,2,2,2,2,2,2,2,2,2,2,2,2,2,2,2,2,4),(-2.9676701370104,-2.94175666738961,
-2.93911264794775,-2.93735604142886,-2.93566511119323,-2.93416660720203,
-2.93228094658283,-2.92931607151012,-2.90954221254287,-2.89532384694272,
-2.88024403955377,-2.87805100644773,-2.87696642087232,-2.87613383411841,
-2.87515776976436,-2.87344594860904,-2.86617758918803,-2.86127925981406,
-2.83190743163019,-2.82242996351109,-2.81982952527453,-2.81816661510919,
-2.81666296236614,-2.81472938693359,-2.81067918087877,-2.78009126943132,
-2.76271514019006,-2.76054530273761,-2.75948399659913,-2.75872588236757,
-2.75776207667931,-2.7561038116788,-2.74952919486424,-2.74289679569286,
-2.71302077081229,-2.70472647192174,-2.70218695668462,-2.70056849673392,
-2.69905081760935,-2.69705384973015,-2.69254035461096,-2.66792153002845,
-2.65164575931562,-2.64681995367273,-2.64359414087782,-2.64234982538102,
-2.64148547827381,-2.64069045329864,-2.63957723660059,-2.63663566807151,
-2.61857598497361,-2.59823043969221,-2.5877324070383,-2.58498800070745,
-2.58332474453713,-2.58182111807604,-2.57988805090804,-2.5758406874834,
-2.54522911815593,-2.5278698895905,-2.52570049068269,-2.52463925327488,
-2.52388112878865,-2.52291722870322,-2.52125862474109,-2.51468032824387,
-2.50804838616223,-2.47816611384685,-2.46987878503141,-2.46733996214793,
-2.46572162242803,-2.4642038312463,-2.4622063880866,-2.45769037600957,-2.43315483291176,
-2.41681549354176,-2.41197926626567,-2.40874824962633,-2.40750312476058,
-2.40663860409561,-2.40584373137623,-2.40473114061371,-2.40179468494817,
-2.38363538680355,-2.3679916574597,-2.35832091319345,-2.35405512121286,
-2.35065967814731,-2.34885648076452,-2.34737742590961,-2.34563004371517,
-2.34258300517303,-2.32884344524328,-2.30416459414037,-2.29255548730127,
-2.29068799029271,-2.28968857269036,-2.2888502841821,-2.28779261726404,
-2.28611404246069,-2.27671606336304,-2.24772936495183,-2.23568382370033,
-2.23282413022014,-2.23113558923967,-2.2296367125002,-2.22774724283736,
-2.22596222870392),.UNSPECIFIED.);
#1516=B_SPLINE_CURVE_WITH_KNOTS('',3,(#99305,#99306,#99307,#99308,#99309,
#99310,#99311,#99312,#99313,#99314,#99315,#99316,#99317,#99318,#99319,#99320,
#99321,#99322,#99323,#99324,#99325,#99326,#99327,#99328,#99329,#99330,#99331,
#99332,#99333,#99334,#99335,#99336,#99337,#99338,#99339,#99340,#99341,#99342,
#99343,#99344,#99345,#99346,#99347,#99348,#99349,#99350,#99351,#99352,#99353,
#99354,#99355,#99356,#99357,#99358,#99359,#99360,#99361,#99362,#99363,#99364,
#99365,#99366,#99367,#99368,#99369,#99370,#99371,#99372,#99373,#99374,#99375,
#99376,#99377,#99378,#99379,#99380,#99381,#99382,#99383,#99384,#99385,#99386,
#99387,#99388,#99389,#99390,#99391,#99392,#99393,#99394,#99395,#99396,#99397,
#99398,#99399,#99400,#99401,#99402,#99403,#99404,#99405,#99406,#99407,#99408,
#99409,#99410,#99411,#99412,#99413,#99414,#99415,#99416,#99417,#99418,#99419,
#99420,#99421,#99422,#99423,#99424,#99425,#99426,#99427,#99428,#99429,#99430,
#99431,#99432,#99433,#99434,#99435,#99436,#99437,#99438,#99439,#99440,#99441,
#99442,#99443,#99444,#99445,#99446,#99447,#99448,#99449,#99450,#99451,#99452,
#99453,#99454,#99455,#99456,#99457,#99458,#99459,#99460,#99461,#99462,#99463,
#99464,#99465,#99466,#99467,#99468,#99469,#99470,#99471,#99472,#99473,#99474,
#99475,#99476,#99477,#99478,#99479,#99480,#99481,#99482,#99483,#99484,#99485,
#99486,#99487,#99488,#99489,#99490,#99491,#99492,#99493,#99494,#99495,#99496,
#99497,#99498,#99499,#99500,#99501,#99502,#99503,#99504,#99505,#99506,#99507,
#99508,#99509,#99510,#99511,#99512,#99513,#99514,#99515,#99516,#99517,#99518,
#99519,#99520),.UNSPECIFIED.,.F.,.F.,(4,2,2,2,2,2,2,2,2,2,2,2,2,2,2,2,2,
2,2,2,2,2,2,2,2,2,2,2,2,2,2,2,2,2,2,2,2,2,2,2,2,2,2,2,2,2,2,2,2,2,2,2,2,
2,2,2,2,2,2,2,2,2,2,2,2,2,2,2,2,2,2,2,2,2,2,2,2,2,2,2,2,2,2,2,2,2,2,2,2,
2,2,2,2,2,2,2,2,2,2,2,2,2,2,2,2,2,2,4),(-1.48420216693846,-1.48081117371075,
-1.4656063909844,-1.46360488387489,-1.4625640121514,-1.46172587250738,-1.46071069853317,
-1.45877011247224,-1.44455498745966,-1.43632198942973,-1.41113250435355,
-1.40663681474194,-1.40464211160295,-1.40312393804102,-1.40150280890822,
-1.39895458212505,-1.39058917641951,-1.3607240811837,-1.35407046888925,
-1.34754095724135,-1.3458856571652,-1.34492210261443,-1.34416324876302,
-1.34309968101823,-1.34092076364548,-1.32326191197243,-1.29304695297833,
-1.28935604326243,-1.28746819059756,-1.28606624721167,-1.28453163077674,
-1.28240556694461,-1.27726605129387,-1.25534986017643,-1.23187639153396,
-1.22910368924323,-1.22801485561443,-1.22722580644576,-1.22635450400148,
-1.22507749517868,-1.22163445716663,-1.20040089788481,-1.17621916959604,
-1.17169290770253,-1.16969276868369,-1.16817362927291,-1.16655452029471,
-1.16401588291926,-1.15574207666808,-1.12580645197037,-1.11916080804386,
-1.11258599987531,-1.11092682671214,-1.10996234694199,-1.10920359471085,
-1.10814124739732,-1.10596870625297,-1.08853818379277,-1.05802357127363,
-1.05396241044446,-1.05202580697739,-1.0505207417855,-1.0488572198512,-1.04611544113931,
-1.03566790215954,-1.01550903437464,-0.997141670835854,-0.994209015949504,
-0.993096305706441,-0.992301010968272,-0.991435622422391,-0.990188554463272,
-0.986948558230927,-0.98209600434782,-0.965662553418826,-0.941259789740869,
-0.936738637592961,-0.934739352991742,-0.933220315039454,-0.931600787648849,
-0.929060388590836,-0.920770528781568,-0.890845751993523,-0.884198472029847,
-0.87763107779755,-0.875972488476971,-0.875008123378191,-0.874249321063157,
-0.873186721438305,-0.871013009961648,-0.853543493258314,-0.823077962683899,
-0.819010277383013,-0.817072394987168,-0.815567129510281,-0.813904191039501,
-0.811165239685877,-0.800752949348432,-0.780717589997058,-0.762182677960775,
-0.759251038299022,-0.758138431894522,-0.757343147558453,-0.756477696797236,
-0.755230417765071,-0.75198919664362,-0.747134232721038,-0.742146480711913),
 .UNSPECIFIED.);
#1517=B_SPLINE_CURVE_WITH_KNOTS('',3,(#99521,#99522,#99523,#99524,#99525,
#99526,#99527,#99528,#99529,#99530,#99531,#99532,#99533,#99534,#99535,#99536,
#99537,#99538,#99539,#99540,#99541,#99542,#99543,#99544,#99545,#99546,#99547,
#99548,#99549,#99550,#99551,#99552,#99553,#99554,#99555,#99556,#99557,#99558,
#99559,#99560,#99561,#99562,#99563,#99564,#99565,#99566,#99567,#99568,#99569,
#99570,#99571,#99572,#99573,#99574,#99575,#99576,#99577,#99578,#99579,#99580,
#99581,#99582,#99583,#99584,#99585,#99586,#99587,#99588,#99589,#99590,#99591,
#99592,#99593,#99594,#99595,#99596,#99597,#99598,#99599,#99600,#99601,#99602,
#99603,#99604,#99605,#99606,#99607,#99608,#99609,#99610,#99611,#99612,#99613,
#99614,#99615,#99616,#99617,#99618,#99619,#99620,#99621,#99622,#99623,#99624,
#99625,#99626,#99627,#99628,#99629,#99630,#99631,#99632,#99633,#99634,#99635,
#99636,#99637,#99638,#99639,#99640,#99641,#99642,#99643,#99644,#99645,#99646,
#99647,#99648,#99649,#99650,#99651,#99652,#99653,#99654,#99655,#99656,#99657,
#99658,#99659,#99660,#99661,#99662,#99663,#99664,#99665,#99666,#99667,#99668,
#99669,#99670,#99671,#99672,#99673,#99674,#99675,#99676,#99677,#99678,#99679,
#99680,#99681,#99682,#99683,#99684,#99685,#99686,#99687,#99688,#99689,#99690,
#99691,#99692,#99693,#99694,#99695,#99696,#99697,#99698,#99699,#99700,#99701,
#99702,#99703,#99704,#99705,#99706,#99707,#99708,#99709,#99710,#99711,#99712,
#99713,#99714,#99715,#99716,#99717,#99718,#99719,#99720,#99721,#99722,#99723,
#99724,#99725,#99726),.UNSPECIFIED.,.F.,.F.,(4,2,2,2,2,2,2,2,2,2,2,2,2,
2,2,2,2,2,2,2,2,2,2,2,2,2,2,2,2,2,2,2,2,2,2,2,2,2,2,2,2,2,2,2,2,2,2,2,2,
2,2,2,2,2,2,2,2,2,2,2,2,2,2,2,2,2,2,2,2,2,2,2,2,2,2,2,2,2,2,2,2,2,2,2,2,
2,2,2,2,2,2,2,2,2,2,2,2,2,2,2,2,2,4),(-2.22596222870392,-2.22476976080297,
-2.20318940350078,-2.18313477087351,-2.17487161453999,-2.17315354888634,
-2.1721862650835,-2.17134425760098,-2.17025990643865,-2.16845292359828,
-2.15466496615236,-2.13375959174518,-2.11920139599229,-2.11581961256073,
-2.11401922318127,-2.11254022155332,-2.11079025655054,-2.10773195555156,
-2.09377458483878,-2.06669502388854,-2.05754061755594,-2.05577465636391,
-2.05479693456033,-2.05395645742597,-2.05286954309243,-2.05109345642804,
-2.03912127154843,-2.0190612341553,-2.00293452490127,-1.99883339538176,
-1.99688995572536,-1.99538484512809,-1.99372659694651,-1.99100580380971,
-1.98190045207522,-1.97546321472832,-1.95167918798749,-1.94398151414005,
-1.94094735507046,-1.93868230994526,-1.93760234797305,-1.93676246146497,
-1.93577985208639,-1.93403966073558,-1.9263604773608,-1.89572667905436,
-1.88345256978119,-1.88057739515835,-1.87888540394194,-1.8773869402259,
-1.87550264055797,-1.87254249054539,-1.85327417467825,-1.83106504551911,
-1.82262575636492,-1.82089760729077,-1.81992808801895,-1.81908639155126,
-1.81800529781344,-1.81620962043365,-1.80366283492563,-1.77397346609612,
-1.7654200274196,-1.76285331455238,-1.76122883542191,-1.75971335741571,
-1.75773062864765,-1.75329852034088,-1.72672859928168,-1.70591066469657,
-1.70374283550844,-1.70268186617172,-1.70192372954294,-1.70095953476934,
-1.69929981736681,-1.69270906636629,-1.68607889498275,-1.65617594406913,
-1.64791292450111,-1.64537657491691,-1.64375870141099,-1.64224056911165,
-1.64024154086236,-1.6357169367613,-1.61151008596343,-1.59491959370344,
-1.59004263984899,-1.58679136311717,-1.58554312917557,-1.58467796615649,
-1.58388371745364,-1.58277360308433,-1.57985691403693,-1.55979584464193,
-1.54070611286403,-1.53416029517888,-1.52941831444084,-1.52735944504096,
-1.52583729136321,-1.52442127220101,-1.52247492705227,-1.51748447566437,
-1.48417870616889),.UNSPECIFIED.);
#1518=B_SPLINE_CURVE_WITH_KNOTS('',3,(#99731,#99732,#99733,#99734,#99735,
#99736,#99737,#99738,#99739,#99740,#99741,#99742,#99743,#99744,#99745,#99746,
#99747,#99748,#99749,#99750,#99751,#99752,#99753,#99754,#99755,#99756,#99757,
#99758,#99759,#99760,#99761,#99762,#99763,#99764,#99765,#99766,#99767,#99768,
#99769,#99770,#99771,#99772,#99773,#99774,#99775,#99776,#99777,#99778,#99779,
#99780,#99781,#99782,#99783,#99784,#99785,#99786,#99787,#99788,#99789,#99790,
#99791,#99792,#99793,#99794,#99795,#99796,#99797,#99798,#99799,#99800,#99801,
#99802,#99803,#99804,#99805,#99806,#99807,#99808,#99809,#99810,#99811,#99812,
#99813,#99814,#99815,#99816,#99817,#99818,#99819,#99820,#99821,#99822,#99823,
#99824,#99825,#99826,#99827,#99828,#99829,#99830,#99831,#99832,#99833,#99834,
#99835,#99836,#99837,#99838,#99839,#99840,#99841,#99842,#99843,#99844,#99845,
#99846,#99847,#99848,#99849,#99850,#99851,#99852,#99853,#99854,#99855,#99856,
#99857,#99858,#99859,#99860,#99861,#99862,#99863,#99864,#99865,#99866,#99867,
#99868,#99869,#99870,#99871,#99872,#99873,#99874,#99875,#99876,#99877,#99878,
#99879,#99880,#99881,#99882,#99883,#99884,#99885,#99886,#99887,#99888,#99889,
#99890,#99891,#99892,#99893,#99894,#99895,#99896,#99897,#99898,#99899,#99900,
#99901,#99902,#99903,#99904,#99905,#99906,#99907,#99908,#99909,#99910,#99911,
#99912,#99913,#99914,#99915,#99916,#99917,#99918,#99919,#99920,#99921,#99922,
#99923,#99924,#99925,#99926,#99927,#99928,#99929,#99930,#99931,#99932,#99933,
#99934,#99935,#99936,#99937,#99938,#99939,#99940,#99941,#99942),
 .UNSPECIFIED.,.F.,.F.,(4,2,2,2,2,2,2,2,2,2,2,2,2,2,2,2,2,2,2,2,2,2,2,2,
2,2,2,2,2,2,2,2,2,2,2,2,2,2,2,2,2,2,2,2,2,2,2,2,2,2,2,2,2,2,2,2,2,2,2,2,
2,2,2,2,2,2,2,2,2,2,2,2,2,2,2,2,2,2,2,2,2,2,2,2,2,2,2,2,2,2,2,2,2,2,2,2,
2,2,2,2,2,2,2,2,2,4),(-2.22616681243302,-2.22604246147792,-2.22453767372853,
-2.22260111388507,-2.21853888542679,-2.18802607251338,-2.17058324476156,
-2.16841057850465,-2.16734833249655,-2.16658972370756,-2.16562550985455,
-2.16396699961134,-2.15739713765143,-2.15076188957102,-2.12085849610008,
-2.11257392064909,-2.11003446589562,-2.10841537359118,-2.10689662546881,
-2.10489754866071,-2.10037613785273,-2.0759801652396,-2.05952909573883,
-2.05467387749143,-2.05143302010607,-2.05018597549344,-2.04932072380644,
-2.04852564810396,-2.04741337769718,-2.04448277941868,-2.02606385120704,
-2.00596938737891,-1.9955410178392,-1.99280121175038,-1.99113832274565,
-1.98963346599106,-1.98769662063731,-1.98363305345516,-1.95312906116816,
-1.93567838150813,-1.93350544611992,-1.93244313006603,-1.93168449628269,
-1.93072028496013,-1.92906185342671,-1.92249328447566,-1.91585758747718,
-1.88595567028374,-1.87766784313493,-1.87512799877584,-1.87350879334234,
-1.87199003386457,-1.86999108035674,-1.86547055734127,-1.84103481852673,
-1.82461287616393,-1.81976231410155,-1.81652374551662,-1.8152770264833,
-1.814411820986,-1.81361664357233,-1.81250404038425,-1.8095709814,-1.79086169529351,
-1.77098631377317,-1.76413109542401,-1.75921852717353,-1.75713003344748,
-1.7556022073965,-1.75419230180041,-1.75227200996737,-1.74845036941389,
-1.71949921476802,-1.70082456986282,-1.69861823578307,-1.69754934406224,
-1.69670989443295,-1.69571816669359,-1.69393908298723,-1.68565535438361,
-1.65560409078445,-1.64340456818339,-1.64053333214333,-1.63884163392006,
-1.63734218593728,-1.63545497775124,-1.63248693931853,-1.60993090572051,
-1.59366313410074,-1.58631735076348,-1.582027395654,-1.58059066880361,-1.57977514760289,
-1.57892338428559,-1.57775215062521,-1.57498474011419,-1.57104927554577,
-1.55954787230436,-1.53206055775014,-1.5251497725076,-1.52268964888888,
-1.52124777940947,-1.5197379733565,-1.51776359585784,-1.51349965249691,
-1.48420216693846),.UNSPECIFIED.);
#1519=B_SPLINE_CURVE_WITH_KNOTS('',3,(#99943,#99944,#99945,#99946,#99947,
#99948,#99949,#99950,#99951,#99952,#99953,#99954,#99955,#99956,#99957,#99958,
#99959,#99960,#99961,#99962,#99963,#99964,#99965,#99966,#99967,#99968,#99969,
#99970,#99971,#99972,#99973,#99974,#99975,#99976,#99977,#99978,#99979,#99980,
#99981,#99982,#99983,#99984,#99985,#99986,#99987,#99988,#99989,#99990,#99991,
#99992,#99993,#99994,#99995,#99996,#99997,#99998,#99999,#100000,#100001,
#100002,#100003,#100004,#100005,#100006,#100007,#100008,#100009,#100010,
#100011,#100012,#100013,#100014,#100015,#100016,#100017,#100018,#100019,
#100020,#100021,#100022,#100023,#100024,#100025,#100026,#100027,#100028,
#100029,#100030,#100031,#100032,#100033,#100034,#100035,#100036,#100037,
#100038,#100039,#100040,#100041,#100042,#100043,#100044,#100045,#100046,
#100047,#100048,#100049,#100050,#100051,#100052,#100053,#100054,#100055,
#100056,#100057,#100058,#100059,#100060,#100061,#100062,#100063,#100064,
#100065,#100066,#100067,#100068,#100069,#100070,#100071,#100072,#100073,
#100074,#100075,#100076,#100077,#100078,#100079,#100080,#100081,#100082,
#100083,#100084,#100085,#100086,#100087,#100088,#100089,#100090,#100091,
#100092,#100093,#100094,#100095,#100096,#100097,#100098,#100099,#100100,
#100101,#100102,#100103,#100104,#100105,#100106,#100107,#100108,#100109,
#100110,#100111,#100112,#100113,#100114,#100115,#100116,#100117,#100118,
#100119,#100120,#100121,#100122,#100123,#100124,#100125,#100126,#100127,
#100128,#100129,#100130,#100131,#100132,#100133,#100134,#100135,#100136,
#100137,#100138,#100139,#100140,#100141,#100142,#100143,#100144,#100145,
#100146,#100147,#100148,#100149,#100150,#100151,#100152,#100153,#100154,
#100155,#100156,#100157,#100158),.UNSPECIFIED.,.F.,.F.,(4,2,2,2,2,2,2,2,
2,2,2,2,2,2,2,2,2,2,2,2,2,2,2,2,2,2,2,2,2,2,2,2,2,2,2,2,2,2,2,2,2,2,2,2,
2,2,2,2,2,2,2,2,2,2,2,2,2,2,2,2,2,2,2,2,2,2,2,2,2,2,2,2,2,2,2,2,2,2,2,2,
2,2,2,2,2,2,2,2,2,2,2,2,2,2,2,2,2,2,2,2,2,2,2,2,2,2,2,4),(-1.48417870616889,
-1.48393864425358,-1.48218042152621,-1.47828722870527,-1.47039019383324,
-1.46863521841759,-1.46764923408789,-1.46680968537757,-1.46573431696964,
-1.46349314672872,-1.46050035275944,-1.45295920686657,-1.43691964324222,
-1.41444181724997,-1.4114850135209,-1.40960160813851,-1.40810308358595,
-1.40641020214032,-1.40353149130104,-1.39120840242425,-1.36021101942625,
-1.35287536391893,-1.3511583709944,-1.35018095479658,-1.34934826346162,
-1.34826491112707,-1.3459827594878,-1.34291950355474,-1.33511230179353,
-1.31066661567715,-1.29666156507403,-1.29360044170085,-1.2918495861168,
-1.29037025048514,-1.28856996568095,-1.28518994678059,-1.26068986106189,
-1.23712084191432,-1.23435220323809,-1.23326430350343,-1.23247570180016,
-1.23160463622985,-1.23032756234818,-1.22688189678002,-1.20560226588492,
-1.1814736562158,-1.17694705254759,-1.17494733752316,-1.1734287539856,-1.17181046799911,
-1.16927361820722,-1.16101056983662,-1.13107979173519,-1.12443765768997,
-1.11784608999374,-1.11618594100828,-1.11522147365623,-1.11446310033037,
-1.11340178474876,-1.11123316954272,-1.0901872640142,-1.06387483590322,
-1.05942866590538,-1.05744305854541,-1.05592672634565,-1.05430264060515,
-1.05173933814198,-1.04322466931433,-1.0134780200184,-1.00090081220348,
-0.999103587016294,-0.998021852613617,-0.997179837181083,-0.996210148631531,
-0.994482184411101,-0.986053134210115,-0.965158653727647,-0.944593332047074,
-0.941621671328921,-0.93973352069584,-0.938234202905426,-0.936543589225841,
-0.933676522086198,-0.921536132578467,-0.891932755995872,-0.883150201351662,
-0.881500942245093,-0.880451909101975,-0.879613650273504,-0.878606096497797,
-0.87670140467154,-0.863910477887846,-0.836205157950646,-0.826223308464406,
-0.823414449814019,-0.821736523109991,-0.820385150800801,-0.818550241131409,
-0.815003470991717,-0.79046657118555,-0.767218981199978,-0.764437960361355,
-0.763347817290045,-0.762558539105024,-0.761687846440725,-0.760413215882158,
-0.756985559074815,-0.742164101532787),.UNSPECIFIED.);
#1520=B_SPLINE_CURVE_WITH_KNOTS('',3,(#100163,#100164,#100165,#100166,#100167,
#100168,#100169,#100170,#100171,#100172,#100173,#100174,#100175,#100176,
#100177,#100178,#100179,#100180,#100181,#100182,#100183,#100184,#100185,
#100186,#100187,#100188,#100189,#100190,#100191,#100192,#100193,#100194,
#100195,#100196,#100197,#100198,#100199,#100200,#100201,#100202,#100203,
#100204,#100205,#100206,#100207,#100208,#100209,#100210,#100211,#100212,
#100213,#100214,#100215,#100216,#100217,#100218,#100219,#100220,#100221,
#100222,#100223,#100224,#100225,#100226,#100227,#100228,#100229,#100230,
#100231,#100232,#100233,#100234,#100235,#100236,#100237,#100238,#100239,
#100240,#100241,#100242,#100243,#100244,#100245,#100246,#100247,#100248,
#100249,#100250,#100251,#100252,#100253,#100254,#100255,#100256,#100257,
#100258,#100259,#100260,#100261,#100262,#100263,#100264,#100265,#100266,
#100267,#100268,#100269,#100270,#100271,#100272,#100273,#100274,#100275,
#100276,#100277,#100278,#100279,#100280,#100281,#100282,#100283,#100284,
#100285,#100286,#100287,#100288,#100289,#100290,#100291,#100292,#100293,
#100294,#100295,#100296,#100297,#100298,#100299,#100300,#100301,#100302,
#100303,#100304,#100305,#100306,#100307,#100308,#100309,#100310,#100311,
#100312,#100313,#100314,#100315,#100316,#100317,#100318,#100319,#100320,
#100321,#100322,#100323,#100324,#100325,#100326,#100327,#100328,#100329,
#100330,#100331,#100332,#100333,#100334,#100335,#100336,#100337,#100338,
#100339,#100340,#100341,#100342,#100343,#100344,#100345,#100346,#100347,
#100348,#100349,#100350,#100351,#100352,#100353,#100354,#100355,#100356,
#100357,#100358,#100359,#100360,#100361,#100362,#100363,#100364,#100365,
#100366,#100367,#100368,#100369,#100370,#100371,#100372),.UNSPECIFIED.,
 .F.,.F.,(4,2,2,2,2,2,2,2,2,2,2,2,2,2,2,2,2,2,2,2,2,2,2,2,2,2,2,2,2,2,2,
2,2,2,2,2,2,2,2,2,2,2,2,2,2,2,2,2,2,2,2,2,2,2,2,2,2,2,2,2,2,2,2,2,2,2,2,
2,2,2,2,2,2,2,2,2,2,2,2,2,2,2,2,2,2,2,2,2,2,2,2,2,2,2,2,2,2,2,2,2,2,2,2,
2,4),(-2.96801447478129,-2.96566606301484,-2.94555217476699,-2.93511874503777,
-2.93237872598084,-2.93071590410633,-2.929211234369,-2.92727480673222,-2.92321278164468,
-2.89270338276873,-2.87526121851301,-2.87308870571027,-2.87202654087673,
-2.87126799255996,-2.87030385899625,-2.86864549428685,-2.86207630690686,
-2.85544156473784,-2.82554080113032,-2.81725658827659,-2.8147173053619,
-2.81309833614395,-2.81157971295625,-2.80958081442194,-2.80505986773348,
-2.78066189864089,-2.76421514327792,-2.75936079912144,-2.75612044229885,
-2.75487353415286,-2.75400835898611,-2.7532133390287,-2.75210112735967,
-2.74917052404422,-2.730782197954,-2.71066771856115,-2.70023399441319,-2.69749390075135,
-2.69583103407927,-2.69432632411209,-2.6923898451321,-2.68832771396066,
-2.65781747701803,-2.64037486183409,-2.63820229131619,-2.63714009813048,
-2.63638152951123,-2.63541737006762,-2.63375896068065,-2.62718959417551,
-2.62055467493251,-2.59065310564982,-2.58236867758816,-2.57982932737951,
-2.57821031496099,-2.57669165104294,-2.57469269859435,-2.57017162863388,
-2.54577309267923,-2.52932583149074,-2.52447134676194,-2.52123089791694,
-2.51998395558743,-2.51911875709964,-2.51832371603074,-2.51721147524773,
-2.51428079871268,-2.49589146325859,-2.47577682827127,-2.46534293431623,
-2.462602776261,-2.46093986702863,-2.45943511631044,-2.45749858174765,-2.45343632217927,
-2.4229254219056,-2.40548222190687,-2.40330958984779,-2.4022473675554,-2.40148877854864,
-2.40052459373867,-2.39886614190593,-2.39229662291705,-2.3856615216754,
-2.35575918801667,-2.34747448976598,-2.34493506642525,-2.34331600953875,
-2.34179730542131,-2.33979830226663,-2.3352771273439,-2.31087730753948,
-2.29443008280833,-2.28957554523006,-2.28633504789604,-2.28508807795948,
-2.28422285742077,-2.28342779376688,-2.28231551832051,-2.27938472497521,
-2.26099858451193,-2.24088067951307,-2.23044572474394,-2.22770542927393,
-2.22616681243302),.UNSPECIFIED.);
#1521=B_SPLINE_CURVE_WITH_KNOTS('',3,(#100373,#100374,#100375,#100376,#100377,
#100378,#100379,#100380,#100381,#100382,#100383,#100384,#100385,#100386,
#100387,#100388,#100389,#100390,#100391,#100392,#100393,#100394,#100395,
#100396,#100397,#100398,#100399,#100400,#100401,#100402,#100403,#100404,
#100405,#100406,#100407,#100408,#100409,#100410,#100411,#100412,#100413,
#100414,#100415,#100416,#100417,#100418,#100419,#100420,#100421,#100422,
#100423,#100424,#100425,#100426,#100427,#100428,#100429,#100430,#100431,
#100432,#100433,#100434,#100435,#100436,#100437,#100438,#100439,#100440,
#100441,#100442,#100443,#100444,#100445,#100446,#100447,#100448,#100449,
#100450,#100451,#100452,#100453,#100454,#100455,#100456,#100457,#100458,
#100459,#100460,#100461,#100462,#100463,#100464,#100465,#100466,#100467,
#100468,#100469,#100470,#100471,#100472,#100473,#100474,#100475,#100476,
#100477,#100478,#100479,#100480,#100481,#100482,#100483,#100484,#100485,
#100486,#100487,#100488,#100489,#100490,#100491,#100492,#100493,#100494,
#100495,#100496,#100497,#100498,#100499,#100500,#100501,#100502,#100503,
#100504,#100505,#100506,#100507,#100508,#100509,#100510,#100511,#100512,
#100513,#100514,#100515,#100516,#100517,#100518,#100519,#100520,#100521,
#100522,#100523,#100524,#100525,#100526,#100527,#100528,#100529,#100530,
#100531,#100532,#100533,#100534,#100535,#100536,#100537,#100538,#100539,
#100540,#100541,#100542,#100543,#100544,#100545,#100546,#100547,#100548,
#100549,#100550,#100551,#100552,#100553,#100554,#100555,#100556,#100557,
#100558,#100559,#100560,#100561,#100562,#100563,#100564,#100565,#100566,
#100567,#100568,#100569,#100570,#100571,#100572,#100573,#100574,#100575,
#100576,#100577,#100578,#100579,#100580,#100581,#100582),.UNSPECIFIED.,
 .F.,.F.,(4,2,2,2,2,2,2,2,2,2,2,2,2,2,2,2,2,2,2,2,2,2,2,2,2,2,2,2,2,2,2,
2,2,2,2,2,2,2,2,2,2,2,2,2,2,2,2,2,2,2,2,2,2,2,2,2,2,2,2,2,2,2,2,2,2,2,2,
2,2,2,2,2,2,2,2,2,2,2,2,2,2,2,2,2,2,2,2,2,2,2,2,2,2,2,2,2,2,2,2,2,2,2,2,
2,4),(-0.742164101532787,-0.735971382998655,-0.711532708451572,-0.7070124647953,
-0.705013628555544,-0.703494959260892,-0.701875857657293,-0.69933620881987,
-0.691049873326518,-0.661129576938896,-0.654484222027339,-0.647901840908411,
-0.646242242945901,-0.645277788803992,-0.644519234492205,-0.643457417216243,
-0.641286886214012,-0.623917327195036,-0.593314120394164,-0.589263609088311,
-0.587329273300069,-0.585824758232584,-0.584160618550969,-0.581414989788193,
-0.57091597675433,-0.550576374908781,-0.532453481139082,-0.529511418512946,
-0.528397670971167,-0.527602207833066,-0.526737308123534,-0.525492077579572,
-0.522263183513004,-0.517432752772695,-0.501135022417639,-0.476543905369007,
-0.472027680492035,-0.470029510502894,-0.468510913727838,-0.466891472113768,
-0.4643504130524,-0.456051281306886,-0.426139443141783,-0.419492756867436,
-0.412916242256106,-0.411257099863112,-0.410292732049222,-0.409534134327624,
-0.408472111783265,-0.40630064270998,-0.38890025524091,-0.358335714082141,
-0.354279965561734,-0.352344596292237,-0.350839914659885,-0.34917623812735,
-0.346432877600162,-0.335962437692785,-0.315724167965985,-0.297456476807057,
-0.294520931592771,-0.293407985434298,-0.292612718982639,-0.291747600778781,
-0.290501342131511,-0.287265818221643,-0.28242210279169,-0.266043159182359,
-0.241558469125866,-0.237039116390008,-0.235040358720029,-0.23352162605094,
-0.231902338489127,-0.229362149280418,-0.221071728653136,-0.191152176746599,
-0.184506077462624,-0.177924993493206,-0.176265432678288,-0.175300949619573,
-0.174542341063625,-0.173480406966033,-0.171309490482136,-0.153930255700701,
-0.123336452654517,-0.119367343876605,-0.117441837365444,-0.11596426221111,
-0.114563975867067,-0.112187479462713,-0.105305352214359,-0.0944571800687469,
-0.0745045971603884,-0.0609820264330281,-0.0591776137768069,-0.0580936989468276,
-0.0572513334793649,-0.0562828133379011,-0.0545606323743867,-0.0462372018743076,
-0.0278881277266695,-0.00534326115204203,-0.00210175747461067,-0.000970090757637366,
-1.00000000580192E-6),.UNSPECIFIED.);
#1522=B_SPLINE_CURVE_WITH_KNOTS('',3,(#100588,#100589,#100590,#100591,#100592,
#100593,#100594,#100595,#100596,#100597,#100598,#100599,#100600,#100601,
#100602,#100603,#100604,#100605,#100606,#100607,#100608,#100609,#100610,
#100611,#100612,#100613,#100614,#100615,#100616,#100617,#100618,#100619,
#100620,#100621,#100622,#100623,#100624,#100625,#100626,#100627,#100628,
#100629,#100630,#100631,#100632,#100633,#100634,#100635,#100636,#100637,
#100638,#100639,#100640,#100641,#100642,#100643,#100644,#100645,#100646,
#100647,#100648,#100649,#100650,#100651,#100652,#100653,#100654,#100655,
#100656,#100657,#100658,#100659,#100660,#100661,#100662,#100663,#100664,
#100665,#100666,#100667,#100668,#100669,#100670,#100671,#100672,#100673,
#100674,#100675,#100676,#100677,#100678,#100679,#100680,#100681,#100682,
#100683,#100684,#100685,#100686,#100687,#100688,#100689,#100690,#100691,
#100692,#100693,#100694,#100695,#100696,#100697,#100698,#100699,#100700,
#100701,#100702,#100703,#100704,#100705,#100706,#100707,#100708,#100709,
#100710,#100711,#100712,#100713,#100714,#100715,#100716,#100717,#100718,
#100719,#100720,#100721,#100722,#100723,#100724,#100725,#100726,#100727,
#100728,#100729,#100730,#100731,#100732,#100733,#100734,#100735,#100736,
#100737,#100738,#100739,#100740,#100741,#100742,#100743,#100744,#100745,
#100746,#100747),.UNSPECIFIED.,.F.,.F.,(4,2,2,2,2,2,2,2,2,2,2,2,2,2,2,2,
2,2,2,2,2,2,2,2,2,2,2,2,2,2,2,2,2,2,2,2,2,2,2,2,2,2,2,2,2,2,2,2,2,2,2,2,
2,2,2,2,2,2,2,2,2,2,2,2,2,2,2,2,2,2,2,2,2,2,2,2,2,2,2,4),(-0.537529498082018,
-0.537417443195381,-0.530769639104979,-0.524200930478091,-0.522542122814459,
-0.521577650601132,-0.520818776390598,-0.519756092171006,-0.517582265426865,
-0.50011444027448,-0.469641508250662,-0.465573988730827,-0.463636024079067,
-0.462130624882595,-0.460467467889012,-0.457727992560687,-0.447311562620452,
-0.427263389015693,-0.408741168195958,-0.405809226986125,-0.40469651006346,
-0.403901147620284,-0.403035612886966,-0.401788214529537,-0.398546692768889,
-0.393691286558525,-0.377241993286614,-0.352854095919316,-0.34833188513093,
-0.346332255798364,-0.344813004064781,-0.343193295057419,-0.340652708371575,
-0.332363144269462,-0.302433377118387,-0.295785344982849,-0.289216411034999,
-0.287557546469063,-0.286593041171085,-0.28583414092853,-0.284771420254957,
-0.282597518939526,-0.2651290945308,-0.234655117241117,-0.230587458182983,
-0.228649427050693,-0.227143976213566,-0.225480762168664,-0.222741192870317,
-0.212324405654129,-0.192275544480842,-0.173752688076481,-0.17082064629093,
-0.169707891198068,-0.168912501471051,-0.168046937046673,-0.16679949589876,
-0.163557862941249,-0.158702290171232,-0.142252432620423,-0.117880397832208,
-0.113440807103225,-0.111586800903833,-0.110053412926676,-0.108547727747675,
-0.106475940296733,-0.104043687813602,-0.0997330197806514,-0.0899153030896199,
-0.0743955965550353,-0.0563009987160674,-0.0533569616062631,-0.0522426885144976,
-0.0514468975801223,-0.0505816833750096,-0.0493360448122893,-0.0461063072858154,
-0.0412746707953448,-0.024972170629327,-9.99999999806711E-7),
 .UNSPECIFIED.);
#1523=B_SPLINE_CURVE_WITH_KNOTS('',3,(#100748,#100749,#100750,#100751,#100752,
#100753,#100754,#100755,#100756,#100757,#100758,#100759,#100760,#100761,
#100762,#100763,#100764,#100765,#100766,#100767,#100768,#100769,#100770,
#100771,#100772,#100773,#100774,#100775,#100776,#100777,#100778,#100779,
#100780,#100781,#100782,#100783,#100784,#100785,#100786,#100787,#100788,
#100789,#100790,#100791,#100792,#100793,#100794,#100795,#100796,#100797,
#100798,#100799,#100800,#100801,#100802,#100803,#100804,#100805,#100806,
#100807,#100808,#100809,#100810,#100811,#100812,#100813,#100814,#100815,
#100816,#100817,#100818,#100819),.UNSPECIFIED.,.F.,.F.,(4,2,2,2,2,2,2,2,
2,2,2,2,2,2,2,2,2,2,2,2,2,2,2,2,2,2,2,2,2,2,2,2,2,2,2,4),(-3.17249563591246,
-3.16985267282884,-3.16781533109578,-3.16633184302089,-3.16490281197556,
-3.163297182562,-3.16081860207664,-3.15373960056998,-3.12036675469528,-3.10955754083093,
-3.10771851416671,-3.10672493238573,-3.10588587908643,-3.10482000713047,
-3.10311487383523,-3.09319993144343,-3.08390891414379,-3.06939590956882,
-3.05862925215487,-3.05404252045242,-3.05150353223612,-3.04928310547904,
-3.0477479089204,-3.04621511743451,-3.04436140389674,-3.03992050257416,
-3.01554427711876,-2.99909803353467,-2.99424384163313,-2.99100358669265,
-2.98975671792045,-2.98889157012816,-2.98809657536929,-2.98698439901021,
-2.98405388921461,-2.96801447478129),.UNSPECIFIED.);
#1524=B_SPLINE_CURVE_WITH_KNOTS('',3,(#100820,#100821,#100822,#100823,#100824,
#100825,#100826,#100827,#100828,#100829,#100830,#100831,#100832,#100833,
#100834,#100835,#100836,#100837,#100838,#100839,#100840,#100841,#100842,
#100843,#100844,#100845,#100846,#100847,#100848,#100849,#100850,#100851,
#100852,#100853,#100854,#100855,#100856,#100857,#100858,#100859,#100860,
#100861,#100862,#100863,#100864,#100865,#100866,#100867,#100868,#100869,
#100870,#100871,#100872,#100873,#100874,#100875,#100876,#100877,#100878,
#100879,#100880,#100881,#100882,#100883,#100884,#100885,#100886,#100887,
#100888,#100889,#100890,#100891,#100892,#100893,#100894,#100895,#100896,
#100897,#100898,#100899,#100900,#100901,#100902,#100903,#100904,#100905,
#100906,#100907,#100908,#100909,#100910,#100911,#100912,#100913,#100914,
#100915,#100916,#100917,#100918,#100919,#100920,#100921,#100922,#100923,
#100924,#100925,#100926,#100927,#100928,#100929,#100930,#100931,#100932,
#100933,#100934,#100935,#100936,#100937,#100938,#100939,#100940,#100941,
#100942,#100943,#100944,#100945,#100946,#100947,#100948,#100949,#100950,
#100951,#100952,#100953,#100954,#100955,#100956,#100957,#100958,#100959,
#100960,#100961,#100962,#100963,#100964,#100965,#100966,#100967,#100968,
#100969,#100970,#100971,#100972,#100973,#100974,#100975,#100976,#100977,
#100978,#100979,#100980,#100981,#100982,#100983,#100984,#100985,#100986,
#100987,#100988,#100989,#100990,#100991,#100992,#100993,#100994,#100995,
#100996,#100997,#100998,#100999,#101000,#101001,#101002,#101003,#101004,
#101005,#101006,#101007,#101008,#101009,#101010,#101011,#101012,#101013,
#101014,#101015,#101016,#101017,#101018,#101019,#101020,#101021,#101022,
#101023,#101024,#101025,#101026,#101027,#101028,#101029,#101030,#101031,
#101032,#101033,#101034,#101035,#101036,#101037,#101038,#101039),
 .UNSPECIFIED.,.F.,.F.,(4,2,2,2,2,2,2,2,2,2,2,2,2,2,2,2,2,2,2,2,2,2,2,2,
2,2,2,2,2,2,2,2,2,2,2,2,2,2,2,2,2,2,2,2,2,2,2,2,2,2,2,2,2,2,2,2,2,2,2,2,
2,2,2,2,2,2,2,2,2,2,2,2,2,2,2,2,2,2,2,2,2,2,2,2,2,2,2,2,2,2,2,2,2,2,2,2,
2,2,2,2,2,2,2,2,2,2,2,2,2,4),(-2.96750086879726,-2.96659381553983,-2.96566234470614,
-2.96397271119722,-2.9610817025472,-2.94935671779514,-2.94114237626293,
-2.92562380844789,-2.91095596322626,-2.90900636756406,-2.90798963910852,
-2.90715199860394,-2.90611398543103,-2.90412423733864,-2.88975693764299,
-2.88480095240155,-2.86754019977096,-2.85866994608347,-2.85271443192878,
-2.85046415054895,-2.8490623648705,-2.8475832178978,-2.84556578763806,-2.84112921401378,
-2.8166088453051,-2.80026584222002,-2.79542855840305,-2.79219684172702,
-2.7909514510463,-2.79008674710252,-2.78929170689931,-2.78817888307029,
-2.78524182367117,-2.76707832462089,-2.75143065220629,-2.74175846499277,
-2.73749195156003,-2.73409590434219,-2.73229234937941,-2.73081298269155,
-2.72906521035275,-2.72601743611279,-2.71227319673704,-2.68759061762133,
-2.67973481679985,-2.67665899579946,-2.67436976402665,-2.6732850808675,
-2.67245229921497,-2.67147586509102,-2.6697630765253,-2.66248541161207,
-2.63145086921952,-2.61912557406169,-2.61624679612206,-2.61455390465507,
-2.61305538734124,-2.61117201287294,-2.60821527221347,-2.58922747840533,
-2.56677171569434,-2.55829014517698,-2.55655950286485,-2.55558937762736,
-2.55474767326373,-2.55366722481265,-2.55187396304261,-2.5393966653032,
-2.50981136243578,-2.50110574645628,-2.49852337370193,-2.49689536759146,
-2.49538099081942,-2.49340600184759,-2.48901808423033,-2.46172759139055,
-2.44155559660842,-2.43938879777495,-2.43832796212388,-2.43756976992492,
-2.43660529723624,-2.43494465111538,-2.42834422747228,-2.42171496317697,
-2.39179468298425,-2.38354933231851,-2.3810146825189,-2.37939706004146,
-2.37787857863445,-2.3758782364563,-2.37134688577835,-2.34745426195576,
-2.33061921715309,-2.3257030358317,-2.32243226483154,-2.32118101744791,
-2.32031520016361,-2.31952149715098,-2.31841365449556,-2.31551489261125,
-2.29482873909818,-2.29315787154553,-2.26771780909957,-2.2643076116996,
-2.26250121043244,-2.26102185618847,-2.25927684515296,-2.25624086117816,
-2.24272104725783,-2.22568207937383),.UNSPECIFIED.);
#1525=B_SPLINE_CURVE_WITH_KNOTS('',3,(#101044,#101045,#101046,#101047,#101048,
#101049,#101050,#101051,#101052,#101053,#101054,#101055,#101056,#101057,
#101058,#101059,#101060,#101061,#101062,#101063,#101064,#101065,#101066,
#101067,#101068,#101069,#101070,#101071,#101072,#101073,#101074,#101075,
#101076,#101077,#101078,#101079,#101080,#101081,#101082,#101083,#101084,
#101085,#101086,#101087,#101088,#101089,#101090,#101091,#101092,#101093,
#101094,#101095,#101096,#101097,#101098,#101099,#101100,#101101,#101102,
#101103,#101104,#101105,#101106,#101107,#101108,#101109,#101110,#101111,
#101112,#101113,#101114,#101115,#101116,#101117,#101118,#101119,#101120,
#101121,#101122,#101123,#101124,#101125,#101126,#101127,#101128,#101129,
#101130,#101131,#101132,#101133,#101134,#101135,#101136,#101137,#101138,
#101139,#101140,#101141,#101142,#101143,#101144,#101145,#101146,#101147,
#101148,#101149,#101150,#101151,#101152,#101153,#101154,#101155,#101156,
#101157,#101158,#101159,#101160,#101161,#101162,#101163,#101164,#101165,
#101166,#101167,#101168,#101169,#101170,#101171,#101172,#101173,#101174,
#101175,#101176,#101177,#101178,#101179,#101180,#101181,#101182,#101183,
#101184,#101185,#101186,#101187,#101188,#101189,#101190,#101191,#101192,
#101193,#101194,#101195,#101196,#101197,#101198,#101199,#101200,#101201,
#101202,#101203,#101204,#101205,#101206,#101207,#101208,#101209,#101210,
#101211,#101212,#101213,#101214,#101215,#101216,#101217,#101218,#101219,
#101220,#101221,#101222,#101223,#101224,#101225,#101226,#101227,#101228,
#101229,#101230,#101231,#101232,#101233,#101234,#101235,#101236,#101237,
#101238,#101239,#101240,#101241,#101242,#101243,#101244,#101245,#101246,
#101247),.UNSPECIFIED.,.F.,.F.,(4,2,2,2,2,2,2,2,2,2,2,2,2,2,2,2,2,2,2,2,
2,2,2,2,2,2,2,2,2,2,2,2,2,2,2,2,2,2,2,2,2,2,2,2,2,2,2,2,2,2,2,2,2,2,2,2,
2,2,2,2,2,2,2,2,2,2,2,2,2,2,2,2,2,2,2,2,2,2,2,2,2,2,2,2,2,2,2,2,2,2,2,2,
2,2,2,2,2,2,2,2,2,4),(-1.27966587227297,-1.272229553693,-1.24231524967437,
-1.23566675406253,-1.22910608887625,-1.22744806857877,-1.22648383674135,
-1.22572501586584,-1.22466222995535,-1.22248756132775,-1.20498420611661,
-1.17456296225542,-1.17048969707102,-1.16855076009953,-1.1670453691952,
-1.1653829949818,-1.16264660018661,-1.15226526909598,-1.13233710476868,
-1.11365923393185,-1.11072765119195,-1.10961505462486,-1.10881977465045,
-1.10795432555878,-1.10670704385205,-1.10346578746735,-1.09861074663655,
-1.08216234110127,-1.05777793164239,-1.05325615177723,-1.05125671993242,
-1.04973762095168,-1.0481180774026,-1.04557775571645,-1.03728910733969,
-1.00736230565903,-1.0007149522592,-0.994146644174214,-0.992487944047101,
-0.991523535473559,-0.990764712032883,-0.989702099812687,-0.987528423598759,
-0.970061955180934,-0.939590808048614,-0.935523591644476,-0.9335857623448,
-0.932080464362188,-0.93041741520764,-0.927678108280225,-0.917262197845361,
-0.897214751229519,-0.878694582583011,-0.875762836113375,-0.874650193336952,
-0.873854883947281,-0.872989407010776,-0.871742092052779,-0.868500787591783,
-0.863645707359806,-0.84719752378669,-0.822811238550126,-0.818289329988472,
-0.816289834188434,-0.8147706838671,-0.813151082937947,-0.810610665694105,
-0.80232165367715,-0.772393885050031,-0.765746296522921,-0.759177801588982,
-0.757519047790598,-0.756554606878571,-0.755795757285973,-0.754733107525846,
-0.752559351221373,-0.735092089804921,-0.704620150260785,-0.700552762210098,
-0.698614860337424,-0.697109509968391,-0.695446406980943,-0.692707020752121,
-0.682290931473667,-0.662243417765353,-0.643721785187141,-0.640789939111242,
-0.639677258289613,-0.638881921650265,-0.63801641499628,-0.636769057104699,
-0.633527640490277,-0.628672391768234,-0.612223631952927,-0.587836526034994,
-0.583314461950113,-0.581314897488488,-0.579795695042388,-0.578176038582264,
-0.575635534320366,-0.567346239168023,-0.537529498082018),.UNSPECIFIED.);
#1526=B_SPLINE_CURVE_WITH_KNOTS('',3,(#101248,#101249,#101250,#101251,#101252,
#101253,#101254,#101255,#101256,#101257,#101258,#101259,#101260,#101261,
#101262,#101263,#101264,#101265,#101266,#101267,#101268,#101269,#101270,
#101271,#101272,#101273,#101274,#101275,#101276,#101277,#101278,#101279,
#101280,#101281,#101282,#101283,#101284,#101285,#101286,#101287,#101288,
#101289,#101290,#101291,#101292,#101293,#101294,#101295,#101296,#101297,
#101298,#101299,#101300,#101301,#101302,#101303,#101304,#101305,#101306,
#101307,#101308,#101309,#101310,#101311,#101312,#101313,#101314,#101315,
#101316,#101317,#101318,#101319,#101320,#101321,#101322,#101323,#101324,
#101325,#101326,#101327,#101328,#101329,#101330,#101331,#101332,#101333,
#101334,#101335,#101336,#101337,#101338,#101339,#101340,#101341,#101342,
#101343,#101344,#101345,#101346,#101347,#101348,#101349,#101350,#101351,
#101352,#101353,#101354,#101355,#101356,#101357,#101358,#101359,#101360,
#101361,#101362,#101363,#101364,#101365,#101366,#101367,#101368,#101369,
#101370,#101371,#101372,#101373,#101374,#101375,#101376,#101377,#101378,
#101379,#101380,#101381,#101382,#101383,#101384,#101385,#101386,#101387,
#101388,#101389,#101390,#101391,#101392,#101393,#101394,#101395,#101396,
#101397,#101398,#101399,#101400,#101401,#101402,#101403,#101404,#101405,
#101406,#101407,#101408,#101409,#101410,#101411,#101412,#101413,#101414,
#101415,#101416,#101417,#101418,#101419,#101420,#101421,#101422,#101423,
#101424,#101425,#101426,#101427,#101428,#101429,#101430,#101431,#101432,
#101433,#101434,#101435,#101436,#101437,#101438,#101439,#101440,#101441,
#101442,#101443,#101444,#101445,#101446,#101447,#101448,#101449,#101450,
#101451,#101452,#101453,#101454,#101455,#101456,#101457),.UNSPECIFIED.,
 .F.,.F.,(4,2,2,2,2,2,2,2,2,2,2,2,2,2,2,2,2,2,2,2,2,2,2,2,2,2,2,2,2,2,2,
2,2,2,2,2,2,2,2,2,2,2,2,2,2,2,2,2,2,2,2,2,2,2,2,2,2,2,2,2,2,2,2,2,2,2,2,
2,2,2,2,2,2,2,2,2,2,2,2,2,2,2,2,2,2,2,2,2,2,2,2,2,2,2,2,2,2,2,2,2,2,2,2,
2,4),(-2.22568207937383,-2.2178550763344,-2.20996050804542,-2.20687464687162,
-2.20457965742834,-2.20349392601551,-2.20265351964583,-2.20167489394261,
-2.19995227863786,-2.19253328554911,-2.16164218072051,-2.14933535492842,
-2.14645796637081,-2.14476546629631,-2.14326703600014,-2.14138342463555,
-2.13842562978174,-2.11934775938661,-2.09697329055344,-2.08850581083454,
-2.08677605707526,-2.08580617431666,-2.0849645132728,-2.08388390907997,
-2.08208995556594,-2.06959072642165,-2.03997372232598,-2.03131741890679,
-2.02874017120338,-2.02711337079791,-2.02559872209595,-2.02362138036714,
-2.01921972390955,-1.99213992946854,-1.97178308683545,-1.96961611262615,
-1.96855529545168,-1.96779715900002,-1.96683281557215,-1.96517251881195,
-1.95857516983299,-1.95194600075082,-1.92203219501182,-1.91378229384877,
-1.91124729777793,-1.90962968979649,-1.90811138723478,-1.90611152209622,
-1.90158231869837,-1.87759287000226,-1.85617778127242,-1.8527232992923,
-1.85144513645397,-1.85057399667539,-1.84978584670233,-1.84869924843294,
-1.84593752013967,-1.82224624669334,-1.79796419568912,-1.79454388347424,
-1.79273544702362,-1.79138724829403,-1.78969202299961,-1.78680208324825,
-1.77588587450665,-1.75216290144899,-1.73794614617645,-1.73507924074646,
-1.73389168897721,-1.73303758273514,-1.73211263980119,-1.73058687994514,
-1.72556001326817,-1.69217385932536,-1.67959524900537,-1.67670038753949,
-1.67500417649623,-1.67350644282145,-1.67162899982318,-1.6686912736257,
-1.65061933690581,-1.62736407286598,-1.61875222682429,-1.61701464193775,
-1.61604311267743,-1.61520180888352,-1.61412391797587,-1.61233907363577,
-1.60009429297636,-1.57082737804266,-1.56165770766578,-1.5590301860362,
-1.55739250652819,-1.55588183691212,-1.55392962898009,-1.54966692078736,
-1.5209293389813,-1.50209108184843,-1.49988146952484,-1.49881232445706,
-1.49797332885811,-1.49698292804261,-1.49520812729529,-1.48698281804791,
-1.48384928743498),.UNSPECIFIED.);
#1527=B_SPLINE_CURVE_WITH_KNOTS('',3,(#101462,#101463,#101464,#101465,#101466,
#101467,#101468,#101469,#101470,#101471,#101472,#101473,#101474,#101475,
#101476,#101477,#101478,#101479,#101480,#101481,#101482,#101483,#101484,
#101485,#101486,#101487,#101488,#101489,#101490,#101491,#101492,#101493,
#101494,#101495,#101496,#101497,#101498,#101499,#101500,#101501,#101502,
#101503,#101504,#101505,#101506,#101507,#101508,#101509,#101510,#101511,
#101512,#101513,#101514,#101515,#101516,#101517,#101518,#101519,#101520,
#101521,#101522,#101523,#101524,#101525,#101526,#101527,#101528,#101529,
#101530,#101531,#101532,#101533,#101534,#101535,#101536,#101537,#101538,
#101539,#101540,#101541,#101542,#101543,#101544,#101545,#101546,#101547,
#101548,#101549,#101550,#101551,#101552,#101553,#101554,#101555,#101556,
#101557,#101558,#101559,#101560,#101561,#101562,#101563,#101564,#101565,
#101566,#101567,#101568,#101569,#101570,#101571,#101572,#101573,#101574,
#101575,#101576,#101577,#101578,#101579,#101580,#101581,#101582,#101583,
#101584,#101585,#101586,#101587,#101588,#101589,#101590,#101591,#101592,
#101593,#101594,#101595,#101596,#101597,#101598,#101599,#101600,#101601,
#101602,#101603,#101604,#101605,#101606,#101607,#101608,#101609,#101610,
#101611,#101612,#101613,#101614,#101615,#101616,#101617,#101618,#101619,
#101620,#101621,#101622,#101623,#101624,#101625,#101626,#101627,#101628,
#101629,#101630,#101631,#101632,#101633,#101634,#101635,#101636,#101637,
#101638,#101639,#101640,#101641,#101642,#101643,#101644,#101645,#101646,
#101647,#101648,#101649,#101650,#101651,#101652,#101653,#101654,#101655,
#101656,#101657,#101658,#101659,#101660,#101661,#101662,#101663,#101664,
#101665,#101666,#101667,#101668,#101669,#101670,#101671,#101672,#101673,
#101674,#101675),.UNSPECIFIED.,.F.,.F.,(4,2,2,2,2,2,2,2,2,2,2,2,2,2,2,2,
2,2,2,2,2,2,2,2,2,2,2,2,2,2,2,2,2,2,2,2,2,2,2,2,2,2,2,2,2,2,2,2,2,2,2,2,
2,2,2,2,2,2,2,2,2,2,2,2,2,2,2,2,2,2,2,2,2,2,2,2,2,2,2,2,2,2,2,2,2,2,2,2,
2,2,2,2,2,2,2,2,2,2,2,2,2,2,2,2,2,2,4),(-2.02162775575412,-2.02147662782479,
-1.99579917719131,-1.99236999230877,-1.9905590974704,-1.98920999891803,
-1.98751485866348,-1.98462806222062,-1.97376679701779,-1.94689196501622,
-1.93427540470258,-1.9323753699355,-1.93136869038776,-1.93053022739403,
-1.92947974854527,-1.92782606531596,-1.91895789189624,-1.88946352597479,
-1.87734105365018,-1.87447490275668,-1.87278426784987,-1.87128457903486,
-1.86939548216155,-1.86642133576316,-1.84379852215493,-1.82744916164141,
-1.81670891442864,-1.81487219767349,-1.8138789560533,-1.81303964054625,
-1.81197273424283,-1.81026462778585,-1.80028619653179,-1.77708718181986,
-1.76179829786174,-1.75780489701819,-1.75588134780566,-1.75437796803572,
-1.75270764804842,-1.74993436713586,-1.73909076913937,-1.71748189494616,
-1.71667938370067,-1.69959312984664,-1.69758663409149,-1.69654469670994,
-1.69570654291272,-1.69469237137944,-1.69275654060829,-1.6787508954603,
-1.6565595797421,-1.64285580237271,-1.63980942276381,-1.63806149034949,
-1.63658142537093,-1.63477632006471,-1.63137519601336,-1.60436196535677,
-1.58351503169303,-1.58062033590652,-1.5795126105778,-1.57871865380714,
-1.57785214722016,-1.57659920134281,-1.57331993583358,-1.56838797398566,
-1.55145656216529,-1.52770656023906,-1.52317234659849,-1.52117081895816,
-1.51965145200251,-1.51803289495087,-1.51549678861445,-1.5072467059908,
-1.47729328112608,-1.47064976042364,-1.46406354056792,-1.46240341567264,
-1.46143871841482,-1.46068000451188,-1.45961798269716,-1.45744708249859,
-1.44007364837657,-1.40948450649961,-1.40543294077683,-1.40349816537977,
-1.40199332725761,-1.40032884344286,-1.39758266129586,-1.38708109250646,
-1.36673193862266,-1.34863137185491,-1.34568832245574,-1.34457429740133,
-1.34377865532294,-1.34291357043371,-1.34166806439913,-1.33843837295501,
-1.33360655304634,-1.31730071386141,-1.29272880313439,-1.28821225078702,
-1.28621377740751,-1.28469487836143,-1.28307503958348,-1.280533186487,-1.27966587227297),
 .UNSPECIFIED.);
#1528=B_SPLINE_CURVE_WITH_KNOTS('',3,(#101676,#101677,#101678,#101679,#101680,
#101681,#101682,#101683,#101684,#101685,#101686,#101687,#101688,#101689,
#101690,#101691,#101692,#101693,#101694,#101695,#101696,#101697,#101698,
#101699,#101700,#101701,#101702,#101703,#101704,#101705,#101706,#101707,
#101708,#101709,#101710,#101711,#101712,#101713,#101714,#101715,#101716,
#101717,#101718,#101719,#101720,#101721,#101722,#101723,#101724,#101725,
#101726,#101727,#101728,#101729,#101730,#101731,#101732,#101733,#101734,
#101735,#101736,#101737,#101738,#101739,#101740,#101741,#101742,#101743,
#101744,#101745,#101746,#101747,#101748,#101749,#101750,#101751,#101752,
#101753,#101754,#101755,#101756,#101757,#101758,#101759,#101760,#101761,
#101762,#101763,#101764,#101765,#101766,#101767,#101768,#101769,#101770,
#101771,#101772,#101773,#101774,#101775,#101776,#101777,#101778,#101779,
#101780,#101781,#101782,#101783,#101784,#101785,#101786,#101787,#101788,
#101789,#101790,#101791,#101792,#101793,#101794,#101795,#101796,#101797,
#101798,#101799,#101800,#101801,#101802,#101803,#101804,#101805,#101806,
#101807,#101808,#101809,#101810,#101811,#101812,#101813,#101814,#101815,
#101816,#101817,#101818,#101819,#101820,#101821,#101822,#101823,#101824,
#101825,#101826,#101827,#101828,#101829,#101830,#101831,#101832,#101833,
#101834,#101835,#101836,#101837,#101838,#101839,#101840,#101841,#101842,
#101843,#101844,#101845,#101846,#101847,#101848,#101849,#101850,#101851,
#101852,#101853,#101854,#101855,#101856,#101857,#101858,#101859,#101860,
#101861,#101862,#101863,#101864,#101865,#101866,#101867,#101868,#101869,
#101870,#101871,#101872,#101873,#101874,#101875,#101876,#101877,#101878,
#101879,#101880,#101881),.UNSPECIFIED.,.F.,.F.,(4,2,2,2,2,2,2,2,2,2,2,2,
2,2,2,2,2,2,2,2,2,2,2,2,2,2,2,2,2,2,2,2,2,2,2,2,2,2,2,2,2,2,2,2,2,2,2,2,
2,2,2,2,2,2,2,2,2,2,2,2,2,2,2,2,2,2,2,2,2,2,2,2,2,2,2,2,2,2,2,2,2,2,2,2,
2,2,2,2,2,2,2,2,2,2,2,2,2,2,2,2,2,2,4),(-1.48384928743498,-1.48371487514913,
-1.45992098907207,-1.45316751042258,-1.44435845282337,-1.44166795103817,
-1.44001642210639,-1.43850972897545,-1.4365533128346,-1.43238267017394,
-1.41570153769621,-1.39714765591542,-1.39052852106685,-1.38382530265048,
-1.38215634381116,-1.38119006452188,-1.38043231583846,-1.37937452679372,
-1.37722256323148,-1.3592887795006,-1.32937980589441,-1.32524768930559,
-1.32331947571404,-1.32181226388046,-1.32016304265725,-1.31748280202988,
-1.30774048718393,-1.28914981928658,-1.26836283430222,-1.26546756892906,
-1.26436028286843,-1.26356680453757,-1.26270102249211,-1.2614494843269,
-1.2581759739495,-1.25325457770005,-1.23638245168105,-1.21257079640948,
-1.20803988659005,-1.20603980200214,-1.20452153433703,-1.20290415785877,
-1.20036993480368,-1.19212659200106,-1.1621924355117,-1.15555392058275,
-1.14895623076907,-1.147295924445,-1.1463316061485,-1.14557349983231,-1.14451275228775,
-1.14234599394355,-1.12188557254686,-1.09494687991804,-1.09053795209298,
-1.08855934383968,-1.08704451734614,-1.08541830061073,-1.08284363912912,
-1.07421277475296,-1.04456084817699,-1.03204279963325,-1.03024818877804,
-1.02916739664843,-1.02832571679146,-1.02735594954993,-1.0256267447897,
-1.01716827935652,-0.994842791709283,-0.975732558151765,-0.972774618471869,
-0.970890933631439,-0.969392468262866,-0.967699953168219,-0.96482260489375,
-0.952518134542969,-0.921665753420448,-0.914186137862191,-0.912459226949321,
-0.911479589805214,-0.910639252803292,-0.909554839380846,-0.907266931489033,
-0.904193666742227,-0.896347999719222,-0.871702172569502,-0.857935787844761,
-0.854887079176965,-0.85313910364302,-0.851659758347692,-0.849856465839474,
-0.84646164810969,-0.821458411157971,-0.798454693664855,-0.795663099149229,
-0.794571323303341,-0.793781759808521,-0.79291180806615,-0.791640045586063,
-0.788230762433554,-0.783031897915181,-0.764315199738776,-0.742062386064265),
 .UNSPECIFIED.);
#1529=B_SPLINE_CURVE_WITH_KNOTS('',3,(#101886,#101887,#101888,#101889,#101890,
#101891,#101892,#101893,#101894,#101895,#101896,#101897,#101898,#101899,
#101900,#101901,#101902,#101903,#101904,#101905,#101906,#101907,#101908,
#101909,#101910,#101911,#101912,#101913,#101914,#101915,#101916,#101917,
#101918,#101919,#101920,#101921,#101922,#101923,#101924,#101925,#101926,
#101927,#101928,#101929,#101930,#101931,#101932,#101933,#101934,#101935,
#101936,#101937,#101938,#101939,#101940,#101941,#101942,#101943,#101944,
#101945,#101946,#101947,#101948,#101949,#101950,#101951,#101952,#101953,
#101954,#101955,#101956,#101957,#101958,#101959,#101960,#101961,#101962,
#101963,#101964,#101965,#101966,#101967,#101968,#101969,#101970,#101971,
#101972,#101973,#101974,#101975,#101976,#101977,#101978,#101979,#101980,
#101981,#101982,#101983,#101984,#101985,#101986,#101987,#101988,#101989,
#101990,#101991,#101992,#101993,#101994,#101995,#101996,#101997,#101998,
#101999,#102000,#102001,#102002,#102003,#102004,#102005,#102006,#102007,
#102008,#102009,#102010,#102011,#102012,#102013,#102014,#102015,#102016,
#102017,#102018,#102019,#102020,#102021,#102022,#102023,#102024,#102025,
#102026,#102027,#102028,#102029,#102030,#102031,#102032,#102033,#102034,
#102035,#102036,#102037,#102038,#102039,#102040,#102041,#102042,#102043,
#102044,#102045,#102046,#102047,#102048,#102049,#102050,#102051,#102052,
#102053,#102054,#102055,#102056,#102057,#102058,#102059,#102060,#102061,
#102062,#102063,#102064,#102065,#102066,#102067,#102068,#102069,#102070,
#102071,#102072,#102073,#102074,#102075,#102076,#102077,#102078,#102079,
#102080,#102081,#102082,#102083,#102084,#102085,#102086,#102087,#102088,
#102089,#102090,#102091,#102092,#102093,#102094,#102095,#102096,#102097,
#102098,#102099,#102100,#102101,#102102,#102103,#102104,#102105),
 .UNSPECIFIED.,.F.,.F.,(4,2,2,2,2,2,2,2,2,2,2,2,2,2,2,2,2,2,2,2,2,2,2,2,
2,2,2,2,2,2,2,2,2,2,2,2,2,2,2,2,2,2,2,2,2,2,2,2,2,2,2,2,2,2,2,2,2,2,2,2,
2,2,2,2,2,2,2,2,2,2,2,2,2,2,2,2,2,2,2,2,2,2,2,2,2,2,2,2,2,2,2,2,2,2,2,2,
2,2,2,2,2,2,2,2,2,2,2,2,2,4),(-2.76357650556602,-2.76333910123122,-2.75848438226922,
-2.7552437508587,-2.75399672052331,-2.7531314552273,-2.75233634816034,-2.75122400896148,
-2.74829302256299,-2.72990936421677,-2.70978783425493,-2.69935159453149,
-2.69661109385011,-2.69494802477304,-2.69344316032543,-2.69150652273189,
-2.68744420997499,-2.65692875403012,-2.63948578767287,-2.63731302871906,
-2.63625073083977,-2.63549208234201,-2.63452781436635,-2.6328692031118,
-2.62629883652042,-2.61966326564236,-2.58975804464378,-2.58147335285329,
-2.57893379777217,-2.57731462708841,-2.5757957953463,-2.57379659373902,
-2.56927483576058,-2.54488179704724,-2.52842665780175,-2.52357066505057,
-2.52032937925598,-2.51908222978033,-2.51821692474097,-2.51742181557619,
-2.51630951891588,-2.51337902209132,-2.49486851842749,-2.47484072004081,
-2.46443123965767,-2.46169288462138,-2.46003025727294,-2.4585252390341,
-2.45658762717991,-2.45252034902333,-2.42204219450288,-2.40456953800957,
-2.40239588673835,-2.40133339592048,-2.40057470858364,-2.39961052682485,
-2.39795235774239,-2.39138761855596,-2.38475079760956,-2.35485375792119,
-2.34655688386981,-2.34401599188356,-2.3423965025242,-2.34087774560954,
-2.33887918760444,-2.33436128514433,-2.30981819664569,-2.29347535034401,
-2.28863751470529,-2.28540522316763,-2.28415941353748,-2.2832943504381,
-2.28249891165476,-2.28138542392974,-2.27844569770715,-2.26032216225262,
-2.24001170065774,-2.22952147075715,-2.22677645841289,-2.22511234354426,
-2.22360761911942,-2.22167268271544,-2.21761964708966,-2.18702854666275,
-2.16964125581399,-2.16747000136533,-2.16640796618303,-2.16564931281343,
-2.16468477479765,-2.16302512669482,-2.1564430865538,-2.14980924478117,
-2.11988478137169,-2.11162305708371,-2.10908585485216,-2.10746713711236,
-2.10594799591339,-2.10394731470303,-2.09941748009255,-2.07537102088888,
-2.05865013439352,-2.05375136047925,-2.05048883559966,-2.04923844510154,
-2.04837247838587,-2.0475780312308,-2.04646833460141,-2.04355830397262,
-2.02328296612591,-2.02162775575412),.UNSPECIFIED.);
#1530=B_SPLINE_CURVE_WITH_KNOTS('',3,(#102106,#102107,#102108,#102109,#102110,
#102111,#102112,#102113,#102114,#102115,#102116,#102117,#102118,#102119,
#102120,#102121,#102122,#102123,#102124,#102125,#102126,#102127,#102128,
#102129,#102130,#102131,#102132,#102133,#102134,#102135,#102136,#102137,
#102138,#102139,#102140,#102141,#102142,#102143,#102144,#102145,#102146,
#102147,#102148,#102149,#102150,#102151,#102152,#102153,#102154,#102155,
#102156,#102157,#102158,#102159,#102160,#102161,#102162,#102163,#102164,
#102165,#102166,#102167,#102168,#102169,#102170,#102171,#102172,#102173,
#102174,#102175,#102176,#102177,#102178,#102179,#102180,#102181,#102182,
#102183,#102184,#102185,#102186,#102187,#102188,#102189,#102190,#102191,
#102192,#102193,#102194,#102195,#102196,#102197,#102198,#102199,#102200,
#102201,#102202,#102203,#102204,#102205,#102206,#102207,#102208,#102209,
#102210,#102211,#102212,#102213,#102214,#102215,#102216,#102217,#102218,
#102219,#102220,#102221,#102222,#102223,#102224,#102225,#102226,#102227,
#102228,#102229,#102230,#102231,#102232,#102233,#102234,#102235,#102236,
#102237,#102238,#102239,#102240,#102241,#102242,#102243,#102244,#102245,
#102246,#102247,#102248,#102249,#102250,#102251,#102252,#102253,#102254,
#102255,#102256,#102257,#102258,#102259,#102260,#102261,#102262,#102263,
#102264,#102265,#102266,#102267,#102268,#102269,#102270,#102271,#102272,
#102273,#102274,#102275,#102276,#102277,#102278,#102279,#102280,#102281,
#102282,#102283,#102284,#102285,#102286,#102287,#102288,#102289,#102290,
#102291,#102292,#102293,#102294,#102295,#102296,#102297,#102298,#102299,
#102300,#102301,#102302,#102303,#102304,#102305,#102306,#102307,#102308,
#102309,#102310,#102311,#102312,#102313,#102314,#102315,#102316,#102317),
 .UNSPECIFIED.,.F.,.F.,(4,2,2,2,2,2,2,2,2,2,2,2,2,2,2,2,2,2,2,2,2,2,2,2,
2,2,2,2,2,2,2,2,2,2,2,2,2,2,2,2,2,2,2,2,2,2,2,2,2,2,2,2,2,2,2,2,2,2,2,2,
2,2,2,2,2,2,2,2,2,2,2,2,2,2,2,2,2,2,2,2,2,2,2,2,2,2,2,2,2,2,2,2,2,2,2,2,
2,2,2,2,2,2,2,2,2,4),(-0.742062386064265,-0.74082383376707,-0.737869415397941,
-0.735986639034777,-0.734488050000979,-0.732794494203004,-0.729913149670426,
-0.717552972081476,-0.686257841443905,-0.679215895273211,-0.677520680049237,
-0.676548181575274,-0.675791032555118,-0.67474111797497,-0.672629736978213,
-0.669857428699497,-0.637223542329692,-0.623024817171694,-0.619953812077845,
-0.618200691867482,-0.616856440607815,-0.615114036658552,-0.612007516490281,
-0.595293529230479,-0.57053124605763,-0.561918932363373,-0.560278648945289,
-0.559232438360717,-0.558394418912458,-0.557384729251122,-0.555469375730979,
-0.542277148593382,-0.510745238808649,-0.504200542749606,-0.501792081941628,
-0.50036044778997,-0.498846718000441,-0.496842545239705,-0.492413052451229,
-0.486422502890039,-0.457038989206241,-0.444712997222777,-0.442924941834431,
-0.441845945351214,-0.441004302802943,-0.440032984615947,-0.438297228970429,
-0.429725133269381,-0.406720517678837,-0.38837707567522,-0.385432126285059,
-0.383552160700355,-0.382053758703231,-0.380358226481331,-0.377468095427148,
-0.364974867739976,-0.332504153034069,-0.326601134473886,-0.324983529793714,
-0.324038031820967,-0.323190646977257,-0.322047689270369,-0.319442850933044,
-0.307766043937616,-0.280185911257941,-0.270093871003887,-0.267264959762892,
-0.265582689793245,-0.264232092710329,-0.262403853495407,-0.258889455265981,
-0.235374619354801,-0.210929544415633,-0.208226356486813,-0.207153561441298,
-0.206368704155963,-0.205493153490716,-0.204194672154184,-0.200598482719977,
-0.195007704204448,-0.174508802421658,-0.153473193464271,-0.150494726168837,
-0.148604457188224,-0.147104848829453,-0.145415380194428,-0.142700409556506,
-0.132719799042709,-0.112848589275792,-0.0938092476952492,-0.0908709478082895,
-0.0897577058029344,-0.0889623967724351,-0.0880974265373271,-0.0868517016312246,
-0.0837240513991225,-0.0690248805669019,-0.0544089790042287,-0.0359591647858924,
-0.0330113274865467,-0.0311302678909457,-0.0296314706306193,-0.0279359999577877,
-0.0261731935859782,-0.0235150047612098,-9.99999999584666E-7),
 .UNSPECIFIED.);
#1531=B_SPLINE_CURVE_WITH_KNOTS('',3,(#102322,#102323,#102324,#102325,#102326,
#102327,#102328,#102329,#102330,#102331,#102332,#102333,#102334,#102335,
#102336,#102337,#102338,#102339,#102340,#102341,#102342,#102343,#102344,
#102345,#102346,#102347,#102348,#102349,#102350,#102351,#102352,#102353,
#102354,#102355,#102356,#102357,#102358,#102359,#102360,#102361,#102362,
#102363,#102364,#102365,#102366,#102367,#102368,#102369,#102370,#102371,
#102372,#102373,#102374,#102375,#102376,#102377,#102378,#102379,#102380,
#102381,#102382,#102383,#102384,#102385,#102386,#102387,#102388,#102389,
#102390,#102391,#102392,#102393,#102394,#102395,#102396,#102397,#102398,
#102399,#102400,#102401,#102402,#102403,#102404,#102405,#102406,#102407,
#102408,#102409,#102410,#102411,#102412,#102413,#102414,#102415,#102416,
#102417,#102418,#102419,#102420,#102421,#102422,#102423,#102424,#102425,
#102426,#102427,#102428,#102429,#102430,#102431,#102432,#102433,#102434,
#102435,#102436,#102437,#102438,#102439,#102440,#102441,#102442,#102443,
#102444,#102445,#102446,#102447,#102448,#102449,#102450,#102451,#102452,
#102453,#102454,#102455,#102456,#102457,#102458,#102459,#102460,#102461,
#102462,#102463,#102464,#102465,#102466,#102467,#102468,#102469,#102470,
#102471,#102472,#102473,#102474,#102475,#102476,#102477,#102478,#102479,
#102480,#102481,#102482,#102483,#102484,#102485,#102486,#102487,#102488,
#102489,#102490,#102491,#102492,#102493,#102494,#102495,#102496,#102497,
#102498,#102499,#102500,#102501,#102502,#102503,#102504,#102505,#102506,
#102507,#102508,#102509,#102510,#102511,#102512,#102513,#102514,#102515,
#102516,#102517,#102518,#102519,#102520,#102521,#102522,#102523,#102524,
#102525),.UNSPECIFIED.,.F.,.F.,(4,2,2,2,2,2,2,2,2,2,2,2,2,2,2,2,2,2,2,2,
2,2,2,2,2,2,2,2,2,2,2,2,2,2,2,2,2,2,2,2,2,2,2,2,2,2,2,2,2,2,2,2,2,2,2,2,
2,2,2,2,2,2,2,2,2,2,2,2,2,2,2,2,2,2,2,2,2,2,2,2,2,2,2,2,2,2,2,2,2,2,2,2,
2,2,2,2,2,2,2,2,2,4),(-3.5055211511763,-3.47946494400775,-3.46168294829212,
-3.45950078978816,-3.45843670135296,-3.45767791091164,-3.45671501789293,
-3.45506213297972,-3.4485584203116,-3.44191116699937,-3.41210875999234,
-3.40651548446923,-3.40359891009418,-3.40119027356962,-3.39960405615639,
-3.39815310481854,-3.39621654399659,-3.39215413455514,-3.3616441099215,
-3.34420039502125,-3.34202775143225,-3.34096552807006,-3.34020694015761,
-3.33924275928536,-3.33758431974529,-3.3310149222981,-3.32437981353755,
-3.2944777058399,-3.28619279835907,-3.2836533559628,-3.28203429697311,-3.28051559792107,
-3.27851661170238,-3.27399552031847,-3.24959614891806,-3.23314855281832,
-3.22829395934054,-3.22505343584816,-3.22380646340187,-3.22294124356671,
-3.22214618251995,-3.22103391331147,-3.21810315791383,-3.1997139511651,
-3.17959838154418,-3.16916410379622,-3.16642386739735,-3.16476091456905,
-3.16325612693956,-3.16131954843232,-3.15725721006259,-3.12674537660817,
-3.10930187620266,-3.10712919391382,-3.1060669459508,-3.10530833815878,
-3.10434412885242,-3.10268563353998,-3.09611592456874,-3.0894806631881,
-3.05957754451498,-3.05129269501063,-3.04875321432321,-3.04713411842615,
-3.04561537600109,-3.04361631992141,-3.03909501427405,-3.01469530255772,
-2.99824712789313,-2.99339238207356,-2.99015176071685,-2.98890475320324,
-2.9880395098748,-2.98724442791264,-2.98613213033272,-2.9832013075556,-2.96481051331061,
-2.94469521644095,-2.93426089143454,-2.93152060068324,-2.92985760749354,
-2.92835277859863,-2.92641614033669,-2.92235365161984,-2.8918413266534,
-2.87439710972965,-2.87222436213446,-2.87116208432121,-2.87040345605727,
-2.86943922188932,-2.86778068632549,-2.86121085106628,-2.85457540284204,
-2.82467156040574,-2.81638638663323,-2.8138468270709,-2.81222768545878,
-2.81070890335604,-2.80870979972494,-2.80418840712191,-2.77978670660156,
-2.76357650556602),.UNSPECIFIED.);
#1532=B_SPLINE_CURVE_WITH_KNOTS('',3,(#102526,#102527,#102528,#102529,#102530,
#102531,#102532,#102533,#102534,#102535,#102536,#102537,#102538,#102539,
#102540,#102541,#102542,#102543,#102544,#102545,#102546,#102547,#102548,
#102549,#102550,#102551,#102552,#102553,#102554,#102555,#102556,#102557,
#102558,#102559,#102560,#102561,#102562,#102563,#102564,#102565,#102566,
#102567,#102568,#102569,#102570,#102571,#102572,#102573,#102574,#102575,
#102576,#102577,#102578,#102579,#102580,#102581,#102582,#102583,#102584,
#102585,#102586,#102587,#102588,#102589,#102590,#102591,#102592,#102593,
#102594,#102595,#102596,#102597,#102598,#102599,#102600,#102601,#102602,
#102603,#102604,#102605,#102606,#102607,#102608,#102609,#102610,#102611,
#102612,#102613,#102614,#102615,#102616,#102617,#102618,#102619,#102620,
#102621,#102622,#102623,#102624,#102625,#102626,#102627,#102628,#102629,
#102630,#102631,#102632,#102633,#102634,#102635,#102636,#102637,#102638,
#102639,#102640,#102641,#102642,#102643,#102644,#102645,#102646,#102647,
#102648,#102649,#102650,#102651,#102652,#102653,#102654,#102655,#102656,
#102657,#102658,#102659,#102660,#102661,#102662,#102663,#102664,#102665,
#102666,#102667,#102668,#102669,#102670,#102671,#102672,#102673,#102674,
#102675,#102676,#102677,#102678,#102679,#102680,#102681,#102682,#102683,
#102684,#102685,#102686,#102687,#102688,#102689,#102690,#102691,#102692,
#102693,#102694,#102695,#102696,#102697,#102698,#102699,#102700,#102701,
#102702,#102703,#102704,#102705,#102706,#102707,#102708,#102709,#102710,
#102711,#102712,#102713,#102714,#102715,#102716,#102717,#102718,#102719,
#102720,#102721,#102722,#102723,#102724,#102725,#102726,#102727,#102728,
#102729,#102730,#102731,#102732,#102733,#102734,#102735),.UNSPECIFIED.,
 .F.,.F.,(4,2,2,2,2,2,2,2,2,2,2,2,2,2,2,2,2,2,2,2,2,2,2,2,2,2,2,2,2,2,2,
2,2,2,2,2,2,2,2,2,2,2,2,2,2,2,2,2,2,2,2,2,2,2,2,2,2,2,2,2,2,2,2,2,2,2,2,
2,2,2,2,2,2,2,2,2,2,2,2,2,2,2,2,2,2,2,2,2,2,2,2,2,2,2,2,2,2,2,2,2,2,2,2,
2,4),(-1.48409509776007,-1.46365215592803,-1.45894857869465,-1.45752538571778,
-1.45627895076673,-1.45541393438915,-1.45461893789389,-1.45350661279528,
-1.45057452074908,-1.43256199634338,-1.41883674487716,-1.40287855432187,
-1.39953011832661,-1.3976885277089,-1.3961930247133,-1.39447035172652,-1.39153381016838,
-1.37951746797466,-1.35060641309532,-1.34119379256165,-1.33942833022474,
-1.33842056381484,-1.33758235370359,-1.33653366860193,-1.33488549223496,
-1.32612181995249,-1.29652178425105,-1.28438393670057,-1.28151713778624,
-1.27982659839912,-1.2783272933426,-1.2764390878579,-1.27346717177484,-1.25290435787762,
-1.23198666126393,-1.22355262278279,-1.22182432778564,-1.22085456877064,
-1.22001256081625,-1.21893093617151,-1.2171341083745,-1.20456891381828,
-1.17484723907971,-1.16632122444403,-1.16375674113247,-1.16213237408773,
-1.16061610126748,-1.15863103527661,-1.15418811222316,-1.12778174831265,
-1.10678708944923,-1.1046251806104,-1.10356516056424,-1.10280690625202,
-1.10184146901521,-1.10017723391488,-1.09353676262251,-1.06185144505965,
-1.04944696007946,-1.04656256101016,-1.04486822415544,-1.04336955914616,
-1.0414875072937,-1.03853581018435,-1.01988347242787,-0.997127035032357,
-0.988594396712029,-0.98686066710911,-0.985889748373163,-0.985047966850505,
-0.983968191967646,-0.98217762928574,-0.969782957786556,-0.940313378555806,
-0.931429311382468,-0.928828797385757,-0.927196613440196,-0.925683306009111,
-0.923716769363117,-0.919538735147668,-0.890475169719944,-0.87726591875141,
-0.872984620645554,-0.870035223591483,-0.868833926873195,-0.867977244406281,
-0.867170964719169,-0.865780332654773,-0.861830798468349,-0.837761487244635,
-0.81552611735145,-0.812055823235516,-0.810236723668568,-0.808887143737685,
-0.807198728495439,-0.804341414157621,-0.793856607299055,-0.766627498662389,
-0.755013942443657,-0.752416297666676,-0.751274643637468,-0.750427480885756,
-0.749481395373951,-0.747861013757768,-0.742040097680754),.UNSPECIFIED.);
#1533=B_SPLINE_CURVE_WITH_KNOTS('',3,(#102740,#102741,#102742,#102743,#102744,
#102745,#102746,#102747,#102748,#102749,#102750,#102751,#102752,#102753,
#102754,#102755,#102756,#102757,#102758,#102759,#102760,#102761,#102762,
#102763,#102764,#102765,#102766,#102767,#102768,#102769,#102770,#102771,
#102772,#102773,#102774,#102775,#102776,#102777,#102778,#102779,#102780,
#102781,#102782,#102783,#102784,#102785,#102786,#102787,#102788,#102789,
#102790,#102791,#102792,#102793,#102794,#102795,#102796,#102797,#102798,
#102799,#102800,#102801,#102802,#102803,#102804,#102805,#102806,#102807,
#102808,#102809,#102810,#102811,#102812,#102813,#102814,#102815,#102816,
#102817,#102818,#102819,#102820,#102821,#102822,#102823,#102824,#102825,
#102826,#102827,#102828,#102829,#102830,#102831,#102832,#102833,#102834,
#102835,#102836,#102837,#102838,#102839,#102840,#102841,#102842,#102843,
#102844,#102845,#102846,#102847,#102848,#102849,#102850,#102851,#102852,
#102853,#102854,#102855,#102856,#102857,#102858,#102859,#102860,#102861,
#102862,#102863,#102864,#102865,#102866,#102867,#102868,#102869,#102870,
#102871,#102872,#102873,#102874,#102875,#102876,#102877,#102878,#102879,
#102880,#102881,#102882,#102883,#102884,#102885,#102886,#102887,#102888,
#102889,#102890,#102891,#102892,#102893,#102894,#102895,#102896,#102897,
#102898,#102899,#102900,#102901,#102902,#102903,#102904,#102905,#102906,
#102907,#102908,#102909,#102910,#102911,#102912,#102913,#102914,#102915,
#102916,#102917,#102918,#102919,#102920,#102921,#102922,#102923,#102924,
#102925,#102926,#102927,#102928,#102929,#102930,#102931,#102932,#102933,
#102934,#102935,#102936,#102937,#102938,#102939,#102940,#102941,#102942,
#102943,#102944,#102945,#102946,#102947,#102948,#102949,#102950,#102951,
#102952,#102953,#102954,#102955,#102956,#102957,#102958,#102959,#102960,
#102961),.UNSPECIFIED.,.F.,.F.,(4,2,2,2,2,2,2,2,2,2,2,2,2,2,2,2,2,2,2,2,
2,2,2,2,2,2,2,2,2,2,2,2,2,2,2,2,2,2,2,2,2,2,2,2,2,2,2,2,2,2,2,2,2,2,2,2,
2,2,2,2,2,2,2,2,2,2,2,2,2,2,2,2,2,2,2,2,2,2,2,2,2,2,2,2,2,2,2,2,2,2,2,2,
2,2,2,2,2,2,2,2,2,2,2,2,2,2,2,2,2,2,4),(-0.742107893903836,-0.723841853319381,
-0.719320036308527,-0.717320605986864,-0.715801515165782,-0.714181987051595,
-0.711641703722723,-0.703353312568062,-0.673426557298028,-0.666779265901727,
-0.660210904579521,-0.658552207345801,-0.657587803307021,-0.656828985198745,
-0.655766382744891,-0.653592734810197,-0.6361268694326,-0.605655289172278,
-0.60158818045023,-0.599650379294435,-0.598145093141986,-0.596482046885033,
-0.593742721155086,-0.583326430438049,-0.563277553853061,-0.544759596113452,
-0.541827866611508,-0.540715230880491,-0.539919926661509,-0.539054455534638,
-0.537807149207063,-0.534565868582421,-0.529710825252761,-0.513262779752363,
-0.488876618375661,-0.48435474083186,-0.482355258491555,-0.480836118297064,
-0.479216528068968,-0.476676127410474,-0.468387167662968,-0.438459600605826,
-0.431812056268836,-0.425243604475989,-0.423584861666512,-0.422620427161542,
-0.421861582615796,-0.420798939934875,-0.418625198170893,-0.40115805633814,
-0.370686314148645,-0.366618953700012,-0.364681064807605,-0.363175724447664,
-0.361512632443314,-0.358773264132004,-0.348357240711471,-0.328309848599026,
-0.309788354462662,-0.30685652783641,-0.30574385439837,-0.304948523037442,
-0.304083022125781,-0.302835672510451,-0.299594277407143,-0.294739060908434,
-0.278290410270541,-0.253903466263959,-0.249381432188862,-0.247381880993904,
-0.245862688625974,-0.244243042909015,-0.241702555495137,-0.233413315282159,
-0.203484717640983,-0.196836945248695,-0.190268268346267,-0.188609468631586,
-0.187645001029137,-0.186886130441864,-0.185823451288419,-0.183649634873507,
-0.166181891192656,-0.135709237451958,-0.131641652756981,-0.129703681301153,
-0.128251772401547,-0.128203928614175,-0.128147838639546,-0.126508698259215,
-0.12379643660391,-0.120540364508337,-0.113995975198164,-0.0949246555972127,
-0.0747877879742402,-0.0718720333933413,-0.0707613980199954,-0.0699665879501811,
-0.0691005743740268,-0.0678506997401898,-0.064592748913196,-0.0597041994055956,
-0.043048780056191,-0.0253408062907407,-0.0160132388697642,-0.0132661212629756,
-0.0116012437553241,-0.0101423569917107,-0.00868747148028448,-0.00682528125065143,
-9.99999999806711E-7),.UNSPECIFIED.);
#1534=B_SPLINE_CURVE_WITH_KNOTS('',3,(#102962,#102963,#102964,#102965,#102966,
#102967,#102968,#102969,#102970,#102971,#102972,#102973,#102974,#102975,
#102976,#102977,#102978,#102979,#102980,#102981,#102982,#102983,#102984,
#102985,#102986,#102987,#102988,#102989,#102990,#102991,#102992,#102993,
#102994,#102995,#102996,#102997,#102998,#102999,#103000,#103001,#103002,
#103003,#103004,#103005,#103006,#103007,#103008,#103009,#103010,#103011,
#103012,#103013,#103014,#103015,#103016,#103017,#103018,#103019,#103020,
#103021,#103022,#103023,#103024,#103025,#103026,#103027,#103028,#103029,
#103030,#103031,#103032,#103033,#103034,#103035,#103036,#103037,#103038,
#103039,#103040,#103041,#103042,#103043,#103044,#103045,#103046,#103047,
#103048,#103049,#103050,#103051,#103052,#103053,#103054,#103055,#103056,
#103057,#103058,#103059,#103060,#103061,#103062,#103063,#103064,#103065,
#103066,#103067,#103068,#103069,#103070,#103071,#103072,#103073,#103074,
#103075,#103076,#103077,#103078,#103079,#103080,#103081,#103082,#103083,
#103084,#103085,#103086,#103087,#103088,#103089,#103090,#103091,#103092,
#103093,#103094,#103095,#103096,#103097,#103098,#103099,#103100,#103101,
#103102,#103103,#103104,#103105,#103106,#103107,#103108,#103109,#103110,
#103111,#103112,#103113,#103114,#103115,#103116,#103117,#103118,#103119,
#103120,#103121,#103122,#103123,#103124,#103125,#103126,#103127,#103128,
#103129,#103130,#103131,#103132,#103133,#103134,#103135,#103136,#103137,
#103138,#103139,#103140,#103141,#103142,#103143,#103144,#103145,#103146,
#103147,#103148,#103149,#103150,#103151,#103152,#103153,#103154,#103155,
#103156,#103157,#103158,#103159,#103160,#103161,#103162,#103163,#103164,
#103165,#103166,#103167,#103168,#103169,#103170,#103171,#103172,#103173),
 .UNSPECIFIED.,.F.,.F.,(4,2,2,2,2,2,2,2,2,2,2,2,2,2,2,2,2,2,2,2,2,2,2,2,
2,2,2,2,2,2,2,2,2,2,2,2,2,2,2,2,2,2,2,2,2,2,2,2,2,2,2,2,2,2,2,2,2,2,2,2,
2,2,2,2,2,2,2,2,2,2,2,2,2,2,2,2,2,2,2,2,2,2,2,2,2,2,2,2,2,2,2,2,2,2,2,2,
2,2,2,2,2,2,2,2,2,4),(-0.742040097680754,-0.741928316738839,-0.729948429837609,
-0.700581075524223,-0.695542425395112,-0.693588135535638,-0.692169801554734,
-0.690648408539036,-0.688596297768509,-0.683895735696293,-0.677424338593979,
-0.658727895265965,-0.638074744638377,-0.635172542237828,-0.63406406152576,
-0.633270081316746,-0.632404161444009,-0.631153103407226,-0.627884682699124,
-0.622974225453668,-0.606176516502152,-0.582251276802361,-0.577720447887504,
-0.575719928478674,-0.574201147600775,-0.5725830485224,-0.570047324567895,
-0.561795679259194,-0.531854350531205,-0.525212905936097,-0.51861528004425,
-0.516954566125179,-0.51598993750859,-0.515231541389359,-0.514170328867937,
-0.512002407706218,-0.491353088467344,-0.464604519631965,-0.460181830168216,
-0.458200327983258,-0.45668459289826,-0.455058675157748,-0.452487210289166,
-0.443893904333654,-0.414201910572,-0.401660160644848,-0.399864180153527,
-0.398782780440167,-0.397940764362255,-0.396970769803733,-0.39524153842414,
-0.386790997580685,-0.364522495549996,-0.345329501187251,-0.342369487243714,
-0.340484806069431,-0.338985753835874,-0.337292794647745,-0.3344152314195,
-0.322119157400736,-0.291358202151315,-0.283771358635228,-0.282036716586524,
-0.281055102043267,-0.280214654522631,-0.279132152861841,-0.276855449423359,
-0.273801868303748,-0.266032681782011,-0.241804682236309,-0.227533902419892,
-0.224458636483646,-0.222704262133171,-0.221359663091233,-0.21961753888327,
-0.216513699605243,-0.199883958266859,-0.185584512826758,-0.176072632947613,
-0.166514301380018,-0.164825063537784,-0.163763899908974,-0.162925019634224,
-0.161927473862387,-0.160070265809172,-0.148775665594381,-0.124625080137313,
-0.110094233000793,-0.107281026250031,-0.105440969704503,-0.104040431693504,
-0.102412525399209,-0.0996952500842602,-0.0964155471588903,-0.0898023748472433,
-0.0703637819504087,-0.0507249973331295,-0.0478029150002421,-0.046691706948221,
-0.0458969147070438,-0.0450314269784657,-0.0437831729049783,-0.040534304718124,
-0.0356636560514601,-0.0191176910841187,-6.62583249990897E-6),
 .UNSPECIFIED.);
#1535=B_SPLINE_CURVE_WITH_KNOTS('',3,(#103178,#103179,#103180,#103181,#103182,
#103183,#103184,#103185,#103186,#103187,#103188,#103189,#103190,#103191,
#103192,#103193,#103194,#103195,#103196,#103197,#103198,#103199,#103200,
#103201,#103202,#103203,#103204,#103205,#103206,#103207,#103208,#103209,
#103210,#103211,#103212,#103213,#103214,#103215,#103216,#103217,#103218,
#103219,#103220,#103221,#103222,#103223,#103224,#103225,#103226,#103227,
#103228,#103229,#103230,#103231,#103232,#103233,#103234,#103235,#103236,
#103237,#103238,#103239,#103240,#103241,#103242,#103243,#103244,#103245,
#103246,#103247,#103248,#103249,#103250,#103251,#103252,#103253,#103254,
#103255,#103256,#103257,#103258,#103259,#103260,#103261,#103262,#103263,
#103264,#103265,#103266,#103267,#103268,#103269,#103270,#103271,#103272,
#103273,#103274,#103275,#103276,#103277,#103278,#103279,#103280,#103281,
#103282,#103283,#103284,#103285,#103286,#103287,#103288,#103289,#103290,
#103291,#103292,#103293,#103294,#103295,#103296,#103297,#103298,#103299,
#103300,#103301,#103302,#103303,#103304,#103305,#103306,#103307,#103308,
#103309,#103310,#103311,#103312,#103313,#103314,#103315,#103316,#103317,
#103318,#103319,#103320,#103321,#103322,#103323,#103324,#103325,#103326,
#103327,#103328,#103329,#103330,#103331,#103332,#103333,#103334,#103335,
#103336,#103337,#103338,#103339,#103340,#103341,#103342,#103343,#103344,
#103345,#103346,#103347,#103348,#103349,#103350,#103351,#103352,#103353,
#103354,#103355,#103356,#103357,#103358,#103359,#103360,#103361,#103362,
#103363,#103364,#103365,#103366,#103367,#103368,#103369,#103370,#103371,
#103372,#103373,#103374,#103375,#103376,#103377,#103378,#103379,#103380,
#103381,#103382,#103383,#103384,#103385,#103386,#103387,#103388,#103389,
#103390,#103391,#103392,#103393,#103394,#103395,#103396,#103397),
 .UNSPECIFIED.,.F.,.F.,(4,2,2,2,2,2,2,2,2,2,2,2,2,2,2,2,2,2,2,2,2,2,2,2,
2,2,2,2,2,2,2,2,2,2,2,2,2,2,2,2,2,2,2,2,2,2,2,2,2,2,2,2,2,2,2,2,2,2,2,2,
2,2,2,2,2,2,2,2,2,2,2,2,2,2,2,2,2,2,2,2,2,2,2,2,2,2,2,2,2,2,2,2,2,2,2,2,
2,2,2,2,2,2,2,2,2,2,2,2,2,4),(-1.48414558948818,-1.48411908994632,-1.48150694578538,
-1.48044544243452,-1.47958552297644,-1.478687693243,-1.477286240022,-1.47288123924991,
-1.46545376461459,-1.44928763031837,-1.42678032231691,-1.42380983174383,
-1.42192176081098,-1.42042207910756,-1.41873059608615,-1.4158609083301,
-1.40368904567457,-1.37386147878574,-1.3653189318069,-1.36368181590189,
-1.36263632346925,-1.36179795944122,-1.36078672343039,-1.35886530984397,
-1.34546393699799,-1.31210485620013,-1.30705775011344,-1.30510175249705,
-1.30368266115583,-1.30216090244843,-1.30010907506394,-1.29541258046905,
-1.28894903780427,-1.27029529868479,-1.2495831918066,-1.24668327816823,
-1.24557485436457,-1.24478071493853,-1.24391437837728,-1.24266228879128,
-1.2393887133285,-1.23446826986368,-1.21760979406714,-1.19376563663291,
-1.18923292319908,-1.18723166497245,-1.18571234965949,-1.18409370081681,
-1.18155714295618,-1.17330273714836,-1.14335281151292,-1.13670895393039,
-1.13012479415659,-1.12846484816156,-1.12750019564856,-1.12674147986364,
-1.12567940743781,-1.12350823216857,-1.10612488555948,-1.0755490087322,
-1.07149577540665,-1.06956068926336,-1.06805582044201,-1.0663915171053,
-1.06364613118333,-1.05315421443957,-1.0328391108324,-1.01469014356287,
-1.01174971615821,-1.0106360266862,-1.00984047645838,-1.00897532116534,
-1.00772943320862,-1.00449719442477,-0.999660242143345,-0.983322816758281,
-0.958793151854156,-0.954275439396426,-0.95227676856374,-0.950757842765568,
-0.949138094133479,-0.946596631904352,-0.938296609111291,-0.908379775618584,
-0.901731632282564,-0.895169287913151,-0.893511132114086,-0.892546871951334,
-0.89178806043779,-0.890725328663062,-0.888550917911768,-0.871056320912156,
-0.840623953302691,-0.836552135988929,-0.83461347987711,-0.833108130388723,
-0.831445622960339,-0.828708594653004,-0.818319460672918,-0.798364245401951,
-0.779722517813475,-0.776791111962173,-0.775678541907763,-0.774883271670317,
-0.77401782250983,-0.77277052317967,-0.769529123387601,-0.764673784720258,
-0.748223465298814,-0.742107893903836),.UNSPECIFIED.);
#1536=B_SPLINE_CURVE_WITH_KNOTS('',3,(#103399,#103400,#103401,#103402),
 .UNSPECIFIED.,.F.,.F.,(4,4),(-6.62583249990897E-6,-1.00000009449833E-6),
 .UNSPECIFIED.);
#1537=B_SPLINE_CURVE_WITH_KNOTS('',3,(#103403,#103404,#103405,#103406,#103407,
#103408,#103409,#103410,#103411,#103412,#103413,#103414,#103415,#103416,
#103417,#103418,#103419,#103420,#103421,#103422,#103423,#103424,#103425,
#103426,#103427,#103428,#103429,#103430,#103431,#103432,#103433,#103434,
#103435,#103436,#103437,#103438,#103439,#103440,#103441,#103442,#103443,
#103444,#103445,#103446,#103447,#103448,#103449,#103450,#103451,#103452,
#103453,#103454,#103455,#103456,#103457,#103458,#103459,#103460,#103461,
#103462,#103463,#103464,#103465,#103466,#103467,#103468,#103469,#103470,
#103471,#103472,#103473,#103474,#103475,#103476,#103477,#103478,#103479,
#103480,#103481,#103482,#103483,#103484,#103485,#103486,#103487,#103488,
#103489,#103490,#103491,#103492,#103493,#103494,#103495,#103496,#103497,
#103498,#103499,#103500,#103501,#103502,#103503,#103504,#103505,#103506,
#103507,#103508,#103509,#103510,#103511,#103512,#103513,#103514,#103515,
#103516,#103517,#103518,#103519,#103520,#103521,#103522,#103523,#103524,
#103525,#103526,#103527,#103528,#103529,#103530,#103531,#103532,#103533,
#103534,#103535,#103536,#103537,#103538,#103539,#103540,#103541,#103542,
#103543,#103544,#103545,#103546,#103547,#103548,#103549,#103550,#103551,
#103552,#103553,#103554,#103555,#103556,#103557,#103558,#103559,#103560,
#103561,#103562,#103563,#103564,#103565,#103566,#103567,#103568,#103569,
#103570,#103571,#103572,#103573,#103574,#103575,#103576,#103577,#103578,
#103579,#103580,#103581,#103582,#103583,#103584,#103585,#103586,#103587,
#103588,#103589,#103590,#103591,#103592,#103593,#103594,#103595,#103596,
#103597,#103598,#103599,#103600,#103601,#103602,#103603,#103604,#103605,
#103606,#103607,#103608,#103609,#103610,#103611,#103612,#103613,#103614,
#103615,#103616,#103617,#103618,#103619,#103620,#103621,#103622,#103623,
#103624,#103625,#103626,#103627,#103628,#103629,#103630,#103631,#103632),
 .UNSPECIFIED.,.F.,.F.,(4,2,2,2,2,2,2,2,2,2,2,2,2,2,2,2,2,2,2,2,2,2,2,2,
2,2,2,2,2,2,2,2,2,2,2,2,2,2,2,2,2,2,2,2,2,2,2,2,2,2,2,2,2,2,2,2,2,2,2,2,
2,2,2,2,2,2,2,2,2,2,2,2,2,2,2,2,2,2,2,2,2,2,2,2,2,2,2,2,2,2,2,2,2,2,2,2,
2,2,2,2,2,2,2,2,2,2,2,2,2,2,2,2,2,2,4),(-2.76158278095296,-2.75605222062093,
-2.75252015463855,-2.75079750115922,-2.74938169103857,-2.74803293709578,
-2.74629352434649,-2.74328139975011,-2.73297222047276,-2.71802590952989,
-2.69561194251482,-2.69209097871679,-2.69080345453194,-2.68993048996875,
-2.68914422690617,-2.68806476187476,-2.68534507673053,-2.66099649518445,
-2.64765672528628,-2.64012478440832,-2.63653375879653,-2.63359968647192,
-2.63191263100535,-2.631881954027,-2.63184891654279,-2.63182858787095,-2.63179966169494,
-2.63175858330605,-2.63155936297703,-2.63004121488427,-2.62804158696779,
-2.62351306993557,-2.59898048444021,-2.58265345838236,-2.57781924489417,
-2.57458923269347,-2.57334426326127,-2.57247977536507,-2.57168487243578,
-2.57057215958468,-2.56763471362048,-2.54949610867631,-2.52920504772647,
-2.5187222996957,-2.51597909259466,-2.51431607421643,-2.51281234893167,
-2.51087871563253,-2.50682852114621,-2.47623740466852,-2.45886160444114,
-2.45669169014394,-2.45563033614326,-2.45487218354769,-2.45390832337159,
-2.45224995217782,-2.44567474974773,-2.43904205359092,-2.40916410391459,
-2.40086988661454,-2.39833029435195,-2.39671176261504,-2.39519400028436,
-2.39319689975507,-2.38868300291224,-2.36406870900622,-2.34778774315513,
-2.34296097751151,-2.33973464471188,-2.33849021145206,-2.33762580945154,
-2.33683075563647,-2.33571752716908,-2.33277616773452,-2.31470907729038,
-2.29436699833418,-2.28386969787479,-2.28112525357769,-2.27946193434801,
-2.27795822519108,-2.27602501577698,-2.27197721992066,-2.24136580158916,
-2.22400435763817,-2.22183480883172,-2.22077350916209,-2.22001534463373,
-2.21905139963574,-2.2173927317497,-2.21081435814262,-2.20418202568458,
-2.17429857455624,-2.16601031918294,-2.1634713120305,-2.16185287700644,
-2.16033501195311,-2.15833749419332,-2.15382141296355,-2.12927870184117,
-2.10835426015475,-2.10493382807543,-2.10366060532023,-2.10279048910964,
-2.10200142775615,-2.1009111982557,-2.09812796403039,-2.07499799568581,
-2.05039910537378,-2.04685190209,-2.04501740115274,-2.0436665820278,-2.04198967101139,
-2.03918329369144,-2.02921902657818,-2.01986711404084),.UNSPECIFIED.);
#1538=B_SPLINE_CURVE_WITH_KNOTS('',3,(#103637,#103638,#103639,#103640,#103641,
#103642,#103643,#103644,#103645,#103646,#103647,#103648,#103649,#103650,
#103651,#103652,#103653,#103654,#103655,#103656,#103657,#103658,#103659,
#103660,#103661,#103662,#103663,#103664,#103665,#103666,#103667,#103668,
#103669,#103670,#103671,#103672,#103673,#103674,#103675,#103676,#103677,
#103678,#103679,#103680,#103681,#103682,#103683,#103684,#103685,#103686,
#103687,#103688,#103689,#103690,#103691,#103692,#103693,#103694,#103695,
#103696,#103697,#103698,#103699,#103700,#103701,#103702,#103703,#103704,
#103705,#103706,#103707,#103708,#103709,#103710,#103711,#103712,#103713,
#103714,#103715,#103716,#103717,#103718,#103719,#103720,#103721,#103722,
#103723,#103724,#103725,#103726,#103727,#103728,#103729,#103730,#103731,
#103732,#103733,#103734,#103735,#103736,#103737,#103738,#103739,#103740,
#103741,#103742,#103743,#103744,#103745,#103746,#103747,#103748,#103749,
#103750,#103751,#103752,#103753,#103754,#103755,#103756,#103757,#103758,
#103759,#103760,#103761,#103762,#103763,#103764,#103765,#103766,#103767,
#103768,#103769,#103770,#103771,#103772,#103773,#103774,#103775,#103776,
#103777,#103778,#103779,#103780,#103781,#103782,#103783,#103784,#103785,
#103786,#103787,#103788,#103789,#103790,#103791,#103792,#103793,#103794,
#103795,#103796,#103797,#103798,#103799,#103800,#103801,#103802,#103803,
#103804,#103805,#103806,#103807,#103808,#103809,#103810,#103811,#103812,
#103813,#103814,#103815,#103816,#103817,#103818,#103819,#103820,#103821,
#103822,#103823,#103824,#103825,#103826,#103827,#103828,#103829,#103830,
#103831,#103832,#103833,#103834,#103835,#103836,#103837,#103838,#103839,
#103840,#103841,#103842),.UNSPECIFIED.,.F.,.F.,(4,2,2,2,2,2,2,2,2,2,2,2,
2,2,2,2,2,2,2,2,2,2,2,2,2,2,2,2,2,2,2,2,2,2,2,2,2,2,2,2,2,2,2,2,2,2,2,2,
2,2,2,2,2,2,2,2,2,2,2,2,2,2,2,2,2,2,2,2,2,2,2,2,2,2,2,2,2,2,2,2,2,2,2,2,
2,2,2,2,2,2,2,2,2,2,2,2,2,2,2,2,2,2,4),(-2.22610704996512,-2.20550128129161,
-2.18810508570363,-2.18593385519407,-2.18487195420598,-2.1841134594657,
-2.18314923262218,-2.18149031312629,-2.17491384539396,-2.16827985191087,
-2.13837887934292,-2.13009701783793,-2.12755806368416,-2.12593922555329,
-2.1244206729256,-2.12242179429114,-2.11790059634646,-2.09350040897706,
-2.07705092748205,-2.07219608325262,-2.06895549397844,-2.06770859199797,
-2.06684343992376,-2.0660483579281,-2.06493610108897,-2.06200560446663,
-2.04355595309435,-2.02348432244987,-2.01306234549602,-2.01032296387726,
-2.00866010635629,-2.00715513115915,-2.00521792529932,-2.00115280592182,
-1.97066490215077,-1.95320548549658,-1.95103219483385,-1.9499697531547,
-1.94921106840316,-1.94824686072143,-1.94658847077552,-1.94002051247477,
-1.93338478398901,-1.9034810789982,-1.89519518906706,-1.89265557121669,
-1.89103642822728,-1.88951767001313,-1.88751863485605,-1.88299756308869,
-1.85858047685114,-1.8421435772716,-1.8372906057663,-1.83405085649242,-1.83280398082922,
-1.83193876343253,-1.83114365292999,-1.83003124939392,-1.82709959948778,
-1.80876320472529,-1.78860697336739,-1.77816086984924,-1.77541960527736,
-1.77375639511096,-1.77225161060185,-1.77031536724202,-1.76625497887861,
-1.73572503766731,-1.71829337251568,-1.71612097124736,-1.71505875868473,
-1.71430012947382,-1.71333582385902,-1.71167704129297,-1.70510458415129,
-1.69846946591539,-1.66856088790109,-1.66028085519697,-1.65774179312133,
-1.65612272761624,-1.65460384775618,-1.6526043682989,-1.64808103411075,
-1.62375393070014,-1.60724954526795,-1.60238561273262,-1.59914038801131,
-1.59789263990009,-1.59702721666021,-1.59623224434579,-1.59512045131583,
-1.5921938729755,-1.57284672147576,-1.55322643404189,-1.54658021882862,
-1.5417822101871,-1.53971306786211,-1.53818853734378,-1.53677400146492,
-1.53483546570562,-1.52989695310677,-1.49640613248406,-1.48414558948818),
 .UNSPECIFIED.);
#1539=B_SPLINE_CURVE_WITH_KNOTS('',3,(#103843,#103844,#103845,#103846,#103847,
#103848,#103849,#103850,#103851,#103852,#103853,#103854,#103855,#103856,
#103857,#103858,#103859,#103860,#103861,#103862,#103863,#103864,#103865,
#103866,#103867,#103868,#103869,#103870,#103871,#103872,#103873,#103874,
#103875,#103876,#103877,#103878,#103879,#103880,#103881,#103882,#103883,
#103884,#103885,#103886,#103887,#103888,#103889,#103890,#103891,#103892,
#103893,#103894,#103895,#103896,#103897,#103898,#103899,#103900,#103901,
#103902,#103903,#103904,#103905,#103906,#103907,#103908,#103909,#103910,
#103911,#103912,#103913,#103914,#103915,#103916,#103917,#103918,#103919,
#103920,#103921,#103922,#103923,#103924,#103925,#103926,#103927,#103928,
#103929,#103930,#103931,#103932,#103933,#103934,#103935,#103936,#103937,
#103938,#103939,#103940,#103941,#103942,#103943,#103944,#103945,#103946,
#103947,#103948,#103949,#103950,#103951,#103952,#103953,#103954,#103955,
#103956,#103957,#103958,#103959,#103960,#103961,#103962,#103963,#103964,
#103965,#103966,#103967,#103968,#103969,#103970,#103971,#103972,#103973,
#103974,#103975,#103976,#103977,#103978,#103979,#103980,#103981,#103982,
#103983,#103984,#103985,#103986,#103987,#103988,#103989,#103990,#103991,
#103992,#103993,#103994,#103995,#103996,#103997,#103998,#103999,#104000,
#104001,#104002,#104003,#104004,#104005,#104006,#104007,#104008,#104009,
#104010,#104011,#104012,#104013,#104014,#104015,#104016,#104017,#104018,
#104019,#104020,#104021,#104022,#104023,#104024,#104025,#104026,#104027,
#104028,#104029,#104030,#104031,#104032,#104033,#104034,#104035,#104036,
#104037,#104038,#104039,#104040,#104041,#104042,#104043,#104044,#104045,
#104046),.UNSPECIFIED.,.F.,.F.,(4,2,2,2,2,2,2,2,2,2,2,2,2,2,2,2,2,2,2,2,
2,2,2,2,2,2,2,2,2,2,2,2,2,2,2,2,2,2,2,2,2,2,2,2,2,2,2,2,2,2,2,2,2,2,2,2,
2,2,2,2,2,2,2,2,2,2,2,2,2,2,2,2,2,2,2,2,2,2,2,2,2,2,2,2,2,2,2,2,2,2,2,2,
2,2,2,2,2,2,2,2,2,4),(-2.01986711404084,-2.00149397536358,-1.98869985377435,
-1.98679560857064,-1.98578840545589,-1.98495050181473,-1.98390199694263,
-1.98225373663555,-1.97347956546237,-1.94390368319916,-1.931772227007,-1.92890662718964,
-1.92721674900399,-1.92571800226443,-1.92383046228648,-1.9208595192094,
-1.90028859243867,-1.87939204285366,-1.87096370576033,-1.86923620077264,
-1.86826683609095,-1.86742513744043,-1.86634386872644,-1.86454754847247,
-1.85198266203283,-1.82226488292153,-1.81375197539902,-1.81118947303606,
-1.80956593526822,-1.80805014172761,-1.80606527759675,-1.80162096948806,
-1.77528345007096,-1.75425352928614,-1.75208531650031,-1.75102428683803,
-1.75026615968043,-1.74930204974309,-1.74764263301021,-1.7410551291592,
-1.73442455992968,-1.70452728965447,-1.69625800657821,-1.69372103577476,
-1.69210305660383,-1.69058502890219,-1.68858643587658,-1.68406412922213,
-1.65976367537816,-1.63862657386854,-1.63519134668002,-1.63391599699051,
-1.63304546003156,-1.63225682721722,-1.63116823537041,-1.6283944876795,
-1.6050159117426,-1.58042201924304,-1.57701317935919,-1.5752071833797,-1.57372800344111,
-1.57198301376457,-1.56894659971462,-1.5554133739678,-1.53056253375716,
-1.51890185659636,-1.51703259176242,-1.5160327895258,-1.51519450479719,
-1.51413725652466,-1.51246011860772,-1.5030928352676,-1.47407727516581,
-1.46202736520136,-1.45916732756614,-1.45747868513583,-1.45597978049687,
-1.4540903588368,-1.45111311843643,-1.42947386717785,-1.40946638269828,
-1.40121265397739,-1.39949510888014,-1.3985279274702,-1.39768589490699,
-1.39660135970672,-1.39479374167545,-1.38096342239752,-1.3469355008027,
-1.34264857626484,-1.34069204048276,-1.33918078914116,-1.33754523156273,
-1.33492714990025,-1.32585541847392,-1.29650904670547,-1.28420692247016,
-1.28242015400097,-1.281341725396,-1.28050039456192,-1.27952928510668,-1.27804052283339),
 .UNSPECIFIED.);
#1540=B_SPLINE_CURVE_WITH_KNOTS('',3,(#104051,#104052,#104053,#104054,#104055,
#104056,#104057,#104058,#104059,#104060,#104061,#104062,#104063,#104064,
#104065,#104066,#104067,#104068,#104069,#104070,#104071,#104072,#104073,
#104074,#104075,#104076,#104077,#104078,#104079,#104080,#104081,#104082,
#104083,#104084,#104085,#104086,#104087,#104088,#104089,#104090,#104091,
#104092,#104093,#104094,#104095,#104096,#104097,#104098,#104099,#104100,
#104101,#104102,#104103,#104104,#104105,#104106,#104107,#104108,#104109,
#104110,#104111,#104112,#104113,#104114,#104115,#104116,#104117,#104118,
#104119,#104120,#104121,#104122,#104123,#104124,#104125,#104126,#104127,
#104128,#104129,#104130,#104131,#104132,#104133,#104134,#104135,#104136,
#104137,#104138,#104139,#104140,#104141,#104142,#104143,#104144,#104145,
#104146,#104147,#104148,#104149,#104150,#104151,#104152,#104153,#104154,
#104155,#104156,#104157,#104158,#104159,#104160,#104161,#104162,#104163,
#104164,#104165,#104166,#104167,#104168,#104169,#104170,#104171,#104172,
#104173,#104174,#104175,#104176,#104177,#104178,#104179,#104180,#104181,
#104182,#104183,#104184,#104185,#104186,#104187,#104188,#104189,#104190,
#104191,#104192,#104193,#104194,#104195,#104196,#104197,#104198,#104199,
#104200,#104201,#104202,#104203,#104204,#104205,#104206,#104207,#104208,
#104209,#104210,#104211,#104212,#104213,#104214,#104215,#104216,#104217,
#104218,#104219,#104220,#104221,#104222,#104223,#104224,#104225,#104226,
#104227,#104228,#104229,#104230,#104231,#104232,#104233,#104234,#104235,
#104236,#104237,#104238,#104239,#104240,#104241,#104242,#104243,#104244,
#104245,#104246,#104247,#104248,#104249,#104250,#104251,#104252,#104253,
#104254,#104255,#104256,#104257,#104258,#104259,#104260,#104261,#104262,
#104263,#104264,#104265,#104266,#104267,#104268,#104269,#104270,#104271,
#104272,#104273,#104274,#104275,#104276,#104277,#104278,#104279,#104280,
#104281,#104282,#104283,#104284,#104285,#104286,#104287,#104288,#104289,
#104290,#104291,#104292,#104293,#104294,#104295,#104296,#104297,#104298,
#104299,#104300,#104301,#104302,#104303,#104304,#104305,#104306,#104307,
#104308),.UNSPECIFIED.,.F.,.F.,(4,2,2,2,2,2,2,2,2,2,2,2,2,2,2,2,2,2,2,2,
2,2,2,2,2,2,2,2,2,2,2,2,2,2,2,2,2,2,2,2,2,2,2,2,2,2,2,2,2,2,2,2,2,2,2,2,
2,2,2,2,2,2,2,2,2,2,2,2,2,2,2,2,2,2,2,2,2,2,2,2,2,2,2,2,2,2,2,2,2,2,2,2,
2,2,2,2,2,2,2,2,2,2,2,2,2,2,2,2,2,2,2,2,2,2,2,2,2,2,2,2,2,2,2,2,2,2,2,2,
4),(-2.96786886973577,-2.95785689286692,-2.95264959365992,-2.95073047369495,
-2.94925312079407,-2.94780454720857,-2.94616584058611,-2.94356098609388,
-2.93557638518036,-2.92530150922596,-2.9068384860444,-2.89433462089359,
-2.89111690778034,-2.88987259097804,-2.88900761898966,-2.88821639909733,
-2.88710809866277,-2.88417945460901,-2.86600747968086,-2.85036799118396,
-2.84068417438163,-2.83642136520946,-2.83306116457156,-2.83128235898923,
-2.83127130736516,-2.8312594227592,-2.83124664029677,-2.83123288978141,
-2.8312180952081,-2.83120217426603,-2.83118503776084,-2.83116658901647,
-2.83114672319152,-2.83112532657952,-2.83110227579331,-2.83107743693406,
-2.83105066467395,-2.83102180126969,-2.83099067553294,-2.83095710172708,
-2.83093194337139,-2.82944293157537,-2.82756454275732,-2.82460236990099,
-2.80196387274249,-2.7857332191819,-2.77468013966401,-2.77284194225298,
-2.77185340971376,-2.77101691528075,-2.76995515792267,-2.76826449997813,
-2.7586911368712,-2.74931880536028,-2.72832012133503,-2.72125262823238,
-2.7162217528034,-2.71411045653806,-2.712575689053,-2.71116608450099,-2.70925639360369,
-2.70548691941654,-2.67619614302823,-2.65797111011836,-2.65577156006441,
-2.65470130444696,-2.65393971134428,-2.6529761248051,-2.65132366454225,
-2.64484129353594,-2.63819073566558,-2.60824849336731,-2.59995769599317,
-2.59741701683377,-2.59579724938962,-2.5942779343384,-2.59227820398957,
-2.58775572281516,-2.56323072573548,-2.54684035798431,-2.54199438052968,
-2.53875813527581,-2.53751200405902,-2.53664717544212,-2.53585278187051,
-2.53474128661837,-2.53181180038879,-2.51337984726407,-2.49329180933647,
-2.48286693582478,-2.48012920001551,-2.47846785795519,-2.47696460859289,
-2.47503014860834,-2.47097292860631,-2.44040951498069,-2.42298648807979,
-2.42081582996354,-2.4197546644234,-2.41899656122737,-2.41803236896773,
-2.41637418906627,-2.40980941399887,-2.40317347318246,-2.37328077728257,
-2.36497910619027,-2.36243722704195,-2.36081719109884,-2.359297970103,-2.35729885772379,
-2.35277983584678,-2.32835023538045,-2.31194752112263,-2.30710001751538,
-2.30386268964697,-2.30261571795862,-2.30175013030088,-2.30095472900709,
-2.29984148358813,-2.29690432031969,-2.2787402395881,-2.25846564675014,
-2.24798655600512,-2.24524264317062,-2.24357887092661,-2.24207424813948,
-2.24013915151677,-2.2360846967586,-2.22610704996512),.UNSPECIFIED.);
#1541=B_SPLINE_CURVE_WITH_KNOTS('',3,(#104309,#104310,#104311,#104312,#104313,
#104314,#104315,#104316,#104317,#104318,#104319,#104320,#104321,#104322,
#104323,#104324,#104325,#104326,#104327,#104328,#104329,#104330,#104331,
#104332,#104333,#104334,#104335,#104336,#104337,#104338,#104339,#104340,
#104341,#104342,#104343,#104344,#104345,#104346,#104347,#104348,#104349,
#104350,#104351,#104352,#104353,#104354,#104355,#104356,#104357,#104358,
#104359,#104360,#104361,#104362,#104363,#104364,#104365,#104366,#104367,
#104368,#104369,#104370,#104371,#104372,#104373,#104374,#104375,#104376,
#104377,#104378,#104379,#104380,#104381,#104382,#104383,#104384,#104385,
#104386,#104387,#104388,#104389,#104390,#104391,#104392,#104393,#104394,
#104395,#104396,#104397,#104398,#104399,#104400,#104401,#104402,#104403,
#104404,#104405,#104406,#104407,#104408,#104409,#104410,#104411,#104412,
#104413,#104414,#104415,#104416,#104417,#104418,#104419,#104420,#104421,
#104422,#104423,#104424,#104425,#104426,#104427,#104428,#104429,#104430,
#104431,#104432,#104433,#104434,#104435,#104436,#104437,#104438,#104439,
#104440,#104441,#104442,#104443,#104444,#104445,#104446,#104447,#104448,
#104449,#104450,#104451,#104452,#104453,#104454,#104455,#104456,#104457,
#104458,#104459,#104460,#104461,#104462,#104463,#104464,#104465,#104466,
#104467,#104468,#104469,#104470,#104471,#104472,#104473,#104474,#104475,
#104476,#104477,#104478,#104479,#104480,#104481,#104482,#104483,#104484,
#104485,#104486,#104487,#104488,#104489,#104490,#104491,#104492,#104493,
#104494,#104495,#104496,#104497,#104498,#104499,#104500,#104501,#104502,
#104503,#104504,#104505,#104506,#104507,#104508,#104509,#104510,#104511,
#104512),.UNSPECIFIED.,.F.,.F.,(4,2,2,2,2,2,2,2,2,2,2,2,2,2,2,2,2,2,2,2,
2,2,2,2,2,2,2,2,2,2,2,2,2,2,2,2,2,2,2,2,2,2,2,2,2,2,2,2,2,2,2,2,2,2,2,2,
2,2,2,2,2,2,2,2,2,2,2,2,2,2,2,2,2,2,2,2,2,2,2,2,2,2,2,2,2,2,2,2,2,2,2,2,
2,2,2,2,2,2,2,2,2,4),(-1.27804052283339,-1.27779354277622,-1.26921374673466,
-1.24615215792371,-1.22788586669804,-1.22494349880741,-1.22306464005362,
-1.22156677634983,-1.21987148606874,-1.216980855906,-1.2044692630371,-1.17179253262613,
-1.16609567259652,-1.16449858396085,-1.16355779691929,-1.16270930512896,
-1.16155756344434,-1.15890186298369,-1.14675613267963,-1.11317457280965,
-1.10821231914223,-1.10627046533854,-1.10485553976076,-1.10333251025302,
-1.10126883004227,-1.0964992625634,-1.0899029086718,-1.07054709728567,-1.05082231426154,
-1.04789966097991,-1.0467887373645,-1.04599425310984,-1.04512934652003,
-1.04388215912375,-1.04063724818695,-1.03577359860831,-1.01926373765555,
-0.994973588639409,-0.990452015073592,-0.988453645411723,-0.986935746151702,
-0.98531786759116,-0.982780987090211,-0.97451173681847,-0.944599183842762,
-0.93795899266781,-0.931367779478571,-0.929708083375804,-0.928743947946152,
-0.927985862467296,-0.926925008439456,-0.92475761153208,-0.904022419282702,
-0.877374135679222,-0.872946620414565,-0.870964609558215,-0.869449144542359,
-0.867824159097486,-0.865255539558594,-0.856685125800273,-0.826982297168291,
-0.814445536666213,-0.812649941824788,-0.81156873662837,-0.810726698109774,
-0.809756282500682,-0.808026064681788,-0.799564003474529,-0.777217344170429,
-0.75815764559839,-0.75519983006914,-0.753315710445747,-0.751816555244499,
-0.750122884427466,-0.747242613863021,-0.734907977080816,-0.703832967923239,
-0.696571717166207,-0.694859865863391,-0.693883548589329,-0.693051219494492,
-0.691967310301918,-0.68967873316349,-0.686603634471189,-0.678748581179012,
-0.654039356211465,-0.640316839892049,-0.637271899617777,-0.635525726446294,
-0.634047723181845,-0.632245863591957,-0.628853210844796,-0.603977633476396,
-0.580825564669791,-0.578041993013366,-0.576952021167913,-0.576163327927914,
-0.575293368524894,-0.574020841920639,-0.570605445405218,-0.54976549363765,
-0.536166236652312),.UNSPECIFIED.);
#1542=B_SPLINE_CURVE_WITH_KNOTS('',3,(#104515,#104516,#104517,#104518,#104519,
#104520,#104521,#104522,#104523,#104524,#104525,#104526,#104527,#104528,
#104529,#104530,#104531,#104532,#104533,#104534,#104535,#104536,#104537,
#104538,#104539,#104540,#104541,#104542,#104543,#104544,#104545,#104546,
#104547,#104548,#104549,#104550,#104551,#104552,#104553,#104554,#104555,
#104556,#104557,#104558,#104559,#104560,#104561,#104562,#104563,#104564,
#104565,#104566,#104567,#104568,#104569,#104570,#104571,#104572,#104573,
#104574,#104575,#104576,#104577,#104578,#104579,#104580,#104581,#104582,
#104583,#104584,#104585,#104586,#104587,#104588,#104589,#104590,#104591,
#104592,#104593,#104594,#104595,#104596,#104597,#104598,#104599,#104600,
#104601,#104602,#104603,#104604,#104605,#104606,#104607,#104608,#104609,
#104610,#104611,#104612,#104613,#104614,#104615,#104616,#104617,#104618,
#104619,#104620,#104621,#104622,#104623,#104624,#104625,#104626,#104627,
#104628,#104629,#104630,#104631,#104632,#104633,#104634,#104635,#104636,
#104637,#104638,#104639,#104640,#104641,#104642,#104643,#104644,#104645,
#104646,#104647,#104648,#104649,#104650,#104651,#104652,#104653,#104654,
#104655,#104656,#104657,#104658,#104659,#104660,#104661,#104662,#104663,
#104664,#104665,#104666,#104667,#104668,#104669,#104670,#104671,#104672,
#104673,#104674,#104675,#104676,#104677,#104678,#104679,#104680,#104681,
#104682,#104683,#104684,#104685,#104686,#104687,#104688,#104689,#104690,
#104691,#104692,#104693,#104694,#104695,#104696,#104697,#104698,#104699,
#104700),.UNSPECIFIED.,.F.,.F.,(4,2,2,2,2,2,2,2,2,2,2,2,2,2,2,2,2,2,2,2,
2,2,2,2,2,2,2,2,2,2,2,2,2,2,2,2,2,2,2,2,2,2,2,2,2,2,2,2,2,2,2,2,2,2,2,2,
2,2,2,2,2,2,2,2,2,2,2,2,2,2,2,2,2,2,2,2,2,2,2,2,2,2,2,2,2,2,2,2,2,2,2,2,
4),(-0.536166236652312,-0.525085231207484,-0.520567953445079,-0.518569339787368,
-0.517050414425168,-0.515430627671845,-0.512889021249871,-0.50458736279753,
-0.474640089736819,-0.467979450327641,-0.461490579047531,-0.45983767900236,
-0.458874081698197,-0.458112632188542,-0.457042813646653,-0.454845013004687,
-0.436674870711717,-0.407327856661352,-0.403149927900042,-0.401209844509549,
-0.399697243559294,-0.398045997313867,-0.395371015272676,-0.385744469389427,
-0.35558106721775,-0.353180361775628,-0.344415240389566,-0.34276649532011,
-0.341717457261505,-0.340881832016273,-0.339882944566339,-0.337995666679841,
-0.325443190434005,-0.298765263304739,-0.287485936178323,-0.284611116821944,
-0.282909955162882,-0.281424291679214,-0.279583588819669,-0.275969299581762,
-0.254886236187246,-0.232378153060786,-0.226389972304301,-0.224770081822884,
-0.223827553192379,-0.222981410989253,-0.221843094348616,-0.219268692304207,
-0.200653577221383,-0.172015795769246,-0.167701309523609,-0.165733192751794,
-0.164213322150942,-0.162568691223491,-0.159936410440464,-0.150810104984887,
-0.121120135557507,-0.109405628083183,-0.107622248750493,-0.106526986897927,
-0.105692523569586,-0.105682773912662,-0.105673291143312,-0.105664064451981,
-0.105655083595332,-0.10564633887878,-0.105637821094948,-0.105629521513252,
-0.105621431843887,-0.105613544210896,-0.105605851112159,-0.105598345430928,
-0.105591020376947,-0.1055838694892,-0.105576886620684,-0.105570065905969,
-0.105563401742921,-0.105556888777833,-0.10555052191761,-0.105544296282815,
-0.104496551007015,-0.103346651016605,-0.101479563606578,-0.0892256042285175,
-0.0570429508974814,-0.0522112497001512,-0.0502726622426464,-0.0488425185149138,
-0.0472858284284697,-0.0451445915942411,-0.0400400193764259,-0.0328700432185351,
-1.00000014535695E-6),.UNSPECIFIED.);
#1543=B_SPLINE_CURVE_WITH_KNOTS('',3,(#104704,#104705,#104706,#104707,#104708,
#104709,#104710,#104711,#104712,#104713,#104714,#104715,#104716,#104717,
#104718,#104719,#104720,#104721,#104722,#104723,#104724,#104725,#104726,
#104727,#104728,#104729,#104730,#104731,#104732,#104733,#104734,#104735,
#104736,#104737,#104738,#104739,#104740,#104741,#104742,#104743,#104744,
#104745,#104746,#104747,#104748,#104749,#104750,#104751,#104752,#104753,
#104754,#104755,#104756,#104757,#104758,#104759,#104760,#104761,#104762,
#104763,#104764,#104765),.UNSPECIFIED.,.F.,.F.,(4,2,2,2,2,2,2,2,2,2,2,2,
2,2,2,2,2,2,2,2,2,2,2,2,2,2,2,2,2,2,4),(5.26465888469903E-5,0.00458003943048162,
0.0076256166217089,0.00923307394815808,0.0105570311839449,0.0118209960109234,
0.0134523997639754,0.0162830945574481,0.0250310363928198,0.0569680207680776,
0.0667585963604424,0.0684856004228339,0.0694262516517115,0.070257611045996,
0.0713168672239314,0.0730035599451736,0.0824114043194782,0.0932430412621605,
0.108440124136716,0.127405659390686,0.130614876340645,0.132680842693845,
0.134340156702719,0.13623440842581,0.139517071288727,0.155909768338738,
0.176205334305,0.183267029437581,0.185053305917431,0.185861120043884,0.186559797993667),
 .UNSPECIFIED.);
#1544=B_SPLINE_CURVE_WITH_KNOTS('',3,(#104766,#104767,#104768,#104769,#104770,
#104771,#104772,#104773,#104774,#104775,#104776,#104777,#104778,#104779,
#104780,#104781,#104782,#104783,#104784,#104785,#104786,#104787,#104788,
#104789,#104790,#104791,#104792,#104793,#104794,#104795,#104796,#104797,
#104798,#104799,#104800,#104801,#104802,#104803,#104804,#104805,#104806,
#104807,#104808,#104809,#104810,#104811,#104812,#104813,#104814,#104815,
#104816,#104817,#104818,#104819,#104820,#104821,#104822,#104823,#104824,
#104825,#104826,#104827,#104828,#104829,#104830,#104831,#104832),
 .UNSPECIFIED.,.F.,.F.,(4,3,3,3,3,3,3,3,3,3,3,3,3,3,3,3,3,3,3,3,3,3,4),
(152.205784650184,152.32550641777,152.44545518428,152.532661347998,152.532706586939,
152.643528857141,152.657043371795,152.776764042929,152.896367880645,153.015907297727,
153.135434595286,153.255084298657,153.374807527798,153.485184154958,153.494746688451,
153.52734741509,153.527400865785,153.641271566567,153.658393831217,153.780909296427,
153.788925130557,153.918783873189,153.938039816989),.UNSPECIFIED.);
#1545=B_SPLINE_CURVE_WITH_KNOTS('',3,(#104835,#104836,#104837,#104838,#104839,
#104840,#104841,#104842,#104843,#104844,#104845,#104846,#104847,#104848,
#104849,#104850,#104851,#104852,#104853,#104854,#104855,#104856,#104857,
#104858,#104859,#104860,#104861,#104862,#104863,#104864,#104865,#104866,
#104867,#104868,#104869,#104870,#104871,#104872,#104873,#104874,#104875,
#104876,#104877,#104878,#104879,#104880,#104881,#104882,#104883,#104884,
#104885,#104886,#104887,#104888,#104889,#104890,#104891,#104892,#104893,
#104894,#104895,#104896,#104897,#104898,#104899,#104900,#104901,#104902,
#104903,#104904,#104905,#104906,#104907,#104908,#104909,#104910,#104911,
#104912,#104913,#104914,#104915,#104916,#104917,#104918,#104919,#104920,
#104921,#104922,#104923,#104924,#104925,#104926,#104927,#104928,#104929,
#104930,#104931,#104932,#104933,#104934,#104935,#104936,#104937,#104938,
#104939,#104940,#104941,#104942,#104943,#104944,#104945,#104946,#104947,
#104948,#104949,#104950,#104951,#104952,#104953,#104954,#104955,#104956,
#104957,#104958,#104959,#104960,#104961,#104962,#104963,#104964,#104965,
#104966,#104967,#104968,#104969,#104970,#104971,#104972,#104973,#104974,
#104975,#104976,#104977,#104978,#104979,#104980,#104981,#104982,#104983,
#104984,#104985,#104986,#104987,#104988,#104989,#104990,#104991,#104992,
#104993,#104994,#104995,#104996,#104997,#104998,#104999,#105000,#105001,
#105002,#105003,#105004,#105005,#105006,#105007,#105008,#105009,#105010,
#105011,#105012,#105013,#105014,#105015,#105016,#105017,#105018,#105019,
#105020,#105021,#105022,#105023,#105024,#105025,#105026,#105027,#105028,
#105029,#105030,#105031,#105032,#105033,#105034,#105035,#105036,#105037,
#105038,#105039,#105040,#105041,#105042,#105043,#105044,#105045,#105046,
#105047,#105048,#105049,#105050,#105051,#105052,#105053,#105054,#105055,
#105056,#105057,#105058,#105059,#105060,#105061,#105062,#105063,#105064,
#105065,#105066,#105067,#105068,#105069,#105070),.UNSPECIFIED.,.F.,.F.,
(4,2,2,2,2,2,2,2,2,2,2,2,2,2,2,2,2,2,2,2,2,2,2,2,2,2,2,2,2,2,2,2,2,2,2,
2,2,2,2,2,2,2,2,2,2,2,2,2,2,2,2,2,2,2,2,2,2,2,2,2,2,2,2,2,2,2,2,2,2,2,2,
2,2,2,2,2,2,2,2,2,2,2,2,2,2,2,2,2,2,2,2,2,2,2,2,2,2,2,2,2,2,2,2,2,2,2,2,
2,2,2,2,2,2,2,2,2,2,4),(2.76458849571582,2.80165031556903,2.80595712423809,
2.8181262917974,2.82112649950848,2.82286401352687,2.82435549965188,2.82616746780645,
2.82959813973857,2.85416452357968,2.87456953748744,2.89265855727155,2.89482601013189,
2.89588753031213,2.89672429239254,2.89770372228433,2.8994747521816,2.90838575829188,
2.94946550338247,2.9516209106145,2.96397553243166,2.96699344821178,2.9687363529125,
2.97021529852142,2.97201954171125,2.97540679408675,2.99806263722299,3.02401248261017,
3.02862601575098,3.03885070485117,3.0406018817737,3.04168340260912,3.04252425522643,
3.04349603569766,3.04521969053163,3.05324472628385,3.07119368038886,3.10633505437255,
3.1112796202855,3.11322598453512,3.11464450555406,3.11616939096845,3.11822793146341,
3.12291942592611,3.14573582176358,3.17035133284012,3.17310849693219,3.1744523527326,
3.18446830513651,3.1862082673416,3.18728583679269,3.18812242788805,3.18908309561103,
3.19079023058684,3.19878265630355,3.21664964225608,3.25246155588452,3.25739226988589,
3.25932556685361,3.26073174056842,3.26224058479881,3.26427241708641,3.26887974521027,
3.28841684839569,3.3170693627333,3.33025295232948,3.33228961748616,3.33333508681242,
3.33416930774878,3.33515763893095,3.33696674428531,3.34656811712221,3.36999616002673,
3.4008104752932,3.40401526821518,3.40595966462003,3.40747501930742,3.40912562733698,
3.41178380794678,3.42096569239179,3.45233426059145,3.47599010303093,3.47810992632144,
3.47917377086082,3.48000984894567,3.48001546626198,3.48002082261248,3.48002593163293,
3.48003139267474,3.48003679562201,3.48004214154125,3.48004743145613,3.48005266638362,
3.48005784732583,3.48006297525967,3.48006805113035,3.48007307586283,3.48007805034535,
3.48008297548347,3.48008785213301,3.48009268113104,3.48009746332489,3.48010219951981,
3.48010689050661,3.48011153705322,3.4811186179993,3.48300274687985,3.49345177287389,
3.5237989557689,3.54465138515542,3.54780944427495,3.5497724456426,3.55130081457342,
3.55299013295557,3.55576687338473,3.56598343040685,3.58447765124171,3.61301883334127),
 .UNSPECIFIED.);
#1546=B_SPLINE_CURVE_WITH_KNOTS('',3,(#105073,#105074,#105075,#105076,#105077,
#105078,#105079,#105080,#105081,#105082,#105083,#105084,#105085,#105086,
#105087,#105088,#105089,#105090,#105091,#105092,#105093,#105094,#105095,
#105096,#105097,#105098,#105099,#105100,#105101,#105102,#105103,#105104,
#105105,#105106,#105107,#105108,#105109,#105110,#105111,#105112,#105113,
#105114,#105115,#105116,#105117,#105118,#105119,#105120,#105121,#105122,
#105123,#105124,#105125,#105126,#105127,#105128,#105129,#105130,#105131,
#105132,#105133,#105134,#105135,#105136,#105137,#105138,#105139,#105140,
#105141,#105142,#105143,#105144,#105145,#105146,#105147,#105148,#105149,
#105150,#105151,#105152,#105153,#105154,#105155,#105156,#105157,#105158,
#105159,#105160,#105161,#105162,#105163,#105164,#105165,#105166,#105167,
#105168,#105169,#105170,#105171,#105172,#105173,#105174,#105175,#105176,
#105177,#105178,#105179,#105180,#105181,#105182,#105183,#105184,#105185,
#105186,#105187,#105188,#105189,#105190,#105191,#105192,#105193,#105194,
#105195,#105196,#105197,#105198,#105199,#105200,#105201,#105202,#105203,
#105204,#105205,#105206,#105207,#105208,#105209,#105210,#105211,#105212,
#105213,#105214,#105215,#105216,#105217,#105218,#105219,#105220,#105221,
#105222,#105223,#105224,#105225,#105226,#105227,#105228,#105229,#105230,
#105231,#105232,#105233,#105234,#105235,#105236,#105237,#105238),
 .UNSPECIFIED.,.F.,.F.,(4,2,2,2,2,2,2,2,2,2,2,2,2,2,2,2,2,2,2,2,2,2,2,2,
2,2,2,2,2,2,2,2,2,2,2,2,2,2,2,2,2,2,2,2,2,2,2,2,2,2,2,2,2,2,2,2,2,2,2,2,
2,2,2,2,2,2,2,2,2,2,2,2,2,2,2,2,2,2,2,2,2,2,4),(5.82345211094344E-5,0.000962432406826108,
0.00218339026927038,0.00510626843170436,0.0281859504736574,0.0497092541387239,
0.060399779900796,0.0633865947713838,0.0652320784528269,0.0669226723266856,
0.0690892029088175,0.0726575785754937,0.104139277570954,0.122704290035139,
0.135602756706391,0.142206590267457,0.143830243929883,0.144790296601867,
0.145627621028536,0.146681926730478,0.148420489755403,0.159598768885037,
0.18798784120411,0.204078066656765,0.210131112885388,0.214581945054722,
0.216530737681881,0.2179716028151,0.219309491332927,0.221140566504419,0.225761634791897,
0.266437087089506,0.282474900800036,0.289912929596359,0.29152368223493,
0.292445971682925,0.293281597898723,0.294357453789363,0.296517608898025,
0.317067504076477,0.347312668885674,0.360861187175288,0.363894074149783,
0.365640323176316,0.367160809205848,0.369035709233282,0.371902596480564,
0.385693878110236,0.422840046100618,0.434096470386929,0.436016443818509,
0.437045950207626,0.437901058644632,0.438953352297794,0.440973129135816,
0.453050999205782,0.483038601769635,0.502247186452089,0.506834410277817,
0.508878002902064,0.510403932807444,0.51183215535006,0.513805602569262,
0.518894269422453,0.552635318881072,0.578948090231822,0.58163614276351,
0.582796255349648,0.583645611773807,0.5845655425837,0.586081192551398,0.590996599683048,
0.622400966429067,0.641278273758192,0.651556558477386,0.654297564592166,
0.655954021965353,0.657445163551626,0.659349476773255,0.662389166147018,
0.680299895717508,0.712120523626618,0.717606620371918),.UNSPECIFIED.);
#1547=B_SPLINE_CURVE_WITH_KNOTS('',3,(#105243,#105244,#105245,#105246,#105247,
#105248,#105249,#105250,#105251,#105252,#105253,#105254,#105255,#105256,
#105257,#105258,#105259,#105260,#105261,#105262,#105263,#105264,#105265,
#105266,#105267,#105268,#105269,#105270,#105271,#105272,#105273,#105274,
#105275,#105276,#105277,#105278,#105279,#105280,#105281,#105282,#105283,
#105284,#105285,#105286,#105287,#105288,#105289,#105290,#105291,#105292,
#105293,#105294,#105295,#105296,#105297,#105298,#105299,#105300,#105301,
#105302,#105303,#105304,#105305,#105306,#105307,#105308,#105309,#105310,
#105311,#105312,#105313,#105314,#105315,#105316,#105317,#105318,#105319,
#105320,#105321),.UNSPECIFIED.,.F.,.F.,(4,3,3,3,3,3,3,3,3,3,3,3,3,3,3,3,
3,3,3,3,3,3,3,3,3,3,4),(-0.272803646496736,-0.263130204428988,-0.245860818959094,
-0.239585991691747,-0.234115749182603,-0.216916546212463,-0.205423868019635,
-0.200353055275459,-0.196895211330308,-0.180142741104203,-0.163804796575999,
-0.154097377599458,-0.147221560984452,-0.144240702043143,-0.128386580298794,
-0.124975120669838,-0.108765198492335,-0.0956970463056653,-0.0926130492690722,
-0.0768457730014618,-0.0611559826881288,-0.053296886616634,-0.0475073198824726,
-0.0447089256306213,-0.0296007544670048,-0.0148003772335024,0.),
 .UNSPECIFIED.);
#1548=B_SPLINE_CURVE_WITH_KNOTS('',3,(#105322,#105323,#105324,#105325,#105326,
#105327,#105328,#105329,#105330,#105331,#105332,#105333,#105334,#105335),
 .UNSPECIFIED.,.F.,.F.,(4,2,2,2,2,2,4),(1.00000221648494E-6,0.0490633756002225,
0.10485433700254,0.159887956090769,0.216674600864298,0.269192125233152,
0.323332368022587),.UNSPECIFIED.);
#1549=B_SPLINE_CURVE_WITH_KNOTS('',3,(#105941,#105942,#105943,#105944,#105945,
#105946),.UNSPECIFIED.,.F.,.F.,(4,2,4),(8.69075182808115E-5,0.00135534780982827,
0.00262696644863166),.UNSPECIFIED.);
#1550=B_SPLINE_CURVE_WITH_KNOTS('',3,(#105947,#105948,#105949,#105950,#105951,
#105952,#105953,#105954,#105955,#105956,#105957,#105958,#105959,#105960),
 .UNSPECIFIED.,.F.,.F.,(4,2,2,2,2,2,4),(4.19423088180546E-5,0.0458823493220878,
0.0903849398187459,0.138485347324558,0.185100854943403,0.232357774450867,
0.273915327518736),.UNSPECIFIED.);
#1551=B_SPLINE_CURVE_WITH_KNOTS('',3,(#105965,#105966,#105967,#105968,#105969,
#105970,#105971,#105972,#105973,#105974,#105975,#105976,#105977,#105978,
#105979,#105980,#105981,#105982,#105983,#105984,#105985,#105986,#105987,
#105988,#105989,#105990,#105991,#105992,#105993,#105994,#105995,#105996,
#105997,#105998,#105999,#106000,#106001,#106002,#106003,#106004,#106005,
#106006,#106007,#106008,#106009,#106010,#106011,#106012,#106013,#106014,
#106015,#106016,#106017,#106018,#106019,#106020,#106021,#106022,#106023,
#106024,#106025,#106026,#106027,#106028,#106029,#106030,#106031,#106032,
#106033,#106034,#106035,#106036,#106037,#106038,#106039,#106040,#106041,
#106042,#106043),.UNSPECIFIED.,.F.,.F.,(4,3,3,3,3,3,3,3,3,3,3,3,3,3,3,3,
3,3,3,3,3,3,3,3,3,3,4),(-0.272803579328725,-0.263130204428921,-0.245860818959034,
-0.239089121769124,-0.233709153701305,-0.216514195238077,-0.200353057339568,
-0.196895211887197,-0.180150634784372,-0.163785286417538,-0.1543299497365,
-0.148620089158273,-0.143731840392854,-0.128386591850485,-0.124975120669821,
-0.108729756337865,-0.101103756501427,-0.0956970454135588,-0.092613048702616,
-0.0768309346477273,-0.0612146988449913,-0.0532968855853477,-0.0475073169611359,
-0.044708922933863,-0.029600746467927,-0.0148003732339635,0.),
 .UNSPECIFIED.);
#1552=B_SPLINE_CURVE_WITH_KNOTS('',3,(#106649,#106650,#106651,#106652,#106653,
#106654),.UNSPECIFIED.,.F.,.F.,(4,2,4),(-0.00257291209214509,-0.00129181487758483,
-1.00000002428626E-6),.UNSPECIFIED.);
#1723=SHAPE_REPRESENTATION_RELATIONSHIP('SRR','None',#135347,#1736);
#1736=ADVANCED_BREP_SHAPE_REPRESENTATION('',(#1762),#135279);
#1749=STYLED_ITEM('',(#135421),#1762);
#1762=MANIFOLD_SOLID_BREP('Body1',#32085);
#1890=CYLINDRICAL_SURFACE('',#33556,1.4635);
#1891=CYLINDRICAL_SURFACE('',#33558,1.4635);
#1892=CYLINDRICAL_SURFACE('',#33559,1.4635);
#1893=CYLINDRICAL_SURFACE('',#33560,1.4635);
#1894=CYLINDRICAL_SURFACE('',#33561,1.4635);
#1895=CYLINDRICAL_SURFACE('',#33562,1.4635);
#1896=CYLINDRICAL_SURFACE('',#33563,1.4635);
#1897=CYLINDRICAL_SURFACE('',#33564,1.4635);
#1898=CYLINDRICAL_SURFACE('',#33565,1.4635);
#1899=CYLINDRICAL_SURFACE('',#33566,1.4635);
#1900=CYLINDRICAL_SURFACE('',#33567,1.4635);
#1901=CYLINDRICAL_SURFACE('',#33568,1.4635);
#1902=CYLINDRICAL_SURFACE('',#33569,1.4635);
#1903=CYLINDRICAL_SURFACE('',#33570,1.4635);
#1904=CYLINDRICAL_SURFACE('',#33571,1.4635);
#1905=CYLINDRICAL_SURFACE('',#33572,1.4635);
#1906=CYLINDRICAL_SURFACE('',#33573,1.4635);
#1907=CYLINDRICAL_SURFACE('',#33574,1.4635);
#1908=CYLINDRICAL_SURFACE('',#33575,1.4635);
#1909=CYLINDRICAL_SURFACE('',#33576,1.4635);
#1910=CYLINDRICAL_SURFACE('',#33577,1.4635);
#1911=CYLINDRICAL_SURFACE('',#33578,1.4635);
#1912=CYLINDRICAL_SURFACE('',#33579,1.4635);
#1913=CYLINDRICAL_SURFACE('',#33580,1.17775);
#1914=CYLINDRICAL_SURFACE('',#33582,1.17775);
#1915=CYLINDRICAL_SURFACE('',#33583,1.17775);
#1916=CYLINDRICAL_SURFACE('',#33584,1.17775);
#1917=CYLINDRICAL_SURFACE('',#33585,1.17775);
#1918=CYLINDRICAL_SURFACE('',#33586,1.17775);
#1919=CYLINDRICAL_SURFACE('',#33587,1.17775);
#1920=CYLINDRICAL_SURFACE('',#33588,1.17775);
#1921=CYLINDRICAL_SURFACE('',#33589,1.17775);
#1922=CYLINDRICAL_SURFACE('',#33590,1.17775);
#1923=CYLINDRICAL_SURFACE('',#33591,1.17775);
#1924=CYLINDRICAL_SURFACE('',#33592,1.17775);
#1925=CYLINDRICAL_SURFACE('',#33593,1.17775);
#1926=CYLINDRICAL_SURFACE('',#33594,1.17775);
#1927=CYLINDRICAL_SURFACE('',#33595,1.17775);
#1928=CYLINDRICAL_SURFACE('',#33596,1.17775);
#1929=CYLINDRICAL_SURFACE('',#33597,1.17775);
#1930=CYLINDRICAL_SURFACE('',#33598,1.17775);
#1931=CYLINDRICAL_SURFACE('',#33599,1.17775);
#1932=CYLINDRICAL_SURFACE('',#33600,1.17775);
#1933=CYLINDRICAL_SURFACE('',#33601,1.17775);
#1934=CYLINDRICAL_SURFACE('',#33602,1.17775);
#1935=CYLINDRICAL_SURFACE('',#33603,1.17775);
#1936=CYLINDRICAL_SURFACE('',#33604,1.17775);
#1937=CYLINDRICAL_SURFACE('',#33606,1.4635);
#1938=CYLINDRICAL_SURFACE('',#33626,2.75);
#1939=CYLINDRICAL_SURFACE('',#33819,1.39337567297406);
#1940=CYLINDRICAL_SURFACE('',#33821,1.39337567297406);
#1941=CYLINDRICAL_SURFACE('',#33823,1.39337567297406);
#1942=CYLINDRICAL_SURFACE('',#33825,1.39337567297406);
#1943=CYLINDRICAL_SURFACE('',#33827,1.39337567297406);
#1944=CYLINDRICAL_SURFACE('',#33829,1.39337567297406);
#2227=FACE_BOUND('',#6701,.T.);
#2228=FACE_BOUND('',#6816,.T.);
#3076=PLANE('',#33608);
#3077=PLANE('',#33611);
#3078=PLANE('',#33617);
#3079=PLANE('',#33621);
#3080=PLANE('',#33622);
#3081=PLANE('',#33624);
#3082=PLANE('',#33625);
#3083=PLANE('',#33701);
#3084=PLANE('',#33702);
#3085=PLANE('',#33703);
#3086=PLANE('',#33706);
#3087=PLANE('',#33707);
#3088=PLANE('',#33708);
#3089=PLANE('',#33709);
#3090=PLANE('',#33710);
#3091=PLANE('',#33711);
#3092=PLANE('',#33712);
#3093=PLANE('',#33713);
#3094=PLANE('',#33714);
#3095=PLANE('',#33715);
#3096=PLANE('',#33716);
#3097=PLANE('',#33717);
#3098=PLANE('',#33718);
#3099=PLANE('',#33719);
#3100=PLANE('',#33720);
#3101=PLANE('',#33721);
#3102=PLANE('',#33722);
#3103=PLANE('',#33723);
#3104=PLANE('',#33724);
#3105=PLANE('',#33725);
#3106=PLANE('',#33726);
#3107=PLANE('',#33727);
#3108=PLANE('',#33728);
#3109=PLANE('',#33729);
#3110=PLANE('',#33730);
#3111=PLANE('',#33731);
#3112=PLANE('',#33732);
#3113=PLANE('',#33733);
#3114=PLANE('',#33734);
#3115=PLANE('',#33735);
#3116=PLANE('',#33736);
#3117=PLANE('',#33737);
#3118=PLANE('',#33738);
#3119=PLANE('',#33739);
#3120=PLANE('',#33740);
#3121=PLANE('',#33741);
#3122=PLANE('',#33742);
#3123=PLANE('',#33743);
#3124=PLANE('',#33744);
#3125=PLANE('',#33745);
#3126=PLANE('',#33746);
#3127=PLANE('',#33747);
#3128=PLANE('',#33748);
#3129=PLANE('',#33749);
#3130=PLANE('',#33750);
#3131=PLANE('',#33751);
#3132=PLANE('',#33752);
#3133=PLANE('',#33753);
#3134=PLANE('',#33754);
#3135=PLANE('',#33755);
#3136=PLANE('',#33756);
#3137=PLANE('',#33757);
#3138=PLANE('',#33758);
#3139=PLANE('',#33759);
#3140=PLANE('',#33760);
#3141=PLANE('',#33761);
#3142=PLANE('',#33762);
#3143=PLANE('',#33763);
#3144=PLANE('',#33764);
#3145=PLANE('',#33765);
#3146=PLANE('',#33766);
#3147=PLANE('',#33767);
#3148=PLANE('',#33768);
#3149=PLANE('',#33769);
#3150=PLANE('',#33770);
#3151=PLANE('',#33771);
#3152=PLANE('',#33772);
#3153=PLANE('',#33773);
#3154=PLANE('',#33774);
#3155=PLANE('',#33775);
#3156=PLANE('',#33776);
#3157=PLANE('',#33777);
#3158=PLANE('',#33778);
#3159=PLANE('',#33779);
#3160=PLANE('',#33780);
#3161=PLANE('',#33781);
#3162=PLANE('',#33782);
#3163=PLANE('',#33783);
#3164=PLANE('',#33784);
#3165=PLANE('',#33785);
#3166=PLANE('',#33786);
#3167=PLANE('',#33787);
#3168=PLANE('',#33788);
#3169=PLANE('',#33789);
#3170=PLANE('',#33790);
#3171=PLANE('',#33791);
#3172=PLANE('',#33792);
#3173=PLANE('',#33793);
#3174=PLANE('',#33794);
#3175=PLANE('',#33795);
#3176=PLANE('',#33796);
#3177=PLANE('',#33797);
#3178=PLANE('',#33798);
#3179=PLANE('',#33799);
#3180=PLANE('',#33800);
#3181=PLANE('',#33801);
#3182=PLANE('',#33802);
#3183=PLANE('',#33803);
#3184=PLANE('',#33804);
#3185=PLANE('',#33805);
#3186=PLANE('',#33806);
#3187=PLANE('',#33807);
#3188=PLANE('',#33810);
#3189=PLANE('',#33831);
#3190=PLANE('',#33832);
#3191=PLANE('',#33833);
#3192=PLANE('',#33834);
#3193=PLANE('',#33835);
#3194=PLANE('',#33836);
#3195=PLANE('',#33837);
#3196=PLANE('',#33838);
#3197=PLANE('',#33839);
#3198=PLANE('',#33840);
#3199=PLANE('',#33842);
#3200=PLANE('',#33844);
#3201=PLANE('',#33846);
#3202=PLANE('',#33848);
#3203=PLANE('',#33850);
#3204=PLANE('',#33853);
#3205=PLANE('',#33854);
#3206=PLANE('',#33855);
#4682=FACE_OUTER_BOUND('',#6647,.T.);
#4683=FACE_OUTER_BOUND('',#6648,.T.);
#4684=FACE_OUTER_BOUND('',#6649,.T.);
#4685=FACE_OUTER_BOUND('',#6650,.T.);
#4686=FACE_OUTER_BOUND('',#6651,.T.);
#4687=FACE_OUTER_BOUND('',#6652,.T.);
#4688=FACE_OUTER_BOUND('',#6653,.T.);
#4689=FACE_OUTER_BOUND('',#6654,.T.);
#4690=FACE_OUTER_BOUND('',#6655,.T.);
#4691=FACE_OUTER_BOUND('',#6656,.T.);
#4692=FACE_OUTER_BOUND('',#6657,.T.);
#4693=FACE_OUTER_BOUND('',#6658,.T.);
#4694=FACE_OUTER_BOUND('',#6659,.T.);
#4695=FACE_OUTER_BOUND('',#6660,.T.);
#4696=FACE_OUTER_BOUND('',#6661,.T.);
#4697=FACE_OUTER_BOUND('',#6662,.T.);
#4698=FACE_OUTER_BOUND('',#6663,.T.);
#4699=FACE_OUTER_BOUND('',#6664,.T.);
#4700=FACE_OUTER_BOUND('',#6665,.T.);
#4701=FACE_OUTER_BOUND('',#6666,.T.);
#4702=FACE_OUTER_BOUND('',#6667,.T.);
#4703=FACE_OUTER_BOUND('',#6668,.T.);
#4704=FACE_OUTER_BOUND('',#6669,.T.);
#4705=FACE_OUTER_BOUND('',#6670,.T.);
#4706=FACE_OUTER_BOUND('',#6671,.T.);
#4707=FACE_OUTER_BOUND('',#6672,.T.);
#4708=FACE_OUTER_BOUND('',#6673,.T.);
#4709=FACE_OUTER_BOUND('',#6674,.T.);
#4710=FACE_OUTER_BOUND('',#6675,.T.);
#4711=FACE_OUTER_BOUND('',#6676,.T.);
#4712=FACE_OUTER_BOUND('',#6677,.T.);
#4713=FACE_OUTER_BOUND('',#6678,.T.);
#4714=FACE_OUTER_BOUND('',#6679,.T.);
#4715=FACE_OUTER_BOUND('',#6680,.T.);
#4716=FACE_OUTER_BOUND('',#6681,.T.);
#4717=FACE_OUTER_BOUND('',#6682,.T.);
#4718=FACE_OUTER_BOUND('',#6683,.T.);
#4719=FACE_OUTER_BOUND('',#6684,.T.);
#4720=FACE_OUTER_BOUND('',#6685,.T.);
#4721=FACE_OUTER_BOUND('',#6686,.T.);
#4722=FACE_OUTER_BOUND('',#6687,.T.);
#4723=FACE_OUTER_BOUND('',#6688,.T.);
#4724=FACE_OUTER_BOUND('',#6689,.T.);
#4725=FACE_OUTER_BOUND('',#6690,.T.);
#4726=FACE_OUTER_BOUND('',#6691,.T.);
#4727=FACE_OUTER_BOUND('',#6692,.T.);
#4728=FACE_OUTER_BOUND('',#6693,.T.);
#4729=FACE_OUTER_BOUND('',#6694,.T.);
#4730=FACE_OUTER_BOUND('',#6695,.T.);
#4731=FACE_OUTER_BOUND('',#6696,.T.);
#4732=FACE_OUTER_BOUND('',#6697,.T.);
#4733=FACE_OUTER_BOUND('',#6698,.T.);
#4734=FACE_OUTER_BOUND('',#6699,.T.);
#4735=FACE_OUTER_BOUND('',#6700,.T.);
#4736=FACE_OUTER_BOUND('',#6702,.T.);
#4737=FACE_OUTER_BOUND('',#6703,.T.);
#4738=FACE_OUTER_BOUND('',#6704,.T.);
#4739=FACE_OUTER_BOUND('',#6705,.T.);
#4740=FACE_OUTER_BOUND('',#6706,.T.);
#4741=FACE_OUTER_BOUND('',#6707,.T.);
#4742=FACE_OUTER_BOUND('',#6708,.T.);
#4743=FACE_OUTER_BOUND('',#6709,.T.);
#4744=FACE_OUTER_BOUND('',#6710,.T.);
#4745=FACE_OUTER_BOUND('',#6711,.T.);
#4746=FACE_OUTER_BOUND('',#6712,.T.);
#4747=FACE_OUTER_BOUND('',#6713,.T.);
#4748=FACE_OUTER_BOUND('',#6714,.T.);
#4749=FACE_OUTER_BOUND('',#6715,.T.);
#4750=FACE_OUTER_BOUND('',#6716,.T.);
#4751=FACE_OUTER_BOUND('',#6717,.T.);
#4752=FACE_OUTER_BOUND('',#6718,.T.);
#4753=FACE_OUTER_BOUND('',#6719,.T.);
#4754=FACE_OUTER_BOUND('',#6720,.T.);
#4755=FACE_OUTER_BOUND('',#6721,.T.);
#4756=FACE_OUTER_BOUND('',#6722,.T.);
#4757=FACE_OUTER_BOUND('',#6723,.T.);
#4758=FACE_OUTER_BOUND('',#6724,.T.);
#4759=FACE_OUTER_BOUND('',#6725,.T.);
#4760=FACE_OUTER_BOUND('',#6726,.T.);
#4761=FACE_OUTER_BOUND('',#6727,.T.);
#4762=FACE_OUTER_BOUND('',#6728,.T.);
#4763=FACE_OUTER_BOUND('',#6729,.T.);
#4764=FACE_OUTER_BOUND('',#6730,.T.);
#4765=FACE_OUTER_BOUND('',#6731,.T.);
#4766=FACE_OUTER_BOUND('',#6732,.T.);
#4767=FACE_OUTER_BOUND('',#6733,.T.);
#4768=FACE_OUTER_BOUND('',#6734,.T.);
#4769=FACE_OUTER_BOUND('',#6735,.T.);
#4770=FACE_OUTER_BOUND('',#6736,.T.);
#4771=FACE_OUTER_BOUND('',#6737,.T.);
#4772=FACE_OUTER_BOUND('',#6738,.T.);
#4773=FACE_OUTER_BOUND('',#6739,.T.);
#4774=FACE_OUTER_BOUND('',#6740,.T.);
#4775=FACE_OUTER_BOUND('',#6741,.T.);
#4776=FACE_OUTER_BOUND('',#6742,.T.);
#4777=FACE_OUTER_BOUND('',#6743,.T.);
#4778=FACE_OUTER_BOUND('',#6744,.T.);
#4779=FACE_OUTER_BOUND('',#6745,.T.);
#4780=FACE_OUTER_BOUND('',#6746,.T.);
#4781=FACE_OUTER_BOUND('',#6747,.T.);
#4782=FACE_OUTER_BOUND('',#6748,.T.);
#4783=FACE_OUTER_BOUND('',#6749,.T.);
#4784=FACE_OUTER_BOUND('',#6750,.T.);
#4785=FACE_OUTER_BOUND('',#6751,.T.);
#4786=FACE_OUTER_BOUND('',#6752,.T.);
#4787=FACE_OUTER_BOUND('',#6753,.T.);
#4788=FACE_OUTER_BOUND('',#6754,.T.);
#4789=FACE_OUTER_BOUND('',#6755,.T.);
#4790=FACE_OUTER_BOUND('',#6756,.T.);
#4791=FACE_OUTER_BOUND('',#6757,.T.);
#4792=FACE_OUTER_BOUND('',#6758,.T.);
#4793=FACE_OUTER_BOUND('',#6759,.T.);
#4794=FACE_OUTER_BOUND('',#6760,.T.);
#4795=FACE_OUTER_BOUND('',#6761,.T.);
#4796=FACE_OUTER_BOUND('',#6762,.T.);
#4797=FACE_OUTER_BOUND('',#6763,.T.);
#4798=FACE_OUTER_BOUND('',#6764,.T.);
#4799=FACE_OUTER_BOUND('',#6765,.T.);
#4800=FACE_OUTER_BOUND('',#6766,.T.);
#4801=FACE_OUTER_BOUND('',#6767,.T.);
#4802=FACE_OUTER_BOUND('',#6768,.T.);
#4803=FACE_OUTER_BOUND('',#6769,.T.);
#4804=FACE_OUTER_BOUND('',#6770,.T.);
#4805=FACE_OUTER_BOUND('',#6771,.T.);
#4806=FACE_OUTER_BOUND('',#6772,.T.);
#4807=FACE_OUTER_BOUND('',#6773,.T.);
#4808=FACE_OUTER_BOUND('',#6774,.T.);
#4809=FACE_OUTER_BOUND('',#6775,.T.);
#4810=FACE_OUTER_BOUND('',#6776,.T.);
#4811=FACE_OUTER_BOUND('',#6777,.T.);
#4812=FACE_OUTER_BOUND('',#6778,.T.);
#4813=FACE_OUTER_BOUND('',#6779,.T.);
#4814=FACE_OUTER_BOUND('',#6780,.T.);
#4815=FACE_OUTER_BOUND('',#6781,.T.);
#4816=FACE_OUTER_BOUND('',#6782,.T.);
#4817=FACE_OUTER_BOUND('',#6783,.T.);
#4818=FACE_OUTER_BOUND('',#6784,.T.);
#4819=FACE_OUTER_BOUND('',#6785,.T.);
#4820=FACE_OUTER_BOUND('',#6786,.T.);
#4821=FACE_OUTER_BOUND('',#6787,.T.);
#4822=FACE_OUTER_BOUND('',#6788,.T.);
#4823=FACE_OUTER_BOUND('',#6789,.T.);
#4824=FACE_OUTER_BOUND('',#6790,.T.);
#4825=FACE_OUTER_BOUND('',#6791,.T.);
#4826=FACE_OUTER_BOUND('',#6792,.T.);
#4827=FACE_OUTER_BOUND('',#6793,.T.);
#4828=FACE_OUTER_BOUND('',#6794,.T.);
#4829=FACE_OUTER_BOUND('',#6795,.T.);
#4830=FACE_OUTER_BOUND('',#6796,.T.);
#4831=FACE_OUTER_BOUND('',#6797,.T.);
#4832=FACE_OUTER_BOUND('',#6798,.T.);
#4833=FACE_OUTER_BOUND('',#6799,.T.);
#4834=FACE_OUTER_BOUND('',#6800,.T.);
#4835=FACE_OUTER_BOUND('',#6801,.T.);
#4836=FACE_OUTER_BOUND('',#6802,.T.);
#4837=FACE_OUTER_BOUND('',#6803,.T.);
#4838=FACE_OUTER_BOUND('',#6804,.T.);
#4839=FACE_OUTER_BOUND('',#6805,.T.);
#4840=FACE_OUTER_BOUND('',#6806,.T.);
#4841=FACE_OUTER_BOUND('',#6807,.T.);
#4842=FACE_OUTER_BOUND('',#6808,.T.);
#4843=FACE_OUTER_BOUND('',#6809,.T.);
#4844=FACE_OUTER_BOUND('',#6810,.T.);
#4845=FACE_OUTER_BOUND('',#6811,.T.);
#4846=FACE_OUTER_BOUND('',#6812,.T.);
#4847=FACE_OUTER_BOUND('',#6813,.T.);
#4848=FACE_OUTER_BOUND('',#6814,.T.);
#4849=FACE_OUTER_BOUND('',#6815,.T.);
#4850=FACE_OUTER_BOUND('',#6817,.T.);
#4851=FACE_OUTER_BOUND('',#6818,.T.);
#4852=FACE_OUTER_BOUND('',#6819,.T.);
#4853=FACE_OUTER_BOUND('',#6820,.T.);
#4854=FACE_OUTER_BOUND('',#6821,.T.);
#4855=FACE_OUTER_BOUND('',#6822,.T.);
#4856=FACE_OUTER_BOUND('',#6823,.T.);
#4857=FACE_OUTER_BOUND('',#6824,.T.);
#4858=FACE_OUTER_BOUND('',#6825,.T.);
#4859=FACE_OUTER_BOUND('',#6826,.T.);
#4860=FACE_OUTER_BOUND('',#6827,.T.);
#4861=FACE_OUTER_BOUND('',#6828,.T.);
#4862=FACE_OUTER_BOUND('',#6829,.T.);
#4863=FACE_OUTER_BOUND('',#6830,.T.);
#4864=FACE_OUTER_BOUND('',#6831,.T.);
#4865=FACE_OUTER_BOUND('',#6832,.T.);
#4866=FACE_OUTER_BOUND('',#6833,.T.);
#4867=FACE_OUTER_BOUND('',#6834,.T.);
#4868=FACE_OUTER_BOUND('',#6835,.T.);
#4869=FACE_OUTER_BOUND('',#6836,.T.);
#4870=FACE_OUTER_BOUND('',#6837,.T.);
#4871=FACE_OUTER_BOUND('',#6838,.T.);
#4872=FACE_OUTER_BOUND('',#6839,.T.);
#4873=FACE_OUTER_BOUND('',#6840,.T.);
#4874=FACE_OUTER_BOUND('',#6841,.T.);
#4875=FACE_OUTER_BOUND('',#6842,.T.);
#6647=EDGE_LOOP('',(#27782,#27783,#27784,#27785));
#6648=EDGE_LOOP('',(#27786,#27787,#27788,#27789));
#6649=EDGE_LOOP('',(#27790,#27791,#27792,#27793));
#6650=EDGE_LOOP('',(#27794,#27795,#27796,#27797,#27798,#27799));
#6651=EDGE_LOOP('',(#27800,#27801,#27802,#27803));
#6652=EDGE_LOOP('',(#27804,#27805,#27806,#27807));
#6653=EDGE_LOOP('',(#27808,#27809,#27810,#27811,#27812,#27813));
#6654=EDGE_LOOP('',(#27814,#27815,#27816,#27817,#27818,#27819));
#6655=EDGE_LOOP('',(#27820,#27821,#27822,#27823));
#6656=EDGE_LOOP('',(#27824,#27825,#27826,#27827));
#6657=EDGE_LOOP('',(#27828,#27829,#27830,#27831,#27832,#27833));
#6658=EDGE_LOOP('',(#27834,#27835,#27836,#27837));
#6659=EDGE_LOOP('',(#27838,#27839,#27840,#27841,#27842,#27843));
#6660=EDGE_LOOP('',(#27844,#27845,#27846,#27847,#27848,#27849));
#6661=EDGE_LOOP('',(#27850,#27851,#27852,#27853));
#6662=EDGE_LOOP('',(#27854,#27855,#27856,#27857));
#6663=EDGE_LOOP('',(#27858,#27859,#27860,#27861,#27862,#27863));
#6664=EDGE_LOOP('',(#27864,#27865,#27866,#27867));
#6665=EDGE_LOOP('',(#27868,#27869,#27870,#27871));
#6666=EDGE_LOOP('',(#27872,#27873,#27874,#27875,#27876,#27877));
#6667=EDGE_LOOP('',(#27878,#27879,#27880,#27881));
#6668=EDGE_LOOP('',(#27882,#27883,#27884,#27885));
#6669=EDGE_LOOP('',(#27886,#27887,#27888,#27889,#27890));
#6670=EDGE_LOOP('',(#27891,#27892,#27893,#27894));
#6671=EDGE_LOOP('',(#27895,#27896,#27897,#27898));
#6672=EDGE_LOOP('',(#27899,#27900,#27901,#27902));
#6673=EDGE_LOOP('',(#27903,#27904,#27905,#27906));
#6674=EDGE_LOOP('',(#27907,#27908,#27909,#27910,#27911));
#6675=EDGE_LOOP('',(#27912,#27913,#27914,#27915,#27916));
#6676=EDGE_LOOP('',(#27917,#27918,#27919,#27920));
#6677=EDGE_LOOP('',(#27921,#27922,#27923,#27924));
#6678=EDGE_LOOP('',(#27925,#27926,#27927,#27928));
#6679=EDGE_LOOP('',(#27929,#27930,#27931,#27932));
#6680=EDGE_LOOP('',(#27933,#27934,#27935,#27936));
#6681=EDGE_LOOP('',(#27937,#27938,#27939,#27940));
#6682=EDGE_LOOP('',(#27941,#27942,#27943,#27944));
#6683=EDGE_LOOP('',(#27945,#27946,#27947,#27948));
#6684=EDGE_LOOP('',(#27949,#27950,#27951,#27952,#27953));
#6685=EDGE_LOOP('',(#27954,#27955,#27956,#27957));
#6686=EDGE_LOOP('',(#27958,#27959,#27960,#27961));
#6687=EDGE_LOOP('',(#27962,#27963,#27964,#27965));
#6688=EDGE_LOOP('',(#27966,#27967,#27968,#27969));
#6689=EDGE_LOOP('',(#27970,#27971,#27972,#27973));
#6690=EDGE_LOOP('',(#27974,#27975,#27976,#27977,#27978));
#6691=EDGE_LOOP('',(#27979,#27980,#27981,#27982));
#6692=EDGE_LOOP('',(#27983,#27984,#27985,#27986));
#6693=EDGE_LOOP('',(#27987,#27988,#27989,#27990,#27991));
#6694=EDGE_LOOP('',(#27992,#27993,#27994,#27995));
#6695=EDGE_LOOP('',(#27996,#27997,#27998,#27999,#28000));
#6696=EDGE_LOOP('',(#28001,#28002,#28003,#28004,#28005,#28006,#28007,#28008,
#28009,#28010,#28011,#28012,#28013,#28014,#28015,#28016,#28017,#28018,#28019,
#28020,#28021,#28022,#28023,#28024,#28025,#28026,#28027,#28028,#28029,#28030,
#28031,#28032,#28033,#28034,#28035,#28036,#28037,#28038,#28039,#28040,#28041,
#28042,#28043,#28044,#28045,#28046,#28047,#28048,#28049,#28050,#28051,#28052,
#28053,#28054,#28055,#28056,#28057,#28058,#28059,#28060,#28061,#28062));
#6697=EDGE_LOOP('',(#28063,#28064,#28065,#28066,#28067));
#6698=EDGE_LOOP('',(#28068,#28069,#28070,#28071,#28072,#28073,#28074,#28075,
#28076,#28077,#28078,#28079,#28080,#28081,#28082,#28083,#28084,#28085,#28086,
#28087,#28088,#28089,#28090,#28091,#28092,#28093,#28094,#28095,#28096,#28097,
#28098,#28099,#28100,#28101,#28102,#28103,#28104,#28105,#28106,#28107,#28108,
#28109,#28110,#28111,#28112,#28113,#28114,#28115,#28116,#28117,#28118,#28119,
#28120,#28121,#28122,#28123,#28124,#28125,#28126,#28127,#28128,#28129));
#6699=EDGE_LOOP('',(#28130,#28131,#28132,#28133,#28134,#28135,#28136));
#6700=EDGE_LOOP('',(#28137));
#6701=EDGE_LOOP('',(#28138));
#6702=EDGE_LOOP('',(#28139,#28140,#28141,#28142,#28143,#28144,#28145));
#6703=EDGE_LOOP('',(#28146));
#6704=EDGE_LOOP('',(#28147,#28148,#28149));
#6705=EDGE_LOOP('',(#28150,#28151,#28152,#28153));
#6706=EDGE_LOOP('',(#28154,#28155,#28156,#28157));
#6707=EDGE_LOOP('',(#28158,#28159,#28160,#28161,#28162,#28163,#28164,#28165,
#28166,#28167,#28168,#28169,#28170,#28171,#28172,#28173,#28174,#28175,#28176,
#28177,#28178,#28179,#28180,#28181,#28182,#28183,#28184,#28185,#28186,#28187,
#28188,#28189,#28190,#28191,#28192,#28193,#28194,#28195,#28196,#28197,#28198,
#28199,#28200,#28201,#28202,#28203,#28204,#28205,#28206,#28207,#28208,#28209,
#28210,#28211,#28212,#28213,#28214,#28215,#28216,#28217,#28218,#28219,#28220,
#28221,#28222,#28223,#28224,#28225,#28226,#28227,#28228,#28229,#28230,#28231,
#28232,#28233,#28234,#28235,#28236,#28237,#28238,#28239,#28240,#28241,#28242,
#28243,#28244,#28245,#28246,#28247,#28248,#28249,#28250,#28251,#28252,#28253,
#28254,#28255,#28256,#28257,#28258,#28259,#28260,#28261,#28262,#28263,#28264,
#28265,#28266,#28267,#28268,#28269,#28270,#28271,#28272,#28273,#28274,#28275,
#28276,#28277,#28278,#28279,#28280,#28281,#28282,#28283,#28284,#28285,#28286,
#28287,#28288,#28289,#28290,#28291,#28292,#28293,#28294,#28295,#28296,#28297,
#28298,#28299,#28300,#28301,#28302,#28303,#28304,#28305,#28306));
#6708=EDGE_LOOP('',(#28307,#28308,#28309,#28310));
#6709=EDGE_LOOP('',(#28311,#28312,#28313,#28314));
#6710=EDGE_LOOP('',(#28315,#28316,#28317));
#6711=EDGE_LOOP('',(#28318,#28319,#28320,#28321,#28322,#28323,#28324,#28325,
#28326,#28327,#28328,#28329,#28330,#28331,#28332,#28333,#28334,#28335,#28336,
#28337,#28338,#28339,#28340,#28341,#28342,#28343,#28344,#28345,#28346,#28347,
#28348,#28349,#28350,#28351,#28352,#28353,#28354,#28355,#28356,#28357,#28358,
#28359,#28360,#28361,#28362,#28363,#28364,#28365,#28366,#28367,#28368,#28369,
#28370,#28371,#28372,#28373,#28374,#28375,#28376,#28377,#28378,#28379,#28380,
#28381,#28382,#28383,#28384,#28385,#28386,#28387,#28388,#28389,#28390,#28391,
#28392,#28393,#28394,#28395,#28396,#28397,#28398,#28399,#28400,#28401,#28402,
#28403,#28404,#28405,#28406,#28407,#28408,#28409,#28410,#28411,#28412,#28413,
#28414,#28415,#28416,#28417,#28418,#28419,#28420,#28421,#28422,#28423,#28424,
#28425,#28426,#28427,#28428));
#6712=EDGE_LOOP('',(#28429,#28430,#28431));
#6713=EDGE_LOOP('',(#28432,#28433,#28434,#28435));
#6714=EDGE_LOOP('',(#28436,#28437,#28438,#28439));
#6715=EDGE_LOOP('',(#28440,#28441,#28442,#28443));
#6716=EDGE_LOOP('',(#28444,#28445,#28446,#28447));
#6717=EDGE_LOOP('',(#28448,#28449,#28450));
#6718=EDGE_LOOP('',(#28451,#28452,#28453));
#6719=EDGE_LOOP('',(#28454,#28455,#28456,#28457));
#6720=EDGE_LOOP('',(#28458,#28459,#28460,#28461));
#6721=EDGE_LOOP('',(#28462,#28463,#28464,#28465));
#6722=EDGE_LOOP('',(#28466,#28467,#28468,#28469));
#6723=EDGE_LOOP('',(#28470,#28471,#28472));
#6724=EDGE_LOOP('',(#28473,#28474,#28475));
#6725=EDGE_LOOP('',(#28476,#28477,#28478,#28479));
#6726=EDGE_LOOP('',(#28480,#28481,#28482,#28483));
#6727=EDGE_LOOP('',(#28484,#28485,#28486,#28487));
#6728=EDGE_LOOP('',(#28488,#28489,#28490,#28491));
#6729=EDGE_LOOP('',(#28492,#28493,#28494));
#6730=EDGE_LOOP('',(#28495,#28496,#28497));
#6731=EDGE_LOOP('',(#28498,#28499,#28500,#28501));
#6732=EDGE_LOOP('',(#28502,#28503,#28504,#28505));
#6733=EDGE_LOOP('',(#28506,#28507,#28508,#28509));
#6734=EDGE_LOOP('',(#28510,#28511,#28512,#28513));
#6735=EDGE_LOOP('',(#28514,#28515,#28516));
#6736=EDGE_LOOP('',(#28517,#28518,#28519));
#6737=EDGE_LOOP('',(#28520,#28521,#28522,#28523));
#6738=EDGE_LOOP('',(#28524,#28525,#28526,#28527));
#6739=EDGE_LOOP('',(#28528,#28529,#28530,#28531));
#6740=EDGE_LOOP('',(#28532,#28533,#28534,#28535));
#6741=EDGE_LOOP('',(#28536,#28537,#28538));
#6742=EDGE_LOOP('',(#28539,#28540,#28541));
#6743=EDGE_LOOP('',(#28542,#28543,#28544,#28545));
#6744=EDGE_LOOP('',(#28546,#28547,#28548,#28549));
#6745=EDGE_LOOP('',(#28550,#28551,#28552,#28553));
#6746=EDGE_LOOP('',(#28554,#28555,#28556,#28557));
#6747=EDGE_LOOP('',(#28558,#28559,#28560));
#6748=EDGE_LOOP('',(#28561,#28562,#28563));
#6749=EDGE_LOOP('',(#28564,#28565,#28566,#28567));
#6750=EDGE_LOOP('',(#28568,#28569,#28570,#28571));
#6751=EDGE_LOOP('',(#28572,#28573,#28574,#28575));
#6752=EDGE_LOOP('',(#28576,#28577,#28578,#28579));
#6753=EDGE_LOOP('',(#28580,#28581,#28582));
#6754=EDGE_LOOP('',(#28583,#28584,#28585));
#6755=EDGE_LOOP('',(#28586,#28587,#28588,#28589));
#6756=EDGE_LOOP('',(#28590,#28591,#28592,#28593));
#6757=EDGE_LOOP('',(#28594,#28595,#28596,#28597));
#6758=EDGE_LOOP('',(#28598,#28599,#28600,#28601));
#6759=EDGE_LOOP('',(#28602,#28603,#28604,#28605));
#6760=EDGE_LOOP('',(#28606,#28607,#28608));
#6761=EDGE_LOOP('',(#28609,#28610,#28611,#28612));
#6762=EDGE_LOOP('',(#28613,#28614,#28615,#28616));
#6763=EDGE_LOOP('',(#28617,#28618,#28619,#28620));
#6764=EDGE_LOOP('',(#28621,#28622,#28623,#28624));
#6765=EDGE_LOOP('',(#28625,#28626,#28627));
#6766=EDGE_LOOP('',(#28628,#28629,#28630));
#6767=EDGE_LOOP('',(#28631,#28632,#28633,#28634));
#6768=EDGE_LOOP('',(#28635,#28636,#28637,#28638));
#6769=EDGE_LOOP('',(#28639,#28640,#28641,#28642));
#6770=EDGE_LOOP('',(#28643,#28644,#28645,#28646));
#6771=EDGE_LOOP('',(#28647,#28648,#28649));
#6772=EDGE_LOOP('',(#28650,#28651,#28652));
#6773=EDGE_LOOP('',(#28653,#28654,#28655,#28656));
#6774=EDGE_LOOP('',(#28657,#28658,#28659,#28660));
#6775=EDGE_LOOP('',(#28661,#28662,#28663,#28664));
#6776=EDGE_LOOP('',(#28665,#28666,#28667,#28668));
#6777=EDGE_LOOP('',(#28669,#28670,#28671));
#6778=EDGE_LOOP('',(#28672,#28673,#28674));
#6779=EDGE_LOOP('',(#28675,#28676,#28677,#28678));
#6780=EDGE_LOOP('',(#28679,#28680,#28681,#28682));
#6781=EDGE_LOOP('',(#28683,#28684,#28685,#28686));
#6782=EDGE_LOOP('',(#28687,#28688,#28689,#28690));
#6783=EDGE_LOOP('',(#28691,#28692,#28693));
#6784=EDGE_LOOP('',(#28694,#28695,#28696));
#6785=EDGE_LOOP('',(#28697,#28698,#28699,#28700));
#6786=EDGE_LOOP('',(#28701,#28702,#28703,#28704));
#6787=EDGE_LOOP('',(#28705,#28706,#28707,#28708));
#6788=EDGE_LOOP('',(#28709,#28710,#28711,#28712));
#6789=EDGE_LOOP('',(#28713,#28714,#28715));
#6790=EDGE_LOOP('',(#28716,#28717,#28718));
#6791=EDGE_LOOP('',(#28719,#28720,#28721,#28722));
#6792=EDGE_LOOP('',(#28723,#28724,#28725,#28726));
#6793=EDGE_LOOP('',(#28727,#28728,#28729,#28730));
#6794=EDGE_LOOP('',(#28731,#28732,#28733,#28734));
#6795=EDGE_LOOP('',(#28735,#28736,#28737));
#6796=EDGE_LOOP('',(#28738,#28739,#28740));
#6797=EDGE_LOOP('',(#28741,#28742,#28743,#28744));
#6798=EDGE_LOOP('',(#28745,#28746,#28747,#28748));
#6799=EDGE_LOOP('',(#28749,#28750,#28751,#28752));
#6800=EDGE_LOOP('',(#28753,#28754,#28755,#28756));
#6801=EDGE_LOOP('',(#28757,#28758,#28759));
#6802=EDGE_LOOP('',(#28760,#28761,#28762));
#6803=EDGE_LOOP('',(#28763,#28764,#28765,#28766));
#6804=EDGE_LOOP('',(#28767,#28768,#28769,#28770));
#6805=EDGE_LOOP('',(#28771,#28772,#28773,#28774));
#6806=EDGE_LOOP('',(#28775,#28776,#28777,#28778));
#6807=EDGE_LOOP('',(#28779,#28780,#28781));
#6808=EDGE_LOOP('',(#28782,#28783,#28784));
#6809=EDGE_LOOP('',(#28785,#28786,#28787,#28788));
#6810=EDGE_LOOP('',(#28789,#28790,#28791,#28792));
#6811=EDGE_LOOP('',(#28793,#28794,#28795,#28796));
#6812=EDGE_LOOP('',(#28797,#28798,#28799,#28800));
#6813=EDGE_LOOP('',(#28801,#28802,#28803));
#6814=EDGE_LOOP('',(#28804,#28805,#28806,#28807,#28808));
#6815=EDGE_LOOP('',(#28809));
#6816=EDGE_LOOP('',(#28810));
#6817=EDGE_LOOP('',(#28811,#28812,#28813,#28814,#28815,#28816,#28817,#28818,
#28819,#28820,#28821,#28822,#28823,#28824,#28825,#28826,#28827,#28828,#28829,
#28830,#28831));
#6818=EDGE_LOOP('',(#28832,#28833,#28834,#28835));
#6819=EDGE_LOOP('',(#28836,#28837,#28838,#28839));
#6820=EDGE_LOOP('',(#28840,#28841,#28842,#28843));
#6821=EDGE_LOOP('',(#28844,#28845,#28846,#28847));
#6822=EDGE_LOOP('',(#28848,#28849,#28850,#28851));
#6823=EDGE_LOOP('',(#28852,#28853,#28854,#28855));
#6824=EDGE_LOOP('',(#28856,#28857,#28858,#28859,#28860,#28861,#28862,#28863));
#6825=EDGE_LOOP('',(#28864,#28865,#28866,#28867,#28868,#28869,#28870,#28871));
#6826=EDGE_LOOP('',(#28872,#28873,#28874,#28875,#28876,#28877,#28878,#28879));
#6827=EDGE_LOOP('',(#28880,#28881));
#6828=EDGE_LOOP('',(#28882,#28883));
#6829=EDGE_LOOP('',(#28884,#28885));
#6830=EDGE_LOOP('',(#28886,#28887));
#6831=EDGE_LOOP('',(#28888,#28889));
#6832=EDGE_LOOP('',(#28890,#28891));
#6833=EDGE_LOOP('',(#28892,#28893));
#6834=EDGE_LOOP('',(#28894,#28895));
#6835=EDGE_LOOP('',(#28896,#28897));
#6836=EDGE_LOOP('',(#28898,#28899));
#6837=EDGE_LOOP('',(#28900,#28901));
#6838=EDGE_LOOP('',(#28902,#28903));
#6839=EDGE_LOOP('',(#28904,#28905,#28906,#28907,#28908,#28909,#28910,#28911));
#6840=EDGE_LOOP('',(#28912,#28913,#28914,#28915,#28916,#28917,#28918,#28919));
#6841=EDGE_LOOP('',(#28920,#28921,#28922,#28923,#28924,#28925,#28926,#28927));
#6842=EDGE_LOOP('',(#28928,#28929,#28930,#28931,#28932,#28933,#28934,#28935));
#9362=LINE('',#84338,#12199);
#9363=LINE('',#84446,#12200);
#9364=LINE('',#84872,#12201);
#9365=LINE('',#85332,#12202);
#9366=LINE('',#85822,#12203);
#9367=LINE('',#86288,#12204);
#9368=LINE('',#86748,#12205);
#9369=LINE('',#87218,#12206);
#9370=LINE('',#87702,#12207);
#9371=LINE('',#88166,#12208);
#9372=LINE('',#88640,#12209);
#9373=LINE('',#89108,#12210);
#9374=LINE('',#89566,#12211);
#9375=LINE('',#90008,#12212);
#9376=LINE('',#90484,#12213);
#9377=LINE('',#90948,#12214);
#9378=LINE('',#91392,#12215);
#9379=LINE('',#91868,#12216);
#9380=LINE('',#92312,#12217);
#9381=LINE('',#92786,#12218);
#9382=LINE('',#93292,#12219);
#9383=LINE('',#93762,#12220);
#9384=LINE('',#94226,#12221);
#9385=LINE('',#94687,#12222);
#9386=LINE('',#94890,#12223);
#9387=LINE('',#95364,#12224);
#9388=LINE('',#95794,#12225);
#9389=LINE('',#96222,#12226);
#9390=LINE('',#96665,#12227);
#9391=LINE('',#97106,#12228);
#9392=LINE('',#97548,#12229);
#9393=LINE('',#97972,#12230);
#9394=LINE('',#98398,#12231);
#9395=LINE('',#98846,#12232);
#9396=LINE('',#99304,#12233);
#9397=LINE('',#99730,#12234);
#9398=LINE('',#100162,#12235);
#9399=LINE('',#100586,#12236);
#9400=LINE('',#101043,#12237);
#9401=LINE('',#101461,#12238);
#9402=LINE('',#101885,#12239);
#9403=LINE('',#102321,#12240);
#9404=LINE('',#102739,#12241);
#9405=LINE('',#103177,#12242);
#9406=LINE('',#103636,#12243);
#9407=LINE('',#104050,#12244);
#9408=LINE('',#106664,#12245);
#9409=LINE('',#106672,#12246);
#9410=LINE('',#106673,#12247);
#9411=LINE('',#106676,#12248);
#9412=LINE('',#106678,#12249);
#9413=LINE('',#106684,#12250);
#9414=LINE('',#106693,#12251);
#9415=LINE('',#106700,#12252);
#9416=LINE('',#106704,#12253);
#9417=LINE('',#106708,#12254);
#9418=LINE('',#106712,#12255);
#9419=LINE('',#106716,#12256);
#9420=LINE('',#106720,#12257);
#9421=LINE('',#106724,#12258);
#9422=LINE('',#106728,#12259);
#9423=LINE('',#106732,#12260);
#9424=LINE('',#106736,#12261);
#9425=LINE('',#106740,#12262);
#9426=LINE('',#106744,#12263);
#9427=LINE('',#106748,#12264);
#9428=LINE('',#106752,#12265);
#9429=LINE('',#106756,#12266);
#9430=LINE('',#106760,#12267);
#9431=LINE('',#106764,#12268);
#9432=LINE('',#106768,#12269);
#9433=LINE('',#106772,#12270);
#9434=LINE('',#106776,#12271);
#9435=LINE('',#106780,#12272);
#9436=LINE('',#106784,#12273);
#9437=LINE('',#106788,#12274);
#9438=LINE('',#106792,#12275);
#9439=LINE('',#106796,#12276);
#9440=LINE('',#106800,#12277);
#9441=LINE('',#106804,#12278);
#9442=LINE('',#106808,#12279);
#9443=LINE('',#106812,#12280);
#9444=LINE('',#106816,#12281);
#9445=LINE('',#106820,#12282);
#9446=LINE('',#106824,#12283);
#9447=LINE('',#106828,#12284);
#9448=LINE('',#106833,#12285);
#9449=LINE('',#106837,#12286);
#9450=LINE('',#106841,#12287);
#9451=LINE('',#106845,#12288);
#9452=LINE('',#106849,#12289);
#9453=LINE('',#106853,#12290);
#9454=LINE('',#106857,#12291);
#9455=LINE('',#106861,#12292);
#9456=LINE('',#106865,#12293);
#9457=LINE('',#106869,#12294);
#9458=LINE('',#106873,#12295);
#9459=LINE('',#106877,#12296);
#9460=LINE('',#106881,#12297);
#9461=LINE('',#106885,#12298);
#9462=LINE('',#106889,#12299);
#9463=LINE('',#106893,#12300);
#9464=LINE('',#106897,#12301);
#9465=LINE('',#106901,#12302);
#9466=LINE('',#106905,#12303);
#9467=LINE('',#106909,#12304);
#9468=LINE('',#106913,#12305);
#9469=LINE('',#106917,#12306);
#9470=LINE('',#106921,#12307);
#9471=LINE('',#106925,#12308);
#9472=LINE('',#106929,#12309);
#9473=LINE('',#106933,#12310);
#9474=LINE('',#106937,#12311);
#9475=LINE('',#106941,#12312);
#9476=LINE('',#106945,#12313);
#9477=LINE('',#106949,#12314);
#9478=LINE('',#106953,#12315);
#9479=LINE('',#106957,#12316);
#9480=LINE('',#106961,#12317);
#9481=LINE('',#106965,#12318);
#9482=LINE('',#106969,#12319);
#9483=LINE('',#106973,#12320);
#9484=LINE('',#106976,#12321);
#9485=LINE('',#106979,#12322);
#9486=LINE('',#106981,#12323);
#9487=LINE('',#106989,#12324);
#9488=LINE('',#107231,#12325);
#9489=LINE('',#107235,#12326);
#9490=LINE('',#107236,#12327);
#9491=LINE('',#107238,#12328);
#9492=LINE('',#107242,#12329);
#9493=LINE('',#107243,#12330);
#9494=LINE('',#107245,#12331);
#9495=LINE('',#107249,#12332);
#9496=LINE('',#107250,#12333);
#9497=LINE('',#107252,#12334);
#9498=LINE('',#107256,#12335);
#9499=LINE('',#107257,#12336);
#9500=LINE('',#107259,#12337);
#9501=LINE('',#107263,#12338);
#9502=LINE('',#107264,#12339);
#9503=LINE('',#107266,#12340);
#9504=LINE('',#107270,#12341);
#9505=LINE('',#107271,#12342);
#9506=LINE('',#107273,#12343);
#9507=LINE('',#107277,#12344);
#9508=LINE('',#107278,#12345);
#9509=LINE('',#107280,#12346);
#9510=LINE('',#107284,#12347);
#9511=LINE('',#107285,#12348);
#9512=LINE('',#107287,#12349);
#9513=LINE('',#107291,#12350);
#9514=LINE('',#107292,#12351);
#9515=LINE('',#107294,#12352);
#9516=LINE('',#107298,#12353);
#9517=LINE('',#107299,#12354);
#9518=LINE('',#107301,#12355);
#9519=LINE('',#107305,#12356);
#9520=LINE('',#107306,#12357);
#9521=LINE('',#107308,#12358);
#9522=LINE('',#107312,#12359);
#9523=LINE('',#107313,#12360);
#9524=LINE('',#107315,#12361);
#9525=LINE('',#107319,#12362);
#9526=LINE('',#107320,#12363);
#9527=LINE('',#107322,#12364);
#9528=LINE('',#107326,#12365);
#9529=LINE('',#107327,#12366);
#9530=LINE('',#107329,#12367);
#9531=LINE('',#107333,#12368);
#9532=LINE('',#107334,#12369);
#9533=LINE('',#107336,#12370);
#9534=LINE('',#107340,#12371);
#9535=LINE('',#107341,#12372);
#9536=LINE('',#107343,#12373);
#9537=LINE('',#107347,#12374);
#9538=LINE('',#107348,#12375);
#9539=LINE('',#107350,#12376);
#9540=LINE('',#107354,#12377);
#9541=LINE('',#107355,#12378);
#9542=LINE('',#107357,#12379);
#9543=LINE('',#107361,#12380);
#9544=LINE('',#107362,#12381);
#9545=LINE('',#107364,#12382);
#9546=LINE('',#107368,#12383);
#9547=LINE('',#107369,#12384);
#9548=LINE('',#107371,#12385);
#9549=LINE('',#107375,#12386);
#9550=LINE('',#107376,#12387);
#9551=LINE('',#107378,#12388);
#9552=LINE('',#107382,#12389);
#9553=LINE('',#107383,#12390);
#9554=LINE('',#107385,#12391);
#9555=LINE('',#107389,#12392);
#9556=LINE('',#107390,#12393);
#9557=LINE('',#107392,#12394);
#9558=LINE('',#107396,#12395);
#9559=LINE('',#107397,#12396);
#9560=LINE('',#107399,#12397);
#9561=LINE('',#107403,#12398);
#9562=LINE('',#107404,#12399);
#9563=LINE('',#107406,#12400);
#9564=LINE('',#107410,#12401);
#9565=LINE('',#107411,#12402);
#9566=LINE('',#107413,#12403);
#9567=LINE('',#107417,#12404);
#9568=LINE('',#107418,#12405);
#9569=LINE('',#107420,#12406);
#9570=LINE('',#107424,#12407);
#9571=LINE('',#107425,#12408);
#9572=LINE('',#107427,#12409);
#9573=LINE('',#107431,#12410);
#9574=LINE('',#107432,#12411);
#9575=LINE('',#107434,#12412);
#9576=LINE('',#107438,#12413);
#9577=LINE('',#107439,#12414);
#9578=LINE('',#107441,#12415);
#9579=LINE('',#107445,#12416);
#9580=LINE('',#107446,#12417);
#9581=LINE('',#107448,#12418);
#9582=LINE('',#107452,#12419);
#9583=LINE('',#107453,#12420);
#9584=LINE('',#107455,#12421);
#9585=LINE('',#107459,#12422);
#9586=LINE('',#107460,#12423);
#9587=LINE('',#107462,#12424);
#9588=LINE('',#107466,#12425);
#9589=LINE('',#107467,#12426);
#9590=LINE('',#107469,#12427);
#9591=LINE('',#107537,#12428);
#9592=LINE('',#107540,#12429);
#9593=LINE('',#107542,#12430);
#9594=LINE('',#107546,#12431);
#9595=LINE('',#107549,#12432);
#9596=LINE('',#107552,#12433);
#9597=LINE('',#107554,#12434);
#9598=LINE('',#107558,#12435);
#9599=LINE('',#107561,#12436);
#9600=LINE('',#107564,#12437);
#9601=LINE('',#107566,#12438);
#9602=LINE('',#107570,#12439);
#9603=LINE('',#107573,#12440);
#9604=LINE('',#107575,#12441);
#9605=LINE('',#107577,#12442);
#9606=LINE('',#107579,#12443);
#9607=LINE('',#107580,#12444);
#9608=LINE('',#107582,#12445);
#9609=LINE('',#107584,#12446);
#9610=LINE('',#107585,#12447);
#9611=LINE('',#107587,#12448);
#9612=LINE('',#107589,#12449);
#9613=LINE('',#107590,#12450);
#9614=LINE('',#107594,#12451);
#9615=LINE('',#107597,#12452);
#9616=LINE('',#107599,#12453);
#9617=LINE('',#107603,#12454);
#9618=LINE('',#107606,#12455);
#9619=LINE('',#107615,#12456);
#9620=LINE('',#107619,#12457);
#9621=LINE('',#107621,#12458);
#9622=LINE('',#107622,#12459);
#12199=VECTOR('',#39166,1.4635);
#12200=VECTOR('',#39171,1.4635);
#12201=VECTOR('',#39174,1.4635);
#12202=VECTOR('',#39177,1.4635);
#12203=VECTOR('',#39180,1.4635);
#12204=VECTOR('',#39183,1.4635);
#12205=VECTOR('',#39186,1.4635);
#12206=VECTOR('',#39189,1.4635);
#12207=VECTOR('',#39192,1.4635);
#12208=VECTOR('',#39195,1.4635);
#12209=VECTOR('',#39198,1.4635);
#12210=VECTOR('',#39201,1.4635);
#12211=VECTOR('',#39204,1.4635);
#12212=VECTOR('',#39207,1.4635);
#12213=VECTOR('',#39210,1.4635);
#12214=VECTOR('',#39213,1.4635);
#12215=VECTOR('',#39216,1.4635);
#12216=VECTOR('',#39219,1.4635);
#12217=VECTOR('',#39222,1.4635);
#12218=VECTOR('',#39225,1.4635);
#12219=VECTOR('',#39228,1.4635);
#12220=VECTOR('',#39231,1.4635);
#12221=VECTOR('',#39234,1.4635);
#12222=VECTOR('',#39237,1.17775);
#12223=VECTOR('',#39242,1.17775);
#12224=VECTOR('',#39245,1.17775);
#12225=VECTOR('',#39248,1.17775);
#12226=VECTOR('',#39251,1.17775);
#12227=VECTOR('',#39254,1.17775);
#12228=VECTOR('',#39257,1.17775);
#12229=VECTOR('',#39260,1.17775);
#12230=VECTOR('',#39263,1.17775);
#12231=VECTOR('',#39266,1.17775);
#12232=VECTOR('',#39269,1.17775);
#12233=VECTOR('',#39272,1.17775);
#12234=VECTOR('',#39275,1.17775);
#12235=VECTOR('',#39278,1.17775);
#12236=VECTOR('',#39281,1.17775);
#12237=VECTOR('',#39284,1.17775);
#12238=VECTOR('',#39287,1.17775);
#12239=VECTOR('',#39290,1.17775);
#12240=VECTOR('',#39293,1.17775);
#12241=VECTOR('',#39296,1.17775);
#12242=VECTOR('',#39299,1.17775);
#12243=VECTOR('',#39302,1.17775);
#12244=VECTOR('',#39305,1.17775);
#12245=VECTOR('',#39338,1.2885);
#12246=VECTOR('',#39347,10.);
#12247=VECTOR('',#39348,10.);
#12248=VECTOR('',#39351,10.);
#12249=VECTOR('',#39352,10.);
#12250=VECTOR('',#39355,10.);
#12251=VECTOR('',#39360,2.75);
#12252=VECTOR('',#39367,10.);
#12253=VECTOR('',#39370,10.);
#12254=VECTOR('',#39373,10.);
#12255=VECTOR('',#39376,10.);
#12256=VECTOR('',#39379,10.);
#12257=VECTOR('',#39382,10.);
#12258=VECTOR('',#39385,10.);
#12259=VECTOR('',#39388,10.);
#12260=VECTOR('',#39391,10.);
#12261=VECTOR('',#39394,10.);
#12262=VECTOR('',#39397,10.);
#12263=VECTOR('',#39400,10.);
#12264=VECTOR('',#39403,10.);
#12265=VECTOR('',#39406,10.);
#12266=VECTOR('',#39409,10.);
#12267=VECTOR('',#39412,10.);
#12268=VECTOR('',#39415,10.);
#12269=VECTOR('',#39418,10.);
#12270=VECTOR('',#39421,10.);
#12271=VECTOR('',#39424,10.);
#12272=VECTOR('',#39427,10.);
#12273=VECTOR('',#39430,10.);
#12274=VECTOR('',#39433,10.);
#12275=VECTOR('',#39436,10.);
#12276=VECTOR('',#39439,10.);
#12277=VECTOR('',#39442,10.);
#12278=VECTOR('',#39445,10.);
#12279=VECTOR('',#39448,10.);
#12280=VECTOR('',#39451,10.);
#12281=VECTOR('',#39454,10.);
#12282=VECTOR('',#39457,10.);
#12283=VECTOR('',#39460,10.);
#12284=VECTOR('',#39463,10.);
#12285=VECTOR('',#39468,10.);
#12286=VECTOR('',#39471,10.);
#12287=VECTOR('',#39474,10.);
#12288=VECTOR('',#39477,10.);
#12289=VECTOR('',#39480,10.);
#12290=VECTOR('',#39483,10.);
#12291=VECTOR('',#39486,10.);
#12292=VECTOR('',#39489,10.);
#12293=VECTOR('',#39492,10.);
#12294=VECTOR('',#39495,10.);
#12295=VECTOR('',#39498,10.);
#12296=VECTOR('',#39501,10.);
#12297=VECTOR('',#39504,10.);
#12298=VECTOR('',#39507,10.);
#12299=VECTOR('',#39510,10.);
#12300=VECTOR('',#39513,10.);
#12301=VECTOR('',#39516,10.);
#12302=VECTOR('',#39519,10.);
#12303=VECTOR('',#39522,10.);
#12304=VECTOR('',#39525,10.);
#12305=VECTOR('',#39528,10.);
#12306=VECTOR('',#39531,10.);
#12307=VECTOR('',#39534,10.);
#12308=VECTOR('',#39537,10.);
#12309=VECTOR('',#39540,10.);
#12310=VECTOR('',#39543,10.);
#12311=VECTOR('',#39546,10.);
#12312=VECTOR('',#39549,10.);
#12313=VECTOR('',#39552,10.);
#12314=VECTOR('',#39555,10.);
#12315=VECTOR('',#39558,10.);
#12316=VECTOR('',#39561,10.);
#12317=VECTOR('',#39564,10.);
#12318=VECTOR('',#39567,10.);
#12319=VECTOR('',#39570,10.);
#12320=VECTOR('',#39573,10.);
#12321=VECTOR('',#39576,10.);
#12322=VECTOR('',#39579,10.);
#12323=VECTOR('',#39580,10.);
#12324=VECTOR('',#39583,10.);
#12325=VECTOR('',#39588,2.6);
#12326=VECTOR('',#39593,10.);
#12327=VECTOR('',#39594,10.);
#12328=VECTOR('',#39597,10.);
#12329=VECTOR('',#39602,10.);
#12330=VECTOR('',#39603,10.);
#12331=VECTOR('',#39606,10.);
#12332=VECTOR('',#39611,10.);
#12333=VECTOR('',#39612,10.);
#12334=VECTOR('',#39615,10.);
#12335=VECTOR('',#39620,10.);
#12336=VECTOR('',#39621,10.);
#12337=VECTOR('',#39624,10.);
#12338=VECTOR('',#39629,10.);
#12339=VECTOR('',#39630,10.);
#12340=VECTOR('',#39633,10.);
#12341=VECTOR('',#39638,10.);
#12342=VECTOR('',#39639,10.);
#12343=VECTOR('',#39642,10.);
#12344=VECTOR('',#39647,10.);
#12345=VECTOR('',#39648,10.);
#12346=VECTOR('',#39651,10.);
#12347=VECTOR('',#39656,10.);
#12348=VECTOR('',#39657,10.);
#12349=VECTOR('',#39660,10.);
#12350=VECTOR('',#39665,10.);
#12351=VECTOR('',#39666,10.);
#12352=VECTOR('',#39669,10.);
#12353=VECTOR('',#39674,10.);
#12354=VECTOR('',#39675,10.);
#12355=VECTOR('',#39678,10.);
#12356=VECTOR('',#39683,10.);
#12357=VECTOR('',#39684,10.);
#12358=VECTOR('',#39687,10.);
#12359=VECTOR('',#39692,10.);
#12360=VECTOR('',#39693,10.);
#12361=VECTOR('',#39696,10.);
#12362=VECTOR('',#39701,10.);
#12363=VECTOR('',#39702,10.);
#12364=VECTOR('',#39705,10.);
#12365=VECTOR('',#39710,10.);
#12366=VECTOR('',#39711,10.);
#12367=VECTOR('',#39714,10.);
#12368=VECTOR('',#39719,10.);
#12369=VECTOR('',#39720,10.);
#12370=VECTOR('',#39723,10.);
#12371=VECTOR('',#39728,10.);
#12372=VECTOR('',#39729,10.);
#12373=VECTOR('',#39732,10.);
#12374=VECTOR('',#39737,10.);
#12375=VECTOR('',#39738,10.);
#12376=VECTOR('',#39741,10.);
#12377=VECTOR('',#39746,10.);
#12378=VECTOR('',#39747,10.);
#12379=VECTOR('',#39750,10.);
#12380=VECTOR('',#39755,10.);
#12381=VECTOR('',#39756,10.);
#12382=VECTOR('',#39759,10.);
#12383=VECTOR('',#39764,10.);
#12384=VECTOR('',#39765,10.);
#12385=VECTOR('',#39768,10.);
#12386=VECTOR('',#39773,10.);
#12387=VECTOR('',#39774,9.99999999999999);
#12388=VECTOR('',#39777,10.);
#12389=VECTOR('',#39782,10.);
#12390=VECTOR('',#39783,10.);
#12391=VECTOR('',#39786,10.);
#12392=VECTOR('',#39791,10.);
#12393=VECTOR('',#39792,10.);
#12394=VECTOR('',#39795,10.);
#12395=VECTOR('',#39800,10.);
#12396=VECTOR('',#39801,10.);
#12397=VECTOR('',#39804,10.);
#12398=VECTOR('',#39809,10.);
#12399=VECTOR('',#39810,10.);
#12400=VECTOR('',#39813,10.);
#12401=VECTOR('',#39818,10.);
#12402=VECTOR('',#39819,10.);
#12403=VECTOR('',#39822,10.);
#12404=VECTOR('',#39827,10.);
#12405=VECTOR('',#39828,10.);
#12406=VECTOR('',#39831,10.);
#12407=VECTOR('',#39836,10.);
#12408=VECTOR('',#39837,10.);
#12409=VECTOR('',#39840,10.);
#12410=VECTOR('',#39845,9.99999999999999);
#12411=VECTOR('',#39846,10.);
#12412=VECTOR('',#39849,10.);
#12413=VECTOR('',#39854,10.);
#12414=VECTOR('',#39855,10.);
#12415=VECTOR('',#39858,10.);
#12416=VECTOR('',#39863,10.);
#12417=VECTOR('',#39864,10.);
#12418=VECTOR('',#39867,10.);
#12419=VECTOR('',#39872,10.);
#12420=VECTOR('',#39873,10.);
#12421=VECTOR('',#39876,10.);
#12422=VECTOR('',#39881,10.);
#12423=VECTOR('',#39882,10.);
#12424=VECTOR('',#39885,10.);
#12425=VECTOR('',#39890,10.);
#12426=VECTOR('',#39891,10.);
#12427=VECTOR('',#39894,10.);
#12428=VECTOR('',#39919,1.49337567297406);
#12429=VECTOR('',#39922,10.);
#12430=VECTOR('',#39923,10.);
#12431=VECTOR('',#39928,10.);
#12432=VECTOR('',#39931,10.);
#12433=VECTOR('',#39934,10.);
#12434=VECTOR('',#39935,10.);
#12435=VECTOR('',#39940,10.);
#12436=VECTOR('',#39943,10.);
#12437=VECTOR('',#39946,10.);
#12438=VECTOR('',#39947,10.);
#12439=VECTOR('',#39952,10.);
#12440=VECTOR('',#39955,10.);
#12441=VECTOR('',#39958,10.);
#12442=VECTOR('',#39959,10.);
#12443=VECTOR('',#39960,10.);
#12444=VECTOR('',#39961,10.);
#12445=VECTOR('',#39964,10.);
#12446=VECTOR('',#39965,10.);
#12447=VECTOR('',#39966,10.);
#12448=VECTOR('',#39969,10.);
#12449=VECTOR('',#39970,10.);
#12450=VECTOR('',#39971,10.);
#12451=VECTOR('',#39978,10.);
#12452=VECTOR('',#39983,10.);
#12453=VECTOR('',#39986,10.);
#12454=VECTOR('',#39989,10.);
#12455=VECTOR('',#39994,10.);
#12456=VECTOR('',#40011,10.);
#12457=VECTOR('',#40016,0.721687836487032);
#12458=VECTOR('',#40019,10.);
#12459=VECTOR('',#40020,10.);
#13011=CIRCLE('',#33557,1.4635);
#13012=CIRCLE('',#33581,1.17775);
#13013=CIRCLE('',#33605,1.17775);
#13014=CIRCLE('',#33607,1.4635);
#13015=CIRCLE('',#33609,1.4635);
#13016=CIRCLE('',#33610,1.4635);
#13017=CIRCLE('',#33612,1.4635);
#13018=CIRCLE('',#33613,1.4635);
#13019=CIRCLE('',#33615,1.5635);
#13020=CIRCLE('',#33616,0.1);
#13021=CIRCLE('',#33618,2.55);
#13022=CIRCLE('',#33620,1.1135);
#13023=CIRCLE('',#33623,2.75);
#13024=CIRCLE('',#33627,2.75);
#13025=CIRCLE('',#33628,2.75);
#13026=CIRCLE('',#33629,2.75);
#13027=CIRCLE('',#33630,2.75);
#13028=CIRCLE('',#33631,2.75);
#13029=CIRCLE('',#33632,2.75);
#13030=CIRCLE('',#33633,2.75);
#13031=CIRCLE('',#33634,2.75);
#13032=CIRCLE('',#33635,2.75);
#13033=CIRCLE('',#33636,2.75);
#13034=CIRCLE('',#33637,2.75);
#13035=CIRCLE('',#33638,2.75);
#13036=CIRCLE('',#33639,2.75);
#13037=CIRCLE('',#33640,2.75);
#13038=CIRCLE('',#33641,2.75);
#13039=CIRCLE('',#33642,2.75);
#13040=CIRCLE('',#33643,2.75);
#13041=CIRCLE('',#33644,2.75);
#13042=CIRCLE('',#33645,2.75);
#13043=CIRCLE('',#33646,2.75);
#13044=CIRCLE('',#33647,2.75);
#13045=CIRCLE('',#33648,2.75);
#13046=CIRCLE('',#33649,2.75);
#13047=CIRCLE('',#33650,2.75);
#13048=CIRCLE('',#33651,2.75);
#13049=CIRCLE('',#33652,2.75);
#13050=CIRCLE('',#33653,2.75);
#13051=CIRCLE('',#33654,2.75);
#13052=CIRCLE('',#33655,2.75);
#13053=CIRCLE('',#33656,2.75);
#13054=CIRCLE('',#33657,2.75);
#13055=CIRCLE('',#33658,2.75);
#13056=CIRCLE('',#33659,2.75);
#13057=CIRCLE('',#33660,2.75);
#13058=CIRCLE('',#33661,2.75);
#13059=CIRCLE('',#33662,2.75);
#13060=CIRCLE('',#33663,2.75);
#13061=CIRCLE('',#33664,2.75);
#13062=CIRCLE('',#33665,2.75);
#13063=CIRCLE('',#33666,2.75);
#13064=CIRCLE('',#33667,2.75);
#13065=CIRCLE('',#33668,2.75);
#13066=CIRCLE('',#33669,2.75);
#13067=CIRCLE('',#33670,2.75);
#13068=CIRCLE('',#33671,2.75);
#13069=CIRCLE('',#33672,2.75);
#13070=CIRCLE('',#33673,2.75);
#13071=CIRCLE('',#33674,2.75);
#13072=CIRCLE('',#33675,2.75);
#13073=CIRCLE('',#33676,2.75);
#13074=CIRCLE('',#33677,2.75);
#13075=CIRCLE('',#33678,2.75);
#13076=CIRCLE('',#33679,2.75);
#13077=CIRCLE('',#33680,2.75);
#13078=CIRCLE('',#33681,2.75);
#13079=CIRCLE('',#33682,2.75);
#13080=CIRCLE('',#33683,2.75);
#13081=CIRCLE('',#33684,2.75);
#13082=CIRCLE('',#33685,2.75);
#13083=CIRCLE('',#33686,2.75);
#13084=CIRCLE('',#33687,2.75);
#13085=CIRCLE('',#33688,2.75);
#13086=CIRCLE('',#33689,2.75);
#13087=CIRCLE('',#33690,2.75);
#13088=CIRCLE('',#33691,2.75);
#13089=CIRCLE('',#33692,2.75);
#13090=CIRCLE('',#33693,2.75);
#13091=CIRCLE('',#33694,2.75);
#13092=CIRCLE('',#33695,2.75);
#13093=CIRCLE('',#33696,2.75);
#13094=CIRCLE('',#33697,2.75);
#13095=CIRCLE('',#33698,2.75);
#13096=CIRCLE('',#33699,2.75);
#13097=CIRCLE('',#33700,2.75);
#13098=CIRCLE('',#33705,2.45);
#13099=CIRCLE('',#33809,0.2);
#13100=CIRCLE('',#33811,1.59337567297406);
#13101=CIRCLE('',#33813,1.39337567297406);
#13102=CIRCLE('',#33814,1.39337567297406);
#13103=CIRCLE('',#33815,1.39337567297406);
#13104=CIRCLE('',#33816,1.39337567297406);
#13105=CIRCLE('',#33817,1.39337567297406);
#13106=CIRCLE('',#33818,1.39337567297406);
#13107=CIRCLE('',#33820,1.39337567297406);
#13108=CIRCLE('',#33822,1.39337567297406);
#13109=CIRCLE('',#33824,1.39337567297406);
#13110=CIRCLE('',#33826,1.39337567297406);
#13111=CIRCLE('',#33828,1.39337567297406);
#13112=CIRCLE('',#33830,1.39337567297406);
#13113=CIRCLE('',#33841,1.44337567297406);
#13114=CIRCLE('',#33843,1.44337567297406);
#13115=CIRCLE('',#33845,1.44337567297406);
#13116=CIRCLE('',#33847,1.44337567297406);
#13117=CIRCLE('',#33849,1.44337567297406);
#13118=CIRCLE('',#33851,1.44337567297406);
#15512=VERTEX_POINT('',#84336);
#15513=VERTEX_POINT('',#84337);
#15514=VERTEX_POINT('',#84339);
#15515=VERTEX_POINT('',#84410);
#15516=VERTEX_POINT('',#84444);
#15517=VERTEX_POINT('',#84445);
#15518=VERTEX_POINT('',#84870);
#15519=VERTEX_POINT('',#84871);
#15520=VERTEX_POINT('',#85330);
#15521=VERTEX_POINT('',#85331);
#15522=VERTEX_POINT('',#85333);
#15523=VERTEX_POINT('',#85564);
#15524=VERTEX_POINT('',#85820);
#15525=VERTEX_POINT('',#85821);
#15526=VERTEX_POINT('',#86286);
#15527=VERTEX_POINT('',#86287);
#15528=VERTEX_POINT('',#86746);
#15529=VERTEX_POINT('',#86747);
#15530=VERTEX_POINT('',#86749);
#15531=VERTEX_POINT('',#86984);
#15532=VERTEX_POINT('',#87216);
#15533=VERTEX_POINT('',#87217);
#15534=VERTEX_POINT('',#87219);
#15535=VERTEX_POINT('',#87442);
#15536=VERTEX_POINT('',#87700);
#15537=VERTEX_POINT('',#87701);
#15538=VERTEX_POINT('',#88164);
#15539=VERTEX_POINT('',#88165);
#15540=VERTEX_POINT('',#88638);
#15541=VERTEX_POINT('',#88639);
#15542=VERTEX_POINT('',#88641);
#15543=VERTEX_POINT('',#88874);
#15544=VERTEX_POINT('',#89106);
#15545=VERTEX_POINT('',#89107);
#15546=VERTEX_POINT('',#89564);
#15547=VERTEX_POINT('',#89565);
#15548=VERTEX_POINT('',#89567);
#15549=VERTEX_POINT('',#89788);
#15550=VERTEX_POINT('',#90006);
#15551=VERTEX_POINT('',#90007);
#15552=VERTEX_POINT('',#90009);
#15553=VERTEX_POINT('',#90250);
#15554=VERTEX_POINT('',#90482);
#15555=VERTEX_POINT('',#90483);
#15556=VERTEX_POINT('',#90946);
#15557=VERTEX_POINT('',#90947);
#15558=VERTEX_POINT('',#91390);
#15559=VERTEX_POINT('',#91391);
#15560=VERTEX_POINT('',#91393);
#15561=VERTEX_POINT('',#91630);
#15562=VERTEX_POINT('',#91866);
#15563=VERTEX_POINT('',#91867);
#15564=VERTEX_POINT('',#92310);
#15565=VERTEX_POINT('',#92311);
#15566=VERTEX_POINT('',#92784);
#15567=VERTEX_POINT('',#92785);
#15568=VERTEX_POINT('',#92787);
#15569=VERTEX_POINT('',#93044);
#15570=VERTEX_POINT('',#93290);
#15571=VERTEX_POINT('',#93291);
#15572=VERTEX_POINT('',#93760);
#15573=VERTEX_POINT('',#93761);
#15574=VERTEX_POINT('',#94224);
#15575=VERTEX_POINT('',#94225);
#15576=VERTEX_POINT('',#94227);
#15577=VERTEX_POINT('',#94685);
#15578=VERTEX_POINT('',#94686);
#15579=VERTEX_POINT('',#94688);
#15580=VERTEX_POINT('',#94803);
#15581=VERTEX_POINT('',#94888);
#15582=VERTEX_POINT('',#94889);
#15583=VERTEX_POINT('',#95362);
#15584=VERTEX_POINT('',#95363);
#15585=VERTEX_POINT('',#95792);
#15586=VERTEX_POINT('',#95793);
#15587=VERTEX_POINT('',#96220);
#15588=VERTEX_POINT('',#96221);
#15589=VERTEX_POINT('',#96223);
#15590=VERTEX_POINT('',#96663);
#15591=VERTEX_POINT('',#96664);
#15592=VERTEX_POINT('',#96886);
#15593=VERTEX_POINT('',#97104);
#15594=VERTEX_POINT('',#97105);
#15595=VERTEX_POINT('',#97546);
#15596=VERTEX_POINT('',#97547);
#15597=VERTEX_POINT('',#97970);
#15598=VERTEX_POINT('',#97971);
#15599=VERTEX_POINT('',#98396);
#15600=VERTEX_POINT('',#98397);
#15601=VERTEX_POINT('',#98844);
#15602=VERTEX_POINT('',#98845);
#15603=VERTEX_POINT('',#99302);
#15604=VERTEX_POINT('',#99303);
#15605=VERTEX_POINT('',#99728);
#15606=VERTEX_POINT('',#99729);
#15607=VERTEX_POINT('',#100160);
#15608=VERTEX_POINT('',#100161);
#15609=VERTEX_POINT('',#100584);
#15610=VERTEX_POINT('',#100585);
#15611=VERTEX_POINT('',#100587);
#15612=VERTEX_POINT('',#101041);
#15613=VERTEX_POINT('',#101042);
#15614=VERTEX_POINT('',#101459);
#15615=VERTEX_POINT('',#101460);
#15616=VERTEX_POINT('',#101883);
#15617=VERTEX_POINT('',#101884);
#15618=VERTEX_POINT('',#102319);
#15619=VERTEX_POINT('',#102320);
#15620=VERTEX_POINT('',#102737);
#15621=VERTEX_POINT('',#102738);
#15622=VERTEX_POINT('',#103175);
#15623=VERTEX_POINT('',#103176);
#15624=VERTEX_POINT('',#103398);
#15625=VERTEX_POINT('',#103634);
#15626=VERTEX_POINT('',#103635);
#15627=VERTEX_POINT('',#104048);
#15628=VERTEX_POINT('',#104049);
#15629=VERTEX_POINT('',#104514);
#15630=VERTEX_POINT('',#104701);
#15631=VERTEX_POINT('',#104703);
#15632=VERTEX_POINT('',#104834);
#15633=VERTEX_POINT('',#105071);
#15634=VERTEX_POINT('',#105240);
#15635=VERTEX_POINT('',#105241);
#15636=VERTEX_POINT('',#105962);
#15637=VERTEX_POINT('',#105963);
#15638=VERTEX_POINT('',#106656);
#15639=VERTEX_POINT('',#106660);
#15640=VERTEX_POINT('',#106663);
#15641=VERTEX_POINT('',#106668);
#15642=VERTEX_POINT('',#106669);
#15643=VERTEX_POINT('',#106671);
#15644=VERTEX_POINT('',#106675);
#15645=VERTEX_POINT('',#106677);
#15646=VERTEX_POINT('',#106683);
#15647=VERTEX_POINT('',#106689);
#15648=VERTEX_POINT('',#106690);
#15649=VERTEX_POINT('',#106692);
#15650=VERTEX_POINT('',#106694);
#15651=VERTEX_POINT('',#106697);
#15652=VERTEX_POINT('',#106699);
#15653=VERTEX_POINT('',#106701);
#15654=VERTEX_POINT('',#106703);
#15655=VERTEX_POINT('',#106705);
#15656=VERTEX_POINT('',#106707);
#15657=VERTEX_POINT('',#106709);
#15658=VERTEX_POINT('',#106711);
#15659=VERTEX_POINT('',#106713);
#15660=VERTEX_POINT('',#106715);
#15661=VERTEX_POINT('',#106717);
#15662=VERTEX_POINT('',#106719);
#15663=VERTEX_POINT('',#106721);
#15664=VERTEX_POINT('',#106723);
#15665=VERTEX_POINT('',#106725);
#15666=VERTEX_POINT('',#106727);
#15667=VERTEX_POINT('',#106729);
#15668=VERTEX_POINT('',#106731);
#15669=VERTEX_POINT('',#106733);
#15670=VERTEX_POINT('',#106735);
#15671=VERTEX_POINT('',#106737);
#15672=VERTEX_POINT('',#106739);
#15673=VERTEX_POINT('',#106741);
#15674=VERTEX_POINT('',#106743);
#15675=VERTEX_POINT('',#106745);
#15676=VERTEX_POINT('',#106747);
#15677=VERTEX_POINT('',#106749);
#15678=VERTEX_POINT('',#106751);
#15679=VERTEX_POINT('',#106753);
#15680=VERTEX_POINT('',#106755);
#15681=VERTEX_POINT('',#106757);
#15682=VERTEX_POINT('',#106759);
#15683=VERTEX_POINT('',#106761);
#15684=VERTEX_POINT('',#106763);
#15685=VERTEX_POINT('',#106765);
#15686=VERTEX_POINT('',#106767);
#15687=VERTEX_POINT('',#106769);
#15688=VERTEX_POINT('',#106771);
#15689=VERTEX_POINT('',#106773);
#15690=VERTEX_POINT('',#106775);
#15691=VERTEX_POINT('',#106777);
#15692=VERTEX_POINT('',#106779);
#15693=VERTEX_POINT('',#106781);
#15694=VERTEX_POINT('',#106783);
#15695=VERTEX_POINT('',#106785);
#15696=VERTEX_POINT('',#106787);
#15697=VERTEX_POINT('',#106789);
#15698=VERTEX_POINT('',#106791);
#15699=VERTEX_POINT('',#106793);
#15700=VERTEX_POINT('',#106795);
#15701=VERTEX_POINT('',#106797);
#15702=VERTEX_POINT('',#106799);
#15703=VERTEX_POINT('',#106801);
#15704=VERTEX_POINT('',#106803);
#15705=VERTEX_POINT('',#106805);
#15706=VERTEX_POINT('',#106807);
#15707=VERTEX_POINT('',#106809);
#15708=VERTEX_POINT('',#106811);
#15709=VERTEX_POINT('',#106813);
#15710=VERTEX_POINT('',#106815);
#15711=VERTEX_POINT('',#106817);
#15712=VERTEX_POINT('',#106819);
#15713=VERTEX_POINT('',#106821);
#15714=VERTEX_POINT('',#106823);
#15715=VERTEX_POINT('',#106825);
#15716=VERTEX_POINT('',#106827);
#15717=VERTEX_POINT('',#106830);
#15718=VERTEX_POINT('',#106832);
#15719=VERTEX_POINT('',#106834);
#15720=VERTEX_POINT('',#106836);
#15721=VERTEX_POINT('',#106838);
#15722=VERTEX_POINT('',#106840);
#15723=VERTEX_POINT('',#106842);
#15724=VERTEX_POINT('',#106844);
#15725=VERTEX_POINT('',#106846);
#15726=VERTEX_POINT('',#106848);
#15727=VERTEX_POINT('',#106850);
#15728=VERTEX_POINT('',#106852);
#15729=VERTEX_POINT('',#106854);
#15730=VERTEX_POINT('',#106856);
#15731=VERTEX_POINT('',#106858);
#15732=VERTEX_POINT('',#106860);
#15733=VERTEX_POINT('',#106862);
#15734=VERTEX_POINT('',#106864);
#15735=VERTEX_POINT('',#106866);
#15736=VERTEX_POINT('',#106868);
#15737=VERTEX_POINT('',#106870);
#15738=VERTEX_POINT('',#106872);
#15739=VERTEX_POINT('',#106874);
#15740=VERTEX_POINT('',#106876);
#15741=VERTEX_POINT('',#106878);
#15742=VERTEX_POINT('',#106880);
#15743=VERTEX_POINT('',#106882);
#15744=VERTEX_POINT('',#106884);
#15745=VERTEX_POINT('',#106886);
#15746=VERTEX_POINT('',#106888);
#15747=VERTEX_POINT('',#106890);
#15748=VERTEX_POINT('',#106892);
#15749=VERTEX_POINT('',#106894);
#15750=VERTEX_POINT('',#106896);
#15751=VERTEX_POINT('',#106898);
#15752=VERTEX_POINT('',#106900);
#15753=VERTEX_POINT('',#106902);
#15754=VERTEX_POINT('',#106904);
#15755=VERTEX_POINT('',#106906);
#15756=VERTEX_POINT('',#106908);
#15757=VERTEX_POINT('',#106910);
#15758=VERTEX_POINT('',#106912);
#15759=VERTEX_POINT('',#106914);
#15760=VERTEX_POINT('',#106916);
#15761=VERTEX_POINT('',#106918);
#15762=VERTEX_POINT('',#106920);
#15763=VERTEX_POINT('',#106922);
#15764=VERTEX_POINT('',#106924);
#15765=VERTEX_POINT('',#106926);
#15766=VERTEX_POINT('',#106928);
#15767=VERTEX_POINT('',#106930);
#15768=VERTEX_POINT('',#106932);
#15769=VERTEX_POINT('',#106934);
#15770=VERTEX_POINT('',#106936);
#15771=VERTEX_POINT('',#106938);
#15772=VERTEX_POINT('',#106940);
#15773=VERTEX_POINT('',#106942);
#15774=VERTEX_POINT('',#106944);
#15775=VERTEX_POINT('',#106946);
#15776=VERTEX_POINT('',#106948);
#15777=VERTEX_POINT('',#106950);
#15778=VERTEX_POINT('',#106952);
#15779=VERTEX_POINT('',#106954);
#15780=VERTEX_POINT('',#106956);
#15781=VERTEX_POINT('',#106958);
#15782=VERTEX_POINT('',#106960);
#15783=VERTEX_POINT('',#106962);
#15784=VERTEX_POINT('',#106964);
#15785=VERTEX_POINT('',#106966);
#15786=VERTEX_POINT('',#106968);
#15787=VERTEX_POINT('',#106970);
#15788=VERTEX_POINT('',#106972);
#15789=VERTEX_POINT('',#106974);
#15790=VERTEX_POINT('',#106978);
#15791=VERTEX_POINT('',#106980);
#15792=VERTEX_POINT('',#106992);
#15793=VERTEX_POINT('',#106996);
#15794=VERTEX_POINT('',#107003);
#15795=VERTEX_POINT('',#107010);
#15796=VERTEX_POINT('',#107017);
#15797=VERTEX_POINT('',#107024);
#15798=VERTEX_POINT('',#107031);
#15799=VERTEX_POINT('',#107038);
#15800=VERTEX_POINT('',#107045);
#15801=VERTEX_POINT('',#107052);
#15802=VERTEX_POINT('',#107059);
#15803=VERTEX_POINT('',#107066);
#15804=VERTEX_POINT('',#107073);
#15805=VERTEX_POINT('',#107080);
#15806=VERTEX_POINT('',#107087);
#15807=VERTEX_POINT('',#107094);
#15808=VERTEX_POINT('',#107101);
#15809=VERTEX_POINT('',#107108);
#15810=VERTEX_POINT('',#107115);
#15811=VERTEX_POINT('',#107122);
#15812=VERTEX_POINT('',#107129);
#15813=VERTEX_POINT('',#107136);
#15814=VERTEX_POINT('',#107143);
#15815=VERTEX_POINT('',#107150);
#15816=VERTEX_POINT('',#107157);
#15817=VERTEX_POINT('',#107164);
#15818=VERTEX_POINT('',#107171);
#15819=VERTEX_POINT('',#107178);
#15820=VERTEX_POINT('',#107185);
#15821=VERTEX_POINT('',#107192);
#15822=VERTEX_POINT('',#107199);
#15823=VERTEX_POINT('',#107206);
#15824=VERTEX_POINT('',#107213);
#15825=VERTEX_POINT('',#107220);
#15826=VERTEX_POINT('',#107230);
#15827=VERTEX_POINT('',#107234);
#15828=VERTEX_POINT('',#107241);
#15829=VERTEX_POINT('',#107248);
#15830=VERTEX_POINT('',#107255);
#15831=VERTEX_POINT('',#107262);
#15832=VERTEX_POINT('',#107269);
#15833=VERTEX_POINT('',#107276);
#15834=VERTEX_POINT('',#107283);
#15835=VERTEX_POINT('',#107290);
#15836=VERTEX_POINT('',#107297);
#15837=VERTEX_POINT('',#107304);
#15838=VERTEX_POINT('',#107311);
#15839=VERTEX_POINT('',#107318);
#15840=VERTEX_POINT('',#107325);
#15841=VERTEX_POINT('',#107332);
#15842=VERTEX_POINT('',#107339);
#15843=VERTEX_POINT('',#107346);
#15844=VERTEX_POINT('',#107353);
#15845=VERTEX_POINT('',#107360);
#15846=VERTEX_POINT('',#107367);
#15847=VERTEX_POINT('',#107374);
#15848=VERTEX_POINT('',#107381);
#15849=VERTEX_POINT('',#107388);
#15850=VERTEX_POINT('',#107395);
#15851=VERTEX_POINT('',#107402);
#15852=VERTEX_POINT('',#107409);
#15853=VERTEX_POINT('',#107416);
#15854=VERTEX_POINT('',#107423);
#15855=VERTEX_POINT('',#107430);
#15856=VERTEX_POINT('',#107437);
#15857=VERTEX_POINT('',#107444);
#15858=VERTEX_POINT('',#107451);
#15859=VERTEX_POINT('',#107458);
#15860=VERTEX_POINT('',#107465);
#15861=VERTEX_POINT('',#107474);
#15862=VERTEX_POINT('',#107477);
#15863=VERTEX_POINT('',#107478);
#15864=VERTEX_POINT('',#107482);
#15865=VERTEX_POINT('',#107484);
#15866=VERTEX_POINT('',#107488);
#15867=VERTEX_POINT('',#107492);
#15868=VERTEX_POINT('',#107494);
#15869=VERTEX_POINT('',#107498);
#15870=VERTEX_POINT('',#107502);
#15871=VERTEX_POINT('',#107504);
#15872=VERTEX_POINT('',#107508);
#15873=VERTEX_POINT('',#107512);
#15874=VERTEX_POINT('',#107514);
#15875=VERTEX_POINT('',#107518);
#15876=VERTEX_POINT('',#107522);
#15877=VERTEX_POINT('',#107524);
#15878=VERTEX_POINT('',#107528);
#15879=VERTEX_POINT('',#107532);
#15880=VERTEX_POINT('',#107539);
#15881=VERTEX_POINT('',#107541);
#15882=VERTEX_POINT('',#107545);
#15883=VERTEX_POINT('',#107547);
#15884=VERTEX_POINT('',#107551);
#15885=VERTEX_POINT('',#107553);
#15886=VERTEX_POINT('',#107557);
#15887=VERTEX_POINT('',#107559);
#15888=VERTEX_POINT('',#107563);
#15889=VERTEX_POINT('',#107565);
#15890=VERTEX_POINT('',#107569);
#15891=VERTEX_POINT('',#107571);
#15892=VERTEX_POINT('',#107576);
#15893=VERTEX_POINT('',#107578);
#15894=VERTEX_POINT('',#107583);
#15895=VERTEX_POINT('',#107588);
#15896=VERTEX_POINT('',#107601);
#15897=VERTEX_POINT('',#107602);
#15898=VERTEX_POINT('',#107618);
#19742=EDGE_CURVE('',#15512,#15513,#9362,.T.);
#19743=EDGE_CURVE('',#15512,#15514,#1429,.T.);
#19744=EDGE_CURVE('',#15515,#15514,#13011,.T.);
#19745=EDGE_CURVE('',#15515,#15513,#1430,.T.);
#19746=EDGE_CURVE('',#15516,#15517,#9363,.T.);
#19747=EDGE_CURVE('',#15516,#15512,#1431,.T.);
#19748=EDGE_CURVE('',#15513,#15517,#1432,.T.);
#19749=EDGE_CURVE('',#15518,#15519,#9364,.T.);
#19750=EDGE_CURVE('',#15518,#15516,#1433,.T.);
#19751=EDGE_CURVE('',#15517,#15519,#1434,.T.);
#19752=EDGE_CURVE('',#15520,#15521,#9365,.T.);
#19753=EDGE_CURVE('',#15520,#15522,#1435,.T.);
#19754=EDGE_CURVE('',#15522,#15518,#1436,.T.);
#19755=EDGE_CURVE('',#15519,#15523,#1437,.T.);
#19756=EDGE_CURVE('',#15523,#15521,#1438,.T.);
#19757=EDGE_CURVE('',#15524,#15525,#9366,.T.);
#19758=EDGE_CURVE('',#15524,#15520,#1439,.T.);
#19759=EDGE_CURVE('',#15521,#15525,#1440,.T.);
#19760=EDGE_CURVE('',#15526,#15527,#9367,.T.);
#19761=EDGE_CURVE('',#15526,#15524,#1441,.T.);
#19762=EDGE_CURVE('',#15525,#15527,#1442,.T.);
#19763=EDGE_CURVE('',#15528,#15529,#9368,.T.);
#19764=EDGE_CURVE('',#15528,#15530,#1443,.T.);
#19765=EDGE_CURVE('',#15530,#15526,#1444,.T.);
#19766=EDGE_CURVE('',#15527,#15531,#1445,.T.);
#19767=EDGE_CURVE('',#15531,#15529,#1446,.T.);
#19768=EDGE_CURVE('',#15532,#15533,#9369,.T.);
#19769=EDGE_CURVE('',#15532,#15534,#1447,.T.);
#19770=EDGE_CURVE('',#15534,#15528,#1448,.T.);
#19771=EDGE_CURVE('',#15529,#15535,#1449,.T.);
#19772=EDGE_CURVE('',#15535,#15533,#1450,.T.);
#19773=EDGE_CURVE('',#15536,#15537,#9370,.T.);
#19774=EDGE_CURVE('',#15536,#15532,#1451,.T.);
#19775=EDGE_CURVE('',#15533,#15537,#1452,.T.);
#19776=EDGE_CURVE('',#15538,#15539,#9371,.T.);
#19777=EDGE_CURVE('',#15538,#15536,#1453,.T.);
#19778=EDGE_CURVE('',#15537,#15539,#1454,.T.);
#19779=EDGE_CURVE('',#15540,#15541,#9372,.T.);
#19780=EDGE_CURVE('',#15540,#15542,#1455,.T.);
#19781=EDGE_CURVE('',#15542,#15538,#1456,.T.);
#19782=EDGE_CURVE('',#15539,#15543,#1457,.T.);
#19783=EDGE_CURVE('',#15543,#15541,#1458,.T.);
#19784=EDGE_CURVE('',#15544,#15545,#9373,.T.);
#19785=EDGE_CURVE('',#15544,#15540,#1459,.T.);
#19786=EDGE_CURVE('',#15541,#15545,#1460,.T.);
#19787=EDGE_CURVE('',#15546,#15547,#9374,.T.);
#19788=EDGE_CURVE('',#15546,#15548,#1461,.T.);
#19789=EDGE_CURVE('',#15548,#15544,#1462,.T.);
#19790=EDGE_CURVE('',#15545,#15549,#1463,.T.);
#19791=EDGE_CURVE('',#15549,#15547,#1464,.T.);
#19792=EDGE_CURVE('',#15550,#15551,#9375,.T.);
#19793=EDGE_CURVE('',#15550,#15552,#1465,.T.);
#19794=EDGE_CURVE('',#15552,#15546,#1466,.T.);
#19795=EDGE_CURVE('',#15547,#15553,#1467,.T.);
#19796=EDGE_CURVE('',#15553,#15551,#1468,.T.);
#19797=EDGE_CURVE('',#15554,#15555,#9376,.T.);
#19798=EDGE_CURVE('',#15554,#15550,#1469,.T.);
#19799=EDGE_CURVE('',#15551,#15555,#1470,.T.);
#19800=EDGE_CURVE('',#15556,#15557,#9377,.T.);
#19801=EDGE_CURVE('',#15556,#15554,#1471,.T.);
#19802=EDGE_CURVE('',#15555,#15557,#1472,.T.);
#19803=EDGE_CURVE('',#15558,#15559,#9378,.T.);
#19804=EDGE_CURVE('',#15558,#15560,#1473,.T.);
#19805=EDGE_CURVE('',#15560,#15556,#1474,.T.);
#19806=EDGE_CURVE('',#15557,#15561,#1475,.T.);
#19807=EDGE_CURVE('',#15561,#15559,#1476,.T.);
#19808=EDGE_CURVE('',#15562,#15563,#9379,.T.);
#19809=EDGE_CURVE('',#15562,#15558,#1477,.T.);
#19810=EDGE_CURVE('',#15559,#15563,#1478,.T.);
#19811=EDGE_CURVE('',#15564,#15565,#9380,.T.);
#19812=EDGE_CURVE('',#15564,#15562,#1479,.T.);
#19813=EDGE_CURVE('',#15563,#15565,#1480,.T.);
#19814=EDGE_CURVE('',#15566,#15567,#9381,.T.);
#19815=EDGE_CURVE('',#15566,#15568,#1481,.T.);
#19816=EDGE_CURVE('',#15568,#15564,#1482,.T.);
#19817=EDGE_CURVE('',#15565,#15569,#1483,.T.);
#19818=EDGE_CURVE('',#15569,#15567,#1484,.T.);
#19819=EDGE_CURVE('',#15570,#15571,#9382,.T.);
#19820=EDGE_CURVE('',#15570,#15566,#1485,.T.);
#19821=EDGE_CURVE('',#15567,#15571,#1486,.T.);
#19822=EDGE_CURVE('',#15572,#15573,#9383,.T.);
#19823=EDGE_CURVE('',#15572,#15570,#1487,.T.);
#19824=EDGE_CURVE('',#15571,#15573,#1488,.T.);
#19825=EDGE_CURVE('',#15574,#15575,#9384,.T.);
#19826=EDGE_CURVE('',#15574,#15576,#1489,.T.);
#19827=EDGE_CURVE('',#15576,#15572,#1490,.T.);
#19828=EDGE_CURVE('',#15573,#15575,#1491,.T.);
#19829=EDGE_CURVE('',#15577,#15578,#9385,.T.);
#19830=EDGE_CURVE('',#15579,#15577,#1492,.F.);
#19831=EDGE_CURVE('',#15580,#15579,#13012,.T.);
#19832=EDGE_CURVE('',#15580,#15578,#1493,.T.);
#19833=EDGE_CURVE('',#15581,#15582,#9386,.T.);
#19834=EDGE_CURVE('',#15577,#15581,#1494,.F.);
#19835=EDGE_CURVE('',#15578,#15582,#1495,.T.);
#19836=EDGE_CURVE('',#15583,#15584,#9387,.T.);
#19837=EDGE_CURVE('',#15581,#15583,#1496,.F.);
#19838=EDGE_CURVE('',#15582,#15584,#1497,.T.);
#19839=EDGE_CURVE('',#15585,#15586,#9388,.T.);
#19840=EDGE_CURVE('',#15583,#15585,#1498,.F.);
#19841=EDGE_CURVE('',#15584,#15586,#1499,.T.);
#19842=EDGE_CURVE('',#15587,#15588,#9389,.T.);
#19843=EDGE_CURVE('',#15589,#15587,#1500,.F.);
#19844=EDGE_CURVE('',#15585,#15589,#1501,.F.);
#19845=EDGE_CURVE('',#15586,#15588,#1502,.T.);
#19846=EDGE_CURVE('',#15590,#15591,#9390,.T.);
#19847=EDGE_CURVE('',#15587,#15590,#1503,.F.);
#19848=EDGE_CURVE('',#15588,#15592,#1504,.T.);
#19849=EDGE_CURVE('',#15592,#15591,#1505,.T.);
#19850=EDGE_CURVE('',#15593,#15594,#9391,.T.);
#19851=EDGE_CURVE('',#15590,#15593,#1506,.F.);
#19852=EDGE_CURVE('',#15591,#15594,#1507,.T.);
#19853=EDGE_CURVE('',#15595,#15596,#9392,.T.);
#19854=EDGE_CURVE('',#15593,#15595,#1508,.F.);
#19855=EDGE_CURVE('',#15594,#15596,#1509,.T.);
#19856=EDGE_CURVE('',#15597,#15598,#9393,.T.);
#19857=EDGE_CURVE('',#15595,#15597,#1510,.F.);
#19858=EDGE_CURVE('',#15596,#15598,#1511,.T.);
#19859=EDGE_CURVE('',#15599,#15600,#9394,.T.);
#19860=EDGE_CURVE('',#15597,#15599,#1512,.F.);
#19861=EDGE_CURVE('',#15598,#15600,#1513,.T.);
#19862=EDGE_CURVE('',#15601,#15602,#9395,.T.);
#19863=EDGE_CURVE('',#15599,#15601,#1514,.F.);
#19864=EDGE_CURVE('',#15600,#15602,#1515,.T.);
#19865=EDGE_CURVE('',#15603,#15604,#9396,.T.);
#19866=EDGE_CURVE('',#15601,#15603,#1516,.F.);
#19867=EDGE_CURVE('',#15602,#15604,#1517,.T.);
#19868=EDGE_CURVE('',#15605,#15606,#9397,.T.);
#19869=EDGE_CURVE('',#15603,#15605,#1518,.F.);
#19870=EDGE_CURVE('',#15604,#15606,#1519,.T.);
#19871=EDGE_CURVE('',#15607,#15608,#9398,.T.);
#19872=EDGE_CURVE('',#15605,#15607,#1520,.F.);
#19873=EDGE_CURVE('',#15606,#15608,#1521,.T.);
#19874=EDGE_CURVE('',#15609,#15610,#9399,.T.);
#19875=EDGE_CURVE('',#15611,#15609,#1522,.F.);
#19876=EDGE_CURVE('',#15607,#15611,#1523,.F.);
#19877=EDGE_CURVE('',#15608,#15610,#1524,.T.);
#19878=EDGE_CURVE('',#15612,#15613,#9400,.T.);
#19879=EDGE_CURVE('',#15609,#15612,#1525,.F.);
#19880=EDGE_CURVE('',#15610,#15613,#1526,.T.);
#19881=EDGE_CURVE('',#15614,#15615,#9401,.T.);
#19882=EDGE_CURVE('',#15612,#15614,#1527,.F.);
#19883=EDGE_CURVE('',#15613,#15615,#1528,.T.);
#19884=EDGE_CURVE('',#15616,#15617,#9402,.T.);
#19885=EDGE_CURVE('',#15614,#15616,#1529,.F.);
#19886=EDGE_CURVE('',#15615,#15617,#1530,.T.);
#19887=EDGE_CURVE('',#15618,#15619,#9403,.T.);
#19888=EDGE_CURVE('',#15616,#15618,#1531,.F.);
#19889=EDGE_CURVE('',#15617,#15619,#1532,.T.);
#19890=EDGE_CURVE('',#15620,#15621,#9404,.T.);
#19891=EDGE_CURVE('',#15618,#15620,#1533,.F.);
#19892=EDGE_CURVE('',#15619,#15621,#1534,.T.);
#19893=EDGE_CURVE('',#15622,#15623,#9405,.T.);
#19894=EDGE_CURVE('',#15620,#15622,#1535,.F.);
#19895=EDGE_CURVE('',#15621,#15624,#1536,.T.);
#19896=EDGE_CURVE('',#15624,#15623,#1537,.T.);
#19897=EDGE_CURVE('',#15625,#15626,#9406,.T.);
#19898=EDGE_CURVE('',#15622,#15625,#1538,.F.);
#19899=EDGE_CURVE('',#15623,#15626,#1539,.T.);
#19900=EDGE_CURVE('',#15627,#15628,#9407,.T.);
#19901=EDGE_CURVE('',#15625,#15627,#1540,.F.);
#19902=EDGE_CURVE('',#15626,#15628,#1541,.T.);
#19903=EDGE_CURVE('',#15628,#15629,#1542,.T.);
#19904=EDGE_CURVE('',#15630,#15629,#13013,.T.);
#19905=EDGE_CURVE('',#15631,#15630,#1543,.T.);
#19906=EDGE_CURVE('',#15627,#15631,#1544,.T.);
#19907=EDGE_CURVE('',#15575,#15632,#1545,.T.);
#19908=EDGE_CURVE('',#15633,#15632,#13014,.T.);
#19909=EDGE_CURVE('',#15633,#15574,#1546,.T.);
#19910=EDGE_CURVE('',#15634,#15635,#13015,.T.);
#19911=EDGE_CURVE('',#15634,#15630,#1547,.T.);
#19912=EDGE_CURVE('',#15629,#15633,#1548,.T.);
#19913=EDGE_CURVE('',#15635,#15633,#13016,.T.);
#19914=EDGE_CURVE('',#15632,#15634,#1549,.T.);
#19915=EDGE_CURVE('',#15579,#15515,#1550,.F.);
#19916=EDGE_CURVE('',#15636,#15637,#13017,.T.);
#19917=EDGE_CURVE('',#15636,#15580,#1551,.T.);
#19918=EDGE_CURVE('',#15637,#15515,#13018,.T.);
#19919=EDGE_CURVE('',#15514,#15636,#1552,.T.);
#19920=EDGE_CURVE('',#15638,#15638,#13019,.T.);
#19921=EDGE_CURVE('',#15638,#15637,#13020,.T.);
#19922=EDGE_CURVE('',#15639,#15639,#13021,.T.);
#19923=EDGE_CURVE('',#15635,#15640,#9408,.T.);
#19924=EDGE_CURVE('',#15640,#15640,#13022,.T.);
#19925=EDGE_CURVE('',#15641,#15642,#13023,.T.);
#19926=EDGE_CURVE('',#15643,#15641,#9409,.T.);
#19927=EDGE_CURVE('',#15642,#15643,#9410,.T.);
#19928=EDGE_CURVE('',#15642,#15644,#9411,.T.);
#19929=EDGE_CURVE('',#15645,#15643,#9412,.T.);
#19930=EDGE_CURVE('',#15644,#15645,#116,.T.);
#19931=EDGE_CURVE('',#15646,#15641,#9413,.T.);
#19932=EDGE_CURVE('',#15645,#15646,#117,.T.);
#19933=EDGE_CURVE('',#15647,#15648,#13024,.T.);
#19934=EDGE_CURVE('',#15648,#15649,#9414,.T.);
#19935=EDGE_CURVE('',#15650,#15649,#13025,.T.);
#19936=EDGE_CURVE('',#15649,#15650,#13026,.T.);
#19937=EDGE_CURVE('',#15648,#15651,#13027,.T.);
#19938=EDGE_CURVE('',#15651,#15652,#9415,.T.);
#19939=EDGE_CURVE('',#15653,#15652,#13028,.T.);
#19940=EDGE_CURVE('',#15653,#15654,#9416,.T.);
#19941=EDGE_CURVE('',#15654,#15655,#13029,.T.);
#19942=EDGE_CURVE('',#15655,#15656,#9417,.T.);
#19943=EDGE_CURVE('',#15657,#15656,#13030,.T.);
#19944=EDGE_CURVE('',#15657,#15658,#9418,.T.);
#19945=EDGE_CURVE('',#15658,#15659,#13031,.T.);
#19946=EDGE_CURVE('',#15659,#15660,#9419,.T.);
#19947=EDGE_CURVE('',#15661,#15660,#13032,.T.);
#19948=EDGE_CURVE('',#15661,#15662,#9420,.T.);
#19949=EDGE_CURVE('',#15662,#15663,#13033,.T.);
#19950=EDGE_CURVE('',#15663,#15664,#9421,.T.);
#19951=EDGE_CURVE('',#15665,#15664,#13034,.T.);
#19952=EDGE_CURVE('',#15665,#15666,#9422,.T.);
#19953=EDGE_CURVE('',#15666,#15667,#13035,.T.);
#19954=EDGE_CURVE('',#15667,#15668,#9423,.T.);
#19955=EDGE_CURVE('',#15669,#15668,#13036,.T.);
#19956=EDGE_CURVE('',#15669,#15670,#9424,.T.);
#19957=EDGE_CURVE('',#15670,#15671,#13037,.T.);
#19958=EDGE_CURVE('',#15671,#15672,#9425,.T.);
#19959=EDGE_CURVE('',#15673,#15672,#13038,.T.);
#19960=EDGE_CURVE('',#15673,#15674,#9426,.T.);
#19961=EDGE_CURVE('',#15674,#15675,#13039,.T.);
#19962=EDGE_CURVE('',#15675,#15676,#9427,.T.);
#19963=EDGE_CURVE('',#15677,#15676,#13040,.T.);
#19964=EDGE_CURVE('',#15677,#15678,#9428,.T.);
#19965=EDGE_CURVE('',#15678,#15679,#13041,.T.);
#19966=EDGE_CURVE('',#15679,#15680,#9429,.T.);
#19967=EDGE_CURVE('',#15681,#15680,#13042,.T.);
#19968=EDGE_CURVE('',#15681,#15682,#9430,.T.);
#19969=EDGE_CURVE('',#15682,#15683,#13043,.T.);
#19970=EDGE_CURVE('',#15683,#15684,#9431,.T.);
#19971=EDGE_CURVE('',#15685,#15684,#13044,.T.);
#19972=EDGE_CURVE('',#15685,#15686,#9432,.T.);
#19973=EDGE_CURVE('',#15686,#15687,#13045,.T.);
#19974=EDGE_CURVE('',#15687,#15688,#9433,.T.);
#19975=EDGE_CURVE('',#15689,#15688,#13046,.T.);
#19976=EDGE_CURVE('',#15689,#15690,#9434,.T.);
#19977=EDGE_CURVE('',#15690,#15691,#13047,.T.);
#19978=EDGE_CURVE('',#15691,#15692,#9435,.T.);
#19979=EDGE_CURVE('',#15693,#15692,#13048,.T.);
#19980=EDGE_CURVE('',#15693,#15694,#9436,.T.);
#19981=EDGE_CURVE('',#15694,#15695,#13049,.T.);
#19982=EDGE_CURVE('',#15695,#15696,#9437,.T.);
#19983=EDGE_CURVE('',#15697,#15696,#13050,.T.);
#19984=EDGE_CURVE('',#15697,#15698,#9438,.T.);
#19985=EDGE_CURVE('',#15698,#15699,#13051,.T.);
#19986=EDGE_CURVE('',#15699,#15700,#9439,.T.);
#19987=EDGE_CURVE('',#15701,#15700,#13052,.T.);
#19988=EDGE_CURVE('',#15701,#15702,#9440,.T.);
#19989=EDGE_CURVE('',#15702,#15703,#13053,.T.);
#19990=EDGE_CURVE('',#15703,#15704,#9441,.T.);
#19991=EDGE_CURVE('',#15705,#15704,#13054,.T.);
#19992=EDGE_CURVE('',#15705,#15706,#9442,.T.);
#19993=EDGE_CURVE('',#15706,#15707,#13055,.T.);
#19994=EDGE_CURVE('',#15707,#15708,#9443,.T.);
#19995=EDGE_CURVE('',#15709,#15708,#13056,.T.);
#19996=EDGE_CURVE('',#15709,#15710,#9444,.T.);
#19997=EDGE_CURVE('',#15710,#15711,#13057,.T.);
#19998=EDGE_CURVE('',#15711,#15712,#9445,.T.);
#19999=EDGE_CURVE('',#15713,#15712,#13058,.T.);
#20000=EDGE_CURVE('',#15713,#15714,#9446,.T.);
#20001=EDGE_CURVE('',#15714,#15715,#13059,.T.);
#20002=EDGE_CURVE('',#15715,#15716,#9447,.T.);
#20003=EDGE_CURVE('',#15646,#15716,#13060,.T.);
#20004=EDGE_CURVE('',#15717,#15644,#13061,.T.);
#20005=EDGE_CURVE('',#15717,#15718,#9448,.T.);
#20006=EDGE_CURVE('',#15718,#15719,#13062,.T.);
#20007=EDGE_CURVE('',#15719,#15720,#9449,.T.);
#20008=EDGE_CURVE('',#15721,#15720,#13063,.T.);
#20009=EDGE_CURVE('',#15721,#15722,#9450,.T.);
#20010=EDGE_CURVE('',#15722,#15723,#13064,.T.);
#20011=EDGE_CURVE('',#15723,#15724,#9451,.T.);
#20012=EDGE_CURVE('',#15725,#15724,#13065,.T.);
#20013=EDGE_CURVE('',#15725,#15726,#9452,.T.);
#20014=EDGE_CURVE('',#15726,#15727,#13066,.T.);
#20015=EDGE_CURVE('',#15727,#15728,#9453,.T.);
#20016=EDGE_CURVE('',#15729,#15728,#13067,.T.);
#20017=EDGE_CURVE('',#15729,#15730,#9454,.T.);
#20018=EDGE_CURVE('',#15730,#15731,#13068,.T.);
#20019=EDGE_CURVE('',#15731,#15732,#9455,.T.);
#20020=EDGE_CURVE('',#15733,#15732,#13069,.T.);
#20021=EDGE_CURVE('',#15733,#15734,#9456,.T.);
#20022=EDGE_CURVE('',#15734,#15735,#13070,.T.);
#20023=EDGE_CURVE('',#15735,#15736,#9457,.T.);
#20024=EDGE_CURVE('',#15737,#15736,#13071,.T.);
#20025=EDGE_CURVE('',#15737,#15738,#9458,.T.);
#20026=EDGE_CURVE('',#15738,#15739,#13072,.T.);
#20027=EDGE_CURVE('',#15739,#15740,#9459,.T.);
#20028=EDGE_CURVE('',#15741,#15740,#13073,.T.);
#20029=EDGE_CURVE('',#15741,#15742,#9460,.T.);
#20030=EDGE_CURVE('',#15742,#15743,#13074,.T.);
#20031=EDGE_CURVE('',#15743,#15744,#9461,.T.);
#20032=EDGE_CURVE('',#15745,#15744,#13075,.T.);
#20033=EDGE_CURVE('',#15745,#15746,#9462,.T.);
#20034=EDGE_CURVE('',#15746,#15747,#13076,.T.);
#20035=EDGE_CURVE('',#15747,#15748,#9463,.T.);
#20036=EDGE_CURVE('',#15749,#15748,#13077,.T.);
#20037=EDGE_CURVE('',#15749,#15750,#9464,.T.);
#20038=EDGE_CURVE('',#15750,#15751,#13078,.T.);
#20039=EDGE_CURVE('',#15751,#15752,#9465,.T.);
#20040=EDGE_CURVE('',#15753,#15752,#13079,.T.);
#20041=EDGE_CURVE('',#15753,#15754,#9466,.T.);
#20042=EDGE_CURVE('',#15754,#15755,#13080,.T.);
#20043=EDGE_CURVE('',#15755,#15756,#9467,.T.);
#20044=EDGE_CURVE('',#15757,#15756,#13081,.T.);
#20045=EDGE_CURVE('',#15757,#15758,#9468,.T.);
#20046=EDGE_CURVE('',#15758,#15759,#13082,.T.);
#20047=EDGE_CURVE('',#15759,#15760,#9469,.T.);
#20048=EDGE_CURVE('',#15761,#15760,#13083,.T.);
#20049=EDGE_CURVE('',#15761,#15762,#9470,.T.);
#20050=EDGE_CURVE('',#15762,#15763,#13084,.T.);
#20051=EDGE_CURVE('',#15763,#15764,#9471,.T.);
#20052=EDGE_CURVE('',#15765,#15764,#13085,.T.);
#20053=EDGE_CURVE('',#15765,#15766,#9472,.T.);
#20054=EDGE_CURVE('',#15766,#15767,#13086,.T.);
#20055=EDGE_CURVE('',#15767,#15768,#9473,.T.);
#20056=EDGE_CURVE('',#15769,#15768,#13087,.T.);
#20057=EDGE_CURVE('',#15769,#15770,#9474,.T.);
#20058=EDGE_CURVE('',#15770,#15771,#13088,.T.);
#20059=EDGE_CURVE('',#15771,#15772,#9475,.T.);
#20060=EDGE_CURVE('',#15773,#15772,#13089,.T.);
#20061=EDGE_CURVE('',#15773,#15774,#9476,.T.);
#20062=EDGE_CURVE('',#15774,#15775,#13090,.T.);
#20063=EDGE_CURVE('',#15775,#15776,#9477,.T.);
#20064=EDGE_CURVE('',#15777,#15776,#13091,.T.);
#20065=EDGE_CURVE('',#15777,#15778,#9478,.T.);
#20066=EDGE_CURVE('',#15778,#15779,#13092,.T.);
#20067=EDGE_CURVE('',#15779,#15780,#9479,.T.);
#20068=EDGE_CURVE('',#15781,#15780,#13093,.T.);
#20069=EDGE_CURVE('',#15781,#15782,#9480,.T.);
#20070=EDGE_CURVE('',#15782,#15783,#13094,.T.);
#20071=EDGE_CURVE('',#15783,#15784,#9481,.T.);
#20072=EDGE_CURVE('',#15785,#15784,#13095,.T.);
#20073=EDGE_CURVE('',#15785,#15786,#9482,.T.);
#20074=EDGE_CURVE('',#15786,#15787,#13096,.T.);
#20075=EDGE_CURVE('',#15787,#15788,#9483,.T.);
#20076=EDGE_CURVE('',#15789,#15788,#13097,.T.);
#20077=EDGE_CURVE('',#15789,#15647,#9484,.T.);
#20078=EDGE_CURVE('',#15715,#15790,#9485,.T.);
#20079=EDGE_CURVE('',#15791,#15790,#9486,.T.);
#20080=EDGE_CURVE('',#15716,#15791,#118,.T.);
#20081=EDGE_CURVE('',#15791,#15713,#119,.T.);
#20082=EDGE_CURVE('',#15790,#15714,#9487,.T.);
#20083=EDGE_CURVE('',#15792,#15789,#120,.T.);
#20084=EDGE_CURVE('',#15788,#15793,#121,.T.);
#20085=EDGE_CURVE('',#15793,#15785,#122,.T.);
#20086=EDGE_CURVE('',#15784,#15794,#123,.T.);
#20087=EDGE_CURVE('',#15794,#15781,#124,.T.);
#20088=EDGE_CURVE('',#15780,#15795,#125,.T.);
#20089=EDGE_CURVE('',#15795,#15777,#126,.T.);
#20090=EDGE_CURVE('',#15776,#15796,#127,.T.);
#20091=EDGE_CURVE('',#15796,#15773,#128,.T.);
#20092=EDGE_CURVE('',#15772,#15797,#129,.T.);
#20093=EDGE_CURVE('',#15797,#15769,#130,.T.);
#20094=EDGE_CURVE('',#15768,#15798,#131,.T.);
#20095=EDGE_CURVE('',#15798,#15765,#132,.T.);
#20096=EDGE_CURVE('',#15764,#15799,#133,.T.);
#20097=EDGE_CURVE('',#15799,#15761,#134,.T.);
#20098=EDGE_CURVE('',#15760,#15800,#135,.T.);
#20099=EDGE_CURVE('',#15800,#15757,#136,.T.);
#20100=EDGE_CURVE('',#15756,#15801,#137,.T.);
#20101=EDGE_CURVE('',#15801,#15753,#138,.T.);
#20102=EDGE_CURVE('',#15752,#15802,#139,.T.);
#20103=EDGE_CURVE('',#15802,#15749,#140,.T.);
#20104=EDGE_CURVE('',#15748,#15803,#141,.T.);
#20105=EDGE_CURVE('',#15803,#15745,#142,.T.);
#20106=EDGE_CURVE('',#15744,#15804,#143,.T.);
#20107=EDGE_CURVE('',#15804,#15741,#144,.T.);
#20108=EDGE_CURVE('',#15740,#15805,#145,.T.);
#20109=EDGE_CURVE('',#15805,#15737,#146,.T.);
#20110=EDGE_CURVE('',#15736,#15806,#147,.T.);
#20111=EDGE_CURVE('',#15806,#15733,#148,.T.);
#20112=EDGE_CURVE('',#15732,#15807,#149,.T.);
#20113=EDGE_CURVE('',#15807,#15729,#150,.T.);
#20114=EDGE_CURVE('',#15728,#15808,#151,.T.);
#20115=EDGE_CURVE('',#15808,#15725,#152,.T.);
#20116=EDGE_CURVE('',#15724,#15809,#153,.T.);
#20117=EDGE_CURVE('',#15809,#15721,#154,.T.);
#20118=EDGE_CURVE('',#15720,#15810,#155,.T.);
#20119=EDGE_CURVE('',#15810,#15717,#156,.T.);
#20120=EDGE_CURVE('',#15712,#15811,#157,.T.);
#20121=EDGE_CURVE('',#15811,#15709,#158,.T.);
#20122=EDGE_CURVE('',#15708,#15812,#159,.T.);
#20123=EDGE_CURVE('',#15812,#15705,#160,.T.);
#20124=EDGE_CURVE('',#15704,#15813,#161,.T.);
#20125=EDGE_CURVE('',#15813,#15701,#162,.T.);
#20126=EDGE_CURVE('',#15700,#15814,#163,.T.);
#20127=EDGE_CURVE('',#15814,#15697,#164,.T.);
#20128=EDGE_CURVE('',#15696,#15815,#165,.T.);
#20129=EDGE_CURVE('',#15815,#15693,#166,.T.);
#20130=EDGE_CURVE('',#15692,#15816,#167,.T.);
#20131=EDGE_CURVE('',#15816,#15689,#168,.T.);
#20132=EDGE_CURVE('',#15688,#15817,#169,.T.);
#20133=EDGE_CURVE('',#15817,#15685,#170,.T.);
#20134=EDGE_CURVE('',#15684,#15818,#171,.T.);
#20135=EDGE_CURVE('',#15818,#15681,#172,.T.);
#20136=EDGE_CURVE('',#15680,#15819,#173,.T.);
#20137=EDGE_CURVE('',#15819,#15677,#174,.T.);
#20138=EDGE_CURVE('',#15676,#15820,#175,.T.);
#20139=EDGE_CURVE('',#15820,#15673,#176,.T.);
#20140=EDGE_CURVE('',#15672,#15821,#177,.T.);
#20141=EDGE_CURVE('',#15821,#15669,#178,.T.);
#20142=EDGE_CURVE('',#15668,#15822,#179,.T.);
#20143=EDGE_CURVE('',#15822,#15665,#180,.T.);
#20144=EDGE_CURVE('',#15664,#15823,#181,.T.);
#20145=EDGE_CURVE('',#15823,#15661,#182,.T.);
#20146=EDGE_CURVE('',#15660,#15824,#183,.T.);
#20147=EDGE_CURVE('',#15824,#15657,#184,.T.);
#20148=EDGE_CURVE('',#15656,#15825,#185,.T.);
#20149=EDGE_CURVE('',#15825,#15653,#186,.T.);
#20150=EDGE_CURVE('',#15652,#15792,#187,.T.);
#20151=EDGE_CURVE('',#15792,#15826,#9488,.T.);
#20152=EDGE_CURVE('',#15826,#15826,#13098,.T.);
#20153=EDGE_CURVE('',#15827,#15710,#9489,.T.);
#20154=EDGE_CURVE('',#15711,#15827,#9490,.T.);
#20155=EDGE_CURVE('',#15811,#15827,#9491,.T.);
#20156=EDGE_CURVE('',#15707,#15828,#9492,.T.);
#20157=EDGE_CURVE('',#15812,#15828,#9493,.T.);
#20158=EDGE_CURVE('',#15828,#15706,#9494,.T.);
#20159=EDGE_CURVE('',#15829,#15702,#9495,.T.);
#20160=EDGE_CURVE('',#15703,#15829,#9496,.T.);
#20161=EDGE_CURVE('',#15813,#15829,#9497,.T.);
#20162=EDGE_CURVE('',#15699,#15830,#9498,.T.);
#20163=EDGE_CURVE('',#15814,#15830,#9499,.T.);
#20164=EDGE_CURVE('',#15830,#15698,#9500,.T.);
#20165=EDGE_CURVE('',#15831,#15694,#9501,.T.);
#20166=EDGE_CURVE('',#15695,#15831,#9502,.T.);
#20167=EDGE_CURVE('',#15815,#15831,#9503,.T.);
#20168=EDGE_CURVE('',#15691,#15832,#9504,.T.);
#20169=EDGE_CURVE('',#15816,#15832,#9505,.T.);
#20170=EDGE_CURVE('',#15832,#15690,#9506,.T.);
#20171=EDGE_CURVE('',#15833,#15686,#9507,.T.);
#20172=EDGE_CURVE('',#15687,#15833,#9508,.T.);
#20173=EDGE_CURVE('',#15817,#15833,#9509,.T.);
#20174=EDGE_CURVE('',#15683,#15834,#9510,.T.);
#20175=EDGE_CURVE('',#15818,#15834,#9511,.T.);
#20176=EDGE_CURVE('',#15834,#15682,#9512,.T.);
#20177=EDGE_CURVE('',#15835,#15678,#9513,.T.);
#20178=EDGE_CURVE('',#15679,#15835,#9514,.T.);
#20179=EDGE_CURVE('',#15819,#15835,#9515,.T.);
#20180=EDGE_CURVE('',#15675,#15836,#9516,.T.);
#20181=EDGE_CURVE('',#15820,#15836,#9517,.T.);
#20182=EDGE_CURVE('',#15836,#15674,#9518,.T.);
#20183=EDGE_CURVE('',#15837,#15670,#9519,.T.);
#20184=EDGE_CURVE('',#15671,#15837,#9520,.T.);
#20185=EDGE_CURVE('',#15821,#15837,#9521,.T.);
#20186=EDGE_CURVE('',#15667,#15838,#9522,.T.);
#20187=EDGE_CURVE('',#15822,#15838,#9523,.T.);
#20188=EDGE_CURVE('',#15838,#15666,#9524,.T.);
#20189=EDGE_CURVE('',#15839,#15662,#9525,.T.);
#20190=EDGE_CURVE('',#15663,#15839,#9526,.T.);
#20191=EDGE_CURVE('',#15823,#15839,#9527,.T.);
#20192=EDGE_CURVE('',#15659,#15840,#9528,.T.);
#20193=EDGE_CURVE('',#15824,#15840,#9529,.T.);
#20194=EDGE_CURVE('',#15840,#15658,#9530,.T.);
#20195=EDGE_CURVE('',#15841,#15654,#9531,.T.);
#20196=EDGE_CURVE('',#15655,#15841,#9532,.T.);
#20197=EDGE_CURVE('',#15825,#15841,#9533,.T.);
#20198=EDGE_CURVE('',#15651,#15842,#9534,.T.);
#20199=EDGE_CURVE('',#15792,#15842,#9535,.T.);
#20200=EDGE_CURVE('',#15842,#15647,#9536,.T.);
#20201=EDGE_CURVE('',#15843,#15786,#9537,.T.);
#20202=EDGE_CURVE('',#15787,#15843,#9538,.T.);
#20203=EDGE_CURVE('',#15793,#15843,#9539,.T.);
#20204=EDGE_CURVE('',#15783,#15844,#9540,.T.);
#20205=EDGE_CURVE('',#15794,#15844,#9541,.T.);
#20206=EDGE_CURVE('',#15844,#15782,#9542,.T.);
#20207=EDGE_CURVE('',#15845,#15778,#9543,.T.);
#20208=EDGE_CURVE('',#15779,#15845,#9544,.T.);
#20209=EDGE_CURVE('',#15795,#15845,#9545,.T.);
#20210=EDGE_CURVE('',#15775,#15846,#9546,.T.);
#20211=EDGE_CURVE('',#15796,#15846,#9547,.T.);
#20212=EDGE_CURVE('',#15846,#15774,#9548,.T.);
#20213=EDGE_CURVE('',#15847,#15770,#9549,.T.);
#20214=EDGE_CURVE('',#15771,#15847,#9550,.T.);
#20215=EDGE_CURVE('',#15797,#15847,#9551,.T.);
#20216=EDGE_CURVE('',#15767,#15848,#9552,.T.);
#20217=EDGE_CURVE('',#15798,#15848,#9553,.T.);
#20218=EDGE_CURVE('',#15848,#15766,#9554,.T.);
#20219=EDGE_CURVE('',#15849,#15762,#9555,.T.);
#20220=EDGE_CURVE('',#15763,#15849,#9556,.T.);
#20221=EDGE_CURVE('',#15799,#15849,#9557,.T.);
#20222=EDGE_CURVE('',#15759,#15850,#9558,.T.);
#20223=EDGE_CURVE('',#15800,#15850,#9559,.T.);
#20224=EDGE_CURVE('',#15850,#15758,#9560,.T.);
#20225=EDGE_CURVE('',#15851,#15754,#9561,.T.);
#20226=EDGE_CURVE('',#15755,#15851,#9562,.T.);
#20227=EDGE_CURVE('',#15801,#15851,#9563,.T.);
#20228=EDGE_CURVE('',#15751,#15852,#9564,.T.);
#20229=EDGE_CURVE('',#15802,#15852,#9565,.T.);
#20230=EDGE_CURVE('',#15852,#15750,#9566,.T.);
#20231=EDGE_CURVE('',#15853,#15746,#9567,.T.);
#20232=EDGE_CURVE('',#15747,#15853,#9568,.T.);
#20233=EDGE_CURVE('',#15803,#15853,#9569,.T.);
#20234=EDGE_CURVE('',#15743,#15854,#9570,.T.);
#20235=EDGE_CURVE('',#15804,#15854,#9571,.T.);
#20236=EDGE_CURVE('',#15854,#15742,#9572,.T.);
#20237=EDGE_CURVE('',#15855,#15738,#9573,.T.);
#20238=EDGE_CURVE('',#15739,#15855,#9574,.T.);
#20239=EDGE_CURVE('',#15805,#15855,#9575,.T.);
#20240=EDGE_CURVE('',#15735,#15856,#9576,.T.);
#20241=EDGE_CURVE('',#15806,#15856,#9577,.T.);
#20242=EDGE_CURVE('',#15856,#15734,#9578,.T.);
#20243=EDGE_CURVE('',#15857,#15730,#9579,.T.);
#20244=EDGE_CURVE('',#15731,#15857,#9580,.T.);
#20245=EDGE_CURVE('',#15807,#15857,#9581,.T.);
#20246=EDGE_CURVE('',#15727,#15858,#9582,.T.);
#20247=EDGE_CURVE('',#15808,#15858,#9583,.T.);
#20248=EDGE_CURVE('',#15858,#15726,#9584,.T.);
#20249=EDGE_CURVE('',#15859,#15722,#9585,.T.);
#20250=EDGE_CURVE('',#15723,#15859,#9586,.T.);
#20251=EDGE_CURVE('',#15809,#15859,#9587,.T.);
#20252=EDGE_CURVE('',#15719,#15860,#9588,.T.);
#20253=EDGE_CURVE('',#15810,#15860,#9589,.T.);
#20254=EDGE_CURVE('',#15860,#15718,#9590,.T.);
#20255=EDGE_CURVE('',#15639,#15650,#13099,.T.);
#20256=EDGE_CURVE('',#15861,#15861,#13100,.T.);
#20257=EDGE_CURVE('',#15862,#15863,#188,.T.);
#20258=EDGE_CURVE('',#15864,#15862,#13101,.T.);
#20259=EDGE_CURVE('',#15865,#15864,#189,.T.);
#20260=EDGE_CURVE('',#15866,#15865,#190,.T.);
#20261=EDGE_CURVE('',#15867,#15866,#13102,.T.);
#20262=EDGE_CURVE('',#15868,#15867,#191,.T.);
#20263=EDGE_CURVE('',#15869,#15868,#192,.T.);
#20264=EDGE_CURVE('',#15870,#15869,#13103,.T.);
#20265=EDGE_CURVE('',#15871,#15870,#193,.T.);
#20266=EDGE_CURVE('',#15872,#15871,#194,.T.);
#20267=EDGE_CURVE('',#15873,#15872,#13104,.T.);
#20268=EDGE_CURVE('',#15874,#15873,#195,.T.);
#20269=EDGE_CURVE('',#15875,#15874,#196,.T.);
#20270=EDGE_CURVE('',#15876,#15875,#13105,.T.);
#20271=EDGE_CURVE('',#15877,#15876,#197,.T.);
#20272=EDGE_CURVE('',#15878,#15877,#198,.T.);
#20273=EDGE_CURVE('',#15879,#15878,#13106,.T.);
#20274=EDGE_CURVE('',#15863,#15879,#199,.T.);
#20275=EDGE_CURVE('',#15863,#15861,#9591,.T.);
#20276=EDGE_CURVE('',#15879,#15880,#9592,.T.);
#20277=EDGE_CURVE('',#15881,#15878,#9593,.T.);
#20278=EDGE_CURVE('',#15880,#15881,#13107,.T.);
#20279=EDGE_CURVE('',#15882,#15875,#9594,.T.);
#20280=EDGE_CURVE('',#15883,#15882,#13108,.T.);
#20281=EDGE_CURVE('',#15876,#15883,#9595,.T.);
#20282=EDGE_CURVE('',#15864,#15884,#9596,.T.);
#20283=EDGE_CURVE('',#15885,#15862,#9597,.T.);
#20284=EDGE_CURVE('',#15884,#15885,#13109,.T.);
#20285=EDGE_CURVE('',#15886,#15872,#9598,.T.);
#20286=EDGE_CURVE('',#15887,#15886,#13110,.T.);
#20287=EDGE_CURVE('',#15873,#15887,#9599,.T.);
#20288=EDGE_CURVE('',#15867,#15888,#9600,.T.);
#20289=EDGE_CURVE('',#15889,#15866,#9601,.T.);
#20290=EDGE_CURVE('',#15888,#15889,#13111,.T.);
#20291=EDGE_CURVE('',#15890,#15869,#9602,.T.);
#20292=EDGE_CURVE('',#15891,#15890,#13112,.T.);
#20293=EDGE_CURVE('',#15870,#15891,#9603,.T.);
#20294=EDGE_CURVE('',#15889,#15888,#9604,.T.);
#20295=EDGE_CURVE('',#15865,#15892,#9605,.T.);
#20296=EDGE_CURVE('',#15892,#15893,#9606,.T.);
#20297=EDGE_CURVE('',#15868,#15893,#9607,.T.);
#20298=EDGE_CURVE('',#15885,#15884,#9608,.T.);
#20299=EDGE_CURVE('',#15863,#15894,#9609,.T.);
#20300=EDGE_CURVE('',#15894,#15892,#9610,.T.);
#20301=EDGE_CURVE('',#15881,#15880,#9611,.T.);
#20302=EDGE_CURVE('',#15877,#15895,#9612,.T.);
#20303=EDGE_CURVE('',#15895,#15894,#9613,.T.);
#20304=EDGE_CURVE('',#15882,#15883,#9614,.T.);
#20305=EDGE_CURVE('',#15886,#15887,#9615,.T.);
#20306=EDGE_CURVE('',#15890,#15891,#9616,.T.);
#20307=EDGE_CURVE('',#15896,#15897,#9617,.T.);
#20308=EDGE_CURVE('',#15897,#15896,#13113,.T.);
#20309=EDGE_CURVE('',#15897,#15895,#9618,.T.);
#20310=EDGE_CURVE('',#15895,#15897,#13114,.T.);
#20311=EDGE_CURVE('',#15894,#15895,#13115,.T.);
#20312=EDGE_CURVE('',#15892,#15894,#13116,.T.);
#20313=EDGE_CURVE('',#15893,#15892,#13117,.T.);
#20314=EDGE_CURVE('',#15893,#15896,#9619,.T.);
#20315=EDGE_CURVE('',#15896,#15893,#13118,.T.);
#20316=EDGE_CURVE('',#15898,#15894,#9620,.T.);
#20317=EDGE_CURVE('',#15871,#15896,#9621,.T.);
#20318=EDGE_CURVE('',#15874,#15897,#9622,.T.);
#27782=ORIENTED_EDGE('',*,*,#19742,.F.);
#27783=ORIENTED_EDGE('',*,*,#19743,.T.);
#27784=ORIENTED_EDGE('',*,*,#19744,.F.);
#27785=ORIENTED_EDGE('',*,*,#19745,.T.);
#27786=ORIENTED_EDGE('',*,*,#19746,.F.);
#27787=ORIENTED_EDGE('',*,*,#19747,.T.);
#27788=ORIENTED_EDGE('',*,*,#19742,.T.);
#27789=ORIENTED_EDGE('',*,*,#19748,.T.);
#27790=ORIENTED_EDGE('',*,*,#19749,.F.);
#27791=ORIENTED_EDGE('',*,*,#19750,.T.);
#27792=ORIENTED_EDGE('',*,*,#19746,.T.);
#27793=ORIENTED_EDGE('',*,*,#19751,.T.);
#27794=ORIENTED_EDGE('',*,*,#19752,.F.);
#27795=ORIENTED_EDGE('',*,*,#19753,.T.);
#27796=ORIENTED_EDGE('',*,*,#19754,.T.);
#27797=ORIENTED_EDGE('',*,*,#19749,.T.);
#27798=ORIENTED_EDGE('',*,*,#19755,.T.);
#27799=ORIENTED_EDGE('',*,*,#19756,.T.);
#27800=ORIENTED_EDGE('',*,*,#19757,.F.);
#27801=ORIENTED_EDGE('',*,*,#19758,.T.);
#27802=ORIENTED_EDGE('',*,*,#19752,.T.);
#27803=ORIENTED_EDGE('',*,*,#19759,.T.);
#27804=ORIENTED_EDGE('',*,*,#19760,.F.);
#27805=ORIENTED_EDGE('',*,*,#19761,.T.);
#27806=ORIENTED_EDGE('',*,*,#19757,.T.);
#27807=ORIENTED_EDGE('',*,*,#19762,.T.);
#27808=ORIENTED_EDGE('',*,*,#19763,.F.);
#27809=ORIENTED_EDGE('',*,*,#19764,.T.);
#27810=ORIENTED_EDGE('',*,*,#19765,.T.);
#27811=ORIENTED_EDGE('',*,*,#19760,.T.);
#27812=ORIENTED_EDGE('',*,*,#19766,.T.);
#27813=ORIENTED_EDGE('',*,*,#19767,.T.);
#27814=ORIENTED_EDGE('',*,*,#19768,.F.);
#27815=ORIENTED_EDGE('',*,*,#19769,.T.);
#27816=ORIENTED_EDGE('',*,*,#19770,.T.);
#27817=ORIENTED_EDGE('',*,*,#19763,.T.);
#27818=ORIENTED_EDGE('',*,*,#19771,.T.);
#27819=ORIENTED_EDGE('',*,*,#19772,.T.);
#27820=ORIENTED_EDGE('',*,*,#19773,.F.);
#27821=ORIENTED_EDGE('',*,*,#19774,.T.);
#27822=ORIENTED_EDGE('',*,*,#19768,.T.);
#27823=ORIENTED_EDGE('',*,*,#19775,.T.);
#27824=ORIENTED_EDGE('',*,*,#19776,.F.);
#27825=ORIENTED_EDGE('',*,*,#19777,.T.);
#27826=ORIENTED_EDGE('',*,*,#19773,.T.);
#27827=ORIENTED_EDGE('',*,*,#19778,.T.);
#27828=ORIENTED_EDGE('',*,*,#19779,.F.);
#27829=ORIENTED_EDGE('',*,*,#19780,.T.);
#27830=ORIENTED_EDGE('',*,*,#19781,.T.);
#27831=ORIENTED_EDGE('',*,*,#19776,.T.);
#27832=ORIENTED_EDGE('',*,*,#19782,.T.);
#27833=ORIENTED_EDGE('',*,*,#19783,.T.);
#27834=ORIENTED_EDGE('',*,*,#19784,.F.);
#27835=ORIENTED_EDGE('',*,*,#19785,.T.);
#27836=ORIENTED_EDGE('',*,*,#19779,.T.);
#27837=ORIENTED_EDGE('',*,*,#19786,.T.);
#27838=ORIENTED_EDGE('',*,*,#19787,.F.);
#27839=ORIENTED_EDGE('',*,*,#19788,.T.);
#27840=ORIENTED_EDGE('',*,*,#19789,.T.);
#27841=ORIENTED_EDGE('',*,*,#19784,.T.);
#27842=ORIENTED_EDGE('',*,*,#19790,.T.);
#27843=ORIENTED_EDGE('',*,*,#19791,.T.);
#27844=ORIENTED_EDGE('',*,*,#19792,.F.);
#27845=ORIENTED_EDGE('',*,*,#19793,.T.);
#27846=ORIENTED_EDGE('',*,*,#19794,.T.);
#27847=ORIENTED_EDGE('',*,*,#19787,.T.);
#27848=ORIENTED_EDGE('',*,*,#19795,.T.);
#27849=ORIENTED_EDGE('',*,*,#19796,.T.);
#27850=ORIENTED_EDGE('',*,*,#19797,.F.);
#27851=ORIENTED_EDGE('',*,*,#19798,.T.);
#27852=ORIENTED_EDGE('',*,*,#19792,.T.);
#27853=ORIENTED_EDGE('',*,*,#19799,.T.);
#27854=ORIENTED_EDGE('',*,*,#19800,.F.);
#27855=ORIENTED_EDGE('',*,*,#19801,.T.);
#27856=ORIENTED_EDGE('',*,*,#19797,.T.);
#27857=ORIENTED_EDGE('',*,*,#19802,.T.);
#27858=ORIENTED_EDGE('',*,*,#19803,.F.);
#27859=ORIENTED_EDGE('',*,*,#19804,.T.);
#27860=ORIENTED_EDGE('',*,*,#19805,.T.);
#27861=ORIENTED_EDGE('',*,*,#19800,.T.);
#27862=ORIENTED_EDGE('',*,*,#19806,.T.);
#27863=ORIENTED_EDGE('',*,*,#19807,.T.);
#27864=ORIENTED_EDGE('',*,*,#19808,.F.);
#27865=ORIENTED_EDGE('',*,*,#19809,.T.);
#27866=ORIENTED_EDGE('',*,*,#19803,.T.);
#27867=ORIENTED_EDGE('',*,*,#19810,.T.);
#27868=ORIENTED_EDGE('',*,*,#19811,.F.);
#27869=ORIENTED_EDGE('',*,*,#19812,.T.);
#27870=ORIENTED_EDGE('',*,*,#19808,.T.);
#27871=ORIENTED_EDGE('',*,*,#19813,.T.);
#27872=ORIENTED_EDGE('',*,*,#19814,.F.);
#27873=ORIENTED_EDGE('',*,*,#19815,.T.);
#27874=ORIENTED_EDGE('',*,*,#19816,.T.);
#27875=ORIENTED_EDGE('',*,*,#19811,.T.);
#27876=ORIENTED_EDGE('',*,*,#19817,.T.);
#27877=ORIENTED_EDGE('',*,*,#19818,.T.);
#27878=ORIENTED_EDGE('',*,*,#19819,.F.);
#27879=ORIENTED_EDGE('',*,*,#19820,.T.);
#27880=ORIENTED_EDGE('',*,*,#19814,.T.);
#27881=ORIENTED_EDGE('',*,*,#19821,.T.);
#27882=ORIENTED_EDGE('',*,*,#19822,.F.);
#27883=ORIENTED_EDGE('',*,*,#19823,.T.);
#27884=ORIENTED_EDGE('',*,*,#19819,.T.);
#27885=ORIENTED_EDGE('',*,*,#19824,.T.);
#27886=ORIENTED_EDGE('',*,*,#19825,.F.);
#27887=ORIENTED_EDGE('',*,*,#19826,.T.);
#27888=ORIENTED_EDGE('',*,*,#19827,.T.);
#27889=ORIENTED_EDGE('',*,*,#19822,.T.);
#27890=ORIENTED_EDGE('',*,*,#19828,.T.);
#27891=ORIENTED_EDGE('',*,*,#19829,.F.);
#27892=ORIENTED_EDGE('',*,*,#19830,.F.);
#27893=ORIENTED_EDGE('',*,*,#19831,.F.);
#27894=ORIENTED_EDGE('',*,*,#19832,.T.);
#27895=ORIENTED_EDGE('',*,*,#19833,.F.);
#27896=ORIENTED_EDGE('',*,*,#19834,.F.);
#27897=ORIENTED_EDGE('',*,*,#19829,.T.);
#27898=ORIENTED_EDGE('',*,*,#19835,.T.);
#27899=ORIENTED_EDGE('',*,*,#19836,.F.);
#27900=ORIENTED_EDGE('',*,*,#19837,.F.);
#27901=ORIENTED_EDGE('',*,*,#19833,.T.);
#27902=ORIENTED_EDGE('',*,*,#19838,.T.);
#27903=ORIENTED_EDGE('',*,*,#19839,.F.);
#27904=ORIENTED_EDGE('',*,*,#19840,.F.);
#27905=ORIENTED_EDGE('',*,*,#19836,.T.);
#27906=ORIENTED_EDGE('',*,*,#19841,.T.);
#27907=ORIENTED_EDGE('',*,*,#19842,.F.);
#27908=ORIENTED_EDGE('',*,*,#19843,.F.);
#27909=ORIENTED_EDGE('',*,*,#19844,.F.);
#27910=ORIENTED_EDGE('',*,*,#19839,.T.);
#27911=ORIENTED_EDGE('',*,*,#19845,.T.);
#27912=ORIENTED_EDGE('',*,*,#19846,.F.);
#27913=ORIENTED_EDGE('',*,*,#19847,.F.);
#27914=ORIENTED_EDGE('',*,*,#19842,.T.);
#27915=ORIENTED_EDGE('',*,*,#19848,.T.);
#27916=ORIENTED_EDGE('',*,*,#19849,.T.);
#27917=ORIENTED_EDGE('',*,*,#19850,.F.);
#27918=ORIENTED_EDGE('',*,*,#19851,.F.);
#27919=ORIENTED_EDGE('',*,*,#19846,.T.);
#27920=ORIENTED_EDGE('',*,*,#19852,.T.);
#27921=ORIENTED_EDGE('',*,*,#19853,.F.);
#27922=ORIENTED_EDGE('',*,*,#19854,.F.);
#27923=ORIENTED_EDGE('',*,*,#19850,.T.);
#27924=ORIENTED_EDGE('',*,*,#19855,.T.);
#27925=ORIENTED_EDGE('',*,*,#19856,.F.);
#27926=ORIENTED_EDGE('',*,*,#19857,.F.);
#27927=ORIENTED_EDGE('',*,*,#19853,.T.);
#27928=ORIENTED_EDGE('',*,*,#19858,.T.);
#27929=ORIENTED_EDGE('',*,*,#19859,.F.);
#27930=ORIENTED_EDGE('',*,*,#19860,.F.);
#27931=ORIENTED_EDGE('',*,*,#19856,.T.);
#27932=ORIENTED_EDGE('',*,*,#19861,.T.);
#27933=ORIENTED_EDGE('',*,*,#19862,.F.);
#27934=ORIENTED_EDGE('',*,*,#19863,.F.);
#27935=ORIENTED_EDGE('',*,*,#19859,.T.);
#27936=ORIENTED_EDGE('',*,*,#19864,.T.);
#27937=ORIENTED_EDGE('',*,*,#19865,.F.);
#27938=ORIENTED_EDGE('',*,*,#19866,.F.);
#27939=ORIENTED_EDGE('',*,*,#19862,.T.);
#27940=ORIENTED_EDGE('',*,*,#19867,.T.);
#27941=ORIENTED_EDGE('',*,*,#19868,.F.);
#27942=ORIENTED_EDGE('',*,*,#19869,.F.);
#27943=ORIENTED_EDGE('',*,*,#19865,.T.);
#27944=ORIENTED_EDGE('',*,*,#19870,.T.);
#27945=ORIENTED_EDGE('',*,*,#19871,.F.);
#27946=ORIENTED_EDGE('',*,*,#19872,.F.);
#27947=ORIENTED_EDGE('',*,*,#19868,.T.);
#27948=ORIENTED_EDGE('',*,*,#19873,.T.);
#27949=ORIENTED_EDGE('',*,*,#19874,.F.);
#27950=ORIENTED_EDGE('',*,*,#19875,.F.);
#27951=ORIENTED_EDGE('',*,*,#19876,.F.);
#27952=ORIENTED_EDGE('',*,*,#19871,.T.);
#27953=ORIENTED_EDGE('',*,*,#19877,.T.);
#27954=ORIENTED_EDGE('',*,*,#19878,.F.);
#27955=ORIENTED_EDGE('',*,*,#19879,.F.);
#27956=ORIENTED_EDGE('',*,*,#19874,.T.);
#27957=ORIENTED_EDGE('',*,*,#19880,.T.);
#27958=ORIENTED_EDGE('',*,*,#19881,.F.);
#27959=ORIENTED_EDGE('',*,*,#19882,.F.);
#27960=ORIENTED_EDGE('',*,*,#19878,.T.);
#27961=ORIENTED_EDGE('',*,*,#19883,.T.);
#27962=ORIENTED_EDGE('',*,*,#19884,.F.);
#27963=ORIENTED_EDGE('',*,*,#19885,.F.);
#27964=ORIENTED_EDGE('',*,*,#19881,.T.);
#27965=ORIENTED_EDGE('',*,*,#19886,.T.);
#27966=ORIENTED_EDGE('',*,*,#19887,.F.);
#27967=ORIENTED_EDGE('',*,*,#19888,.F.);
#27968=ORIENTED_EDGE('',*,*,#19884,.T.);
#27969=ORIENTED_EDGE('',*,*,#19889,.T.);
#27970=ORIENTED_EDGE('',*,*,#19890,.F.);
#27971=ORIENTED_EDGE('',*,*,#19891,.F.);
#27972=ORIENTED_EDGE('',*,*,#19887,.T.);
#27973=ORIENTED_EDGE('',*,*,#19892,.T.);
#27974=ORIENTED_EDGE('',*,*,#19893,.F.);
#27975=ORIENTED_EDGE('',*,*,#19894,.F.);
#27976=ORIENTED_EDGE('',*,*,#19890,.T.);
#27977=ORIENTED_EDGE('',*,*,#19895,.T.);
#27978=ORIENTED_EDGE('',*,*,#19896,.T.);
#27979=ORIENTED_EDGE('',*,*,#19897,.F.);
#27980=ORIENTED_EDGE('',*,*,#19898,.F.);
#27981=ORIENTED_EDGE('',*,*,#19893,.T.);
#27982=ORIENTED_EDGE('',*,*,#19899,.T.);
#27983=ORIENTED_EDGE('',*,*,#19900,.F.);
#27984=ORIENTED_EDGE('',*,*,#19901,.F.);
#27985=ORIENTED_EDGE('',*,*,#19897,.T.);
#27986=ORIENTED_EDGE('',*,*,#19902,.T.);
#27987=ORIENTED_EDGE('',*,*,#19900,.T.);
#27988=ORIENTED_EDGE('',*,*,#19903,.T.);
#27989=ORIENTED_EDGE('',*,*,#19904,.F.);
#27990=ORIENTED_EDGE('',*,*,#19905,.F.);
#27991=ORIENTED_EDGE('',*,*,#19906,.F.);
#27992=ORIENTED_EDGE('',*,*,#19825,.T.);
#27993=ORIENTED_EDGE('',*,*,#19907,.T.);
#27994=ORIENTED_EDGE('',*,*,#19908,.F.);
#27995=ORIENTED_EDGE('',*,*,#19909,.T.);
#27996=ORIENTED_EDGE('',*,*,#19910,.F.);
#27997=ORIENTED_EDGE('',*,*,#19911,.T.);
#27998=ORIENTED_EDGE('',*,*,#19904,.T.);
#27999=ORIENTED_EDGE('',*,*,#19912,.T.);
#28000=ORIENTED_EDGE('',*,*,#19913,.F.);
#28001=ORIENTED_EDGE('',*,*,#19911,.F.);
#28002=ORIENTED_EDGE('',*,*,#19914,.F.);
#28003=ORIENTED_EDGE('',*,*,#19907,.F.);
#28004=ORIENTED_EDGE('',*,*,#19828,.F.);
#28005=ORIENTED_EDGE('',*,*,#19824,.F.);
#28006=ORIENTED_EDGE('',*,*,#19821,.F.);
#28007=ORIENTED_EDGE('',*,*,#19818,.F.);
#28008=ORIENTED_EDGE('',*,*,#19817,.F.);
#28009=ORIENTED_EDGE('',*,*,#19813,.F.);
#28010=ORIENTED_EDGE('',*,*,#19810,.F.);
#28011=ORIENTED_EDGE('',*,*,#19807,.F.);
#28012=ORIENTED_EDGE('',*,*,#19806,.F.);
#28013=ORIENTED_EDGE('',*,*,#19802,.F.);
#28014=ORIENTED_EDGE('',*,*,#19799,.F.);
#28015=ORIENTED_EDGE('',*,*,#19796,.F.);
#28016=ORIENTED_EDGE('',*,*,#19795,.F.);
#28017=ORIENTED_EDGE('',*,*,#19791,.F.);
#28018=ORIENTED_EDGE('',*,*,#19790,.F.);
#28019=ORIENTED_EDGE('',*,*,#19786,.F.);
#28020=ORIENTED_EDGE('',*,*,#19783,.F.);
#28021=ORIENTED_EDGE('',*,*,#19782,.F.);
#28022=ORIENTED_EDGE('',*,*,#19778,.F.);
#28023=ORIENTED_EDGE('',*,*,#19775,.F.);
#28024=ORIENTED_EDGE('',*,*,#19772,.F.);
#28025=ORIENTED_EDGE('',*,*,#19771,.F.);
#28026=ORIENTED_EDGE('',*,*,#19767,.F.);
#28027=ORIENTED_EDGE('',*,*,#19766,.F.);
#28028=ORIENTED_EDGE('',*,*,#19762,.F.);
#28029=ORIENTED_EDGE('',*,*,#19759,.F.);
#28030=ORIENTED_EDGE('',*,*,#19756,.F.);
#28031=ORIENTED_EDGE('',*,*,#19755,.F.);
#28032=ORIENTED_EDGE('',*,*,#19751,.F.);
#28033=ORIENTED_EDGE('',*,*,#19748,.F.);
#28034=ORIENTED_EDGE('',*,*,#19745,.F.);
#28035=ORIENTED_EDGE('',*,*,#19915,.F.);
#28036=ORIENTED_EDGE('',*,*,#19830,.T.);
#28037=ORIENTED_EDGE('',*,*,#19834,.T.);
#28038=ORIENTED_EDGE('',*,*,#19837,.T.);
#28039=ORIENTED_EDGE('',*,*,#19840,.T.);
#28040=ORIENTED_EDGE('',*,*,#19844,.T.);
#28041=ORIENTED_EDGE('',*,*,#19843,.T.);
#28042=ORIENTED_EDGE('',*,*,#19847,.T.);
#28043=ORIENTED_EDGE('',*,*,#19851,.T.);
#28044=ORIENTED_EDGE('',*,*,#19854,.T.);
#28045=ORIENTED_EDGE('',*,*,#19857,.T.);
#28046=ORIENTED_EDGE('',*,*,#19860,.T.);
#28047=ORIENTED_EDGE('',*,*,#19863,.T.);
#28048=ORIENTED_EDGE('',*,*,#19866,.T.);
#28049=ORIENTED_EDGE('',*,*,#19869,.T.);
#28050=ORIENTED_EDGE('',*,*,#19872,.T.);
#28051=ORIENTED_EDGE('',*,*,#19876,.T.);
#28052=ORIENTED_EDGE('',*,*,#19875,.T.);
#28053=ORIENTED_EDGE('',*,*,#19879,.T.);
#28054=ORIENTED_EDGE('',*,*,#19882,.T.);
#28055=ORIENTED_EDGE('',*,*,#19885,.T.);
#28056=ORIENTED_EDGE('',*,*,#19888,.T.);
#28057=ORIENTED_EDGE('',*,*,#19891,.T.);
#28058=ORIENTED_EDGE('',*,*,#19894,.T.);
#28059=ORIENTED_EDGE('',*,*,#19898,.T.);
#28060=ORIENTED_EDGE('',*,*,#19901,.T.);
#28061=ORIENTED_EDGE('',*,*,#19906,.T.);
#28062=ORIENTED_EDGE('',*,*,#19905,.T.);
#28063=ORIENTED_EDGE('',*,*,#19916,.F.);
#28064=ORIENTED_EDGE('',*,*,#19917,.T.);
#28065=ORIENTED_EDGE('',*,*,#19831,.T.);
#28066=ORIENTED_EDGE('',*,*,#19915,.T.);
#28067=ORIENTED_EDGE('',*,*,#19918,.F.);
#28068=ORIENTED_EDGE('',*,*,#19912,.F.);
#28069=ORIENTED_EDGE('',*,*,#19903,.F.);
#28070=ORIENTED_EDGE('',*,*,#19902,.F.);
#28071=ORIENTED_EDGE('',*,*,#19899,.F.);
#28072=ORIENTED_EDGE('',*,*,#19896,.F.);
#28073=ORIENTED_EDGE('',*,*,#19895,.F.);
#28074=ORIENTED_EDGE('',*,*,#19892,.F.);
#28075=ORIENTED_EDGE('',*,*,#19889,.F.);
#28076=ORIENTED_EDGE('',*,*,#19886,.F.);
#28077=ORIENTED_EDGE('',*,*,#19883,.F.);
#28078=ORIENTED_EDGE('',*,*,#19880,.F.);
#28079=ORIENTED_EDGE('',*,*,#19877,.F.);
#28080=ORIENTED_EDGE('',*,*,#19873,.F.);
#28081=ORIENTED_EDGE('',*,*,#19870,.F.);
#28082=ORIENTED_EDGE('',*,*,#19867,.F.);
#28083=ORIENTED_EDGE('',*,*,#19864,.F.);
#28084=ORIENTED_EDGE('',*,*,#19861,.F.);
#28085=ORIENTED_EDGE('',*,*,#19858,.F.);
#28086=ORIENTED_EDGE('',*,*,#19855,.F.);
#28087=ORIENTED_EDGE('',*,*,#19852,.F.);
#28088=ORIENTED_EDGE('',*,*,#19849,.F.);
#28089=ORIENTED_EDGE('',*,*,#19848,.F.);
#28090=ORIENTED_EDGE('',*,*,#19845,.F.);
#28091=ORIENTED_EDGE('',*,*,#19841,.F.);
#28092=ORIENTED_EDGE('',*,*,#19838,.F.);
#28093=ORIENTED_EDGE('',*,*,#19835,.F.);
#28094=ORIENTED_EDGE('',*,*,#19832,.F.);
#28095=ORIENTED_EDGE('',*,*,#19917,.F.);
#28096=ORIENTED_EDGE('',*,*,#19919,.F.);
#28097=ORIENTED_EDGE('',*,*,#19743,.F.);
#28098=ORIENTED_EDGE('',*,*,#19747,.F.);
#28099=ORIENTED_EDGE('',*,*,#19750,.F.);
#28100=ORIENTED_EDGE('',*,*,#19754,.F.);
#28101=ORIENTED_EDGE('',*,*,#19753,.F.);
#28102=ORIENTED_EDGE('',*,*,#19758,.F.);
#28103=ORIENTED_EDGE('',*,*,#19761,.F.);
#28104=ORIENTED_EDGE('',*,*,#19765,.F.);
#28105=ORIENTED_EDGE('',*,*,#19764,.F.);
#28106=ORIENTED_EDGE('',*,*,#19770,.F.);
#28107=ORIENTED_EDGE('',*,*,#19769,.F.);
#28108=ORIENTED_EDGE('',*,*,#19774,.F.);
#28109=ORIENTED_EDGE('',*,*,#19777,.F.);
#28110=ORIENTED_EDGE('',*,*,#19781,.F.);
#28111=ORIENTED_EDGE('',*,*,#19780,.F.);
#28112=ORIENTED_EDGE('',*,*,#19785,.F.);
#28113=ORIENTED_EDGE('',*,*,#19789,.F.);
#28114=ORIENTED_EDGE('',*,*,#19788,.F.);
#28115=ORIENTED_EDGE('',*,*,#19794,.F.);
#28116=ORIENTED_EDGE('',*,*,#19793,.F.);
#28117=ORIENTED_EDGE('',*,*,#19798,.F.);
#28118=ORIENTED_EDGE('',*,*,#19801,.F.);
#28119=ORIENTED_EDGE('',*,*,#19805,.F.);
#28120=ORIENTED_EDGE('',*,*,#19804,.F.);
#28121=ORIENTED_EDGE('',*,*,#19809,.F.);
#28122=ORIENTED_EDGE('',*,*,#19812,.F.);
#28123=ORIENTED_EDGE('',*,*,#19816,.F.);
#28124=ORIENTED_EDGE('',*,*,#19815,.F.);
#28125=ORIENTED_EDGE('',*,*,#19820,.F.);
#28126=ORIENTED_EDGE('',*,*,#19823,.F.);
#28127=ORIENTED_EDGE('',*,*,#19827,.F.);
#28128=ORIENTED_EDGE('',*,*,#19826,.F.);
#28129=ORIENTED_EDGE('',*,*,#19909,.F.);
#28130=ORIENTED_EDGE('',*,*,#19920,.T.);
#28131=ORIENTED_EDGE('',*,*,#19921,.T.);
#28132=ORIENTED_EDGE('',*,*,#19918,.T.);
#28133=ORIENTED_EDGE('',*,*,#19744,.T.);
#28134=ORIENTED_EDGE('',*,*,#19919,.T.);
#28135=ORIENTED_EDGE('',*,*,#19916,.T.);
#28136=ORIENTED_EDGE('',*,*,#19921,.F.);
#28137=ORIENTED_EDGE('',*,*,#19922,.F.);
#28138=ORIENTED_EDGE('',*,*,#19920,.F.);
#28139=ORIENTED_EDGE('',*,*,#19910,.T.);
#28140=ORIENTED_EDGE('',*,*,#19923,.T.);
#28141=ORIENTED_EDGE('',*,*,#19924,.T.);
#28142=ORIENTED_EDGE('',*,*,#19923,.F.);
#28143=ORIENTED_EDGE('',*,*,#19913,.T.);
#28144=ORIENTED_EDGE('',*,*,#19908,.T.);
#28145=ORIENTED_EDGE('',*,*,#19914,.T.);
#28146=ORIENTED_EDGE('',*,*,#19924,.F.);
#28147=ORIENTED_EDGE('',*,*,#19925,.F.);
#28148=ORIENTED_EDGE('',*,*,#19926,.F.);
#28149=ORIENTED_EDGE('',*,*,#19927,.F.);
#28150=ORIENTED_EDGE('',*,*,#19928,.F.);
#28151=ORIENTED_EDGE('',*,*,#19927,.T.);
#28152=ORIENTED_EDGE('',*,*,#19929,.F.);
#28153=ORIENTED_EDGE('',*,*,#19930,.F.);
#28154=ORIENTED_EDGE('',*,*,#19931,.F.);
#28155=ORIENTED_EDGE('',*,*,#19932,.F.);
#28156=ORIENTED_EDGE('',*,*,#19929,.T.);
#28157=ORIENTED_EDGE('',*,*,#19926,.T.);
#28158=ORIENTED_EDGE('',*,*,#19933,.T.);
#28159=ORIENTED_EDGE('',*,*,#19934,.T.);
#28160=ORIENTED_EDGE('',*,*,#19935,.F.);
#28161=ORIENTED_EDGE('',*,*,#19936,.F.);
#28162=ORIENTED_EDGE('',*,*,#19934,.F.);
#28163=ORIENTED_EDGE('',*,*,#19937,.T.);
#28164=ORIENTED_EDGE('',*,*,#19938,.T.);
#28165=ORIENTED_EDGE('',*,*,#19939,.F.);
#28166=ORIENTED_EDGE('',*,*,#19940,.T.);
#28167=ORIENTED_EDGE('',*,*,#19941,.T.);
#28168=ORIENTED_EDGE('',*,*,#19942,.T.);
#28169=ORIENTED_EDGE('',*,*,#19943,.F.);
#28170=ORIENTED_EDGE('',*,*,#19944,.T.);
#28171=ORIENTED_EDGE('',*,*,#19945,.T.);
#28172=ORIENTED_EDGE('',*,*,#19946,.T.);
#28173=ORIENTED_EDGE('',*,*,#19947,.F.);
#28174=ORIENTED_EDGE('',*,*,#19948,.T.);
#28175=ORIENTED_EDGE('',*,*,#19949,.T.);
#28176=ORIENTED_EDGE('',*,*,#19950,.T.);
#28177=ORIENTED_EDGE('',*,*,#19951,.F.);
#28178=ORIENTED_EDGE('',*,*,#19952,.T.);
#28179=ORIENTED_EDGE('',*,*,#19953,.T.);
#28180=ORIENTED_EDGE('',*,*,#19954,.T.);
#28181=ORIENTED_EDGE('',*,*,#19955,.F.);
#28182=ORIENTED_EDGE('',*,*,#19956,.T.);
#28183=ORIENTED_EDGE('',*,*,#19957,.T.);
#28184=ORIENTED_EDGE('',*,*,#19958,.T.);
#28185=ORIENTED_EDGE('',*,*,#19959,.F.);
#28186=ORIENTED_EDGE('',*,*,#19960,.T.);
#28187=ORIENTED_EDGE('',*,*,#19961,.T.);
#28188=ORIENTED_EDGE('',*,*,#19962,.T.);
#28189=ORIENTED_EDGE('',*,*,#19963,.F.);
#28190=ORIENTED_EDGE('',*,*,#19964,.T.);
#28191=ORIENTED_EDGE('',*,*,#19965,.T.);
#28192=ORIENTED_EDGE('',*,*,#19966,.T.);
#28193=ORIENTED_EDGE('',*,*,#19967,.F.);
#28194=ORIENTED_EDGE('',*,*,#19968,.T.);
#28195=ORIENTED_EDGE('',*,*,#19969,.T.);
#28196=ORIENTED_EDGE('',*,*,#19970,.T.);
#28197=ORIENTED_EDGE('',*,*,#19971,.F.);
#28198=ORIENTED_EDGE('',*,*,#19972,.T.);
#28199=ORIENTED_EDGE('',*,*,#19973,.T.);
#28200=ORIENTED_EDGE('',*,*,#19974,.T.);
#28201=ORIENTED_EDGE('',*,*,#19975,.F.);
#28202=ORIENTED_EDGE('',*,*,#19976,.T.);
#28203=ORIENTED_EDGE('',*,*,#19977,.T.);
#28204=ORIENTED_EDGE('',*,*,#19978,.T.);
#28205=ORIENTED_EDGE('',*,*,#19979,.F.);
#28206=ORIENTED_EDGE('',*,*,#19980,.T.);
#28207=ORIENTED_EDGE('',*,*,#19981,.T.);
#28208=ORIENTED_EDGE('',*,*,#19982,.T.);
#28209=ORIENTED_EDGE('',*,*,#19983,.F.);
#28210=ORIENTED_EDGE('',*,*,#19984,.T.);
#28211=ORIENTED_EDGE('',*,*,#19985,.T.);
#28212=ORIENTED_EDGE('',*,*,#19986,.T.);
#28213=ORIENTED_EDGE('',*,*,#19987,.F.);
#28214=ORIENTED_EDGE('',*,*,#19988,.T.);
#28215=ORIENTED_EDGE('',*,*,#19989,.T.);
#28216=ORIENTED_EDGE('',*,*,#19990,.T.);
#28217=ORIENTED_EDGE('',*,*,#19991,.F.);
#28218=ORIENTED_EDGE('',*,*,#19992,.T.);
#28219=ORIENTED_EDGE('',*,*,#19993,.T.);
#28220=ORIENTED_EDGE('',*,*,#19994,.T.);
#28221=ORIENTED_EDGE('',*,*,#19995,.F.);
#28222=ORIENTED_EDGE('',*,*,#19996,.T.);
#28223=ORIENTED_EDGE('',*,*,#19997,.T.);
#28224=ORIENTED_EDGE('',*,*,#19998,.T.);
#28225=ORIENTED_EDGE('',*,*,#19999,.F.);
#28226=ORIENTED_EDGE('',*,*,#20000,.T.);
#28227=ORIENTED_EDGE('',*,*,#20001,.T.);
#28228=ORIENTED_EDGE('',*,*,#20002,.T.);
#28229=ORIENTED_EDGE('',*,*,#20003,.F.);
#28230=ORIENTED_EDGE('',*,*,#19931,.T.);
#28231=ORIENTED_EDGE('',*,*,#19925,.T.);
#28232=ORIENTED_EDGE('',*,*,#19928,.T.);
#28233=ORIENTED_EDGE('',*,*,#20004,.F.);
#28234=ORIENTED_EDGE('',*,*,#20005,.T.);
#28235=ORIENTED_EDGE('',*,*,#20006,.T.);
#28236=ORIENTED_EDGE('',*,*,#20007,.T.);
#28237=ORIENTED_EDGE('',*,*,#20008,.F.);
#28238=ORIENTED_EDGE('',*,*,#20009,.T.);
#28239=ORIENTED_EDGE('',*,*,#20010,.T.);
#28240=ORIENTED_EDGE('',*,*,#20011,.T.);
#28241=ORIENTED_EDGE('',*,*,#20012,.F.);
#28242=ORIENTED_EDGE('',*,*,#20013,.T.);
#28243=ORIENTED_EDGE('',*,*,#20014,.T.);
#28244=ORIENTED_EDGE('',*,*,#20015,.T.);
#28245=ORIENTED_EDGE('',*,*,#20016,.F.);
#28246=ORIENTED_EDGE('',*,*,#20017,.T.);
#28247=ORIENTED_EDGE('',*,*,#20018,.T.);
#28248=ORIENTED_EDGE('',*,*,#20019,.T.);
#28249=ORIENTED_EDGE('',*,*,#20020,.F.);
#28250=ORIENTED_EDGE('',*,*,#20021,.T.);
#28251=ORIENTED_EDGE('',*,*,#20022,.T.);
#28252=ORIENTED_EDGE('',*,*,#20023,.T.);
#28253=ORIENTED_EDGE('',*,*,#20024,.F.);
#28254=ORIENTED_EDGE('',*,*,#20025,.T.);
#28255=ORIENTED_EDGE('',*,*,#20026,.T.);
#28256=ORIENTED_EDGE('',*,*,#20027,.T.);
#28257=ORIENTED_EDGE('',*,*,#20028,.F.);
#28258=ORIENTED_EDGE('',*,*,#20029,.T.);
#28259=ORIENTED_EDGE('',*,*,#20030,.T.);
#28260=ORIENTED_EDGE('',*,*,#20031,.T.);
#28261=ORIENTED_EDGE('',*,*,#20032,.F.);
#28262=ORIENTED_EDGE('',*,*,#20033,.T.);
#28263=ORIENTED_EDGE('',*,*,#20034,.T.);
#28264=ORIENTED_EDGE('',*,*,#20035,.T.);
#28265=ORIENTED_EDGE('',*,*,#20036,.F.);
#28266=ORIENTED_EDGE('',*,*,#20037,.T.);
#28267=ORIENTED_EDGE('',*,*,#20038,.T.);
#28268=ORIENTED_EDGE('',*,*,#20039,.T.);
#28269=ORIENTED_EDGE('',*,*,#20040,.F.);
#28270=ORIENTED_EDGE('',*,*,#20041,.T.);
#28271=ORIENTED_EDGE('',*,*,#20042,.T.);
#28272=ORIENTED_EDGE('',*,*,#20043,.T.);
#28273=ORIENTED_EDGE('',*,*,#20044,.F.);
#28274=ORIENTED_EDGE('',*,*,#20045,.T.);
#28275=ORIENTED_EDGE('',*,*,#20046,.T.);
#28276=ORIENTED_EDGE('',*,*,#20047,.T.);
#28277=ORIENTED_EDGE('',*,*,#20048,.F.);
#28278=ORIENTED_EDGE('',*,*,#20049,.T.);
#28279=ORIENTED_EDGE('',*,*,#20050,.T.);
#28280=ORIENTED_EDGE('',*,*,#20051,.T.);
#28281=ORIENTED_EDGE('',*,*,#20052,.F.);
#28282=ORIENTED_EDGE('',*,*,#20053,.T.);
#28283=ORIENTED_EDGE('',*,*,#20054,.T.);
#28284=ORIENTED_EDGE('',*,*,#20055,.T.);
#28285=ORIENTED_EDGE('',*,*,#20056,.F.);
#28286=ORIENTED_EDGE('',*,*,#20057,.T.);
#28287=ORIENTED_EDGE('',*,*,#20058,.T.);
#28288=ORIENTED_EDGE('',*,*,#20059,.T.);
#28289=ORIENTED_EDGE('',*,*,#20060,.F.);
#28290=ORIENTED_EDGE('',*,*,#20061,.T.);
#28291=ORIENTED_EDGE('',*,*,#20062,.T.);
#28292=ORIENTED_EDGE('',*,*,#20063,.T.);
#28293=ORIENTED_EDGE('',*,*,#20064,.F.);
#28294=ORIENTED_EDGE('',*,*,#20065,.T.);
#28295=ORIENTED_EDGE('',*,*,#20066,.T.);
#28296=ORIENTED_EDGE('',*,*,#20067,.T.);
#28297=ORIENTED_EDGE('',*,*,#20068,.F.);
#28298=ORIENTED_EDGE('',*,*,#20069,.T.);
#28299=ORIENTED_EDGE('',*,*,#20070,.T.);
#28300=ORIENTED_EDGE('',*,*,#20071,.T.);
#28301=ORIENTED_EDGE('',*,*,#20072,.F.);
#28302=ORIENTED_EDGE('',*,*,#20073,.T.);
#28303=ORIENTED_EDGE('',*,*,#20074,.T.);
#28304=ORIENTED_EDGE('',*,*,#20075,.T.);
#28305=ORIENTED_EDGE('',*,*,#20076,.F.);
#28306=ORIENTED_EDGE('',*,*,#20077,.T.);
#28307=ORIENTED_EDGE('',*,*,#20002,.F.);
#28308=ORIENTED_EDGE('',*,*,#20078,.T.);
#28309=ORIENTED_EDGE('',*,*,#20079,.F.);
#28310=ORIENTED_EDGE('',*,*,#20080,.F.);
#28311=ORIENTED_EDGE('',*,*,#20081,.F.);
#28312=ORIENTED_EDGE('',*,*,#20079,.T.);
#28313=ORIENTED_EDGE('',*,*,#20082,.T.);
#28314=ORIENTED_EDGE('',*,*,#20000,.F.);
#28315=ORIENTED_EDGE('',*,*,#20001,.F.);
#28316=ORIENTED_EDGE('',*,*,#20082,.F.);
#28317=ORIENTED_EDGE('',*,*,#20078,.F.);
#28318=ORIENTED_EDGE('',*,*,#20083,.T.);
#28319=ORIENTED_EDGE('',*,*,#20076,.T.);
#28320=ORIENTED_EDGE('',*,*,#20084,.T.);
#28321=ORIENTED_EDGE('',*,*,#20085,.T.);
#28322=ORIENTED_EDGE('',*,*,#20072,.T.);
#28323=ORIENTED_EDGE('',*,*,#20086,.T.);
#28324=ORIENTED_EDGE('',*,*,#20087,.T.);
#28325=ORIENTED_EDGE('',*,*,#20068,.T.);
#28326=ORIENTED_EDGE('',*,*,#20088,.T.);
#28327=ORIENTED_EDGE('',*,*,#20089,.T.);
#28328=ORIENTED_EDGE('',*,*,#20064,.T.);
#28329=ORIENTED_EDGE('',*,*,#20090,.T.);
#28330=ORIENTED_EDGE('',*,*,#20091,.T.);
#28331=ORIENTED_EDGE('',*,*,#20060,.T.);
#28332=ORIENTED_EDGE('',*,*,#20092,.T.);
#28333=ORIENTED_EDGE('',*,*,#20093,.T.);
#28334=ORIENTED_EDGE('',*,*,#20056,.T.);
#28335=ORIENTED_EDGE('',*,*,#20094,.T.);
#28336=ORIENTED_EDGE('',*,*,#20095,.T.);
#28337=ORIENTED_EDGE('',*,*,#20052,.T.);
#28338=ORIENTED_EDGE('',*,*,#20096,.T.);
#28339=ORIENTED_EDGE('',*,*,#20097,.T.);
#28340=ORIENTED_EDGE('',*,*,#20048,.T.);
#28341=ORIENTED_EDGE('',*,*,#20098,.T.);
#28342=ORIENTED_EDGE('',*,*,#20099,.T.);
#28343=ORIENTED_EDGE('',*,*,#20044,.T.);
#28344=ORIENTED_EDGE('',*,*,#20100,.T.);
#28345=ORIENTED_EDGE('',*,*,#20101,.T.);
#28346=ORIENTED_EDGE('',*,*,#20040,.T.);
#28347=ORIENTED_EDGE('',*,*,#20102,.T.);
#28348=ORIENTED_EDGE('',*,*,#20103,.T.);
#28349=ORIENTED_EDGE('',*,*,#20036,.T.);
#28350=ORIENTED_EDGE('',*,*,#20104,.T.);
#28351=ORIENTED_EDGE('',*,*,#20105,.T.);
#28352=ORIENTED_EDGE('',*,*,#20032,.T.);
#28353=ORIENTED_EDGE('',*,*,#20106,.T.);
#28354=ORIENTED_EDGE('',*,*,#20107,.T.);
#28355=ORIENTED_EDGE('',*,*,#20028,.T.);
#28356=ORIENTED_EDGE('',*,*,#20108,.T.);
#28357=ORIENTED_EDGE('',*,*,#20109,.T.);
#28358=ORIENTED_EDGE('',*,*,#20024,.T.);
#28359=ORIENTED_EDGE('',*,*,#20110,.T.);
#28360=ORIENTED_EDGE('',*,*,#20111,.T.);
#28361=ORIENTED_EDGE('',*,*,#20020,.T.);
#28362=ORIENTED_EDGE('',*,*,#20112,.T.);
#28363=ORIENTED_EDGE('',*,*,#20113,.T.);
#28364=ORIENTED_EDGE('',*,*,#20016,.T.);
#28365=ORIENTED_EDGE('',*,*,#20114,.T.);
#28366=ORIENTED_EDGE('',*,*,#20115,.T.);
#28367=ORIENTED_EDGE('',*,*,#20012,.T.);
#28368=ORIENTED_EDGE('',*,*,#20116,.T.);
#28369=ORIENTED_EDGE('',*,*,#20117,.T.);
#28370=ORIENTED_EDGE('',*,*,#20008,.T.);
#28371=ORIENTED_EDGE('',*,*,#20118,.T.);
#28372=ORIENTED_EDGE('',*,*,#20119,.T.);
#28373=ORIENTED_EDGE('',*,*,#20004,.T.);
#28374=ORIENTED_EDGE('',*,*,#19930,.T.);
#28375=ORIENTED_EDGE('',*,*,#19932,.T.);
#28376=ORIENTED_EDGE('',*,*,#20003,.T.);
#28377=ORIENTED_EDGE('',*,*,#20080,.T.);
#28378=ORIENTED_EDGE('',*,*,#20081,.T.);
#28379=ORIENTED_EDGE('',*,*,#19999,.T.);
#28380=ORIENTED_EDGE('',*,*,#20120,.T.);
#28381=ORIENTED_EDGE('',*,*,#20121,.T.);
#28382=ORIENTED_EDGE('',*,*,#19995,.T.);
#28383=ORIENTED_EDGE('',*,*,#20122,.T.);
#28384=ORIENTED_EDGE('',*,*,#20123,.T.);
#28385=ORIENTED_EDGE('',*,*,#19991,.T.);
#28386=ORIENTED_EDGE('',*,*,#20124,.T.);
#28387=ORIENTED_EDGE('',*,*,#20125,.T.);
#28388=ORIENTED_EDGE('',*,*,#19987,.T.);
#28389=ORIENTED_EDGE('',*,*,#20126,.T.);
#28390=ORIENTED_EDGE('',*,*,#20127,.T.);
#28391=ORIENTED_EDGE('',*,*,#19983,.T.);
#28392=ORIENTED_EDGE('',*,*,#20128,.T.);
#28393=ORIENTED_EDGE('',*,*,#20129,.T.);
#28394=ORIENTED_EDGE('',*,*,#19979,.T.);
#28395=ORIENTED_EDGE('',*,*,#20130,.T.);
#28396=ORIENTED_EDGE('',*,*,#20131,.T.);
#28397=ORIENTED_EDGE('',*,*,#19975,.T.);
#28398=ORIENTED_EDGE('',*,*,#20132,.T.);
#28399=ORIENTED_EDGE('',*,*,#20133,.T.);
#28400=ORIENTED_EDGE('',*,*,#19971,.T.);
#28401=ORIENTED_EDGE('',*,*,#20134,.T.);
#28402=ORIENTED_EDGE('',*,*,#20135,.T.);
#28403=ORIENTED_EDGE('',*,*,#19967,.T.);
#28404=ORIENTED_EDGE('',*,*,#20136,.T.);
#28405=ORIENTED_EDGE('',*,*,#20137,.T.);
#28406=ORIENTED_EDGE('',*,*,#19963,.T.);
#28407=ORIENTED_EDGE('',*,*,#20138,.T.);
#28408=ORIENTED_EDGE('',*,*,#20139,.T.);
#28409=ORIENTED_EDGE('',*,*,#19959,.T.);
#28410=ORIENTED_EDGE('',*,*,#20140,.T.);
#28411=ORIENTED_EDGE('',*,*,#20141,.T.);
#28412=ORIENTED_EDGE('',*,*,#19955,.T.);
#28413=ORIENTED_EDGE('',*,*,#20142,.T.);
#28414=ORIENTED_EDGE('',*,*,#20143,.T.);
#28415=ORIENTED_EDGE('',*,*,#19951,.T.);
#28416=ORIENTED_EDGE('',*,*,#20144,.T.);
#28417=ORIENTED_EDGE('',*,*,#20145,.T.);
#28418=ORIENTED_EDGE('',*,*,#19947,.T.);
#28419=ORIENTED_EDGE('',*,*,#20146,.T.);
#28420=ORIENTED_EDGE('',*,*,#20147,.T.);
#28421=ORIENTED_EDGE('',*,*,#19943,.T.);
#28422=ORIENTED_EDGE('',*,*,#20148,.T.);
#28423=ORIENTED_EDGE('',*,*,#20149,.T.);
#28424=ORIENTED_EDGE('',*,*,#19939,.T.);
#28425=ORIENTED_EDGE('',*,*,#20150,.T.);
#28426=ORIENTED_EDGE('',*,*,#20151,.T.);
#28427=ORIENTED_EDGE('',*,*,#20152,.T.);
#28428=ORIENTED_EDGE('',*,*,#20151,.F.);
#28429=ORIENTED_EDGE('',*,*,#19997,.F.);
#28430=ORIENTED_EDGE('',*,*,#20153,.F.);
#28431=ORIENTED_EDGE('',*,*,#20154,.F.);
#28432=ORIENTED_EDGE('',*,*,#19998,.F.);
#28433=ORIENTED_EDGE('',*,*,#20154,.T.);
#28434=ORIENTED_EDGE('',*,*,#20155,.F.);
#28435=ORIENTED_EDGE('',*,*,#20120,.F.);
#28436=ORIENTED_EDGE('',*,*,#19996,.F.);
#28437=ORIENTED_EDGE('',*,*,#20121,.F.);
#28438=ORIENTED_EDGE('',*,*,#20155,.T.);
#28439=ORIENTED_EDGE('',*,*,#20153,.T.);
#28440=ORIENTED_EDGE('',*,*,#19994,.F.);
#28441=ORIENTED_EDGE('',*,*,#20156,.T.);
#28442=ORIENTED_EDGE('',*,*,#20157,.F.);
#28443=ORIENTED_EDGE('',*,*,#20122,.F.);
#28444=ORIENTED_EDGE('',*,*,#20123,.F.);
#28445=ORIENTED_EDGE('',*,*,#20157,.T.);
#28446=ORIENTED_EDGE('',*,*,#20158,.T.);
#28447=ORIENTED_EDGE('',*,*,#19992,.F.);
#28448=ORIENTED_EDGE('',*,*,#19993,.F.);
#28449=ORIENTED_EDGE('',*,*,#20158,.F.);
#28450=ORIENTED_EDGE('',*,*,#20156,.F.);
#28451=ORIENTED_EDGE('',*,*,#19989,.F.);
#28452=ORIENTED_EDGE('',*,*,#20159,.F.);
#28453=ORIENTED_EDGE('',*,*,#20160,.F.);
#28454=ORIENTED_EDGE('',*,*,#19990,.F.);
#28455=ORIENTED_EDGE('',*,*,#20160,.T.);
#28456=ORIENTED_EDGE('',*,*,#20161,.F.);
#28457=ORIENTED_EDGE('',*,*,#20124,.F.);
#28458=ORIENTED_EDGE('',*,*,#19988,.F.);
#28459=ORIENTED_EDGE('',*,*,#20125,.F.);
#28460=ORIENTED_EDGE('',*,*,#20161,.T.);
#28461=ORIENTED_EDGE('',*,*,#20159,.T.);
#28462=ORIENTED_EDGE('',*,*,#19986,.F.);
#28463=ORIENTED_EDGE('',*,*,#20162,.T.);
#28464=ORIENTED_EDGE('',*,*,#20163,.F.);
#28465=ORIENTED_EDGE('',*,*,#20126,.F.);
#28466=ORIENTED_EDGE('',*,*,#20127,.F.);
#28467=ORIENTED_EDGE('',*,*,#20163,.T.);
#28468=ORIENTED_EDGE('',*,*,#20164,.T.);
#28469=ORIENTED_EDGE('',*,*,#19984,.F.);
#28470=ORIENTED_EDGE('',*,*,#19985,.F.);
#28471=ORIENTED_EDGE('',*,*,#20164,.F.);
#28472=ORIENTED_EDGE('',*,*,#20162,.F.);
#28473=ORIENTED_EDGE('',*,*,#19981,.F.);
#28474=ORIENTED_EDGE('',*,*,#20165,.F.);
#28475=ORIENTED_EDGE('',*,*,#20166,.F.);
#28476=ORIENTED_EDGE('',*,*,#19982,.F.);
#28477=ORIENTED_EDGE('',*,*,#20166,.T.);
#28478=ORIENTED_EDGE('',*,*,#20167,.F.);
#28479=ORIENTED_EDGE('',*,*,#20128,.F.);
#28480=ORIENTED_EDGE('',*,*,#19980,.F.);
#28481=ORIENTED_EDGE('',*,*,#20129,.F.);
#28482=ORIENTED_EDGE('',*,*,#20167,.T.);
#28483=ORIENTED_EDGE('',*,*,#20165,.T.);
#28484=ORIENTED_EDGE('',*,*,#19978,.F.);
#28485=ORIENTED_EDGE('',*,*,#20168,.T.);
#28486=ORIENTED_EDGE('',*,*,#20169,.F.);
#28487=ORIENTED_EDGE('',*,*,#20130,.F.);
#28488=ORIENTED_EDGE('',*,*,#20131,.F.);
#28489=ORIENTED_EDGE('',*,*,#20169,.T.);
#28490=ORIENTED_EDGE('',*,*,#20170,.T.);
#28491=ORIENTED_EDGE('',*,*,#19976,.F.);
#28492=ORIENTED_EDGE('',*,*,#19977,.F.);
#28493=ORIENTED_EDGE('',*,*,#20170,.F.);
#28494=ORIENTED_EDGE('',*,*,#20168,.F.);
#28495=ORIENTED_EDGE('',*,*,#19973,.F.);
#28496=ORIENTED_EDGE('',*,*,#20171,.F.);
#28497=ORIENTED_EDGE('',*,*,#20172,.F.);
#28498=ORIENTED_EDGE('',*,*,#19974,.F.);
#28499=ORIENTED_EDGE('',*,*,#20172,.T.);
#28500=ORIENTED_EDGE('',*,*,#20173,.F.);
#28501=ORIENTED_EDGE('',*,*,#20132,.F.);
#28502=ORIENTED_EDGE('',*,*,#19972,.F.);
#28503=ORIENTED_EDGE('',*,*,#20133,.F.);
#28504=ORIENTED_EDGE('',*,*,#20173,.T.);
#28505=ORIENTED_EDGE('',*,*,#20171,.T.);
#28506=ORIENTED_EDGE('',*,*,#19970,.F.);
#28507=ORIENTED_EDGE('',*,*,#20174,.T.);
#28508=ORIENTED_EDGE('',*,*,#20175,.F.);
#28509=ORIENTED_EDGE('',*,*,#20134,.F.);
#28510=ORIENTED_EDGE('',*,*,#20135,.F.);
#28511=ORIENTED_EDGE('',*,*,#20175,.T.);
#28512=ORIENTED_EDGE('',*,*,#20176,.T.);
#28513=ORIENTED_EDGE('',*,*,#19968,.F.);
#28514=ORIENTED_EDGE('',*,*,#19969,.F.);
#28515=ORIENTED_EDGE('',*,*,#20176,.F.);
#28516=ORIENTED_EDGE('',*,*,#20174,.F.);
#28517=ORIENTED_EDGE('',*,*,#19965,.F.);
#28518=ORIENTED_EDGE('',*,*,#20177,.F.);
#28519=ORIENTED_EDGE('',*,*,#20178,.F.);
#28520=ORIENTED_EDGE('',*,*,#19966,.F.);
#28521=ORIENTED_EDGE('',*,*,#20178,.T.);
#28522=ORIENTED_EDGE('',*,*,#20179,.F.);
#28523=ORIENTED_EDGE('',*,*,#20136,.F.);
#28524=ORIENTED_EDGE('',*,*,#19964,.F.);
#28525=ORIENTED_EDGE('',*,*,#20137,.F.);
#28526=ORIENTED_EDGE('',*,*,#20179,.T.);
#28527=ORIENTED_EDGE('',*,*,#20177,.T.);
#28528=ORIENTED_EDGE('',*,*,#19962,.F.);
#28529=ORIENTED_EDGE('',*,*,#20180,.T.);
#28530=ORIENTED_EDGE('',*,*,#20181,.F.);
#28531=ORIENTED_EDGE('',*,*,#20138,.F.);
#28532=ORIENTED_EDGE('',*,*,#20139,.F.);
#28533=ORIENTED_EDGE('',*,*,#20181,.T.);
#28534=ORIENTED_EDGE('',*,*,#20182,.T.);
#28535=ORIENTED_EDGE('',*,*,#19960,.F.);
#28536=ORIENTED_EDGE('',*,*,#19961,.F.);
#28537=ORIENTED_EDGE('',*,*,#20182,.F.);
#28538=ORIENTED_EDGE('',*,*,#20180,.F.);
#28539=ORIENTED_EDGE('',*,*,#19957,.F.);
#28540=ORIENTED_EDGE('',*,*,#20183,.F.);
#28541=ORIENTED_EDGE('',*,*,#20184,.F.);
#28542=ORIENTED_EDGE('',*,*,#19958,.F.);
#28543=ORIENTED_EDGE('',*,*,#20184,.T.);
#28544=ORIENTED_EDGE('',*,*,#20185,.F.);
#28545=ORIENTED_EDGE('',*,*,#20140,.F.);
#28546=ORIENTED_EDGE('',*,*,#19956,.F.);
#28547=ORIENTED_EDGE('',*,*,#20141,.F.);
#28548=ORIENTED_EDGE('',*,*,#20185,.T.);
#28549=ORIENTED_EDGE('',*,*,#20183,.T.);
#28550=ORIENTED_EDGE('',*,*,#19954,.F.);
#28551=ORIENTED_EDGE('',*,*,#20186,.T.);
#28552=ORIENTED_EDGE('',*,*,#20187,.F.);
#28553=ORIENTED_EDGE('',*,*,#20142,.F.);
#28554=ORIENTED_EDGE('',*,*,#20143,.F.);
#28555=ORIENTED_EDGE('',*,*,#20187,.T.);
#28556=ORIENTED_EDGE('',*,*,#20188,.T.);
#28557=ORIENTED_EDGE('',*,*,#19952,.F.);
#28558=ORIENTED_EDGE('',*,*,#19953,.F.);
#28559=ORIENTED_EDGE('',*,*,#20188,.F.);
#28560=ORIENTED_EDGE('',*,*,#20186,.F.);
#28561=ORIENTED_EDGE('',*,*,#19949,.F.);
#28562=ORIENTED_EDGE('',*,*,#20189,.F.);
#28563=ORIENTED_EDGE('',*,*,#20190,.F.);
#28564=ORIENTED_EDGE('',*,*,#19950,.F.);
#28565=ORIENTED_EDGE('',*,*,#20190,.T.);
#28566=ORIENTED_EDGE('',*,*,#20191,.F.);
#28567=ORIENTED_EDGE('',*,*,#20144,.F.);
#28568=ORIENTED_EDGE('',*,*,#19948,.F.);
#28569=ORIENTED_EDGE('',*,*,#20145,.F.);
#28570=ORIENTED_EDGE('',*,*,#20191,.T.);
#28571=ORIENTED_EDGE('',*,*,#20189,.T.);
#28572=ORIENTED_EDGE('',*,*,#19946,.F.);
#28573=ORIENTED_EDGE('',*,*,#20192,.T.);
#28574=ORIENTED_EDGE('',*,*,#20193,.F.);
#28575=ORIENTED_EDGE('',*,*,#20146,.F.);
#28576=ORIENTED_EDGE('',*,*,#20147,.F.);
#28577=ORIENTED_EDGE('',*,*,#20193,.T.);
#28578=ORIENTED_EDGE('',*,*,#20194,.T.);
#28579=ORIENTED_EDGE('',*,*,#19944,.F.);
#28580=ORIENTED_EDGE('',*,*,#19945,.F.);
#28581=ORIENTED_EDGE('',*,*,#20194,.F.);
#28582=ORIENTED_EDGE('',*,*,#20192,.F.);
#28583=ORIENTED_EDGE('',*,*,#19941,.F.);
#28584=ORIENTED_EDGE('',*,*,#20195,.F.);
#28585=ORIENTED_EDGE('',*,*,#20196,.F.);
#28586=ORIENTED_EDGE('',*,*,#19942,.F.);
#28587=ORIENTED_EDGE('',*,*,#20196,.T.);
#28588=ORIENTED_EDGE('',*,*,#20197,.F.);
#28589=ORIENTED_EDGE('',*,*,#20148,.F.);
#28590=ORIENTED_EDGE('',*,*,#19940,.F.);
#28591=ORIENTED_EDGE('',*,*,#20149,.F.);
#28592=ORIENTED_EDGE('',*,*,#20197,.T.);
#28593=ORIENTED_EDGE('',*,*,#20195,.T.);
#28594=ORIENTED_EDGE('',*,*,#19938,.F.);
#28595=ORIENTED_EDGE('',*,*,#20198,.T.);
#28596=ORIENTED_EDGE('',*,*,#20199,.F.);
#28597=ORIENTED_EDGE('',*,*,#20150,.F.);
#28598=ORIENTED_EDGE('',*,*,#20083,.F.);
#28599=ORIENTED_EDGE('',*,*,#20199,.T.);
#28600=ORIENTED_EDGE('',*,*,#20200,.T.);
#28601=ORIENTED_EDGE('',*,*,#20077,.F.);
#28602=ORIENTED_EDGE('',*,*,#19933,.F.);
#28603=ORIENTED_EDGE('',*,*,#20200,.F.);
#28604=ORIENTED_EDGE('',*,*,#20198,.F.);
#28605=ORIENTED_EDGE('',*,*,#19937,.F.);
#28606=ORIENTED_EDGE('',*,*,#20074,.F.);
#28607=ORIENTED_EDGE('',*,*,#20201,.F.);
#28608=ORIENTED_EDGE('',*,*,#20202,.F.);
#28609=ORIENTED_EDGE('',*,*,#20075,.F.);
#28610=ORIENTED_EDGE('',*,*,#20202,.T.);
#28611=ORIENTED_EDGE('',*,*,#20203,.F.);
#28612=ORIENTED_EDGE('',*,*,#20084,.F.);
#28613=ORIENTED_EDGE('',*,*,#20073,.F.);
#28614=ORIENTED_EDGE('',*,*,#20085,.F.);
#28615=ORIENTED_EDGE('',*,*,#20203,.T.);
#28616=ORIENTED_EDGE('',*,*,#20201,.T.);
#28617=ORIENTED_EDGE('',*,*,#20071,.F.);
#28618=ORIENTED_EDGE('',*,*,#20204,.T.);
#28619=ORIENTED_EDGE('',*,*,#20205,.F.);
#28620=ORIENTED_EDGE('',*,*,#20086,.F.);
#28621=ORIENTED_EDGE('',*,*,#20087,.F.);
#28622=ORIENTED_EDGE('',*,*,#20205,.T.);
#28623=ORIENTED_EDGE('',*,*,#20206,.T.);
#28624=ORIENTED_EDGE('',*,*,#20069,.F.);
#28625=ORIENTED_EDGE('',*,*,#20070,.F.);
#28626=ORIENTED_EDGE('',*,*,#20206,.F.);
#28627=ORIENTED_EDGE('',*,*,#20204,.F.);
#28628=ORIENTED_EDGE('',*,*,#20066,.F.);
#28629=ORIENTED_EDGE('',*,*,#20207,.F.);
#28630=ORIENTED_EDGE('',*,*,#20208,.F.);
#28631=ORIENTED_EDGE('',*,*,#20067,.F.);
#28632=ORIENTED_EDGE('',*,*,#20208,.T.);
#28633=ORIENTED_EDGE('',*,*,#20209,.F.);
#28634=ORIENTED_EDGE('',*,*,#20088,.F.);
#28635=ORIENTED_EDGE('',*,*,#20065,.F.);
#28636=ORIENTED_EDGE('',*,*,#20089,.F.);
#28637=ORIENTED_EDGE('',*,*,#20209,.T.);
#28638=ORIENTED_EDGE('',*,*,#20207,.T.);
#28639=ORIENTED_EDGE('',*,*,#20063,.F.);
#28640=ORIENTED_EDGE('',*,*,#20210,.T.);
#28641=ORIENTED_EDGE('',*,*,#20211,.F.);
#28642=ORIENTED_EDGE('',*,*,#20090,.F.);
#28643=ORIENTED_EDGE('',*,*,#20091,.F.);
#28644=ORIENTED_EDGE('',*,*,#20211,.T.);
#28645=ORIENTED_EDGE('',*,*,#20212,.T.);
#28646=ORIENTED_EDGE('',*,*,#20061,.F.);
#28647=ORIENTED_EDGE('',*,*,#20062,.F.);
#28648=ORIENTED_EDGE('',*,*,#20212,.F.);
#28649=ORIENTED_EDGE('',*,*,#20210,.F.);
#28650=ORIENTED_EDGE('',*,*,#20058,.F.);
#28651=ORIENTED_EDGE('',*,*,#20213,.F.);
#28652=ORIENTED_EDGE('',*,*,#20214,.F.);
#28653=ORIENTED_EDGE('',*,*,#20059,.F.);
#28654=ORIENTED_EDGE('',*,*,#20214,.T.);
#28655=ORIENTED_EDGE('',*,*,#20215,.F.);
#28656=ORIENTED_EDGE('',*,*,#20092,.F.);
#28657=ORIENTED_EDGE('',*,*,#20057,.F.);
#28658=ORIENTED_EDGE('',*,*,#20093,.F.);
#28659=ORIENTED_EDGE('',*,*,#20215,.T.);
#28660=ORIENTED_EDGE('',*,*,#20213,.T.);
#28661=ORIENTED_EDGE('',*,*,#20055,.F.);
#28662=ORIENTED_EDGE('',*,*,#20216,.T.);
#28663=ORIENTED_EDGE('',*,*,#20217,.F.);
#28664=ORIENTED_EDGE('',*,*,#20094,.F.);
#28665=ORIENTED_EDGE('',*,*,#20095,.F.);
#28666=ORIENTED_EDGE('',*,*,#20217,.T.);
#28667=ORIENTED_EDGE('',*,*,#20218,.T.);
#28668=ORIENTED_EDGE('',*,*,#20053,.F.);
#28669=ORIENTED_EDGE('',*,*,#20054,.F.);
#28670=ORIENTED_EDGE('',*,*,#20218,.F.);
#28671=ORIENTED_EDGE('',*,*,#20216,.F.);
#28672=ORIENTED_EDGE('',*,*,#20050,.F.);
#28673=ORIENTED_EDGE('',*,*,#20219,.F.);
#28674=ORIENTED_EDGE('',*,*,#20220,.F.);
#28675=ORIENTED_EDGE('',*,*,#20051,.F.);
#28676=ORIENTED_EDGE('',*,*,#20220,.T.);
#28677=ORIENTED_EDGE('',*,*,#20221,.F.);
#28678=ORIENTED_EDGE('',*,*,#20096,.F.);
#28679=ORIENTED_EDGE('',*,*,#20049,.F.);
#28680=ORIENTED_EDGE('',*,*,#20097,.F.);
#28681=ORIENTED_EDGE('',*,*,#20221,.T.);
#28682=ORIENTED_EDGE('',*,*,#20219,.T.);
#28683=ORIENTED_EDGE('',*,*,#20047,.F.);
#28684=ORIENTED_EDGE('',*,*,#20222,.T.);
#28685=ORIENTED_EDGE('',*,*,#20223,.F.);
#28686=ORIENTED_EDGE('',*,*,#20098,.F.);
#28687=ORIENTED_EDGE('',*,*,#20099,.F.);
#28688=ORIENTED_EDGE('',*,*,#20223,.T.);
#28689=ORIENTED_EDGE('',*,*,#20224,.T.);
#28690=ORIENTED_EDGE('',*,*,#20045,.F.);
#28691=ORIENTED_EDGE('',*,*,#20046,.F.);
#28692=ORIENTED_EDGE('',*,*,#20224,.F.);
#28693=ORIENTED_EDGE('',*,*,#20222,.F.);
#28694=ORIENTED_EDGE('',*,*,#20042,.F.);
#28695=ORIENTED_EDGE('',*,*,#20225,.F.);
#28696=ORIENTED_EDGE('',*,*,#20226,.F.);
#28697=ORIENTED_EDGE('',*,*,#20043,.F.);
#28698=ORIENTED_EDGE('',*,*,#20226,.T.);
#28699=ORIENTED_EDGE('',*,*,#20227,.F.);
#28700=ORIENTED_EDGE('',*,*,#20100,.F.);
#28701=ORIENTED_EDGE('',*,*,#20041,.F.);
#28702=ORIENTED_EDGE('',*,*,#20101,.F.);
#28703=ORIENTED_EDGE('',*,*,#20227,.T.);
#28704=ORIENTED_EDGE('',*,*,#20225,.T.);
#28705=ORIENTED_EDGE('',*,*,#20039,.F.);
#28706=ORIENTED_EDGE('',*,*,#20228,.T.);
#28707=ORIENTED_EDGE('',*,*,#20229,.F.);
#28708=ORIENTED_EDGE('',*,*,#20102,.F.);
#28709=ORIENTED_EDGE('',*,*,#20103,.F.);
#28710=ORIENTED_EDGE('',*,*,#20229,.T.);
#28711=ORIENTED_EDGE('',*,*,#20230,.T.);
#28712=ORIENTED_EDGE('',*,*,#20037,.F.);
#28713=ORIENTED_EDGE('',*,*,#20038,.F.);
#28714=ORIENTED_EDGE('',*,*,#20230,.F.);
#28715=ORIENTED_EDGE('',*,*,#20228,.F.);
#28716=ORIENTED_EDGE('',*,*,#20034,.F.);
#28717=ORIENTED_EDGE('',*,*,#20231,.F.);
#28718=ORIENTED_EDGE('',*,*,#20232,.F.);
#28719=ORIENTED_EDGE('',*,*,#20035,.F.);
#28720=ORIENTED_EDGE('',*,*,#20232,.T.);
#28721=ORIENTED_EDGE('',*,*,#20233,.F.);
#28722=ORIENTED_EDGE('',*,*,#20104,.F.);
#28723=ORIENTED_EDGE('',*,*,#20033,.F.);
#28724=ORIENTED_EDGE('',*,*,#20105,.F.);
#28725=ORIENTED_EDGE('',*,*,#20233,.T.);
#28726=ORIENTED_EDGE('',*,*,#20231,.T.);
#28727=ORIENTED_EDGE('',*,*,#20031,.F.);
#28728=ORIENTED_EDGE('',*,*,#20234,.T.);
#28729=ORIENTED_EDGE('',*,*,#20235,.F.);
#28730=ORIENTED_EDGE('',*,*,#20106,.F.);
#28731=ORIENTED_EDGE('',*,*,#20107,.F.);
#28732=ORIENTED_EDGE('',*,*,#20235,.T.);
#28733=ORIENTED_EDGE('',*,*,#20236,.T.);
#28734=ORIENTED_EDGE('',*,*,#20029,.F.);
#28735=ORIENTED_EDGE('',*,*,#20030,.F.);
#28736=ORIENTED_EDGE('',*,*,#20236,.F.);
#28737=ORIENTED_EDGE('',*,*,#20234,.F.);
#28738=ORIENTED_EDGE('',*,*,#20026,.F.);
#28739=ORIENTED_EDGE('',*,*,#20237,.F.);
#28740=ORIENTED_EDGE('',*,*,#20238,.F.);
#28741=ORIENTED_EDGE('',*,*,#20027,.F.);
#28742=ORIENTED_EDGE('',*,*,#20238,.T.);
#28743=ORIENTED_EDGE('',*,*,#20239,.F.);
#28744=ORIENTED_EDGE('',*,*,#20108,.F.);
#28745=ORIENTED_EDGE('',*,*,#20025,.F.);
#28746=ORIENTED_EDGE('',*,*,#20109,.F.);
#28747=ORIENTED_EDGE('',*,*,#20239,.T.);
#28748=ORIENTED_EDGE('',*,*,#20237,.T.);
#28749=ORIENTED_EDGE('',*,*,#20023,.F.);
#28750=ORIENTED_EDGE('',*,*,#20240,.T.);
#28751=ORIENTED_EDGE('',*,*,#20241,.F.);
#28752=ORIENTED_EDGE('',*,*,#20110,.F.);
#28753=ORIENTED_EDGE('',*,*,#20111,.F.);
#28754=ORIENTED_EDGE('',*,*,#20241,.T.);
#28755=ORIENTED_EDGE('',*,*,#20242,.T.);
#28756=ORIENTED_EDGE('',*,*,#20021,.F.);
#28757=ORIENTED_EDGE('',*,*,#20022,.F.);
#28758=ORIENTED_EDGE('',*,*,#20242,.F.);
#28759=ORIENTED_EDGE('',*,*,#20240,.F.);
#28760=ORIENTED_EDGE('',*,*,#20018,.F.);
#28761=ORIENTED_EDGE('',*,*,#20243,.F.);
#28762=ORIENTED_EDGE('',*,*,#20244,.F.);
#28763=ORIENTED_EDGE('',*,*,#20019,.F.);
#28764=ORIENTED_EDGE('',*,*,#20244,.T.);
#28765=ORIENTED_EDGE('',*,*,#20245,.F.);
#28766=ORIENTED_EDGE('',*,*,#20112,.F.);
#28767=ORIENTED_EDGE('',*,*,#20017,.F.);
#28768=ORIENTED_EDGE('',*,*,#20113,.F.);
#28769=ORIENTED_EDGE('',*,*,#20245,.T.);
#28770=ORIENTED_EDGE('',*,*,#20243,.T.);
#28771=ORIENTED_EDGE('',*,*,#20015,.F.);
#28772=ORIENTED_EDGE('',*,*,#20246,.T.);
#28773=ORIENTED_EDGE('',*,*,#20247,.F.);
#28774=ORIENTED_EDGE('',*,*,#20114,.F.);
#28775=ORIENTED_EDGE('',*,*,#20115,.F.);
#28776=ORIENTED_EDGE('',*,*,#20247,.T.);
#28777=ORIENTED_EDGE('',*,*,#20248,.T.);
#28778=ORIENTED_EDGE('',*,*,#20013,.F.);
#28779=ORIENTED_EDGE('',*,*,#20014,.F.);
#28780=ORIENTED_EDGE('',*,*,#20248,.F.);
#28781=ORIENTED_EDGE('',*,*,#20246,.F.);
#28782=ORIENTED_EDGE('',*,*,#20010,.F.);
#28783=ORIENTED_EDGE('',*,*,#20249,.F.);
#28784=ORIENTED_EDGE('',*,*,#20250,.F.);
#28785=ORIENTED_EDGE('',*,*,#20011,.F.);
#28786=ORIENTED_EDGE('',*,*,#20250,.T.);
#28787=ORIENTED_EDGE('',*,*,#20251,.F.);
#28788=ORIENTED_EDGE('',*,*,#20116,.F.);
#28789=ORIENTED_EDGE('',*,*,#20009,.F.);
#28790=ORIENTED_EDGE('',*,*,#20117,.F.);
#28791=ORIENTED_EDGE('',*,*,#20251,.T.);
#28792=ORIENTED_EDGE('',*,*,#20249,.T.);
#28793=ORIENTED_EDGE('',*,*,#20007,.F.);
#28794=ORIENTED_EDGE('',*,*,#20252,.T.);
#28795=ORIENTED_EDGE('',*,*,#20253,.F.);
#28796=ORIENTED_EDGE('',*,*,#20118,.F.);
#28797=ORIENTED_EDGE('',*,*,#20119,.F.);
#28798=ORIENTED_EDGE('',*,*,#20253,.T.);
#28799=ORIENTED_EDGE('',*,*,#20254,.T.);
#28800=ORIENTED_EDGE('',*,*,#20005,.F.);
#28801=ORIENTED_EDGE('',*,*,#20006,.F.);
#28802=ORIENTED_EDGE('',*,*,#20254,.F.);
#28803=ORIENTED_EDGE('',*,*,#20252,.F.);
#28804=ORIENTED_EDGE('',*,*,#19922,.T.);
#28805=ORIENTED_EDGE('',*,*,#20255,.T.);
#28806=ORIENTED_EDGE('',*,*,#19935,.T.);
#28807=ORIENTED_EDGE('',*,*,#19936,.T.);
#28808=ORIENTED_EDGE('',*,*,#20255,.F.);
#28809=ORIENTED_EDGE('',*,*,#20152,.F.);
#28810=ORIENTED_EDGE('',*,*,#20256,.T.);
#28811=ORIENTED_EDGE('',*,*,#20257,.F.);
#28812=ORIENTED_EDGE('',*,*,#20258,.F.);
#28813=ORIENTED_EDGE('',*,*,#20259,.F.);
#28814=ORIENTED_EDGE('',*,*,#20260,.F.);
#28815=ORIENTED_EDGE('',*,*,#20261,.F.);
#28816=ORIENTED_EDGE('',*,*,#20262,.F.);
#28817=ORIENTED_EDGE('',*,*,#20263,.F.);
#28818=ORIENTED_EDGE('',*,*,#20264,.F.);
#28819=ORIENTED_EDGE('',*,*,#20265,.F.);
#28820=ORIENTED_EDGE('',*,*,#20266,.F.);
#28821=ORIENTED_EDGE('',*,*,#20267,.F.);
#28822=ORIENTED_EDGE('',*,*,#20268,.F.);
#28823=ORIENTED_EDGE('',*,*,#20269,.F.);
#28824=ORIENTED_EDGE('',*,*,#20270,.F.);
#28825=ORIENTED_EDGE('',*,*,#20271,.F.);
#28826=ORIENTED_EDGE('',*,*,#20272,.F.);
#28827=ORIENTED_EDGE('',*,*,#20273,.F.);
#28828=ORIENTED_EDGE('',*,*,#20274,.F.);
#28829=ORIENTED_EDGE('',*,*,#20275,.T.);
#28830=ORIENTED_EDGE('',*,*,#20256,.F.);
#28831=ORIENTED_EDGE('',*,*,#20275,.F.);
#28832=ORIENTED_EDGE('',*,*,#20276,.F.);
#28833=ORIENTED_EDGE('',*,*,#20273,.T.);
#28834=ORIENTED_EDGE('',*,*,#20277,.F.);
#28835=ORIENTED_EDGE('',*,*,#20278,.F.);
#28836=ORIENTED_EDGE('',*,*,#20279,.F.);
#28837=ORIENTED_EDGE('',*,*,#20280,.F.);
#28838=ORIENTED_EDGE('',*,*,#20281,.F.);
#28839=ORIENTED_EDGE('',*,*,#20270,.T.);
#28840=ORIENTED_EDGE('',*,*,#20282,.F.);
#28841=ORIENTED_EDGE('',*,*,#20258,.T.);
#28842=ORIENTED_EDGE('',*,*,#20283,.F.);
#28843=ORIENTED_EDGE('',*,*,#20284,.F.);
#28844=ORIENTED_EDGE('',*,*,#20285,.F.);
#28845=ORIENTED_EDGE('',*,*,#20286,.F.);
#28846=ORIENTED_EDGE('',*,*,#20287,.F.);
#28847=ORIENTED_EDGE('',*,*,#20267,.T.);
#28848=ORIENTED_EDGE('',*,*,#20288,.F.);
#28849=ORIENTED_EDGE('',*,*,#20261,.T.);
#28850=ORIENTED_EDGE('',*,*,#20289,.F.);
#28851=ORIENTED_EDGE('',*,*,#20290,.F.);
#28852=ORIENTED_EDGE('',*,*,#20291,.F.);
#28853=ORIENTED_EDGE('',*,*,#20292,.F.);
#28854=ORIENTED_EDGE('',*,*,#20293,.F.);
#28855=ORIENTED_EDGE('',*,*,#20264,.T.);
#28856=ORIENTED_EDGE('',*,*,#20262,.T.);
#28857=ORIENTED_EDGE('',*,*,#20288,.T.);
#28858=ORIENTED_EDGE('',*,*,#20294,.F.);
#28859=ORIENTED_EDGE('',*,*,#20289,.T.);
#28860=ORIENTED_EDGE('',*,*,#20260,.T.);
#28861=ORIENTED_EDGE('',*,*,#20295,.T.);
#28862=ORIENTED_EDGE('',*,*,#20296,.T.);
#28863=ORIENTED_EDGE('',*,*,#20297,.F.);
#28864=ORIENTED_EDGE('',*,*,#20259,.T.);
#28865=ORIENTED_EDGE('',*,*,#20282,.T.);
#28866=ORIENTED_EDGE('',*,*,#20298,.F.);
#28867=ORIENTED_EDGE('',*,*,#20283,.T.);
#28868=ORIENTED_EDGE('',*,*,#20257,.T.);
#28869=ORIENTED_EDGE('',*,*,#20299,.T.);
#28870=ORIENTED_EDGE('',*,*,#20300,.T.);
#28871=ORIENTED_EDGE('',*,*,#20295,.F.);
#28872=ORIENTED_EDGE('',*,*,#20274,.T.);
#28873=ORIENTED_EDGE('',*,*,#20276,.T.);
#28874=ORIENTED_EDGE('',*,*,#20301,.F.);
#28875=ORIENTED_EDGE('',*,*,#20277,.T.);
#28876=ORIENTED_EDGE('',*,*,#20272,.T.);
#28877=ORIENTED_EDGE('',*,*,#20302,.T.);
#28878=ORIENTED_EDGE('',*,*,#20303,.T.);
#28879=ORIENTED_EDGE('',*,*,#20299,.F.);
#28880=ORIENTED_EDGE('',*,*,#20278,.T.);
#28881=ORIENTED_EDGE('',*,*,#20301,.T.);
#28882=ORIENTED_EDGE('',*,*,#20284,.T.);
#28883=ORIENTED_EDGE('',*,*,#20298,.T.);
#28884=ORIENTED_EDGE('',*,*,#20280,.T.);
#28885=ORIENTED_EDGE('',*,*,#20304,.T.);
#28886=ORIENTED_EDGE('',*,*,#20290,.T.);
#28887=ORIENTED_EDGE('',*,*,#20294,.T.);
#28888=ORIENTED_EDGE('',*,*,#20286,.T.);
#28889=ORIENTED_EDGE('',*,*,#20305,.T.);
#28890=ORIENTED_EDGE('',*,*,#20292,.T.);
#28891=ORIENTED_EDGE('',*,*,#20306,.T.);
#28892=ORIENTED_EDGE('',*,*,#20307,.F.);
#28893=ORIENTED_EDGE('',*,*,#20308,.F.);
#28894=ORIENTED_EDGE('',*,*,#20309,.F.);
#28895=ORIENTED_EDGE('',*,*,#20310,.F.);
#28896=ORIENTED_EDGE('',*,*,#20303,.F.);
#28897=ORIENTED_EDGE('',*,*,#20311,.F.);
#28898=ORIENTED_EDGE('',*,*,#20300,.F.);
#28899=ORIENTED_EDGE('',*,*,#20312,.F.);
#28900=ORIENTED_EDGE('',*,*,#20296,.F.);
#28901=ORIENTED_EDGE('',*,*,#20313,.F.);
#28902=ORIENTED_EDGE('',*,*,#20314,.F.);
#28903=ORIENTED_EDGE('',*,*,#20315,.F.);
#28904=ORIENTED_EDGE('',*,*,#20316,.T.);
#28905=ORIENTED_EDGE('',*,*,#20311,.T.);
#28906=ORIENTED_EDGE('',*,*,#20310,.T.);
#28907=ORIENTED_EDGE('',*,*,#20308,.T.);
#28908=ORIENTED_EDGE('',*,*,#20315,.T.);
#28909=ORIENTED_EDGE('',*,*,#20313,.T.);
#28910=ORIENTED_EDGE('',*,*,#20312,.T.);
#28911=ORIENTED_EDGE('',*,*,#20316,.F.);
#28912=ORIENTED_EDGE('',*,*,#20266,.T.);
#28913=ORIENTED_EDGE('',*,*,#20317,.T.);
#28914=ORIENTED_EDGE('',*,*,#20307,.T.);
#28915=ORIENTED_EDGE('',*,*,#20318,.F.);
#28916=ORIENTED_EDGE('',*,*,#20268,.T.);
#28917=ORIENTED_EDGE('',*,*,#20287,.T.);
#28918=ORIENTED_EDGE('',*,*,#20305,.F.);
#28919=ORIENTED_EDGE('',*,*,#20285,.T.);
#28920=ORIENTED_EDGE('',*,*,#20263,.T.);
#28921=ORIENTED_EDGE('',*,*,#20297,.T.);
#28922=ORIENTED_EDGE('',*,*,#20314,.T.);
#28923=ORIENTED_EDGE('',*,*,#20317,.F.);
#28924=ORIENTED_EDGE('',*,*,#20265,.T.);
#28925=ORIENTED_EDGE('',*,*,#20293,.T.);
#28926=ORIENTED_EDGE('',*,*,#20306,.F.);
#28927=ORIENTED_EDGE('',*,*,#20291,.T.);
#28928=ORIENTED_EDGE('',*,*,#20269,.T.);
#28929=ORIENTED_EDGE('',*,*,#20318,.T.);
#28930=ORIENTED_EDGE('',*,*,#20309,.T.);
#28931=ORIENTED_EDGE('',*,*,#20302,.F.);
#28932=ORIENTED_EDGE('',*,*,#20271,.T.);
#28933=ORIENTED_EDGE('',*,*,#20281,.T.);
#28934=ORIENTED_EDGE('',*,*,#20304,.F.);
#28935=ORIENTED_EDGE('',*,*,#20279,.T.);
#30310=CONICAL_SURFACE('',#33619,1.2885,0.785398163397447);
#30311=CONICAL_SURFACE('',#33704,2.6,0.785398163397448);
#30312=CONICAL_SURFACE('',#33812,1.49337567297406,0.785398163397454);
#30313=CONICAL_SURFACE('',#33852,0.721687836487032,1.02974425867665);
#31657=ADVANCED_FACE('',(#4682),#1890,.T.);
#31658=ADVANCED_FACE('',(#4683),#1891,.T.);
#31659=ADVANCED_FACE('',(#4684),#1892,.T.);
#31660=ADVANCED_FACE('',(#4685),#1893,.T.);
#31661=ADVANCED_FACE('',(#4686),#1894,.T.);
#31662=ADVANCED_FACE('',(#4687),#1895,.T.);
#31663=ADVANCED_FACE('',(#4688),#1896,.T.);
#31664=ADVANCED_FACE('',(#4689),#1897,.T.);
#31665=ADVANCED_FACE('',(#4690),#1898,.T.);
#31666=ADVANCED_FACE('',(#4691),#1899,.T.);
#31667=ADVANCED_FACE('',(#4692),#1900,.T.);
#31668=ADVANCED_FACE('',(#4693),#1901,.T.);
#31669=ADVANCED_FACE('',(#4694),#1902,.T.);
#31670=ADVANCED_FACE('',(#4695),#1903,.T.);
#31671=ADVANCED_FACE('',(#4696),#1904,.T.);
#31672=ADVANCED_FACE('',(#4697),#1905,.T.);
#31673=ADVANCED_FACE('',(#4698),#1906,.T.);
#31674=ADVANCED_FACE('',(#4699),#1907,.T.);
#31675=ADVANCED_FACE('',(#4700),#1908,.T.);
#31676=ADVANCED_FACE('',(#4701),#1909,.T.);
#31677=ADVANCED_FACE('',(#4702),#1910,.T.);
#31678=ADVANCED_FACE('',(#4703),#1911,.T.);
#31679=ADVANCED_FACE('',(#4704),#1912,.T.);
#31680=ADVANCED_FACE('',(#4705),#1913,.T.);
#31681=ADVANCED_FACE('',(#4706),#1914,.T.);
#31682=ADVANCED_FACE('',(#4707),#1915,.T.);
#31683=ADVANCED_FACE('',(#4708),#1916,.T.);
#31684=ADVANCED_FACE('',(#4709),#1917,.T.);
#31685=ADVANCED_FACE('',(#4710),#1918,.T.);
#31686=ADVANCED_FACE('',(#4711),#1919,.T.);
#31687=ADVANCED_FACE('',(#4712),#1920,.T.);
#31688=ADVANCED_FACE('',(#4713),#1921,.T.);
#31689=ADVANCED_FACE('',(#4714),#1922,.T.);
#31690=ADVANCED_FACE('',(#4715),#1923,.T.);
#31691=ADVANCED_FACE('',(#4716),#1924,.T.);
#31692=ADVANCED_FACE('',(#4717),#1925,.T.);
#31693=ADVANCED_FACE('',(#4718),#1926,.T.);
#31694=ADVANCED_FACE('',(#4719),#1927,.T.);
#31695=ADVANCED_FACE('',(#4720),#1928,.T.);
#31696=ADVANCED_FACE('',(#4721),#1929,.T.);
#31697=ADVANCED_FACE('',(#4722),#1930,.T.);
#31698=ADVANCED_FACE('',(#4723),#1931,.T.);
#31699=ADVANCED_FACE('',(#4724),#1932,.T.);
#31700=ADVANCED_FACE('',(#4725),#1933,.T.);
#31701=ADVANCED_FACE('',(#4726),#1934,.T.);
#31702=ADVANCED_FACE('',(#4727),#1935,.T.);
#31703=ADVANCED_FACE('',(#4728),#1936,.T.);
#31704=ADVANCED_FACE('',(#4729),#1937,.T.);
#31705=ADVANCED_FACE('',(#4730),#3076,.F.);
#31706=ADVANCED_FACE('',(#4731),#611,.F.);
#31707=ADVANCED_FACE('',(#4732),#3077,.T.);
#31708=ADVANCED_FACE('',(#4733),#612,.F.);
#31709=ADVANCED_FACE('',(#4734),#95,.F.);
#31710=ADVANCED_FACE('',(#4735,#2227),#3078,.T.);
#31711=ADVANCED_FACE('',(#4736),#30310,.T.);
#31712=ADVANCED_FACE('',(#4737),#3079,.T.);
#31713=ADVANCED_FACE('',(#4738),#3080,.F.);
#31714=ADVANCED_FACE('',(#4739),#3081,.F.);
#31715=ADVANCED_FACE('',(#4740),#3082,.F.);
#31716=ADVANCED_FACE('',(#4741),#1938,.T.);
#31717=ADVANCED_FACE('',(#4742),#3083,.F.);
#31718=ADVANCED_FACE('',(#4743),#3084,.F.);
#31719=ADVANCED_FACE('',(#4744),#3085,.F.);
#31720=ADVANCED_FACE('',(#4745),#30311,.T.);
#31721=ADVANCED_FACE('',(#4746),#3086,.F.);
#31722=ADVANCED_FACE('',(#4747),#3087,.F.);
#31723=ADVANCED_FACE('',(#4748),#3088,.F.);
#31724=ADVANCED_FACE('',(#4749),#3089,.F.);
#31725=ADVANCED_FACE('',(#4750),#3090,.F.);
#31726=ADVANCED_FACE('',(#4751),#3091,.F.);
#31727=ADVANCED_FACE('',(#4752),#3092,.F.);
#31728=ADVANCED_FACE('',(#4753),#3093,.F.);
#31729=ADVANCED_FACE('',(#4754),#3094,.F.);
#31730=ADVANCED_FACE('',(#4755),#3095,.F.);
#31731=ADVANCED_FACE('',(#4756),#3096,.F.);
#31732=ADVANCED_FACE('',(#4757),#3097,.F.);
#31733=ADVANCED_FACE('',(#4758),#3098,.F.);
#31734=ADVANCED_FACE('',(#4759),#3099,.F.);
#31735=ADVANCED_FACE('',(#4760),#3100,.F.);
#31736=ADVANCED_FACE('',(#4761),#3101,.F.);
#31737=ADVANCED_FACE('',(#4762),#3102,.F.);
#31738=ADVANCED_FACE('',(#4763),#3103,.F.);
#31739=ADVANCED_FACE('',(#4764),#3104,.F.);
#31740=ADVANCED_FACE('',(#4765),#3105,.F.);
#31741=ADVANCED_FACE('',(#4766),#3106,.F.);
#31742=ADVANCED_FACE('',(#4767),#3107,.F.);
#31743=ADVANCED_FACE('',(#4768),#3108,.F.);
#31744=ADVANCED_FACE('',(#4769),#3109,.F.);
#31745=ADVANCED_FACE('',(#4770),#3110,.F.);
#31746=ADVANCED_FACE('',(#4771),#3111,.F.);
#31747=ADVANCED_FACE('',(#4772),#3112,.F.);
#31748=ADVANCED_FACE('',(#4773),#3113,.F.);
#31749=ADVANCED_FACE('',(#4774),#3114,.F.);
#31750=ADVANCED_FACE('',(#4775),#3115,.F.);
#31751=ADVANCED_FACE('',(#4776),#3116,.F.);
#31752=ADVANCED_FACE('',(#4777),#3117,.F.);
#31753=ADVANCED_FACE('',(#4778),#3118,.F.);
#31754=ADVANCED_FACE('',(#4779),#3119,.F.);
#31755=ADVANCED_FACE('',(#4780),#3120,.F.);
#31756=ADVANCED_FACE('',(#4781),#3121,.F.);
#31757=ADVANCED_FACE('',(#4782),#3122,.F.);
#31758=ADVANCED_FACE('',(#4783),#3123,.F.);
#31759=ADVANCED_FACE('',(#4784),#3124,.F.);
#31760=ADVANCED_FACE('',(#4785),#3125,.F.);
#31761=ADVANCED_FACE('',(#4786),#3126,.F.);
#31762=ADVANCED_FACE('',(#4787),#3127,.F.);
#31763=ADVANCED_FACE('',(#4788),#3128,.F.);
#31764=ADVANCED_FACE('',(#4789),#3129,.F.);
#31765=ADVANCED_FACE('',(#4790),#3130,.F.);
#31766=ADVANCED_FACE('',(#4791),#3131,.F.);
#31767=ADVANCED_FACE('',(#4792),#3132,.F.);
#31768=ADVANCED_FACE('',(#4793),#3133,.F.);
#31769=ADVANCED_FACE('',(#4794),#3134,.F.);
#31770=ADVANCED_FACE('',(#4795),#3135,.F.);
#31771=ADVANCED_FACE('',(#4796),#3136,.F.);
#31772=ADVANCED_FACE('',(#4797),#3137,.F.);
#31773=ADVANCED_FACE('',(#4798),#3138,.F.);
#31774=ADVANCED_FACE('',(#4799),#3139,.F.);
#31775=ADVANCED_FACE('',(#4800),#3140,.F.);
#31776=ADVANCED_FACE('',(#4801),#3141,.F.);
#31777=ADVANCED_FACE('',(#4802),#3142,.F.);
#31778=ADVANCED_FACE('',(#4803),#3143,.F.);
#31779=ADVANCED_FACE('',(#4804),#3144,.F.);
#31780=ADVANCED_FACE('',(#4805),#3145,.F.);
#31781=ADVANCED_FACE('',(#4806),#3146,.F.);
#31782=ADVANCED_FACE('',(#4807),#3147,.F.);
#31783=ADVANCED_FACE('',(#4808),#3148,.F.);
#31784=ADVANCED_FACE('',(#4809),#3149,.F.);
#31785=ADVANCED_FACE('',(#4810),#3150,.F.);
#31786=ADVANCED_FACE('',(#4811),#3151,.F.);
#31787=ADVANCED_FACE('',(#4812),#3152,.F.);
#31788=ADVANCED_FACE('',(#4813),#3153,.F.);
#31789=ADVANCED_FACE('',(#4814),#3154,.F.);
#31790=ADVANCED_FACE('',(#4815),#3155,.F.);
#31791=ADVANCED_FACE('',(#4816),#3156,.F.);
#31792=ADVANCED_FACE('',(#4817),#3157,.F.);
#31793=ADVANCED_FACE('',(#4818),#3158,.F.);
#31794=ADVANCED_FACE('',(#4819),#3159,.F.);
#31795=ADVANCED_FACE('',(#4820),#3160,.F.);
#31796=ADVANCED_FACE('',(#4821),#3161,.F.);
#31797=ADVANCED_FACE('',(#4822),#3162,.F.);
#31798=ADVANCED_FACE('',(#4823),#3163,.F.);
#31799=ADVANCED_FACE('',(#4824),#3164,.F.);
#31800=ADVANCED_FACE('',(#4825),#3165,.F.);
#31801=ADVANCED_FACE('',(#4826),#3166,.F.);
#31802=ADVANCED_FACE('',(#4827),#3167,.F.);
#31803=ADVANCED_FACE('',(#4828),#3168,.F.);
#31804=ADVANCED_FACE('',(#4829),#3169,.F.);
#31805=ADVANCED_FACE('',(#4830),#3170,.F.);
#31806=ADVANCED_FACE('',(#4831),#3171,.F.);
#31807=ADVANCED_FACE('',(#4832),#3172,.F.);
#31808=ADVANCED_FACE('',(#4833),#3173,.F.);
#31809=ADVANCED_FACE('',(#4834),#3174,.F.);
#31810=ADVANCED_FACE('',(#4835),#3175,.F.);
#31811=ADVANCED_FACE('',(#4836),#3176,.F.);
#31812=ADVANCED_FACE('',(#4837),#3177,.F.);
#31813=ADVANCED_FACE('',(#4838),#3178,.F.);
#31814=ADVANCED_FACE('',(#4839),#3179,.F.);
#31815=ADVANCED_FACE('',(#4840),#3180,.F.);
#31816=ADVANCED_FACE('',(#4841),#3181,.F.);
#31817=ADVANCED_FACE('',(#4842),#3182,.F.);
#31818=ADVANCED_FACE('',(#4843),#3183,.F.);
#31819=ADVANCED_FACE('',(#4844),#3184,.F.);
#31820=ADVANCED_FACE('',(#4845),#3185,.F.);
#31821=ADVANCED_FACE('',(#4846),#3186,.F.);
#31822=ADVANCED_FACE('',(#4847),#3187,.F.);
#31823=ADVANCED_FACE('',(#4848),#96,.T.);
#31824=ADVANCED_FACE('',(#4849,#2228),#3188,.F.);
#31825=ADVANCED_FACE('',(#4850),#30312,.F.);
#31826=ADVANCED_FACE('',(#4851),#1939,.T.);
#31827=ADVANCED_FACE('',(#4852),#1940,.T.);
#31828=ADVANCED_FACE('',(#4853),#1941,.T.);
#31829=ADVANCED_FACE('',(#4854),#1942,.T.);
#31830=ADVANCED_FACE('',(#4855),#1943,.T.);
#31831=ADVANCED_FACE('',(#4856),#1944,.T.);
#31832=ADVANCED_FACE('',(#4857),#3189,.F.);
#31833=ADVANCED_FACE('',(#4858),#3190,.F.);
#31834=ADVANCED_FACE('',(#4859),#3191,.F.);
#31835=ADVANCED_FACE('',(#4860),#3192,.F.);
#31836=ADVANCED_FACE('',(#4861),#3193,.F.);
#31837=ADVANCED_FACE('',(#4862),#3194,.F.);
#31838=ADVANCED_FACE('',(#4863),#3195,.F.);
#31839=ADVANCED_FACE('',(#4864),#3196,.F.);
#31840=ADVANCED_FACE('',(#4865),#3197,.F.);
#31841=ADVANCED_FACE('',(#4866),#3198,.F.);
#31842=ADVANCED_FACE('',(#4867),#3199,.F.);
#31843=ADVANCED_FACE('',(#4868),#3200,.F.);
#31844=ADVANCED_FACE('',(#4869),#3201,.F.);
#31845=ADVANCED_FACE('',(#4870),#3202,.F.);
#31846=ADVANCED_FACE('',(#4871),#3203,.F.);
#31847=ADVANCED_FACE('',(#4872),#30313,.F.);
#31848=ADVANCED_FACE('',(#4873),#3204,.F.);
#31849=ADVANCED_FACE('',(#4874),#3205,.F.);
#31850=ADVANCED_FACE('',(#4875),#3206,.F.);
#32085=CLOSED_SHELL('',(#31657,#31658,#31659,#31660,#31661,#31662,#31663,
#31664,#31665,#31666,#31667,#31668,#31669,#31670,#31671,#31672,#31673,#31674,
#31675,#31676,#31677,#31678,#31679,#31680,#31681,#31682,#31683,#31684,#31685,
#31686,#31687,#31688,#31689,#31690,#31691,#31692,#31693,#31694,#31695,#31696,
#31697,#31698,#31699,#31700,#31701,#31702,#31703,#31704,#31705,#31706,#31707,
#31708,#31709,#31710,#31711,#31712,#31713,#31714,#31715,#31716,#31717,#31718,
#31719,#31720,#31721,#31722,#31723,#31724,#31725,#31726,#31727,#31728,#31729,
#31730,#31731,#31732,#31733,#31734,#31735,#31736,#31737,#31738,#31739,#31740,
#31741,#31742,#31743,#31744,#31745,#31746,#31747,#31748,#31749,#31750,#31751,
#31752,#31753,#31754,#31755,#31756,#31757,#31758,#31759,#31760,#31761,#31762,
#31763,#31764,#31765,#31766,#31767,#31768,#31769,#31770,#31771,#31772,#31773,
#31774,#31775,#31776,#31777,#31778,#31779,#31780,#31781,#31782,#31783,#31784,
#31785,#31786,#31787,#31788,#31789,#31790,#31791,#31792,#31793,#31794,#31795,
#31796,#31797,#31798,#31799,#31800,#31801,#31802,#31803,#31804,#31805,#31806,
#31807,#31808,#31809,#31810,#31811,#31812,#31813,#31814,#31815,#31816,#31817,
#31818,#31819,#31820,#31821,#31822,#31823,#31824,#31825,#31826,#31827,#31828,
#31829,#31830,#31831,#31832,#31833,#31834,#31835,#31836,#31837,#31838,#31839,
#31840,#31841,#31842,#31843,#31844,#31845,#31846,#31847,#31848,#31849,#31850));
#33555=AXIS2_PLACEMENT_3D('',#84334,#39162,#39163);
#33556=AXIS2_PLACEMENT_3D('',#84335,#39164,#39165);
#33557=AXIS2_PLACEMENT_3D('',#84411,#39167,#39168);
#33558=AXIS2_PLACEMENT_3D('',#84443,#39169,#39170);
#33559=AXIS2_PLACEMENT_3D('',#84869,#39172,#39173);
#33560=AXIS2_PLACEMENT_3D('',#85329,#39175,#39176);
#33561=AXIS2_PLACEMENT_3D('',#85819,#39178,#39179);
#33562=AXIS2_PLACEMENT_3D('',#86285,#39181,#39182);
#33563=AXIS2_PLACEMENT_3D('',#86745,#39184,#39185);
#33564=AXIS2_PLACEMENT_3D('',#87215,#39187,#39188);
#33565=AXIS2_PLACEMENT_3D('',#87699,#39190,#39191);
#33566=AXIS2_PLACEMENT_3D('',#88163,#39193,#39194);
#33567=AXIS2_PLACEMENT_3D('',#88637,#39196,#39197);
#33568=AXIS2_PLACEMENT_3D('',#89105,#39199,#39200);
#33569=AXIS2_PLACEMENT_3D('',#89563,#39202,#39203);
#33570=AXIS2_PLACEMENT_3D('',#90005,#39205,#39206);
#33571=AXIS2_PLACEMENT_3D('',#90481,#39208,#39209);
#33572=AXIS2_PLACEMENT_3D('',#90945,#39211,#39212);
#33573=AXIS2_PLACEMENT_3D('',#91389,#39214,#39215);
#33574=AXIS2_PLACEMENT_3D('',#91865,#39217,#39218);
#33575=AXIS2_PLACEMENT_3D('',#92309,#39220,#39221);
#33576=AXIS2_PLACEMENT_3D('',#92783,#39223,#39224);
#33577=AXIS2_PLACEMENT_3D('',#93289,#39226,#39227);
#33578=AXIS2_PLACEMENT_3D('',#93759,#39229,#39230);
#33579=AXIS2_PLACEMENT_3D('',#94223,#39232,#39233);
#33580=AXIS2_PLACEMENT_3D('',#94684,#39235,#39236);
#33581=AXIS2_PLACEMENT_3D('',#94804,#39238,#39239);
#33582=AXIS2_PLACEMENT_3D('',#94887,#39240,#39241);
#33583=AXIS2_PLACEMENT_3D('',#95361,#39243,#39244);
#33584=AXIS2_PLACEMENT_3D('',#95791,#39246,#39247);
#33585=AXIS2_PLACEMENT_3D('',#96219,#39249,#39250);
#33586=AXIS2_PLACEMENT_3D('',#96662,#39252,#39253);
#33587=AXIS2_PLACEMENT_3D('',#97103,#39255,#39256);
#33588=AXIS2_PLACEMENT_3D('',#97545,#39258,#39259);
#33589=AXIS2_PLACEMENT_3D('',#97969,#39261,#39262);
#33590=AXIS2_PLACEMENT_3D('',#98395,#39264,#39265);
#33591=AXIS2_PLACEMENT_3D('',#98843,#39267,#39268);
#33592=AXIS2_PLACEMENT_3D('',#99301,#39270,#39271);
#33593=AXIS2_PLACEMENT_3D('',#99727,#39273,#39274);
#33594=AXIS2_PLACEMENT_3D('',#100159,#39276,#39277);
#33595=AXIS2_PLACEMENT_3D('',#100583,#39279,#39280);
#33596=AXIS2_PLACEMENT_3D('',#101040,#39282,#39283);
#33597=AXIS2_PLACEMENT_3D('',#101458,#39285,#39286);
#33598=AXIS2_PLACEMENT_3D('',#101882,#39288,#39289);
#33599=AXIS2_PLACEMENT_3D('',#102318,#39291,#39292);
#33600=AXIS2_PLACEMENT_3D('',#102736,#39294,#39295);
#33601=AXIS2_PLACEMENT_3D('',#103174,#39297,#39298);
#33602=AXIS2_PLACEMENT_3D('',#103633,#39300,#39301);
#33603=AXIS2_PLACEMENT_3D('',#104047,#39303,#39304);
#33604=AXIS2_PLACEMENT_3D('',#104513,#39306,#39307);
#33605=AXIS2_PLACEMENT_3D('',#104702,#39308,#39309);
#33606=AXIS2_PLACEMENT_3D('',#104833,#39310,#39311);
#33607=AXIS2_PLACEMENT_3D('',#105072,#39312,#39313);
#33608=AXIS2_PLACEMENT_3D('',#105239,#39314,#39315);
#33609=AXIS2_PLACEMENT_3D('',#105242,#39316,#39317);
#33610=AXIS2_PLACEMENT_3D('',#105336,#39318,#39319);
#33611=AXIS2_PLACEMENT_3D('',#105961,#39320,#39321);
#33612=AXIS2_PLACEMENT_3D('',#105964,#39322,#39323);
#33613=AXIS2_PLACEMENT_3D('',#106044,#39324,#39325);
#33614=AXIS2_PLACEMENT_3D('',#106655,#39326,#39327);
#33615=AXIS2_PLACEMENT_3D('',#106657,#39328,#39329);
#33616=AXIS2_PLACEMENT_3D('',#106658,#39330,#39331);
#33617=AXIS2_PLACEMENT_3D('',#106659,#39332,#39333);
#33618=AXIS2_PLACEMENT_3D('',#106661,#39334,#39335);
#33619=AXIS2_PLACEMENT_3D('',#106662,#39336,#39337);
#33620=AXIS2_PLACEMENT_3D('',#106665,#39339,#39340);
#33621=AXIS2_PLACEMENT_3D('',#106666,#39341,#39342);
#33622=AXIS2_PLACEMENT_3D('',#106667,#39343,#39344);
#33623=AXIS2_PLACEMENT_3D('',#106670,#39345,#39346);
#33624=AXIS2_PLACEMENT_3D('',#106674,#39349,#39350);
#33625=AXIS2_PLACEMENT_3D('',#106682,#39353,#39354);
#33626=AXIS2_PLACEMENT_3D('',#106688,#39356,#39357);
#33627=AXIS2_PLACEMENT_3D('',#106691,#39358,#39359);
#33628=AXIS2_PLACEMENT_3D('',#106695,#39361,#39362);
#33629=AXIS2_PLACEMENT_3D('',#106696,#39363,#39364);
#33630=AXIS2_PLACEMENT_3D('',#106698,#39365,#39366);
#33631=AXIS2_PLACEMENT_3D('',#106702,#39368,#39369);
#33632=AXIS2_PLACEMENT_3D('',#106706,#39371,#39372);
#33633=AXIS2_PLACEMENT_3D('',#106710,#39374,#39375);
#33634=AXIS2_PLACEMENT_3D('',#106714,#39377,#39378);
#33635=AXIS2_PLACEMENT_3D('',#106718,#39380,#39381);
#33636=AXIS2_PLACEMENT_3D('',#106722,#39383,#39384);
#33637=AXIS2_PLACEMENT_3D('',#106726,#39386,#39387);
#33638=AXIS2_PLACEMENT_3D('',#106730,#39389,#39390);
#33639=AXIS2_PLACEMENT_3D('',#106734,#39392,#39393);
#33640=AXIS2_PLACEMENT_3D('',#106738,#39395,#39396);
#33641=AXIS2_PLACEMENT_3D('',#106742,#39398,#39399);
#33642=AXIS2_PLACEMENT_3D('',#106746,#39401,#39402);
#33643=AXIS2_PLACEMENT_3D('',#106750,#39404,#39405);
#33644=AXIS2_PLACEMENT_3D('',#106754,#39407,#39408);
#33645=AXIS2_PLACEMENT_3D('',#106758,#39410,#39411);
#33646=AXIS2_PLACEMENT_3D('',#106762,#39413,#39414);
#33647=AXIS2_PLACEMENT_3D('',#106766,#39416,#39417);
#33648=AXIS2_PLACEMENT_3D('',#106770,#39419,#39420);
#33649=AXIS2_PLACEMENT_3D('',#106774,#39422,#39423);
#33650=AXIS2_PLACEMENT_3D('',#106778,#39425,#39426);
#33651=AXIS2_PLACEMENT_3D('',#106782,#39428,#39429);
#33652=AXIS2_PLACEMENT_3D('',#106786,#39431,#39432);
#33653=AXIS2_PLACEMENT_3D('',#106790,#39434,#39435);
#33654=AXIS2_PLACEMENT_3D('',#106794,#39437,#39438);
#33655=AXIS2_PLACEMENT_3D('',#106798,#39440,#39441);
#33656=AXIS2_PLACEMENT_3D('',#106802,#39443,#39444);
#33657=AXIS2_PLACEMENT_3D('',#106806,#39446,#39447);
#33658=AXIS2_PLACEMENT_3D('',#106810,#39449,#39450);
#33659=AXIS2_PLACEMENT_3D('',#106814,#39452,#39453);
#33660=AXIS2_PLACEMENT_3D('',#106818,#39455,#39456);
#33661=AXIS2_PLACEMENT_3D('',#106822,#39458,#39459);
#33662=AXIS2_PLACEMENT_3D('',#106826,#39461,#39462);
#33663=AXIS2_PLACEMENT_3D('',#106829,#39464,#39465);
#33664=AXIS2_PLACEMENT_3D('',#106831,#39466,#39467);
#33665=AXIS2_PLACEMENT_3D('',#106835,#39469,#39470);
#33666=AXIS2_PLACEMENT_3D('',#106839,#39472,#39473);
#33667=AXIS2_PLACEMENT_3D('',#106843,#39475,#39476);
#33668=AXIS2_PLACEMENT_3D('',#106847,#39478,#39479);
#33669=AXIS2_PLACEMENT_3D('',#106851,#39481,#39482);
#33670=AXIS2_PLACEMENT_3D('',#106855,#39484,#39485);
#33671=AXIS2_PLACEMENT_3D('',#106859,#39487,#39488);
#33672=AXIS2_PLACEMENT_3D('',#106863,#39490,#39491);
#33673=AXIS2_PLACEMENT_3D('',#106867,#39493,#39494);
#33674=AXIS2_PLACEMENT_3D('',#106871,#39496,#39497);
#33675=AXIS2_PLACEMENT_3D('',#106875,#39499,#39500);
#33676=AXIS2_PLACEMENT_3D('',#106879,#39502,#39503);
#33677=AXIS2_PLACEMENT_3D('',#106883,#39505,#39506);
#33678=AXIS2_PLACEMENT_3D('',#106887,#39508,#39509);
#33679=AXIS2_PLACEMENT_3D('',#106891,#39511,#39512);
#33680=AXIS2_PLACEMENT_3D('',#106895,#39514,#39515);
#33681=AXIS2_PLACEMENT_3D('',#106899,#39517,#39518);
#33682=AXIS2_PLACEMENT_3D('',#106903,#39520,#39521);
#33683=AXIS2_PLACEMENT_3D('',#106907,#39523,#39524);
#33684=AXIS2_PLACEMENT_3D('',#106911,#39526,#39527);
#33685=AXIS2_PLACEMENT_3D('',#106915,#39529,#39530);
#33686=AXIS2_PLACEMENT_3D('',#106919,#39532,#39533);
#33687=AXIS2_PLACEMENT_3D('',#106923,#39535,#39536);
#33688=AXIS2_PLACEMENT_3D('',#106927,#39538,#39539);
#33689=AXIS2_PLACEMENT_3D('',#106931,#39541,#39542);
#33690=AXIS2_PLACEMENT_3D('',#106935,#39544,#39545);
#33691=AXIS2_PLACEMENT_3D('',#106939,#39547,#39548);
#33692=AXIS2_PLACEMENT_3D('',#106943,#39550,#39551);
#33693=AXIS2_PLACEMENT_3D('',#106947,#39553,#39554);
#33694=AXIS2_PLACEMENT_3D('',#106951,#39556,#39557);
#33695=AXIS2_PLACEMENT_3D('',#106955,#39559,#39560);
#33696=AXIS2_PLACEMENT_3D('',#106959,#39562,#39563);
#33697=AXIS2_PLACEMENT_3D('',#106963,#39565,#39566);
#33698=AXIS2_PLACEMENT_3D('',#106967,#39568,#39569);
#33699=AXIS2_PLACEMENT_3D('',#106971,#39571,#39572);
#33700=AXIS2_PLACEMENT_3D('',#106975,#39574,#39575);
#33701=AXIS2_PLACEMENT_3D('',#106977,#39577,#39578);
#33702=AXIS2_PLACEMENT_3D('',#106985,#39581,#39582);
#33703=AXIS2_PLACEMENT_3D('',#106990,#39584,#39585);
#33704=AXIS2_PLACEMENT_3D('',#106991,#39586,#39587);
#33705=AXIS2_PLACEMENT_3D('',#107232,#39589,#39590);
#33706=AXIS2_PLACEMENT_3D('',#107233,#39591,#39592);
#33707=AXIS2_PLACEMENT_3D('',#107237,#39595,#39596);
#33708=AXIS2_PLACEMENT_3D('',#107239,#39598,#39599);
#33709=AXIS2_PLACEMENT_3D('',#107240,#39600,#39601);
#33710=AXIS2_PLACEMENT_3D('',#107244,#39604,#39605);
#33711=AXIS2_PLACEMENT_3D('',#107246,#39607,#39608);
#33712=AXIS2_PLACEMENT_3D('',#107247,#39609,#39610);
#33713=AXIS2_PLACEMENT_3D('',#107251,#39613,#39614);
#33714=AXIS2_PLACEMENT_3D('',#107253,#39616,#39617);
#33715=AXIS2_PLACEMENT_3D('',#107254,#39618,#39619);
#33716=AXIS2_PLACEMENT_3D('',#107258,#39622,#39623);
#33717=AXIS2_PLACEMENT_3D('',#107260,#39625,#39626);
#33718=AXIS2_PLACEMENT_3D('',#107261,#39627,#39628);
#33719=AXIS2_PLACEMENT_3D('',#107265,#39631,#39632);
#33720=AXIS2_PLACEMENT_3D('',#107267,#39634,#39635);
#33721=AXIS2_PLACEMENT_3D('',#107268,#39636,#39637);
#33722=AXIS2_PLACEMENT_3D('',#107272,#39640,#39641);
#33723=AXIS2_PLACEMENT_3D('',#107274,#39643,#39644);
#33724=AXIS2_PLACEMENT_3D('',#107275,#39645,#39646);
#33725=AXIS2_PLACEMENT_3D('',#107279,#39649,#39650);
#33726=AXIS2_PLACEMENT_3D('',#107281,#39652,#39653);
#33727=AXIS2_PLACEMENT_3D('',#107282,#39654,#39655);
#33728=AXIS2_PLACEMENT_3D('',#107286,#39658,#39659);
#33729=AXIS2_PLACEMENT_3D('',#107288,#39661,#39662);
#33730=AXIS2_PLACEMENT_3D('',#107289,#39663,#39664);
#33731=AXIS2_PLACEMENT_3D('',#107293,#39667,#39668);
#33732=AXIS2_PLACEMENT_3D('',#107295,#39670,#39671);
#33733=AXIS2_PLACEMENT_3D('',#107296,#39672,#39673);
#33734=AXIS2_PLACEMENT_3D('',#107300,#39676,#39677);
#33735=AXIS2_PLACEMENT_3D('',#107302,#39679,#39680);
#33736=AXIS2_PLACEMENT_3D('',#107303,#39681,#39682);
#33737=AXIS2_PLACEMENT_3D('',#107307,#39685,#39686);
#33738=AXIS2_PLACEMENT_3D('',#107309,#39688,#39689);
#33739=AXIS2_PLACEMENT_3D('',#107310,#39690,#39691);
#33740=AXIS2_PLACEMENT_3D('',#107314,#39694,#39695);
#33741=AXIS2_PLACEMENT_3D('',#107316,#39697,#39698);
#33742=AXIS2_PLACEMENT_3D('',#107317,#39699,#39700);
#33743=AXIS2_PLACEMENT_3D('',#107321,#39703,#39704);
#33744=AXIS2_PLACEMENT_3D('',#107323,#39706,#39707);
#33745=AXIS2_PLACEMENT_3D('',#107324,#39708,#39709);
#33746=AXIS2_PLACEMENT_3D('',#107328,#39712,#39713);
#33747=AXIS2_PLACEMENT_3D('',#107330,#39715,#39716);
#33748=AXIS2_PLACEMENT_3D('',#107331,#39717,#39718);
#33749=AXIS2_PLACEMENT_3D('',#107335,#39721,#39722);
#33750=AXIS2_PLACEMENT_3D('',#107337,#39724,#39725);
#33751=AXIS2_PLACEMENT_3D('',#107338,#39726,#39727);
#33752=AXIS2_PLACEMENT_3D('',#107342,#39730,#39731);
#33753=AXIS2_PLACEMENT_3D('',#107344,#39733,#39734);
#33754=AXIS2_PLACEMENT_3D('',#107345,#39735,#39736);
#33755=AXIS2_PLACEMENT_3D('',#107349,#39739,#39740);
#33756=AXIS2_PLACEMENT_3D('',#107351,#39742,#39743);
#33757=AXIS2_PLACEMENT_3D('',#107352,#39744,#39745);
#33758=AXIS2_PLACEMENT_3D('',#107356,#39748,#39749);
#33759=AXIS2_PLACEMENT_3D('',#107358,#39751,#39752);
#33760=AXIS2_PLACEMENT_3D('',#107359,#39753,#39754);
#33761=AXIS2_PLACEMENT_3D('',#107363,#39757,#39758);
#33762=AXIS2_PLACEMENT_3D('',#107365,#39760,#39761);
#33763=AXIS2_PLACEMENT_3D('',#107366,#39762,#39763);
#33764=AXIS2_PLACEMENT_3D('',#107370,#39766,#39767);
#33765=AXIS2_PLACEMENT_3D('',#107372,#39769,#39770);
#33766=AXIS2_PLACEMENT_3D('',#107373,#39771,#39772);
#33767=AXIS2_PLACEMENT_3D('',#107377,#39775,#39776);
#33768=AXIS2_PLACEMENT_3D('',#107379,#39778,#39779);
#33769=AXIS2_PLACEMENT_3D('',#107380,#39780,#39781);
#33770=AXIS2_PLACEMENT_3D('',#107384,#39784,#39785);
#33771=AXIS2_PLACEMENT_3D('',#107386,#39787,#39788);
#33772=AXIS2_PLACEMENT_3D('',#107387,#39789,#39790);
#33773=AXIS2_PLACEMENT_3D('',#107391,#39793,#39794);
#33774=AXIS2_PLACEMENT_3D('',#107393,#39796,#39797);
#33775=AXIS2_PLACEMENT_3D('',#107394,#39798,#39799);
#33776=AXIS2_PLACEMENT_3D('',#107398,#39802,#39803);
#33777=AXIS2_PLACEMENT_3D('',#107400,#39805,#39806);
#33778=AXIS2_PLACEMENT_3D('',#107401,#39807,#39808);
#33779=AXIS2_PLACEMENT_3D('',#107405,#39811,#39812);
#33780=AXIS2_PLACEMENT_3D('',#107407,#39814,#39815);
#33781=AXIS2_PLACEMENT_3D('',#107408,#39816,#39817);
#33782=AXIS2_PLACEMENT_3D('',#107412,#39820,#39821);
#33783=AXIS2_PLACEMENT_3D('',#107414,#39823,#39824);
#33784=AXIS2_PLACEMENT_3D('',#107415,#39825,#39826);
#33785=AXIS2_PLACEMENT_3D('',#107419,#39829,#39830);
#33786=AXIS2_PLACEMENT_3D('',#107421,#39832,#39833);
#33787=AXIS2_PLACEMENT_3D('',#107422,#39834,#39835);
#33788=AXIS2_PLACEMENT_3D('',#107426,#39838,#39839);
#33789=AXIS2_PLACEMENT_3D('',#107428,#39841,#39842);
#33790=AXIS2_PLACEMENT_3D('',#107429,#39843,#39844);
#33791=AXIS2_PLACEMENT_3D('',#107433,#39847,#39848);
#33792=AXIS2_PLACEMENT_3D('',#107435,#39850,#39851);
#33793=AXIS2_PLACEMENT_3D('',#107436,#39852,#39853);
#33794=AXIS2_PLACEMENT_3D('',#107440,#39856,#39857);
#33795=AXIS2_PLACEMENT_3D('',#107442,#39859,#39860);
#33796=AXIS2_PLACEMENT_3D('',#107443,#39861,#39862);
#33797=AXIS2_PLACEMENT_3D('',#107447,#39865,#39866);
#33798=AXIS2_PLACEMENT_3D('',#107449,#39868,#39869);
#33799=AXIS2_PLACEMENT_3D('',#107450,#39870,#39871);
#33800=AXIS2_PLACEMENT_3D('',#107454,#39874,#39875);
#33801=AXIS2_PLACEMENT_3D('',#107456,#39877,#39878);
#33802=AXIS2_PLACEMENT_3D('',#107457,#39879,#39880);
#33803=AXIS2_PLACEMENT_3D('',#107461,#39883,#39884);
#33804=AXIS2_PLACEMENT_3D('',#107463,#39886,#39887);
#33805=AXIS2_PLACEMENT_3D('',#107464,#39888,#39889);
#33806=AXIS2_PLACEMENT_3D('',#107468,#39892,#39893);
#33807=AXIS2_PLACEMENT_3D('',#107470,#39895,#39896);
#33808=AXIS2_PLACEMENT_3D('',#107471,#39897,#39898);
#33809=AXIS2_PLACEMENT_3D('',#107472,#39899,#39900);
#33810=AXIS2_PLACEMENT_3D('',#107473,#39901,#39902);
#33811=AXIS2_PLACEMENT_3D('',#107475,#39903,#39904);
#33812=AXIS2_PLACEMENT_3D('',#107476,#39905,#39906);
#33813=AXIS2_PLACEMENT_3D('',#107483,#39907,#39908);
#33814=AXIS2_PLACEMENT_3D('',#107493,#39909,#39910);
#33815=AXIS2_PLACEMENT_3D('',#107503,#39911,#39912);
#33816=AXIS2_PLACEMENT_3D('',#107513,#39913,#39914);
#33817=AXIS2_PLACEMENT_3D('',#107523,#39915,#39916);
#33818=AXIS2_PLACEMENT_3D('',#107533,#39917,#39918);
#33819=AXIS2_PLACEMENT_3D('',#107538,#39920,#39921);
#33820=AXIS2_PLACEMENT_3D('',#107543,#39924,#39925);
#33821=AXIS2_PLACEMENT_3D('',#107544,#39926,#39927);
#33822=AXIS2_PLACEMENT_3D('',#107548,#39929,#39930);
#33823=AXIS2_PLACEMENT_3D('',#107550,#39932,#39933);
#33824=AXIS2_PLACEMENT_3D('',#107555,#39936,#39937);
#33825=AXIS2_PLACEMENT_3D('',#107556,#39938,#39939);
#33826=AXIS2_PLACEMENT_3D('',#107560,#39941,#39942);
#33827=AXIS2_PLACEMENT_3D('',#107562,#39944,#39945);
#33828=AXIS2_PLACEMENT_3D('',#107567,#39948,#39949);
#33829=AXIS2_PLACEMENT_3D('',#107568,#39950,#39951);
#33830=AXIS2_PLACEMENT_3D('',#107572,#39953,#39954);
#33831=AXIS2_PLACEMENT_3D('',#107574,#39956,#39957);
#33832=AXIS2_PLACEMENT_3D('',#107581,#39962,#39963);
#33833=AXIS2_PLACEMENT_3D('',#107586,#39967,#39968);
#33834=AXIS2_PLACEMENT_3D('',#107591,#39972,#39973);
#33835=AXIS2_PLACEMENT_3D('',#107592,#39974,#39975);
#33836=AXIS2_PLACEMENT_3D('',#107593,#39976,#39977);
#33837=AXIS2_PLACEMENT_3D('',#107595,#39979,#39980);
#33838=AXIS2_PLACEMENT_3D('',#107596,#39981,#39982);
#33839=AXIS2_PLACEMENT_3D('',#107598,#39984,#39985);
#33840=AXIS2_PLACEMENT_3D('',#107600,#39987,#39988);
#33841=AXIS2_PLACEMENT_3D('',#107604,#39990,#39991);
#33842=AXIS2_PLACEMENT_3D('',#107605,#39992,#39993);
#33843=AXIS2_PLACEMENT_3D('',#107607,#39995,#39996);
#33844=AXIS2_PLACEMENT_3D('',#107608,#39997,#39998);
#33845=AXIS2_PLACEMENT_3D('',#107609,#39999,#40000);
#33846=AXIS2_PLACEMENT_3D('',#107610,#40001,#40002);
#33847=AXIS2_PLACEMENT_3D('',#107611,#40003,#40004);
#33848=AXIS2_PLACEMENT_3D('',#107612,#40005,#40006);
#33849=AXIS2_PLACEMENT_3D('',#107613,#40007,#40008);
#33850=AXIS2_PLACEMENT_3D('',#107614,#40009,#40010);
#33851=AXIS2_PLACEMENT_3D('',#107616,#40012,#40013);
#33852=AXIS2_PLACEMENT_3D('',#107617,#40014,#40015);
#33853=AXIS2_PLACEMENT_3D('',#107620,#40017,#40018);
#33854=AXIS2_PLACEMENT_3D('',#107623,#40021,#40022);
#33855=AXIS2_PLACEMENT_3D('',#107624,#40023,#40024);
#39162=DIRECTION('axis',(0.,0.,1.));
#39163=DIRECTION('refdir',(1.,0.,0.));
#39164=DIRECTION('center_axis',(0.,1.,0.));
#39165=DIRECTION('ref_axis',(1.,0.,0.));
#39166=DIRECTION('',(0.,-1.,0.));
#39167=DIRECTION('center_axis',(0.,-1.,0.));
#39168=DIRECTION('ref_axis',(1.,0.,0.));
#39169=DIRECTION('center_axis',(0.,1.,0.));
#39170=DIRECTION('ref_axis',(1.,0.,0.));
#39171=DIRECTION('',(0.,-1.,0.));
#39172=DIRECTION('center_axis',(0.,1.,0.));
#39173=DIRECTION('ref_axis',(1.,0.,0.));
#39174=DIRECTION('',(0.,-1.,0.));
#39175=DIRECTION('center_axis',(0.,1.,0.));
#39176=DIRECTION('ref_axis',(1.,0.,0.));
#39177=DIRECTION('',(0.,-1.,0.));
#39178=DIRECTION('center_axis',(0.,1.,0.));
#39179=DIRECTION('ref_axis',(1.,0.,0.));
#39180=DIRECTION('',(0.,-1.,0.));
#39181=DIRECTION('center_axis',(0.,1.,0.));
#39182=DIRECTION('ref_axis',(1.,0.,0.));
#39183=DIRECTION('',(0.,-1.,0.));
#39184=DIRECTION('center_axis',(0.,1.,0.));
#39185=DIRECTION('ref_axis',(1.,0.,0.));
#39186=DIRECTION('',(0.,-1.,0.));
#39187=DIRECTION('center_axis',(0.,1.,0.));
#39188=DIRECTION('ref_axis',(1.,0.,0.));
#39189=DIRECTION('',(0.,-1.,0.));
#39190=DIRECTION('center_axis',(0.,1.,0.));
#39191=DIRECTION('ref_axis',(1.,0.,0.));
#39192=DIRECTION('',(0.,-1.,0.));
#39193=DIRECTION('center_axis',(0.,1.,0.));
#39194=DIRECTION('ref_axis',(1.,0.,0.));
#39195=DIRECTION('',(0.,-1.,0.));
#39196=DIRECTION('center_axis',(0.,1.,0.));
#39197=DIRECTION('ref_axis',(1.,0.,0.));
#39198=DIRECTION('',(0.,-1.,0.));
#39199=DIRECTION('center_axis',(0.,1.,0.));
#39200=DIRECTION('ref_axis',(1.,0.,0.));
#39201=DIRECTION('',(0.,-1.,0.));
#39202=DIRECTION('center_axis',(0.,1.,0.));
#39203=DIRECTION('ref_axis',(1.,0.,0.));
#39204=DIRECTION('',(0.,-1.,0.));
#39205=DIRECTION('center_axis',(0.,1.,0.));
#39206=DIRECTION('ref_axis',(1.,0.,0.));
#39207=DIRECTION('',(0.,-1.,0.));
#39208=DIRECTION('center_axis',(0.,1.,0.));
#39209=DIRECTION('ref_axis',(1.,0.,0.));
#39210=DIRECTION('',(0.,-1.,0.));
#39211=DIRECTION('center_axis',(0.,1.,0.));
#39212=DIRECTION('ref_axis',(1.,0.,0.));
#39213=DIRECTION('',(0.,-1.,0.));
#39214=DIRECTION('center_axis',(0.,1.,0.));
#39215=DIRECTION('ref_axis',(1.,0.,0.));
#39216=DIRECTION('',(0.,-1.,0.));
#39217=DIRECTION('center_axis',(0.,1.,0.));
#39218=DIRECTION('ref_axis',(1.,0.,0.));
#39219=DIRECTION('',(0.,-1.,0.));
#39220=DIRECTION('center_axis',(0.,1.,0.));
#39221=DIRECTION('ref_axis',(1.,0.,0.));
#39222=DIRECTION('',(0.,-1.,0.));
#39223=DIRECTION('center_axis',(0.,1.,0.));
#39224=DIRECTION('ref_axis',(1.,0.,0.));
#39225=DIRECTION('',(0.,-1.,0.));
#39226=DIRECTION('center_axis',(0.,1.,0.));
#39227=DIRECTION('ref_axis',(1.,0.,0.));
#39228=DIRECTION('',(0.,-1.,0.));
#39229=DIRECTION('center_axis',(0.,1.,0.));
#39230=DIRECTION('ref_axis',(1.,0.,0.));
#39231=DIRECTION('',(0.,-1.,0.));
#39232=DIRECTION('center_axis',(0.,1.,0.));
#39233=DIRECTION('ref_axis',(1.,0.,0.));
#39234=DIRECTION('',(0.,-1.,0.));
#39235=DIRECTION('center_axis',(0.,1.,0.));
#39236=DIRECTION('ref_axis',(-0.160387124847653,0.,0.987054188068266));
#39237=DIRECTION('',(0.,-1.,0.));
#39238=DIRECTION('center_axis',(0.,-1.,0.));
#39239=DIRECTION('ref_axis',(1.,0.,-2.68659360660725E-14));
#39240=DIRECTION('center_axis',(0.,1.,0.));
#39241=DIRECTION('ref_axis',(-0.160387124847653,0.,0.987054188068266));
#39242=DIRECTION('',(0.,-1.,0.));
#39243=DIRECTION('center_axis',(0.,1.,0.));
#39244=DIRECTION('ref_axis',(-0.160387124847653,0.,0.987054188068266));
#39245=DIRECTION('',(0.,-1.,0.));
#39246=DIRECTION('center_axis',(0.,1.,0.));
#39247=DIRECTION('ref_axis',(-0.160387124847653,0.,0.987054188068266));
#39248=DIRECTION('',(0.,-1.,0.));
#39249=DIRECTION('center_axis',(0.,1.,0.));
#39250=DIRECTION('ref_axis',(-0.160387124847653,0.,0.987054188068266));
#39251=DIRECTION('',(0.,-1.,0.));
#39252=DIRECTION('center_axis',(0.,1.,0.));
#39253=DIRECTION('ref_axis',(-0.160387124847653,0.,0.987054188068266));
#39254=DIRECTION('',(0.,-1.,0.));
#39255=DIRECTION('center_axis',(0.,1.,0.));
#39256=DIRECTION('ref_axis',(-0.160387124847653,0.,0.987054188068266));
#39257=DIRECTION('',(0.,-1.,0.));
#39258=DIRECTION('center_axis',(0.,1.,0.));
#39259=DIRECTION('ref_axis',(-0.160387124847653,0.,0.987054188068266));
#39260=DIRECTION('',(0.,-1.,0.));
#39261=DIRECTION('center_axis',(0.,1.,0.));
#39262=DIRECTION('ref_axis',(-0.160387124847653,0.,0.987054188068266));
#39263=DIRECTION('',(0.,-1.,0.));
#39264=DIRECTION('center_axis',(0.,1.,0.));
#39265=DIRECTION('ref_axis',(-0.160387124847653,0.,0.987054188068266));
#39266=DIRECTION('',(0.,-1.,0.));
#39267=DIRECTION('center_axis',(0.,1.,0.));
#39268=DIRECTION('ref_axis',(-0.160387124847653,0.,0.987054188068266));
#39269=DIRECTION('',(0.,-1.,0.));
#39270=DIRECTION('center_axis',(0.,1.,0.));
#39271=DIRECTION('ref_axis',(-0.160387124847653,0.,0.987054188068266));
#39272=DIRECTION('',(0.,-1.,0.));
#39273=DIRECTION('center_axis',(0.,1.,0.));
#39274=DIRECTION('ref_axis',(-0.160387124847653,0.,0.987054188068266));
#39275=DIRECTION('',(0.,-1.,0.));
#39276=DIRECTION('center_axis',(0.,1.,0.));
#39277=DIRECTION('ref_axis',(-0.160387124847653,0.,0.987054188068266));
#39278=DIRECTION('',(0.,-1.,0.));
#39279=DIRECTION('center_axis',(0.,1.,0.));
#39280=DIRECTION('ref_axis',(-0.160387124847653,0.,0.987054188068266));
#39281=DIRECTION('',(0.,-1.,0.));
#39282=DIRECTION('center_axis',(0.,1.,0.));
#39283=DIRECTION('ref_axis',(-0.160387124847653,0.,0.987054188068266));
#39284=DIRECTION('',(0.,-1.,0.));
#39285=DIRECTION('center_axis',(0.,1.,0.));
#39286=DIRECTION('ref_axis',(-0.160387124847653,0.,0.987054188068266));
#39287=DIRECTION('',(0.,-1.,0.));
#39288=DIRECTION('center_axis',(0.,1.,0.));
#39289=DIRECTION('ref_axis',(-0.160387124847653,0.,0.987054188068266));
#39290=DIRECTION('',(0.,-1.,0.));
#39291=DIRECTION('center_axis',(0.,1.,0.));
#39292=DIRECTION('ref_axis',(-0.160387124847653,0.,0.987054188068266));
#39293=DIRECTION('',(0.,-1.,0.));
#39294=DIRECTION('center_axis',(0.,1.,0.));
#39295=DIRECTION('ref_axis',(-0.160387124847653,0.,0.987054188068266));
#39296=DIRECTION('',(0.,-1.,0.));
#39297=DIRECTION('center_axis',(0.,1.,0.));
#39298=DIRECTION('ref_axis',(-0.160387124847653,0.,0.987054188068266));
#39299=DIRECTION('',(0.,-1.,0.));
#39300=DIRECTION('center_axis',(0.,1.,0.));
#39301=DIRECTION('ref_axis',(-0.160387124847653,0.,0.987054188068266));
#39302=DIRECTION('',(0.,-1.,0.));
#39303=DIRECTION('center_axis',(0.,1.,0.));
#39304=DIRECTION('ref_axis',(-0.160387124847653,0.,0.987054188068266));
#39305=DIRECTION('',(0.,-1.,0.));
#39306=DIRECTION('center_axis',(0.,1.,0.));
#39307=DIRECTION('ref_axis',(-0.160387124847653,0.,0.987054188068266));
#39308=DIRECTION('center_axis',(0.,1.,0.));
#39309=DIRECTION('ref_axis',(1.,0.,-2.68659360660725E-14));
#39310=DIRECTION('center_axis',(0.,1.,0.));
#39311=DIRECTION('ref_axis',(1.,0.,0.));
#39312=DIRECTION('center_axis',(0.,1.,0.));
#39313=DIRECTION('ref_axis',(1.,0.,0.));
#39314=DIRECTION('center_axis',(0.,1.,0.));
#39315=DIRECTION('ref_axis',(0.,0.,1.));
#39316=DIRECTION('center_axis',(0.,1.,0.));
#39317=DIRECTION('ref_axis',(1.,0.,0.));
#39318=DIRECTION('center_axis',(0.,1.,0.));
#39319=DIRECTION('ref_axis',(1.,0.,0.));
#39320=DIRECTION('center_axis',(0.,1.,0.));
#39321=DIRECTION('ref_axis',(0.,0.,1.));
#39322=DIRECTION('center_axis',(0.,-1.,0.));
#39323=DIRECTION('ref_axis',(1.,0.,0.));
#39324=DIRECTION('center_axis',(0.,-1.,0.));
#39325=DIRECTION('ref_axis',(1.,0.,0.));
#39326=DIRECTION('center_axis',(0.,-1.,0.));
#39327=DIRECTION('ref_axis',(0.,0.,-1.));
#39328=DIRECTION('center_axis',(0.,1.,0.));
#39329=DIRECTION('ref_axis',(1.,0.,0.));
#39330=DIRECTION('center_axis',(1.,0.,0.));
#39331=DIRECTION('ref_axis',(0.,0.,1.));
#39332=DIRECTION('center_axis',(0.,1.,0.));
#39333=DIRECTION('ref_axis',(1.,0.,0.));
#39334=DIRECTION('center_axis',(0.,-1.,0.));
#39335=DIRECTION('ref_axis',(1.,0.,0.));
#39336=DIRECTION('center_axis',(0.,-1.,0.));
#39337=DIRECTION('ref_axis',(1.,0.,0.));
#39338=DIRECTION('',(0.707106781186547,0.707106781186549,8.65956056235492E-17));
#39339=DIRECTION('center_axis',(0.,-1.,0.));
#39340=DIRECTION('ref_axis',(1.,0.,0.));
#39341=DIRECTION('center_axis',(0.,1.,0.));
#39342=DIRECTION('ref_axis',(1.,0.,0.));
#39343=DIRECTION('center_axis',(0.,1.,0.));
#39344=DIRECTION('ref_axis',(-0.17364817766693,0.,0.984807753012208));
#39345=DIRECTION('center_axis',(0.,1.,0.));
#39346=DIRECTION('ref_axis',(1.,0.,0.));
#39347=DIRECTION('',(0.869726513699833,0.,0.49353398197848));
#39348=DIRECTION('',(-0.986074150277955,0.,0.166306254102512));
#39349=DIRECTION('center_axis',(-0.166306254102512,0.,-0.986074150277955));
#39350=DIRECTION('ref_axis',(-0.986074150277955,0.,0.166306254102512));
#39351=DIRECTION('',(0.,-1.,0.));
#39352=DIRECTION('',(0.,1.,0.));
#39353=DIRECTION('center_axis',(-0.49353398197848,0.,0.869726513699833));
#39354=DIRECTION('ref_axis',(0.869726513699833,0.,0.49353398197848));
#39355=DIRECTION('',(0.,1.,0.));
#39356=DIRECTION('center_axis',(0.,-1.,0.));
#39357=DIRECTION('ref_axis',(1.,0.,0.));
#39358=DIRECTION('center_axis',(0.,1.,0.));
#39359=DIRECTION('ref_axis',(1.,0.,0.));
#39360=DIRECTION('',(0.,1.,0.));
#39361=DIRECTION('center_axis',(0.,1.,0.));
#39362=DIRECTION('ref_axis',(1.,0.,0.));
#39363=DIRECTION('center_axis',(0.,1.,0.));
#39364=DIRECTION('ref_axis',(1.,0.,0.));
#39365=DIRECTION('center_axis',(0.,1.,0.));
#39366=DIRECTION('ref_axis',(1.,0.,0.));
#39367=DIRECTION('',(0.,-1.,0.));
#39368=DIRECTION('center_axis',(0.,-1.,0.));
#39369=DIRECTION('ref_axis',(1.,0.,0.));
#39370=DIRECTION('',(0.,1.,0.));
#39371=DIRECTION('center_axis',(0.,1.,0.));
#39372=DIRECTION('ref_axis',(1.,0.,0.));
#39373=DIRECTION('',(0.,-1.,0.));
#39374=DIRECTION('center_axis',(0.,-1.,0.));
#39375=DIRECTION('ref_axis',(1.,0.,0.));
#39376=DIRECTION('',(0.,1.,0.));
#39377=DIRECTION('center_axis',(0.,1.,0.));
#39378=DIRECTION('ref_axis',(1.,0.,0.));
#39379=DIRECTION('',(0.,-1.,0.));
#39380=DIRECTION('center_axis',(0.,-1.,0.));
#39381=DIRECTION('ref_axis',(1.,0.,0.));
#39382=DIRECTION('',(0.,1.,0.));
#39383=DIRECTION('center_axis',(0.,1.,0.));
#39384=DIRECTION('ref_axis',(1.,0.,0.));
#39385=DIRECTION('',(0.,-1.,0.));
#39386=DIRECTION('center_axis',(0.,-1.,0.));
#39387=DIRECTION('ref_axis',(1.,0.,0.));
#39388=DIRECTION('',(0.,1.,0.));
#39389=DIRECTION('center_axis',(0.,1.,0.));
#39390=DIRECTION('ref_axis',(1.,0.,0.));
#39391=DIRECTION('',(0.,-1.,0.));
#39392=DIRECTION('center_axis',(0.,-1.,0.));
#39393=DIRECTION('ref_axis',(1.,0.,0.));
#39394=DIRECTION('',(0.,1.,0.));
#39395=DIRECTION('center_axis',(0.,1.,0.));
#39396=DIRECTION('ref_axis',(1.,0.,0.));
#39397=DIRECTION('',(0.,-1.,0.));
#39398=DIRECTION('center_axis',(0.,-1.,0.));
#39399=DIRECTION('ref_axis',(1.,0.,0.));
#39400=DIRECTION('',(0.,1.,0.));
#39401=DIRECTION('center_axis',(0.,1.,0.));
#39402=DIRECTION('ref_axis',(1.,0.,0.));
#39403=DIRECTION('',(0.,-1.,0.));
#39404=DIRECTION('center_axis',(0.,-1.,0.));
#39405=DIRECTION('ref_axis',(1.,0.,0.));
#39406=DIRECTION('',(0.,1.,0.));
#39407=DIRECTION('center_axis',(0.,1.,0.));
#39408=DIRECTION('ref_axis',(1.,0.,0.));
#39409=DIRECTION('',(0.,-1.,0.));
#39410=DIRECTION('center_axis',(0.,-1.,0.));
#39411=DIRECTION('ref_axis',(1.,0.,0.));
#39412=DIRECTION('',(0.,1.,0.));
#39413=DIRECTION('center_axis',(0.,1.,0.));
#39414=DIRECTION('ref_axis',(1.,0.,0.));
#39415=DIRECTION('',(0.,-1.,0.));
#39416=DIRECTION('center_axis',(0.,-1.,0.));
#39417=DIRECTION('ref_axis',(1.,0.,0.));
#39418=DIRECTION('',(0.,1.,0.));
#39419=DIRECTION('center_axis',(0.,1.,0.));
#39420=DIRECTION('ref_axis',(1.,0.,0.));
#39421=DIRECTION('',(0.,-1.,0.));
#39422=DIRECTION('center_axis',(0.,-1.,0.));
#39423=DIRECTION('ref_axis',(1.,0.,0.));
#39424=DIRECTION('',(0.,1.,0.));
#39425=DIRECTION('center_axis',(0.,1.,0.));
#39426=DIRECTION('ref_axis',(1.,0.,0.));
#39427=DIRECTION('',(0.,-1.,0.));
#39428=DIRECTION('center_axis',(0.,-1.,0.));
#39429=DIRECTION('ref_axis',(1.,0.,0.));
#39430=DIRECTION('',(0.,1.,0.));
#39431=DIRECTION('center_axis',(0.,1.,0.));
#39432=DIRECTION('ref_axis',(1.,0.,0.));
#39433=DIRECTION('',(0.,-1.,0.));
#39434=DIRECTION('center_axis',(0.,-1.,0.));
#39435=DIRECTION('ref_axis',(1.,0.,0.));
#39436=DIRECTION('',(0.,1.,0.));
#39437=DIRECTION('center_axis',(0.,1.,0.));
#39438=DIRECTION('ref_axis',(1.,0.,0.));
#39439=DIRECTION('',(0.,-1.,0.));
#39440=DIRECTION('center_axis',(0.,-1.,0.));
#39441=DIRECTION('ref_axis',(1.,0.,0.));
#39442=DIRECTION('',(0.,1.,0.));
#39443=DIRECTION('center_axis',(0.,1.,0.));
#39444=DIRECTION('ref_axis',(1.,0.,0.));
#39445=DIRECTION('',(0.,-1.,0.));
#39446=DIRECTION('center_axis',(0.,-1.,0.));
#39447=DIRECTION('ref_axis',(1.,0.,0.));
#39448=DIRECTION('',(0.,1.,0.));
#39449=DIRECTION('center_axis',(0.,1.,0.));
#39450=DIRECTION('ref_axis',(1.,0.,0.));
#39451=DIRECTION('',(0.,-1.,0.));
#39452=DIRECTION('center_axis',(0.,-1.,0.));
#39453=DIRECTION('ref_axis',(1.,0.,0.));
#39454=DIRECTION('',(0.,1.,0.));
#39455=DIRECTION('center_axis',(0.,1.,0.));
#39456=DIRECTION('ref_axis',(1.,0.,0.));
#39457=DIRECTION('',(0.,-1.,0.));
#39458=DIRECTION('center_axis',(0.,-1.,0.));
#39459=DIRECTION('ref_axis',(1.,0.,0.));
#39460=DIRECTION('',(0.,1.,0.));
#39461=DIRECTION('center_axis',(0.,1.,0.));
#39462=DIRECTION('ref_axis',(1.,0.,0.));
#39463=DIRECTION('',(0.,-1.,0.));
#39464=DIRECTION('center_axis',(0.,-1.,0.));
#39465=DIRECTION('ref_axis',(1.,0.,0.));
#39466=DIRECTION('center_axis',(0.,-1.,0.));
#39467=DIRECTION('ref_axis',(1.,0.,0.));
#39468=DIRECTION('',(0.,1.,0.));
#39469=DIRECTION('center_axis',(0.,1.,0.));
#39470=DIRECTION('ref_axis',(1.,0.,0.));
#39471=DIRECTION('',(0.,-1.,0.));
#39472=DIRECTION('center_axis',(0.,-1.,0.));
#39473=DIRECTION('ref_axis',(1.,0.,0.));
#39474=DIRECTION('',(0.,1.,0.));
#39475=DIRECTION('center_axis',(0.,1.,0.));
#39476=DIRECTION('ref_axis',(1.,0.,0.));
#39477=DIRECTION('',(0.,-1.,0.));
#39478=DIRECTION('center_axis',(0.,-1.,0.));
#39479=DIRECTION('ref_axis',(1.,0.,0.));
#39480=DIRECTION('',(0.,1.,0.));
#39481=DIRECTION('center_axis',(0.,1.,0.));
#39482=DIRECTION('ref_axis',(1.,0.,0.));
#39483=DIRECTION('',(0.,-1.,0.));
#39484=DIRECTION('center_axis',(0.,-1.,0.));
#39485=DIRECTION('ref_axis',(1.,0.,0.));
#39486=DIRECTION('',(0.,1.,0.));
#39487=DIRECTION('center_axis',(0.,1.,0.));
#39488=DIRECTION('ref_axis',(1.,0.,0.));
#39489=DIRECTION('',(0.,-1.,0.));
#39490=DIRECTION('center_axis',(0.,-1.,0.));
#39491=DIRECTION('ref_axis',(1.,0.,0.));
#39492=DIRECTION('',(0.,1.,0.));
#39493=DIRECTION('center_axis',(0.,1.,0.));
#39494=DIRECTION('ref_axis',(1.,0.,0.));
#39495=DIRECTION('',(0.,-1.,0.));
#39496=DIRECTION('center_axis',(0.,-1.,0.));
#39497=DIRECTION('ref_axis',(1.,0.,0.));
#39498=DIRECTION('',(0.,1.,0.));
#39499=DIRECTION('center_axis',(0.,1.,0.));
#39500=DIRECTION('ref_axis',(1.,0.,0.));
#39501=DIRECTION('',(0.,-1.,0.));
#39502=DIRECTION('center_axis',(0.,-1.,0.));
#39503=DIRECTION('ref_axis',(1.,0.,0.));
#39504=DIRECTION('',(0.,1.,0.));
#39505=DIRECTION('center_axis',(0.,1.,0.));
#39506=DIRECTION('ref_axis',(1.,0.,0.));
#39507=DIRECTION('',(0.,-1.,0.));
#39508=DIRECTION('center_axis',(0.,-1.,0.));
#39509=DIRECTION('ref_axis',(1.,0.,0.));
#39510=DIRECTION('',(0.,1.,0.));
#39511=DIRECTION('center_axis',(0.,1.,0.));
#39512=DIRECTION('ref_axis',(1.,0.,0.));
#39513=DIRECTION('',(0.,-1.,0.));
#39514=DIRECTION('center_axis',(0.,-1.,0.));
#39515=DIRECTION('ref_axis',(1.,0.,0.));
#39516=DIRECTION('',(0.,1.,0.));
#39517=DIRECTION('center_axis',(0.,1.,0.));
#39518=DIRECTION('ref_axis',(1.,0.,0.));
#39519=DIRECTION('',(0.,-1.,0.));
#39520=DIRECTION('center_axis',(0.,-1.,0.));
#39521=DIRECTION('ref_axis',(1.,0.,0.));
#39522=DIRECTION('',(0.,1.,0.));
#39523=DIRECTION('center_axis',(0.,1.,0.));
#39524=DIRECTION('ref_axis',(1.,0.,0.));
#39525=DIRECTION('',(0.,-1.,0.));
#39526=DIRECTION('center_axis',(0.,-1.,0.));
#39527=DIRECTION('ref_axis',(1.,0.,0.));
#39528=DIRECTION('',(0.,1.,0.));
#39529=DIRECTION('center_axis',(0.,1.,0.));
#39530=DIRECTION('ref_axis',(1.,0.,0.));
#39531=DIRECTION('',(0.,-1.,0.));
#39532=DIRECTION('center_axis',(0.,-1.,0.));
#39533=DIRECTION('ref_axis',(1.,0.,0.));
#39534=DIRECTION('',(0.,1.,0.));
#39535=DIRECTION('center_axis',(0.,1.,0.));
#39536=DIRECTION('ref_axis',(1.,0.,0.));
#39537=DIRECTION('',(0.,-1.,0.));
#39538=DIRECTION('center_axis',(0.,-1.,0.));
#39539=DIRECTION('ref_axis',(1.,0.,0.));
#39540=DIRECTION('',(0.,1.,0.));
#39541=DIRECTION('center_axis',(0.,1.,0.));
#39542=DIRECTION('ref_axis',(1.,0.,0.));
#39543=DIRECTION('',(0.,-1.,0.));
#39544=DIRECTION('center_axis',(0.,-1.,0.));
#39545=DIRECTION('ref_axis',(1.,0.,0.));
#39546=DIRECTION('',(0.,1.,0.));
#39547=DIRECTION('center_axis',(0.,1.,0.));
#39548=DIRECTION('ref_axis',(1.,0.,0.));
#39549=DIRECTION('',(0.,-1.,0.));
#39550=DIRECTION('center_axis',(0.,-1.,0.));
#39551=DIRECTION('ref_axis',(1.,0.,0.));
#39552=DIRECTION('',(0.,1.,0.));
#39553=DIRECTION('center_axis',(0.,1.,0.));
#39554=DIRECTION('ref_axis',(1.,0.,0.));
#39555=DIRECTION('',(0.,-1.,0.));
#39556=DIRECTION('center_axis',(0.,-1.,0.));
#39557=DIRECTION('ref_axis',(1.,0.,0.));
#39558=DIRECTION('',(0.,1.,0.));
#39559=DIRECTION('center_axis',(0.,1.,0.));
#39560=DIRECTION('ref_axis',(1.,0.,0.));
#39561=DIRECTION('',(0.,-1.,0.));
#39562=DIRECTION('center_axis',(0.,-1.,0.));
#39563=DIRECTION('ref_axis',(1.,0.,0.));
#39564=DIRECTION('',(0.,1.,0.));
#39565=DIRECTION('center_axis',(0.,1.,0.));
#39566=DIRECTION('ref_axis',(1.,0.,0.));
#39567=DIRECTION('',(0.,-1.,0.));
#39568=DIRECTION('center_axis',(0.,-1.,0.));
#39569=DIRECTION('ref_axis',(1.,0.,0.));
#39570=DIRECTION('',(0.,1.,0.));
#39571=DIRECTION('center_axis',(0.,1.,0.));
#39572=DIRECTION('ref_axis',(1.,0.,0.));
#39573=DIRECTION('',(0.,-1.,0.));
#39574=DIRECTION('center_axis',(0.,-1.,0.));
#39575=DIRECTION('ref_axis',(1.,0.,0.));
#39576=DIRECTION('',(0.,1.,0.));
#39577=DIRECTION('center_axis',(0.0074502908256619,0.,-0.99997224619817));
#39578=DIRECTION('ref_axis',(-0.99997224619817,0.,-0.0074502908256619));
#39579=DIRECTION('',(-0.99997224619817,0.,-0.0074502908256619));
#39580=DIRECTION('',(0.,1.,0.));
#39581=DIRECTION('center_axis',(-0.637062515999984,0.,0.770812137104606));
#39582=DIRECTION('ref_axis',(0.770812137104606,0.,0.637062515999984));
#39583=DIRECTION('',(0.770812137104606,0.,0.637062515999984));
#39584=DIRECTION('center_axis',(0.,1.,0.));
#39585=DIRECTION('ref_axis',(-0.342020143325669,0.,0.939692620785908));
#39586=DIRECTION('center_axis',(0.,1.,0.));
#39587=DIRECTION('ref_axis',(1.,0.,0.));
#39588=DIRECTION('',(0.707106781186547,-0.707106781186548,-8.65956056235493E-17));
#39589=DIRECTION('center_axis',(0.,1.,0.));
#39590=DIRECTION('ref_axis',(1.,0.,0.));
#39591=DIRECTION('center_axis',(0.,1.,0.));
#39592=DIRECTION('ref_axis',(-0.5,0.,0.866025403784438));
#39593=DIRECTION('',(0.648477023773219,0.,0.761234227842015));
#39594=DIRECTION('',(-0.983486691428025,0.,-0.180980462437127));
#39595=DIRECTION('center_axis',(0.180980462437127,0.,-0.983486691428025));
#39596=DIRECTION('ref_axis',(-0.983486691428025,0.,-0.180980462437127));
#39597=DIRECTION('',(0.,1.,0.));
#39598=DIRECTION('center_axis',(-0.761234227842015,0.,0.648477023773219));
#39599=DIRECTION('ref_axis',(0.648477023773219,0.,0.761234227842015));
#39600=DIRECTION('center_axis',(0.349011634277972,0.,-0.937118391207119));
#39601=DIRECTION('ref_axis',(-0.937118391207119,0.,-0.349011634277972));
#39602=DIRECTION('',(-0.937118391207119,0.,-0.349011634277972));
#39603=DIRECTION('',(0.,1.,0.));
#39604=DIRECTION('center_axis',(-0.862276222874172,0.,0.506438264219689));
#39605=DIRECTION('ref_axis',(0.506438264219689,0.,0.862276222874172));
#39606=DIRECTION('',(0.506438264219689,0.,0.862276222874172));
#39607=DIRECTION('center_axis',(0.,1.,0.));
#39608=DIRECTION('ref_axis',(-0.64278760968654,0.,0.766044443118978));
#39609=DIRECTION('center_axis',(0.,1.,0.));
#39610=DIRECTION('ref_axis',(-0.766044443118978,0.,0.642787609686539));
#39611=DIRECTION('',(0.349011634277972,0.,0.937118391207119));
#39612=DIRECTION('',(-0.862276222874171,0.,-0.50643826421969));
#39613=DIRECTION('center_axis',(0.50643826421969,0.,-0.862276222874171));
#39614=DIRECTION('ref_axis',(-0.862276222874171,0.,-0.50643826421969));
#39615=DIRECTION('',(0.,1.,0.));
#39616=DIRECTION('center_axis',(-0.937118391207119,0.,0.349011634277972));
#39617=DIRECTION('ref_axis',(0.349011634277972,0.,0.937118391207119));
#39618=DIRECTION('center_axis',(0.648477023773219,0.,-0.761234227842014));
#39619=DIRECTION('ref_axis',(-0.761234227842014,0.,-0.648477023773219));
#39620=DIRECTION('',(-0.761234227842014,0.,-0.648477023773219));
#39621=DIRECTION('',(0.,1.,0.));
#39622=DIRECTION('center_axis',(-0.983486691428025,0.,0.180980462437126));
#39623=DIRECTION('ref_axis',(0.180980462437126,0.,0.983486691428025));
#39624=DIRECTION('',(0.180980462437126,0.,0.983486691428025));
#39625=DIRECTION('center_axis',(0.,1.,0.));
#39626=DIRECTION('ref_axis',(-0.866025403784439,0.,0.5));
#39627=DIRECTION('center_axis',(0.,1.,0.));
#39628=DIRECTION('ref_axis',(-0.939692620785909,0.,0.342020143325668));
#39629=DIRECTION('',(0.00745029082566051,0.,0.99997224619817));
#39630=DIRECTION('',(-0.637062515999983,0.,-0.770812137104607));
#39631=DIRECTION('center_axis',(0.770812137104607,0.,-0.637062515999983));
#39632=DIRECTION('ref_axis',(-0.637062515999983,0.,-0.770812137104607));
#39633=DIRECTION('',(0.,1.,0.));
#39634=DIRECTION('center_axis',(-0.99997224619817,0.,0.00745029082566051));
#39635=DIRECTION('ref_axis',(0.00745029082566051,0.,0.99997224619817));
#39636=DIRECTION('center_axis',(0.869726513699833,0.,-0.49353398197848));
#39637=DIRECTION('ref_axis',(-0.49353398197848,0.,-0.869726513699833));
#39638=DIRECTION('',(-0.49353398197848,0.,-0.869726513699833));
#39639=DIRECTION('',(0.,1.,0.));
#39640=DIRECTION('center_axis',(-0.986074150277955,0.,-0.166306254102513));
#39641=DIRECTION('ref_axis',(-0.166306254102513,0.,0.986074150277955));
#39642=DIRECTION('',(-0.166306254102513,0.,0.986074150277955));
#39643=DIRECTION('center_axis',(0.,1.,0.));
#39644=DIRECTION('ref_axis',(-0.984807753012208,0.,0.17364817766693));
#39645=DIRECTION('center_axis',(0.,1.,0.));
#39646=DIRECTION('ref_axis',(-1.,0.,-1.83697019872103E-16));
#39647=DIRECTION('',(-0.335009667654806,0.,0.94221469027914));
#39648=DIRECTION('',(-0.335009667654806,0.,-0.94221469027914));
#39649=DIRECTION('center_axis',(0.94221469027914,0.,-0.335009667654806));
#39650=DIRECTION('ref_axis',(-0.335009667654806,0.,-0.94221469027914));
#39651=DIRECTION('',(0.,1.,0.));
#39652=DIRECTION('center_axis',(-0.94221469027914,0.,-0.335009667654806));
#39653=DIRECTION('ref_axis',(-0.335009667654806,0.,0.94221469027914));
#39654=DIRECTION('center_axis',(0.986074150277955,0.,-0.166306254102512));
#39655=DIRECTION('ref_axis',(-0.166306254102512,0.,-0.986074150277955));
#39656=DIRECTION('',(-0.166306254102512,0.,-0.986074150277955));
#39657=DIRECTION('',(0.,1.,0.));
#39658=DIRECTION('center_axis',(-0.869726513699833,0.,-0.49353398197848));
#39659=DIRECTION('ref_axis',(-0.49353398197848,0.,0.869726513699833));
#39660=DIRECTION('',(-0.49353398197848,0.,0.869726513699833));
#39661=DIRECTION('center_axis',(0.,1.,0.));
#39662=DIRECTION('ref_axis',(-0.984807753012208,0.,-0.17364817766693));
#39663=DIRECTION('center_axis',(0.,1.,0.));
#39664=DIRECTION('ref_axis',(-0.939692620785908,0.,-0.342020143325669));
#39665=DIRECTION('',(-0.637062515999984,0.,0.770812137104606));
#39666=DIRECTION('',(0.00745029082566179,0.,-0.99997224619817));
#39667=DIRECTION('center_axis',(0.99997224619817,0.,0.00745029082566179));
#39668=DIRECTION('ref_axis',(0.00745029082566179,0.,-0.99997224619817));
#39669=DIRECTION('',(0.,1.,0.));
#39670=DIRECTION('center_axis',(-0.770812137104606,0.,-0.637062515999984));
#39671=DIRECTION('ref_axis',(-0.637062515999984,0.,0.770812137104606));
#39672=DIRECTION('center_axis',(0.983486691428025,0.,0.180980462437127));
#39673=DIRECTION('ref_axis',(0.180980462437127,0.,-0.983486691428025));
#39674=DIRECTION('',(0.180980462437127,0.,-0.983486691428025));
#39675=DIRECTION('',(0.,1.,0.));
#39676=DIRECTION('center_axis',(-0.648477023773219,0.,-0.761234227842015));
#39677=DIRECTION('ref_axis',(-0.761234227842015,0.,0.648477023773219));
#39678=DIRECTION('',(-0.761234227842015,0.,0.648477023773219));
#39679=DIRECTION('center_axis',(0.,1.,0.));
#39680=DIRECTION('ref_axis',(-0.866025403784438,0.,-0.5));
#39681=DIRECTION('center_axis',(0.,1.,0.));
#39682=DIRECTION('ref_axis',(-0.766044443118978,0.,-0.642787609686539));
#39683=DIRECTION('',(-0.862276222874172,0.,0.506438264219689));
#39684=DIRECTION('',(0.349011634277972,0.,-0.937118391207119));
#39685=DIRECTION('center_axis',(0.937118391207119,0.,0.349011634277972));
#39686=DIRECTION('ref_axis',(0.349011634277972,0.,-0.937118391207119));
#39687=DIRECTION('',(0.,1.,0.));
#39688=DIRECTION('center_axis',(-0.506438264219689,0.,-0.862276222874172));
#39689=DIRECTION('ref_axis',(-0.862276222874172,0.,0.506438264219689));
#39690=DIRECTION('center_axis',(0.862276222874171,0.,0.50643826421969));
#39691=DIRECTION('ref_axis',(0.50643826421969,0.,-0.862276222874171));
#39692=DIRECTION('',(0.50643826421969,0.,-0.862276222874171));
#39693=DIRECTION('',(0.,1.,0.));
#39694=DIRECTION('center_axis',(-0.349011634277972,0.,-0.937118391207119));
#39695=DIRECTION('ref_axis',(-0.937118391207119,0.,0.349011634277972));
#39696=DIRECTION('',(-0.937118391207119,0.,0.349011634277972));
#39697=DIRECTION('center_axis',(0.,1.,0.));
#39698=DIRECTION('ref_axis',(-0.642787609686539,0.,-0.766044443118978));
#39699=DIRECTION('center_axis',(0.,1.,0.));
#39700=DIRECTION('ref_axis',(-0.5,0.,-0.866025403784439));
#39701=DIRECTION('',(-0.983486691428025,0.,0.180980462437126));
#39702=DIRECTION('',(0.648477023773219,0.,-0.761234227842014));
#39703=DIRECTION('center_axis',(0.761234227842014,0.,0.648477023773219));
#39704=DIRECTION('ref_axis',(0.648477023773219,0.,-0.761234227842014));
#39705=DIRECTION('',(0.,1.,0.));
#39706=DIRECTION('center_axis',(-0.180980462437126,0.,-0.983486691428025));
#39707=DIRECTION('ref_axis',(-0.983486691428025,0.,0.180980462437126));
#39708=DIRECTION('center_axis',(0.637062515999983,0.,0.770812137104607));
#39709=DIRECTION('ref_axis',(0.770812137104607,0.,-0.637062515999983));
#39710=DIRECTION('',(0.770812137104607,0.,-0.637062515999983));
#39711=DIRECTION('',(0.,1.,0.));
#39712=DIRECTION('center_axis',(-0.00745029082566107,0.,-0.99997224619817));
#39713=DIRECTION('ref_axis',(-0.99997224619817,0.,0.00745029082566107));
#39714=DIRECTION('',(-0.99997224619817,0.,0.00745029082566107));
#39715=DIRECTION('center_axis',(0.,1.,0.));
#39716=DIRECTION('ref_axis',(-0.342020143325669,0.,-0.939692620785908));
#39717=DIRECTION('center_axis',(0.,1.,0.));
#39718=DIRECTION('ref_axis',(-0.17364817766693,0.,-0.984807753012208));
#39719=DIRECTION('',(-0.986074150277955,0.,-0.166306254102513));
#39720=DIRECTION('',(0.869726513699833,0.,-0.49353398197848));
#39721=DIRECTION('center_axis',(0.49353398197848,0.,0.869726513699833));
#39722=DIRECTION('ref_axis',(0.869726513699833,0.,-0.49353398197848));
#39723=DIRECTION('',(0.,1.,0.));
#39724=DIRECTION('center_axis',(0.166306254102513,0.,-0.986074150277955));
#39725=DIRECTION('ref_axis',(-0.986074150277955,0.,-0.166306254102513));
#39726=DIRECTION('center_axis',(0.335009667654806,0.,0.94221469027914));
#39727=DIRECTION('ref_axis',(0.94221469027914,0.,-0.335009667654806));
#39728=DIRECTION('',(0.94221469027914,0.,-0.335009667654806));
#39729=DIRECTION('',(0.,1.,0.));
#39730=DIRECTION('center_axis',(0.335009667654806,0.,-0.94221469027914));
#39731=DIRECTION('ref_axis',(-0.94221469027914,0.,-0.335009667654806));
#39732=DIRECTION('',(-0.94221469027914,0.,-0.335009667654806));
#39733=DIRECTION('center_axis',(0.,1.,0.));
#39734=DIRECTION('ref_axis',(1.22464679914735E-16,0.,-1.));
#39735=DIRECTION('center_axis',(0.,1.,0.));
#39736=DIRECTION('ref_axis',(0.173648177666931,0.,-0.984807753012208));
#39737=DIRECTION('',(-0.869726513699832,0.,-0.493533981978481));
#39738=DIRECTION('',(0.986074150277955,0.,-0.166306254102512));
#39739=DIRECTION('center_axis',(0.166306254102512,0.,0.986074150277955));
#39740=DIRECTION('ref_axis',(0.986074150277955,0.,-0.166306254102512));
#39741=DIRECTION('',(0.,1.,0.));
#39742=DIRECTION('center_axis',(0.493533981978481,0.,-0.869726513699832));
#39743=DIRECTION('ref_axis',(-0.869726513699832,0.,-0.493533981978481));
#39744=DIRECTION('center_axis',(-0.00745029082566129,0.,0.99997224619817));
#39745=DIRECTION('ref_axis',(0.99997224619817,0.,0.00745029082566129));
#39746=DIRECTION('',(0.99997224619817,0.,0.00745029082566129));
#39747=DIRECTION('',(0.,1.,0.));
#39748=DIRECTION('center_axis',(0.637062515999983,0.,-0.770812137104607));
#39749=DIRECTION('ref_axis',(-0.770812137104607,0.,-0.637062515999983));
#39750=DIRECTION('',(-0.770812137104607,0.,-0.637062515999983));
#39751=DIRECTION('center_axis',(0.,1.,0.));
#39752=DIRECTION('ref_axis',(0.342020143325669,0.,-0.939692620785908));
#39753=DIRECTION('center_axis',(0.,1.,0.));
#39754=DIRECTION('ref_axis',(0.5,0.,-0.866025403784439));
#39755=DIRECTION('',(-0.648477023773219,0.,-0.761234227842014));
#39756=DIRECTION('',(0.983486691428025,0.,0.180980462437126));
#39757=DIRECTION('center_axis',(-0.180980462437126,0.,0.983486691428025));
#39758=DIRECTION('ref_axis',(0.983486691428025,0.,0.180980462437126));
#39759=DIRECTION('',(0.,1.,0.));
#39760=DIRECTION('center_axis',(0.761234227842014,0.,-0.648477023773219));
#39761=DIRECTION('ref_axis',(-0.648477023773219,0.,-0.761234227842014));
#39762=DIRECTION('center_axis',(-0.349011634277972,0.,0.937118391207119));
#39763=DIRECTION('ref_axis',(0.937118391207119,0.,0.349011634277972));
#39764=DIRECTION('',(0.937118391207119,0.,0.349011634277972));
#39765=DIRECTION('',(0.,1.,0.));
#39766=DIRECTION('center_axis',(0.862276222874172,0.,-0.506438264219689));
#39767=DIRECTION('ref_axis',(-0.506438264219689,0.,-0.862276222874172));
#39768=DIRECTION('',(-0.506438264219689,0.,-0.862276222874172));
#39769=DIRECTION('center_axis',(0.,1.,0.));
#39770=DIRECTION('ref_axis',(0.642787609686539,0.,-0.766044443118978));
#39771=DIRECTION('center_axis',(0.,1.,0.));
#39772=DIRECTION('ref_axis',(0.766044443118978,0.,-0.642787609686539));
#39773=DIRECTION('',(-0.349011634277972,0.,-0.937118391207119));
#39774=DIRECTION('',(0.862276222874172,0.,0.506438264219689));
#39775=DIRECTION('center_axis',(-0.50643826421969,0.,0.862276222874171));
#39776=DIRECTION('ref_axis',(0.862276222874171,0.,0.50643826421969));
#39777=DIRECTION('',(0.,1.,0.));
#39778=DIRECTION('center_axis',(0.937118391207119,0.,-0.349011634277972));
#39779=DIRECTION('ref_axis',(-0.349011634277972,0.,-0.937118391207119));
#39780=DIRECTION('center_axis',(-0.648477023773219,0.,0.761234227842014));
#39781=DIRECTION('ref_axis',(0.761234227842014,0.,0.648477023773219));
#39782=DIRECTION('',(0.761234227842014,0.,0.648477023773219));
#39783=DIRECTION('',(0.,1.,0.));
#39784=DIRECTION('center_axis',(0.983486691428025,0.,-0.180980462437126));
#39785=DIRECTION('ref_axis',(-0.180980462437126,0.,-0.983486691428025));
#39786=DIRECTION('',(-0.180980462437126,0.,-0.983486691428025));
#39787=DIRECTION('center_axis',(0.,1.,0.));
#39788=DIRECTION('ref_axis',(0.866025403784439,0.,-0.5));
#39789=DIRECTION('center_axis',(0.,1.,0.));
#39790=DIRECTION('ref_axis',(0.939692620785908,0.,-0.342020143325669));
#39791=DIRECTION('',(-0.00745029082566112,0.,-0.99997224619817));
#39792=DIRECTION('',(0.637062515999983,0.,0.770812137104607));
#39793=DIRECTION('center_axis',(-0.770812137104607,0.,0.637062515999983));
#39794=DIRECTION('ref_axis',(0.637062515999983,0.,0.770812137104607));
#39795=DIRECTION('',(0.,1.,0.));
#39796=DIRECTION('center_axis',(0.99997224619817,0.,-0.00745029082566112));
#39797=DIRECTION('ref_axis',(-0.00745029082566112,0.,-0.99997224619817));
#39798=DIRECTION('center_axis',(-0.869726513699833,0.,0.49353398197848));
#39799=DIRECTION('ref_axis',(0.49353398197848,0.,0.869726513699833));
#39800=DIRECTION('',(0.49353398197848,0.,0.869726513699833));
#39801=DIRECTION('',(0.,1.,0.));
#39802=DIRECTION('center_axis',(0.986074150277955,0.,0.166306254102512));
#39803=DIRECTION('ref_axis',(0.166306254102512,0.,-0.986074150277955));
#39804=DIRECTION('',(0.166306254102512,0.,-0.986074150277955));
#39805=DIRECTION('center_axis',(0.,1.,0.));
#39806=DIRECTION('ref_axis',(0.984807753012208,0.,-0.17364817766693));
#39807=DIRECTION('center_axis',(0.,1.,0.));
#39808=DIRECTION('ref_axis',(1.,0.,6.12323399573677E-17));
#39809=DIRECTION('',(0.335009667654806,0.,-0.94221469027914));
#39810=DIRECTION('',(0.335009667654806,0.,0.94221469027914));
#39811=DIRECTION('center_axis',(-0.94221469027914,0.,0.335009667654806));
#39812=DIRECTION('ref_axis',(0.335009667654806,0.,0.94221469027914));
#39813=DIRECTION('',(0.,1.,0.));
#39814=DIRECTION('center_axis',(0.94221469027914,0.,0.335009667654806));
#39815=DIRECTION('ref_axis',(0.335009667654806,0.,-0.94221469027914));
#39816=DIRECTION('center_axis',(-0.986074150277955,0.,0.166306254102512));
#39817=DIRECTION('ref_axis',(0.166306254102512,0.,0.986074150277955));
#39818=DIRECTION('',(0.166306254102512,0.,0.986074150277955));
#39819=DIRECTION('',(0.,1.,0.));
#39820=DIRECTION('center_axis',(0.869726513699833,0.,0.49353398197848));
#39821=DIRECTION('ref_axis',(0.49353398197848,0.,-0.869726513699833));
#39822=DIRECTION('',(0.49353398197848,0.,-0.869726513699833));
#39823=DIRECTION('center_axis',(0.,1.,0.));
#39824=DIRECTION('ref_axis',(0.984807753012208,0.,0.17364817766693));
#39825=DIRECTION('center_axis',(0.,1.,0.));
#39826=DIRECTION('ref_axis',(0.939692620785908,0.,0.342020143325669));
#39827=DIRECTION('',(0.637062515999983,0.,-0.770812137104607));
#39828=DIRECTION('',(-0.00745029082566129,0.,0.99997224619817));
#39829=DIRECTION('center_axis',(-0.99997224619817,0.,-0.00745029082566129));
#39830=DIRECTION('ref_axis',(-0.00745029082566129,0.,0.99997224619817));
#39831=DIRECTION('',(0.,1.,0.));
#39832=DIRECTION('center_axis',(0.770812137104607,0.,0.637062515999983));
#39833=DIRECTION('ref_axis',(0.637062515999983,0.,-0.770812137104607));
#39834=DIRECTION('center_axis',(-0.983486691428025,0.,-0.180980462437126));
#39835=DIRECTION('ref_axis',(-0.180980462437126,0.,0.983486691428025));
#39836=DIRECTION('',(-0.180980462437126,0.,0.983486691428025));
#39837=DIRECTION('',(0.,1.,0.));
#39838=DIRECTION('center_axis',(0.648477023773219,0.,0.761234227842014));
#39839=DIRECTION('ref_axis',(0.761234227842014,0.,-0.648477023773219));
#39840=DIRECTION('',(0.761234227842014,0.,-0.648477023773219));
#39841=DIRECTION('center_axis',(0.,1.,0.));
#39842=DIRECTION('ref_axis',(0.866025403784439,0.,0.5));
#39843=DIRECTION('center_axis',(0.,1.,0.));
#39844=DIRECTION('ref_axis',(0.766044443118978,0.,0.642787609686539));
#39845=DIRECTION('',(0.862276222874172,0.,-0.506438264219689));
#39846=DIRECTION('',(-0.349011634277972,0.,0.937118391207119));
#39847=DIRECTION('center_axis',(-0.937118391207119,0.,-0.349011634277972));
#39848=DIRECTION('ref_axis',(-0.349011634277972,0.,0.937118391207119));
#39849=DIRECTION('',(0.,1.,0.));
#39850=DIRECTION('center_axis',(0.50643826421969,0.,0.862276222874171));
#39851=DIRECTION('ref_axis',(0.862276222874171,0.,-0.50643826421969));
#39852=DIRECTION('center_axis',(-0.862276222874171,0.,-0.50643826421969));
#39853=DIRECTION('ref_axis',(-0.50643826421969,0.,0.862276222874171));
#39854=DIRECTION('',(-0.50643826421969,0.,0.862276222874171));
#39855=DIRECTION('',(0.,1.,0.));
#39856=DIRECTION('center_axis',(0.349011634277972,0.,0.937118391207119));
#39857=DIRECTION('ref_axis',(0.937118391207119,0.,-0.349011634277972));
#39858=DIRECTION('',(0.937118391207119,0.,-0.349011634277972));
#39859=DIRECTION('center_axis',(0.,1.,0.));
#39860=DIRECTION('ref_axis',(0.642787609686539,0.,0.766044443118978));
#39861=DIRECTION('center_axis',(0.,1.,0.));
#39862=DIRECTION('ref_axis',(0.5,0.,0.866025403784439));
#39863=DIRECTION('',(0.983486691428025,0.,-0.180980462437126));
#39864=DIRECTION('',(-0.648477023773219,0.,0.761234227842014));
#39865=DIRECTION('center_axis',(-0.761234227842014,0.,-0.648477023773219));
#39866=DIRECTION('ref_axis',(-0.648477023773219,0.,0.761234227842014));
#39867=DIRECTION('',(0.,1.,0.));
#39868=DIRECTION('center_axis',(0.180980462437126,0.,0.983486691428025));
#39869=DIRECTION('ref_axis',(0.983486691428025,0.,-0.180980462437126));
#39870=DIRECTION('center_axis',(-0.637062515999983,0.,-0.770812137104607));
#39871=DIRECTION('ref_axis',(-0.770812137104607,0.,0.637062515999983));
#39872=DIRECTION('',(-0.770812137104607,0.,0.637062515999983));
#39873=DIRECTION('',(0.,1.,0.));
#39874=DIRECTION('center_axis',(0.00745029082566112,0.,0.99997224619817));
#39875=DIRECTION('ref_axis',(0.99997224619817,0.,-0.00745029082566112));
#39876=DIRECTION('',(0.99997224619817,0.,-0.00745029082566112));
#39877=DIRECTION('center_axis',(0.,1.,0.));
#39878=DIRECTION('ref_axis',(0.342020143325669,0.,0.939692620785908));
#39879=DIRECTION('center_axis',(0.,1.,0.));
#39880=DIRECTION('ref_axis',(0.17364817766693,0.,0.984807753012208));
#39881=DIRECTION('',(0.986074150277955,0.,0.166306254102512));
#39882=DIRECTION('',(-0.869726513699833,0.,0.49353398197848));
#39883=DIRECTION('center_axis',(-0.49353398197848,0.,-0.869726513699833));
#39884=DIRECTION('ref_axis',(-0.869726513699833,0.,0.49353398197848));
#39885=DIRECTION('',(0.,1.,0.));
#39886=DIRECTION('center_axis',(-0.166306254102512,0.,0.986074150277955));
#39887=DIRECTION('ref_axis',(0.986074150277955,0.,0.166306254102512));
#39888=DIRECTION('center_axis',(-0.335009667654806,0.,-0.94221469027914));
#39889=DIRECTION('ref_axis',(-0.94221469027914,0.,0.335009667654806));
#39890=DIRECTION('',(-0.94221469027914,0.,0.335009667654806));
#39891=DIRECTION('',(0.,1.,0.));
#39892=DIRECTION('center_axis',(-0.335009667654806,0.,0.94221469027914));
#39893=DIRECTION('ref_axis',(0.94221469027914,0.,0.335009667654806));
#39894=DIRECTION('',(0.94221469027914,0.,0.335009667654806));
#39895=DIRECTION('center_axis',(0.,1.,0.));
#39896=DIRECTION('ref_axis',(0.,0.,1.));
#39897=DIRECTION('center_axis',(0.,1.,0.));
#39898=DIRECTION('ref_axis',(0.,0.,1.));
#39899=DIRECTION('center_axis',(-1.,0.,0.));
#39900=DIRECTION('ref_axis',(0.,0.,-1.));
#39901=DIRECTION('center_axis',(0.,1.,0.));
#39902=DIRECTION('ref_axis',(1.,0.,0.));
#39903=DIRECTION('center_axis',(0.,1.,0.));
#39904=DIRECTION('ref_axis',(1.,0.,0.));
#39905=DIRECTION('center_axis',(0.,-1.,0.));
#39906=DIRECTION('ref_axis',(1.,0.,0.));
#39907=DIRECTION('center_axis',(0.,-1.,0.));
#39908=DIRECTION('ref_axis',(1.,0.,0.));
#39909=DIRECTION('center_axis',(0.,-1.,0.));
#39910=DIRECTION('ref_axis',(1.,0.,0.));
#39911=DIRECTION('center_axis',(0.,-1.,0.));
#39912=DIRECTION('ref_axis',(1.,0.,0.));
#39913=DIRECTION('center_axis',(0.,-1.,0.));
#39914=DIRECTION('ref_axis',(1.,0.,0.));
#39915=DIRECTION('center_axis',(0.,-1.,0.));
#39916=DIRECTION('ref_axis',(1.,0.,0.));
#39917=DIRECTION('center_axis',(0.,-1.,0.));
#39918=DIRECTION('ref_axis',(1.,0.,0.));
#39919=DIRECTION('',(-0.707106781186552,-0.707106781186543,-8.65956056235498E-17));
#39920=DIRECTION('center_axis',(0.,-1.,0.));
#39921=DIRECTION('ref_axis',(1.,0.,0.));
#39922=DIRECTION('',(0.,-1.,0.));
#39923=DIRECTION('',(0.,1.,0.));
#39924=DIRECTION('center_axis',(0.,-1.,0.));
#39925=DIRECTION('ref_axis',(1.,0.,0.));
#39926=DIRECTION('center_axis',(0.,-1.,0.));
#39927=DIRECTION('ref_axis',(1.,0.,0.));
#39928=DIRECTION('',(0.,1.,0.));
#39929=DIRECTION('center_axis',(0.,-1.,0.));
#39930=DIRECTION('ref_axis',(1.,0.,0.));
#39931=DIRECTION('',(0.,-1.,0.));
#39932=DIRECTION('center_axis',(0.,-1.,0.));
#39933=DIRECTION('ref_axis',(1.,0.,0.));
#39934=DIRECTION('',(0.,-1.,0.));
#39935=DIRECTION('',(0.,1.,0.));
#39936=DIRECTION('center_axis',(0.,-1.,0.));
#39937=DIRECTION('ref_axis',(1.,0.,0.));
#39938=DIRECTION('center_axis',(0.,-1.,0.));
#39939=DIRECTION('ref_axis',(1.,0.,0.));
#39940=DIRECTION('',(0.,1.,0.));
#39941=DIRECTION('center_axis',(0.,-1.,0.));
#39942=DIRECTION('ref_axis',(1.,0.,0.));
#39943=DIRECTION('',(0.,-1.,0.));
#39944=DIRECTION('center_axis',(0.,-1.,0.));
#39945=DIRECTION('ref_axis',(1.,0.,0.));
#39946=DIRECTION('',(0.,-1.,0.));
#39947=DIRECTION('',(0.,1.,0.));
#39948=DIRECTION('center_axis',(0.,-1.,0.));
#39949=DIRECTION('ref_axis',(1.,0.,0.));
#39950=DIRECTION('center_axis',(0.,-1.,0.));
#39951=DIRECTION('ref_axis',(1.,0.,0.));
#39952=DIRECTION('',(0.,1.,0.));
#39953=DIRECTION('center_axis',(0.,-1.,0.));
#39954=DIRECTION('ref_axis',(1.,0.,0.));
#39955=DIRECTION('',(0.,-1.,0.));
#39956=DIRECTION('center_axis',(0.,0.,1.));
#39957=DIRECTION('ref_axis',(1.,0.,0.));
#39958=DIRECTION('',(1.,0.,0.));
#39959=DIRECTION('',(0.,1.,0.));
#39960=DIRECTION('',(1.,0.,0.));
#39961=DIRECTION('',(0.,1.,0.));
#39962=DIRECTION('center_axis',(-0.866025403784439,0.,0.499999999999999));
#39963=DIRECTION('ref_axis',(0.499999999999999,0.,0.866025403784439));
#39964=DIRECTION('',(0.499999999999999,0.,0.866025403784439));
#39965=DIRECTION('',(0.,1.,0.));
#39966=DIRECTION('',(0.499999999999999,0.,0.866025403784439));
#39967=DIRECTION('center_axis',(-0.866025403784439,0.,-0.499999999999999));
#39968=DIRECTION('ref_axis',(-0.499999999999999,0.,0.866025403784439));
#39969=DIRECTION('',(-0.499999999999999,0.,0.866025403784439));
#39970=DIRECTION('',(0.,1.,0.));
#39971=DIRECTION('',(-0.499999999999999,0.,0.866025403784439));
#39972=DIRECTION('center_axis',(0.,1.,0.));
#39973=DIRECTION('ref_axis',(1.,0.,0.));
#39974=DIRECTION('center_axis',(0.,1.,0.));
#39975=DIRECTION('ref_axis',(1.,0.,0.));
#39976=DIRECTION('center_axis',(0.,1.,0.));
#39977=DIRECTION('ref_axis',(1.,0.,0.));
#39978=DIRECTION('',(-1.,0.,0.));
#39979=DIRECTION('center_axis',(0.,1.,0.));
#39980=DIRECTION('ref_axis',(1.,0.,0.));
#39981=DIRECTION('center_axis',(0.,1.,0.));
#39982=DIRECTION('ref_axis',(1.,0.,0.));
#39983=DIRECTION('',(-0.5,0.,-0.866025403784439));
#39984=DIRECTION('center_axis',(0.,1.,0.));
#39985=DIRECTION('ref_axis',(1.,0.,0.));
#39986=DIRECTION('',(0.5,0.,-0.866025403784439));
#39987=DIRECTION('center_axis',(0.,-1.,0.));
#39988=DIRECTION('ref_axis',(0.,0.,-1.));
#39989=DIRECTION('',(-0.5,0.,-0.866025403784439));
#39990=DIRECTION('center_axis',(0.,-1.,0.));
#39991=DIRECTION('ref_axis',(1.,0.,0.));
#39992=DIRECTION('center_axis',(0.,-1.,0.));
#39993=DIRECTION('ref_axis',(0.,0.,-1.));
#39994=DIRECTION('',(-1.,0.,0.));
#39995=DIRECTION('center_axis',(0.,-1.,0.));
#39996=DIRECTION('ref_axis',(1.,0.,0.));
#39997=DIRECTION('center_axis',(0.,-1.,0.));
#39998=DIRECTION('ref_axis',(0.,0.,-1.));
#39999=DIRECTION('center_axis',(0.,-1.,0.));
#40000=DIRECTION('ref_axis',(1.,0.,0.));
#40001=DIRECTION('center_axis',(0.,-1.,0.));
#40002=DIRECTION('ref_axis',(0.,0.,-1.));
#40003=DIRECTION('center_axis',(0.,-1.,0.));
#40004=DIRECTION('ref_axis',(1.,0.,0.));
#40005=DIRECTION('center_axis',(0.,-1.,0.));
#40006=DIRECTION('ref_axis',(0.,0.,-1.));
#40007=DIRECTION('center_axis',(0.,-1.,0.));
#40008=DIRECTION('ref_axis',(1.,0.,0.));
#40009=DIRECTION('center_axis',(0.,-1.,0.));
#40010=DIRECTION('ref_axis',(0.,0.,-1.));
#40011=DIRECTION('',(0.5,0.,-0.866025403784439));
#40012=DIRECTION('center_axis',(0.,-1.,0.));
#40013=DIRECTION('ref_axis',(1.,0.,0.));
#40014=DIRECTION('center_axis',(0.,-1.,0.));
#40015=DIRECTION('ref_axis',(1.,0.,0.));
#40016=DIRECTION('',(-0.85716730070211,-0.515038074910058,-1.04972719113862E-16));
#40017=DIRECTION('center_axis',(0.866025403784439,0.,-0.5));
#40018=DIRECTION('ref_axis',(-0.5,0.,-0.866025403784439));
#40019=DIRECTION('',(0.,1.,0.));
#40020=DIRECTION('',(0.,1.,0.));
#40021=DIRECTION('center_axis',(0.866025403784439,0.,0.5));
#40022=DIRECTION('ref_axis',(0.5,0.,-0.866025403784439));
#40023=DIRECTION('center_axis',(0.,0.,-1.));
#40024=DIRECTION('ref_axis',(-1.,0.,0.));
#84334=CARTESIAN_POINT('',(0.,0.,0.));
#84335=CARTESIAN_POINT('Origin',(-10.,13.2,3.5));
#84336=CARTESIAN_POINT('',(-11.4635,13.4616367005047,3.50000000259583));
#84337=CARTESIAN_POINT('',(-11.4634991472179,13.3893449541571,3.49842009727736));
#84338=CARTESIAN_POINT('',(-11.4635,13.2,3.5));
#84339=CARTESIAN_POINT('',(-9.36566843221574,13.3006902612923,2.18111573215603));
#84340=CARTESIAN_POINT('Ctrl Pts',(-11.4635,13.4616367005047,3.50000000259583));
#84341=CARTESIAN_POINT('Ctrl Pts',(-11.4635000000769,13.4594692264253,3.45664071964579));
#84342=CARTESIAN_POINT('Ctrl Pts',(-11.4615730750431,13.4572524781583,3.41330134333718));
#84343=CARTESIAN_POINT('Ctrl Pts',(-11.4570944001824,13.4545591997314,3.36303805100765));
#84344=CARTESIAN_POINT('Ctrl Pts',(-11.4564127667556,13.4541776568914,3.35597043620558));
#84345=CARTESIAN_POINT('Ctrl Pts',(-11.4553183718019,13.4536038460783,3.34542659047019));
#84346=CARTESIAN_POINT('Ctrl Pts',(-11.4549445129957,13.4534136947061,3.34194631982525));
#84347=CARTESIAN_POINT('Ctrl Pts',(-11.4542514885814,13.4530713334346,3.33570581660528));
#84348=CARTESIAN_POINT('Ctrl Pts',(-11.4539369444619,13.4529193833867,3.33294512288282));
#84349=CARTESIAN_POINT('Ctrl Pts',(-11.4532344551081,13.4525873268,3.32693181026965));
#84350=CARTESIAN_POINT('Ctrl Pts',(-11.4528434538211,13.4524070545936,3.32367961528733));
#84351=CARTESIAN_POINT('Ctrl Pts',(-11.4517110420546,13.4518974628054,3.31452022986426));
#84352=CARTESIAN_POINT('Ctrl Pts',(-11.4509445077889,13.451566787266,3.3086162818247));
#84353=CARTESIAN_POINT('Ctrl Pts',(-11.4460147637586,13.4495243520316,3.27237981472014));
#84354=CARTESIAN_POINT('Ctrl Pts',(-11.4409368346681,13.4477669423748,3.24218143057608));
#84355=CARTESIAN_POINT('Ctrl Pts',(-11.4054411893259,13.4372267871199,3.06522729157856));
#84356=CARTESIAN_POINT('Ctrl Pts',(-11.3535717993129,13.4279212793678,2.92367650435652));
#84357=CARTESIAN_POINT('Ctrl Pts',(-11.2636712071939,13.4172531649537,2.76090173424482));
#84358=CARTESIAN_POINT('Ctrl Pts',(-11.2450865575485,13.4152229539322,2.73000587678491));
#84359=CARTESIAN_POINT('Ctrl Pts',(-11.2201031001592,13.4127009082363,2.69174646122165));
#84360=CARTESIAN_POINT('Ctrl Pts',(-11.2147474778138,13.4121712784354,2.68371945425952));
#84361=CARTESIAN_POINT('Ctrl Pts',(-11.2060868213118,13.4113319597054,2.67101288472951));
#84362=CARTESIAN_POINT('Ctrl Pts',(-11.2028330858424,13.4110203716262,2.66629883847623));
#84363=CARTESIAN_POINT('Ctrl Pts',(-11.1966858210542,13.4104385885131,2.65750351763395));
#84364=CARTESIAN_POINT('Ctrl Pts',(-11.193798885466,13.4101681513858,2.65341775412679));
#84365=CARTESIAN_POINT('Ctrl Pts',(-11.1872944466276,13.4095649864841,2.64431171863613));
#84366=CARTESIAN_POINT('Ctrl Pts',(-11.1836659282499,13.4092326826582,2.63929940760112));
#84367=CARTESIAN_POINT('Ctrl Pts',(-11.1728692343824,13.4082560013332,2.62458263455339));
#84368=CARTESIAN_POINT('Ctrl Pts',(-11.1656126291685,13.4076150133666,2.61494349620032));
#84369=CARTESIAN_POINT('Ctrl Pts',(-11.092662928475,13.401318311072,2.52049613728245));
#84370=CARTESIAN_POINT('Ctrl Pts',(-11.0179522223292,13.3960590647726,2.44306260042212));
#84371=CARTESIAN_POINT('Ctrl Pts',(-10.8622094018413,13.3861975082971,2.31362134557764));
#84372=CARTESIAN_POINT('Ctrl Pts',(-10.7832221702084,13.3815991271004,2.26005726325232));
#84373=CARTESIAN_POINT('Ctrl Pts',(-10.6899904553064,13.3759949982724,2.20931597205417));
#84374=CARTESIAN_POINT('Ctrl Pts',(-10.6803170670352,13.3754114274331,2.20419107785057));
#84375=CARTESIAN_POINT('Ctrl Pts',(-10.6667905505303,13.3745912607967,2.19721803101913));
#84376=CARTESIAN_POINT('Ctrl Pts',(-10.6629852137812,13.3743600764605,2.19527738489373));
#84377=CARTESIAN_POINT('Ctrl Pts',(-10.6565718222941,13.3739695991742,2.19204198448465));
#84378=CARTESIAN_POINT('Ctrl Pts',(-10.6539683131556,13.3738108502423,2.19073830977841));
#84379=CARTESIAN_POINT('Ctrl Pts',(-10.6487281495498,13.3734908373348,2.18813389347963));
#84380=CARTESIAN_POINT('Ctrl Pts',(-10.6460915013723,13.3733295733911,2.18683334454379));
#84381=CARTESIAN_POINT('Ctrl Pts',(-10.6407323454947,13.3730013235739,2.18420994324195));
#84382=CARTESIAN_POINT('Ctrl Pts',(-10.6380096170278,13.3728343102812,2.18288757492739));
#84383=CARTESIAN_POINT('Ctrl Pts',(-10.6276778956324,13.3721996856272,2.17790924198447));
#84384=CARTESIAN_POINT('Ctrl Pts',(-10.6200415730722,13.3717288373096,2.17431076261737));
#84385=CARTESIAN_POINT('Ctrl Pts',(-10.6019316987249,13.370608738785,2.16596751020181));
#84386=CARTESIAN_POINT('Ctrl Pts',(-10.5914326228172,13.3699566628213,2.1612797560522));
#84387=CARTESIAN_POINT('Ctrl Pts',(-10.5533537362692,13.367584748646,2.14481320251804));
#84388=CARTESIAN_POINT('Ctrl Pts',(-10.5254697749396,13.3658350196347,2.13375955971625));
#84389=CARTESIAN_POINT('Ctrl Pts',(-10.4349209780345,13.3601532833078,2.1010466672274));
#84390=CARTESIAN_POINT('Ctrl Pts',(-10.3711169814764,13.3561537800153,2.08278486941994));
#84391=CARTESIAN_POINT('Ctrl Pts',(-10.2146204612242,13.3466022489873,2.04928995599158));
#84392=CARTESIAN_POINT('Ctrl Pts',(-10.1212603883285,13.3411269864733,2.03852046886337));
#84393=CARTESIAN_POINT('Ctrl Pts',(-10.0168214938582,13.3353405102178,2.03655770780648));
#84394=CARTESIAN_POINT('Ctrl Pts',(-10.0061416505944,13.3347524372917,2.03647391765776));
#84395=CARTESIAN_POINT('Ctrl Pts',(-9.98894652604875,13.3338113372643,2.03652724045638));
#84396=CARTESIAN_POINT('Ctrl Pts',(-9.98243154168301,13.3334560913878,2.03659094974347));
#84397=CARTESIAN_POINT('Ctrl Pts',(-9.9708169785602,13.3328250872998,2.03678210104788));
#84398=CARTESIAN_POINT('Ctrl Pts',(-9.9657172610516,13.3325488200792,2.03689270275051));
#84399=CARTESIAN_POINT('Ctrl Pts',(-9.95503956958434,13.3319720055825,2.03718013646321));
#84400=CARTESIAN_POINT('Ctrl Pts',(-9.94946181114394,13.3316716231658,2.03736221637199));
#84401=CARTESIAN_POINT('Ctrl Pts',(-9.93484842948733,13.3308870162885,2.03792294802465));
#84402=CARTESIAN_POINT('Ctrl Pts',(-9.92581495916483,13.3304043833784,2.03835345666247));
#84403=CARTESIAN_POINT('Ctrl Pts',(-9.8849919337385,13.328233552819,2.04067840038425));
#84404=CARTESIAN_POINT('Ctrl Pts',(-9.85326419092452,13.326574703922,2.04352645668856));
#84405=CARTESIAN_POINT('Ctrl Pts',(-9.76637832118243,13.3220893944813,2.05419416590938));
#84406=CARTESIAN_POINT('Ctrl Pts',(-9.71153349824011,13.3193238498333,2.06413046537932));
#84407=CARTESIAN_POINT('Ctrl Pts',(-9.55673011949273,13.3115244326859,2.10140675421736));
#84408=CARTESIAN_POINT('Ctrl Pts',(-9.45894154015568,13.3066184055781,2.13625411982279));
#84409=CARTESIAN_POINT('Ctrl Pts',(-9.36565800289699,13.3013233430428,2.18112074824442));
#84410=CARTESIAN_POINT('',(-10.6340070945752,13.3,2.18095972236315));
#84411=CARTESIAN_POINT('Origin',(-10.,13.3,3.5));
#84412=CARTESIAN_POINT('Ctrl Pts',(-10.6340070945752,13.3,2.18095972236315));
#84413=CARTESIAN_POINT('Ctrl Pts',(-10.6850438328051,13.3030790375799,2.20549093241817));
#84414=CARTESIAN_POINT('Ctrl Pts',(-10.7346958992828,13.3061580751599,2.23300784107455));
#84415=CARTESIAN_POINT('Ctrl Pts',(-10.7826083532765,13.3092371127398,2.26332849334117));
#84416=CARTESIAN_POINT('Ctrl Pts',(-10.8304973178774,13.3123146408015,2.29363428071045));
#84417=CARTESIAN_POINT('Ctrl Pts',(-10.8766479449887,13.3153921688632,2.32674082310971));
#84418=CARTESIAN_POINT('Ctrl Pts',(-10.9207316621788,13.3184696969249,2.36242123074426));
#84419=CARTESIAN_POINT('Ctrl Pts',(-10.964804673546,13.3215464776025,2.39809297331719));
#84420=CARTESIAN_POINT('Ctrl Pts',(-11.0068113885096,13.32462325828,2.43633702988196));
#84421=CARTESIAN_POINT('Ctrl Pts',(-11.046455477424,13.3277000389576,2.47688554708218));
#84422=CARTESIAN_POINT('Ctrl Pts',(-11.0861023040175,13.3307770321066,2.51743686441816));
#84423=CARTESIAN_POINT('Ctrl Pts',(-11.1233858362807,13.3338540252557,2.5602926053304));
#84424=CARTESIAN_POINT('Ctrl Pts',(-11.1580471976943,13.3369310184047,2.60514865038241));
#84425=CARTESIAN_POINT('Ctrl Pts',(-11.1927217650378,13.3400091838839,2.6500217855244));
#84426=CARTESIAN_POINT('Ctrl Pts',(-11.2247718768695,13.343087349363,2.69689634758693));
#84427=CARTESIAN_POINT('Ctrl Pts',(-11.2539806258271,13.3461655148421,2.7454373186738));
#84428=CARTESIAN_POINT('Ctrl Pts',(-11.2832337604374,13.3492483579054,2.79405205268298));
#84429=CARTESIAN_POINT('Ctrl Pts',(-11.3096366589622,13.3523312009688,2.84433782677361));
#84430=CARTESIAN_POINT('Ctrl Pts',(-11.3330177139849,13.3554140440321,2.89593375843158));
#84431=CARTESIAN_POINT('Ctrl Pts',(-11.3564177009697,13.3584993833159,2.9475714680258));
#84432=CARTESIAN_POINT('Ctrl Pts',(-11.3767907926723,13.3615847225997,3.0005209880128));
#84433=CARTESIAN_POINT('Ctrl Pts',(-11.3940142001552,13.3646700618836,3.05440302989634));
#84434=CARTESIAN_POINT('Ctrl Pts',(-11.4112733415321,13.3677618024086,3.10839686238641));
#84435=CARTESIAN_POINT('Ctrl Pts',(-11.4253696219277,13.3708535429337,3.16332660322355));
#84436=CARTESIAN_POINT('Ctrl Pts',(-11.4362308040338,13.3739452834588,3.21880019995678));
#84437=CARTESIAN_POINT('Ctrl Pts',(-11.4423316239996,13.3756819408631,3.24996019922882));
#84438=CARTESIAN_POINT('Ctrl Pts',(-11.4474126501818,13.3774185982674,3.28129164813557));
#84439=CARTESIAN_POINT('Ctrl Pts',(-11.4514682711404,13.3791552556717,3.31272451342262));
#84440=CARTESIAN_POINT('Ctrl Pts',(-11.459400281725,13.3825518218335,3.37420112149529));
#84441=CARTESIAN_POINT('Ctrl Pts',(-11.4634320084862,13.3859483879953,3.43622799192429));
#84442=CARTESIAN_POINT('Ctrl Pts',(-11.4634991472179,13.3893449541571,3.49842009727736));
#84443=CARTESIAN_POINT('Origin',(-10.,13.2,3.5));
#84444=CARTESIAN_POINT('',(-11.4635,13.9594225818479,3.50000000603013));
#84445=CARTESIAN_POINT('',(-11.4629363565808,13.890319544931,3.49951158075118));
#84446=CARTESIAN_POINT('',(-11.4635,13.2,3.5));
#84447=CARTESIAN_POINT('Ctrl Pts',(-11.4635,13.9594225818479,3.50000000603013));
#84448=CARTESIAN_POINT('Ctrl Pts',(-11.4635000000932,13.9582466062511,3.47738503015688));
#84449=CARTESIAN_POINT('Ctrl Pts',(-11.4629758096419,13.9570856371282,3.45477011473293));
#84450=CARTESIAN_POINT('Ctrl Pts',(-11.4551533251145,13.9485175930481,3.28616518543354));
#84451=CARTESIAN_POINT('Ctrl Pts',(-11.4265472801892,13.9417767639844,3.14201777790797));
#84452=CARTESIAN_POINT('Ctrl Pts',(-11.3670356613366,13.9328211398458,2.97662230864313));
#84453=CARTESIAN_POINT('Ctrl Pts',(-11.3561568005029,13.9312807746578,2.9490470039185));
#84454=CARTESIAN_POINT('Ctrl Pts',(-11.3422380561025,13.9293950845638,2.91668141253647));
#84455=CARTESIAN_POINT('Ctrl Pts',(-11.3399975341956,13.9290939131093,2.91155273807459));
#84456=CARTESIAN_POINT('Ctrl Pts',(-11.3362970383369,13.9286001099927,2.9032128368399));
#84457=CARTESIAN_POINT('Ctrl Pts',(-11.3348547534459,13.9284085183133,2.89999376715706));
#84458=CARTESIAN_POINT('Ctrl Pts',(-11.3322524321439,13.928064319768,2.8942414092527));
#84459=CARTESIAN_POINT('Ctrl Pts',(-11.3310967859915,13.9279119802224,2.89170618992729));
#84460=CARTESIAN_POINT('Ctrl Pts',(-11.3285700688749,13.9275799993336,2.8862048391398));
#84461=CARTESIAN_POINT('Ctrl Pts',(-11.3271963201307,13.9274001996067,2.88324003469209));
#84462=CARTESIAN_POINT('Ctrl Pts',(-11.3233026177517,13.9268925753011,2.87490995177149));
#84463=CARTESIAN_POINT('Ctrl Pts',(-11.3207600096875,13.9265634084605,2.86955541012884));
#84464=CARTESIAN_POINT('Ctrl Pts',(-11.3050471655727,13.9245438356597,2.83697759536428));
#84465=CARTESIAN_POINT('Ctrl Pts',(-11.291069095096,13.9228089061138,2.81015425998862));
#84466=CARTESIAN_POINT('Ctrl Pts',(-11.2052562762834,13.9125753020144,2.65723863443827));
#84467=CARTESIAN_POINT('Ctrl Pts',(-11.1158132283642,13.9035763970159,2.54194922444878));
#84468=CARTESIAN_POINT('Ctrl Pts',(-10.9823275852265,13.8929469874535,2.41444915989708));
#84469=CARTESIAN_POINT('Ctrl Pts',(-10.9527125558145,13.8907196795358,2.38836727534984));
#84470=CARTESIAN_POINT('Ctrl Pts',(-10.9143802523893,13.8879940245031,2.35726675995235));
#84471=CARTESIAN_POINT('Ctrl Pts',(-10.9066194226553,13.8874498136532,2.35109977233512));
#84472=CARTESIAN_POINT('Ctrl Pts',(-10.89424240565,13.8865937367087,2.34146814125312));
#84473=CARTESIAN_POINT('Ctrl Pts',(-10.8896674470801,13.886279815974,2.33795121327366));
#84474=CARTESIAN_POINT('Ctrl Pts',(-10.8811126233196,13.8856974242563,2.33145496087006));
#84475=CARTESIAN_POINT('Ctrl Pts',(-10.8771381595618,13.8854286844339,2.32846868870981));
#84476=CARTESIAN_POINT('Ctrl Pts',(-10.8682837061934,13.8848339895568,2.32188608279294));
#84477=CARTESIAN_POINT('Ctrl Pts',(-10.863396417653,13.8845084214412,2.31829968949218));
#84478=CARTESIAN_POINT('Ctrl Pts',(-10.8491360596189,13.8835661086115,2.30797084216438));
#84479=CARTESIAN_POINT('Ctrl Pts',(-10.8397051896972,13.8829524328757,2.3013087280542));
#84480=CARTESIAN_POINT('Ctrl Pts',(-10.75794967512,13.877711150996,2.24499375678881));
#84481=CARTESIAN_POINT('Ctrl Pts',(-10.6813718847936,13.8733405340097,2.20182308177545));
#84482=CARTESIAN_POINT('Ctrl Pts',(-10.5356758122848,13.8655304543736,2.13615333959942));
#84483=CARTESIAN_POINT('Ctrl Pts',(-10.4678765224952,13.8620703494366,2.11143339811311));
#84484=CARTESIAN_POINT('Ctrl Pts',(-10.3812138451641,13.8575964485435,2.08690683275938));
#84485=CARTESIAN_POINT('Ctrl Pts',(-10.3638043571153,13.8566949105505,2.08232491307433));
#84486=CARTESIAN_POINT('Ctrl Pts',(-10.3139648081243,13.8540953389334,2.07018638305261));
#84487=CARTESIAN_POINT('Ctrl Pts',(-10.2813572106567,13.8523722979068,2.06341422949068));
#84488=CARTESIAN_POINT('Ctrl Pts',(-10.2428440253955,13.8502820368155,2.05677702700672));
#84489=CARTESIAN_POINT('Ctrl Pts',(-10.2371327576853,13.8499706495551,2.05582763374375));
#84490=CARTESIAN_POINT('Ctrl Pts',(-10.2278749273723,13.8494633946948,2.05434508648266));
#84491=CARTESIAN_POINT('Ctrl Pts',(-10.2243317186376,13.8492686626496,2.05379102790929));
#84492=CARTESIAN_POINT('Ctrl Pts',(-10.2180262116206,13.8489210071784,2.05282875306515));
#84493=CARTESIAN_POINT('Ctrl Pts',(-10.2152647443401,13.8487683727909,2.05241541296835));
#84494=CARTESIAN_POINT('Ctrl Pts',(-10.2093072205452,13.8484382488928,2.05154110713939));
#84495=CARTESIAN_POINT('Ctrl Pts',(-10.2061108626171,13.8482606174844,2.05108282197535));
#84496=CARTESIAN_POINT('Ctrl Pts',(-10.1972250165376,13.8477654325336,2.04983879148628));
#84497=CARTESIAN_POINT('Ctrl Pts',(-10.1915324441188,13.8474466398496,2.04907596393223));
#84498=CARTESIAN_POINT('Ctrl Pts',(-10.1590337832059,13.8456183464952,2.04491559801112));
#84499=CARTESIAN_POINT('Ctrl Pts',(-10.1321437466162,13.8440733896872,2.04222765816543));
#84500=CARTESIAN_POINT('Ctrl Pts',(-10.0444080224075,13.8389609006446,2.03590484615251));
#84501=CARTESIAN_POINT('Ctrl Pts',(-9.9834083088122,13.8352969350701,2.03532576228975));
#84502=CARTESIAN_POINT('Ctrl Pts',(-9.80664840950789,13.8246386580238,2.04469273879405));
#84503=CARTESIAN_POINT('Ctrl Pts',(-9.69186441666404,13.8177042430711,2.0646026870416));
#84504=CARTESIAN_POINT('Ctrl Pts',(-9.56473590207054,13.8102871618157,2.10262656021611));
#84505=CARTESIAN_POINT('Ctrl Pts',(-9.54892640258902,13.8093686328021,2.10764946702432));
#84506=CARTESIAN_POINT('Ctrl Pts',(-9.52705109525389,13.8081026449642,2.11501128296192));
#84507=CARTESIAN_POINT('Ctrl Pts',(-9.52091074011626,13.8077478316051,2.11712332589203));
#84508=CARTESIAN_POINT('Ctrl Pts',(-9.5103317775379,13.8071374353213,2.12084099613906));
#84509=CARTESIAN_POINT('Ctrl Pts',(-9.50588654070424,13.8068812242043,2.12242734634818));
#84510=CARTESIAN_POINT('Ctrl Pts',(-9.49669009329876,13.8063517101734,2.12575947942917));
#84511=CARTESIAN_POINT('Ctrl Pts',(-9.49194010454745,13.8060785170797,2.12750846484077));
#84512=CARTESIAN_POINT('Ctrl Pts',(-9.48081921475893,13.8054395726164,2.13166891287029));
#84513=CARTESIAN_POINT('Ctrl Pts',(-9.47445585660575,13.8050744861701,2.13410029385447));
#84514=CARTESIAN_POINT('Ctrl Pts',(-9.45373388380511,13.8038871255502,2.14218421939232));
#84515=CARTESIAN_POINT('Ctrl Pts',(-9.4394473933587,13.8030709326886,2.14801954051584));
#84516=CARTESIAN_POINT('Ctrl Pts',(-9.36511376197395,13.7988331598728,2.17976202314754));
#84517=CARTESIAN_POINT('Ctrl Pts',(-9.30675796476374,13.7955416671563,2.20944756530999));
#84518=CARTESIAN_POINT('Ctrl Pts',(-9.1772978469926,13.7881127463837,2.28662779009391));
#84519=CARTESIAN_POINT('Ctrl Pts',(-9.10798034530001,13.7840406018752,2.33663799170221));
#84520=CARTESIAN_POINT('Ctrl Pts',(-9.00311977632505,13.7771772823459,2.4272013350867));
#84521=CARTESIAN_POINT('Ctrl Pts',(-8.96475704843755,13.7744821341029,2.46417276740201));
#84522=CARTESIAN_POINT('Ctrl Pts',(-8.92363169648773,13.7712600813543,2.50837781449751));
#84523=CARTESIAN_POINT('Ctrl Pts',(-8.91880422234596,13.7708762607193,2.51364358884478));
#84524=CARTESIAN_POINT('Ctrl Pts',(-8.91165492421536,13.7702990355094,2.52155754009971));
#84525=CARTESIAN_POINT('Ctrl Pts',(-8.9093037212749,13.7701077579779,2.52417917712055));
#84526=CARTESIAN_POINT('Ctrl Pts',(-8.90510997094335,13.7697639329295,2.52888938253385));
#84527=CARTESIAN_POINT('Ctrl Pts',(-8.90326390156836,13.7696116507789,2.5309747488697));
#84528=CARTESIAN_POINT('Ctrl Pts',(-8.89926360226851,13.7692796205003,2.53551966199074));
#84529=CARTESIAN_POINT('Ctrl Pts',(-8.89711168865999,13.7690997129631,2.53798112701712));
#84530=CARTESIAN_POINT('Ctrl Pts',(-8.89107011014472,13.7685910028816,2.54493869621058));
#84531=CARTESIAN_POINT('Ctrl Pts',(-8.88719961420015,13.7682608462765,2.54945126716448));
#84532=CARTESIAN_POINT('Ctrl Pts',(-8.8635497141802,13.766217808896,2.57736685216161));
#84533=CARTESIAN_POINT('Ctrl Pts',(-8.84448315881396,13.7644591635936,2.60136117517366));
#84534=CARTESIAN_POINT('Ctrl Pts',(-8.73554217686856,13.7538079833206,2.74766201824499));
#84535=CARTESIAN_POINT('Ctrl Pts',(-8.66437662775479,13.744385681221,2.88275561968854));
#84536=CARTESIAN_POINT('Ctrl Pts',(-8.60442310346896,13.7337897297474,3.05805391710281));
#84537=CARTESIAN_POINT('Ctrl Pts',(-8.59468597150639,13.7319093371147,3.09006835616096));
#84538=CARTESIAN_POINT('Ctrl Pts',(-8.58360833507799,13.7295414318251,3.13154817302867));
#84539=CARTESIAN_POINT('Ctrl Pts',(-8.58125162591186,13.7290215125677,3.14072969197802));
#84540=CARTESIAN_POINT('Ctrl Pts',(-8.57764152850863,13.7281982488104,3.1553840703986));
#84541=CARTESIAN_POINT('Ctrl Pts',(-8.57633016892955,13.7278930570218,3.16084225840401));
#84542=CARTESIAN_POINT('Ctrl Pts',(-8.5740278861272,13.7273458954099,3.17067358926938));
#84543=CARTESIAN_POINT('Ctrl Pts',(-8.57302560010035,13.72710356593,3.17504397682378));
#84544=CARTESIAN_POINT('Ctrl Pts',(-8.57072262296208,13.7265368628499,3.18530207299097));
#84545=CARTESIAN_POINT('Ctrl Pts',(-8.56943819569798,13.7262130100459,3.19119337549489));
#84546=CARTESIAN_POINT('Ctrl Pts',(-8.56582892874529,13.7252797152414,3.20825397631357));
#84547=CARTESIAN_POINT('Ctrl Pts',(-8.56359820630299,13.7246732572833,3.21944287418016));
#84548=CARTESIAN_POINT('Ctrl Pts',(-8.5465582654733,13.7197838869832,3.31044941212668));
#84549=CARTESIAN_POINT('Ctrl Pts',(-8.53828190275751,13.7157184060523,3.39135046083801));
#84550=CARTESIAN_POINT('Ctrl Pts',(-8.53509529062912,13.7073972452405,3.56108490611073));
#84551=CARTESIAN_POINT('Ctrl Pts',(-8.54147527872705,13.7031744766665,3.64960375252398));
#84552=CARTESIAN_POINT('Ctrl Pts',(-8.56246164039444,13.6966733533247,3.77748744368947));
#84553=CARTESIAN_POINT('Ctrl Pts',(-8.57080550919317,13.6945687004384,3.81767649339344));
#84554=CARTESIAN_POINT('Ctrl Pts',(-8.58246251612846,13.6920189662021,3.86395692465306));
#84555=CARTESIAN_POINT('Ctrl Pts',(-8.58414395658109,13.6916586415886,3.87044408762766));
#84556=CARTESIAN_POINT('Ctrl Pts',(-8.58676456801308,13.6911077640926,3.88027612630479));
#84557=CARTESIAN_POINT('Ctrl Pts',(-8.58767121655815,13.6909190241075,3.88362967222534));
#84558=CARTESIAN_POINT('Ctrl Pts',(-8.58932536283157,13.69057790384,3.88966274734633));
#84559=CARTESIAN_POINT('Ctrl Pts',(-8.59006856730329,13.6904257711126,3.89234339997065));
#84560=CARTESIAN_POINT('Ctrl Pts',(-8.59171206152173,13.690091794407,3.89820631503039));
#84561=CARTESIAN_POINT('Ctrl Pts',(-8.59261548591959,13.6899097753758,3.90138761325441));
#84562=CARTESIAN_POINT('Ctrl Pts',(-8.59521934268837,13.6893896238694,3.91043990430011));
#84563=CARTESIAN_POINT('Ctrl Pts',(-8.59694576235166,13.6890500432456,3.91630327134095));
#84564=CARTESIAN_POINT('Ctrl Pts',(-8.60849927347496,13.6868122429452,3.95465366924297));
#84565=CARTESIAN_POINT('Ctrl Pts',(-8.61941656009519,13.6848578935218,3.98679897354983));
#84566=CARTESIAN_POINT('Ctrl Pts',(-8.66499946123898,13.6773169190869,4.10710551010846));
#84567=CARTESIAN_POINT('Ctrl Pts',(-8.70707712835278,13.6715271629977,4.19220958991921));
#84568=CARTESIAN_POINT('Ctrl Pts',(-8.80072929427249,13.6609514406805,4.34286216015206));
#84569=CARTESIAN_POINT('Ctrl Pts',(-8.85025105331755,13.6561484314662,4.40925671616065));
#84570=CARTESIAN_POINT('Ctrl Pts',(-8.91223078849635,13.6509717821927,4.47913488835436));
#84571=CARTESIAN_POINT('Ctrl Pts',(-8.91942643893409,13.6503817623822,4.48707029880919));
#84572=CARTESIAN_POINT('Ctrl Pts',(-8.93110771747107,13.6494411612357,4.49967165085258));
#84573=CARTESIAN_POINT('Ctrl Pts',(-8.93553820752311,13.6490882799397,4.50438798051702));
#84574=CARTESIAN_POINT('Ctrl Pts',(-8.94346542384514,13.6484636659082,4.51271526213057));
#84575=CARTESIAN_POINT('Ctrl Pts',(-8.94694972544813,13.6481914098162,4.51633785371999));
#84576=CARTESIAN_POINT('Ctrl Pts',(-8.95425630603311,13.6476251940673,4.52385651543028));
#84577=CARTESIAN_POINT('Ctrl Pts',(-8.9580818611004,13.6473313823767,4.52774930338147));
#84578=CARTESIAN_POINT('Ctrl Pts',(-8.96809807728009,13.6465688991416,4.53782814611052));
#84579=CARTESIAN_POINT('Ctrl Pts',(-8.97432265855781,13.6461017182843,4.5439802846348));
#84580=CARTESIAN_POINT('Ctrl Pts',(-9.00200868570563,13.6440523804781,4.5708574520043));
#84581=CARTESIAN_POINT('Ctrl Pts',(-9.02404653451883,13.6424960837332,4.59097999108372));
#84582=CARTESIAN_POINT('Ctrl Pts',(-9.0853633609575,13.6383462068342,4.64362175013917));
#84583=CARTESIAN_POINT('Ctrl Pts',(-9.1257518097775,13.6358029756795,4.67478573593734));
#84584=CARTESIAN_POINT('Ctrl Pts',(-9.24114667256317,13.6289054313731,4.75457167589954));
#84585=CARTESIAN_POINT('Ctrl Pts',(-9.31909810842037,13.624649504223,4.79852985739633));
#84586=CARTESIAN_POINT('Ctrl Pts',(-9.41064137953276,13.6196378831124,4.8396307855888));
#84587=CARTESIAN_POINT('Ctrl Pts',(-9.42076743193361,13.6190831709443,4.84404012198047));
#84588=CARTESIAN_POINT('Ctrl Pts',(-9.4629288745006,13.6167684568911,4.86183414723024));
#84589=CARTESIAN_POINT('Ctrl Pts',(-9.4953834119252,13.6149746874378,4.87419044353775));
#84590=CARTESIAN_POINT('Ctrl Pts',(-9.53379444185724,13.612804973922,4.88727034426828));
#84591=CARTESIAN_POINT('Ctrl Pts',(-9.53935616335689,13.6124896817394,4.88912702226633));
#84592=CARTESIAN_POINT('Ctrl Pts',(-9.54836048889752,13.611977186569,4.89207292877823));
#84593=CARTESIAN_POINT('Ctrl Pts',(-9.55179628516663,13.6117811543679,4.89318294436378));
#84594=CARTESIAN_POINT('Ctrl Pts',(-9.55790403022811,13.6114317660788,4.89513126463055));
#84595=CARTESIAN_POINT('Ctrl Pts',(-9.56057431345817,13.6112787057201,4.89597462651518));
#84596=CARTESIAN_POINT('Ctrl Pts',(-9.5663286415538,13.6109481914429,4.89777388284596));
#84597=CARTESIAN_POINT('Ctrl Pts',(-9.5694133933102,13.6107705986127,4.89872722445381));
#84598=CARTESIAN_POINT('Ctrl Pts',(-9.57796055429666,13.6102774381241,4.90133776822581));
#84599=CARTESIAN_POINT('Ctrl Pts',(-9.58342948263533,13.6099606579149,4.90297321295187));
#84600=CARTESIAN_POINT('Ctrl Pts',(-9.6140959532309,13.6081780259888,4.91194869252319));
#84601=CARTESIAN_POINT('Ctrl Pts',(-9.63947636422258,13.6066789062582,4.91864145458542));
#84602=CARTESIAN_POINT('Ctrl Pts',(-9.72142668071614,13.6017923649351,4.93791050661331));
#84603=CARTESIAN_POINT('Ctrl Pts',(-9.77856697895659,13.5983175247031,4.94781089984347));
#84604=CARTESIAN_POINT('Ctrl Pts',(-9.95505635661787,13.5876327799909,4.96769647384994));
#84605=CARTESIAN_POINT('Ctrl Pts',(-10.0751896132792,13.5804711804802,4.96646142213768));
#84606=CARTESIAN_POINT('Ctrl Pts',(-10.2099635213672,13.5728752368683,4.94845160092698));
#84607=CARTESIAN_POINT('Ctrl Pts',(-10.2260461936635,13.5719749975809,4.94602899997067));
#84608=CARTESIAN_POINT('Ctrl Pts',(-10.2484436898104,13.5707295514294,4.94227235476854));
#84609=CARTESIAN_POINT('Ctrl Pts',(-10.2547947165544,13.5703773236158,4.94116392773745));
#84610=CARTESIAN_POINT('Ctrl Pts',(-10.2657772029017,13.569769799548,4.939172316186));
#84611=CARTESIAN_POINT('Ctrl Pts',(-10.2704120670037,13.5695138939623,4.93830865672145));
#84612=CARTESIAN_POINT('Ctrl Pts',(-10.280035425227,13.5689835369843,4.93646728136238));
#84613=CARTESIAN_POINT('Ctrl Pts',(-10.285023166984,13.5687092037159,4.93548594036558));
#84614=CARTESIAN_POINT('Ctrl Pts',(-10.296758206342,13.5680650083923,4.93311349040502));
#84615=CARTESIAN_POINT('Ctrl Pts',(-10.3035010274427,13.5676958366373,4.93170068029508));
#84616=CARTESIAN_POINT('Ctrl Pts',(-10.3256932994976,13.5664838503899,4.92688695024322));
#84617=CARTESIAN_POINT('Ctrl Pts',(-10.3410978844261,13.5656474572788,4.92328308954725));
#84618=CARTESIAN_POINT('Ctrl Pts',(-10.4228401171124,13.561231270936,4.90275631766725));
#84619=CARTESIAN_POINT('Ctrl Pts',(-10.4879903292252,13.5577946123582,4.88144340446504));
#84620=CARTESIAN_POINT('Ctrl Pts',(-10.6308570509259,13.5502089456224,4.82333173734331));
#84621=CARTESIAN_POINT('Ctrl Pts',(-10.7073017897354,13.5461166784398,4.7840991962932));
#84622=CARTESIAN_POINT('Ctrl Pts',(-10.7921411472125,13.5411329603865,4.73067257558485));
#84623=CARTESIAN_POINT('Ctrl Pts',(-10.8042976167603,13.5404071780409,4.72276241043271));
#84624=CARTESIAN_POINT('Ctrl Pts',(-10.8460586041076,13.5378661800646,4.69469648358011));
#84625=CARTESIAN_POINT('Ctrl Pts',(-10.8750374289745,13.5360182903242,4.67363706176502));
#84626=CARTESIAN_POINT('Ctrl Pts',(-10.9078697001915,13.5337875407603,4.64788496434825));
#84627=CARTESIAN_POINT('Ctrl Pts',(-10.9125046703904,13.5334693134436,4.64420387521335));
#84628=CARTESIAN_POINT('Ctrl Pts',(-10.9199122754855,13.5329551542494,4.63824712632199));
#84629=CARTESIAN_POINT('Ctrl Pts',(-10.9226991433255,13.5327604391648,4.63598917491196));
#84630=CARTESIAN_POINT('Ctrl Pts',(-10.9276408041016,13.532412832639,4.63195520490714));
#84631=CARTESIAN_POINT('Ctrl Pts',(-10.9297988855222,13.5322602287105,4.63018320628363));
#84632=CARTESIAN_POINT('Ctrl Pts',(-10.934388960798,13.5319339148781,4.62639225431527));
#84633=CARTESIAN_POINT('Ctrl Pts',(-10.9368194853879,13.531760083796,4.62437159873695));
#84634=CARTESIAN_POINT('Ctrl Pts',(-10.9434705181101,13.5312815814992,4.61880561922792));
#84635=CARTESIAN_POINT('Ctrl Pts',(-10.9476775274277,13.5309757776052,4.61524433832486));
#84636=CARTESIAN_POINT('Ctrl Pts',(-10.9701241157657,13.5293277513058,4.5960243288098));
#84637=CARTESIAN_POINT('Ctrl Pts',(-10.98799491515,13.5279572386478,4.57994260845164));
#84638=CARTESIAN_POINT('Ctrl Pts',(-11.0419494396188,13.5236572263307,4.52892920382205));
#84639=CARTESIAN_POINT('Ctrl Pts',(-11.076636453377,13.5206592227322,4.49257608025498));
#84640=CARTESIAN_POINT('Ctrl Pts',(-11.1923353415791,13.5099902721221,4.35810511989452));
#84641=CARTESIAN_POINT('Ctrl Pts',(-11.2623822355807,13.5023051830361,4.25127249846792));
#84642=CARTESIAN_POINT('Ctrl Pts',(-11.3262086327459,13.4940676108242,4.11917871858112));
#84643=CARTESIAN_POINT('Ctrl Pts',(-11.3343319135663,13.4929858020648,4.101473207523));
#84644=CARTESIAN_POINT('Ctrl Pts',(-11.3451579691168,13.4914948834813,4.07657706026865));
#84645=CARTESIAN_POINT('Ctrl Pts',(-11.3481610218037,13.4910755909108,4.0695199125207));
#84646=CARTESIAN_POINT('Ctrl Pts',(-11.3529060979015,13.4904036106651,4.058121150634));
#84647=CARTESIAN_POINT('Ctrl Pts',(-11.354682995527,13.4901497452288,4.05379428569315));
#84648=CARTESIAN_POINT('Ctrl Pts',(-11.3583266831376,13.4896244685637,4.04479918142102));
#84649=CARTESIAN_POINT('Ctrl Pts',(-11.3601902250354,13.4893531695293,4.04012968701556));
#84650=CARTESIAN_POINT('Ctrl Pts',(-11.3645121780949,13.488717620863,4.02913590363951));
#84651=CARTESIAN_POINT('Ctrl Pts',(-11.3669507546732,13.4883540400027,4.02280390694054));
#84652=CARTESIAN_POINT('Ctrl Pts',(-11.3747978217616,13.487167279424,4.00199794760603));
#84653=CARTESIAN_POINT('Ctrl Pts',(-11.3800212443667,13.4863502529278,3.98745500236345));
#84654=CARTESIAN_POINT('Ctrl Pts',(-11.406319013975,13.4820841955652,3.91042385655824));
#84655=CARTESIAN_POINT('Ctrl Pts',(-11.4233832728651,13.4787684450086,3.84664427799868));
#84656=CARTESIAN_POINT('Ctrl Pts',(-11.4523955575071,13.4713531112475,3.69885980015698));
#84657=CARTESIAN_POINT('Ctrl Pts',(-11.4614643780711,13.4673149955992,3.61453917439005));
#84658=CARTESIAN_POINT('Ctrl Pts',(-11.4633981313327,13.462630799978,3.51993994582104));
#84659=CARTESIAN_POINT('Ctrl Pts',(-11.4634999999823,13.4621350600777,3.50996944764625));
#84660=CARTESIAN_POINT('Ctrl Pts',(-11.4635,13.4616367005047,3.50000000259583));
#84661=CARTESIAN_POINT('Ctrl Pts',(-11.4638034778342,13.3888174556321,3.49845133854934));
#84662=CARTESIAN_POINT('Ctrl Pts',(-11.4637389471014,13.3919645434129,3.55221748613726));
#84663=CARTESIAN_POINT('Ctrl Pts',(-11.4606820604459,13.3951565851578,3.60609881299289));
#84664=CARTESIAN_POINT('Ctrl Pts',(-11.4546528039997,13.3983331287172,3.65973463770758));
#84665=CARTESIAN_POINT('Ctrl Pts',(-11.4486311466748,13.4015056686419,3.71330286119413));
#84666=CARTESIAN_POINT('Ctrl Pts',(-11.4396448753746,13.4046624601302,3.76662621772362));
#84667=CARTESIAN_POINT('Ctrl Pts',(-11.427751489726,13.4077628611718,3.81935395290464));
#84668=CARTESIAN_POINT('Ctrl Pts',(-11.4158679180049,13.4108607038912,3.87203817935049));
#84669=CARTESIAN_POINT('Ctrl Pts',(-11.4010370563809,13.4138754519379,3.92411692140531));
#84670=CARTESIAN_POINT('Ctrl Pts',(-11.3833734100942,13.4168000700608,3.97524255973066));
#84671=CARTESIAN_POINT('Ctrl Pts',(-11.365716659341,13.4197235464714,4.02634823963184));
#84672=CARTESIAN_POINT('Ctrl Pts',(-11.3453758482529,13.422647278177,4.07655708571848));
#84673=CARTESIAN_POINT('Ctrl Pts',(-11.3223609188837,13.4255094599703,4.12551597861373));
#84674=CARTESIAN_POINT('Ctrl Pts',(-11.2993281844628,13.4283738560348,4.17451274760263));
#84675=CARTESIAN_POINT('Ctrl Pts',(-11.2735457975972,13.4311296631554,4.22221618697834));
#84676=CARTESIAN_POINT('Ctrl Pts',(-11.2452411977534,13.4338443445426,4.2683285929259));
#84677=CARTESIAN_POINT('Ctrl Pts',(-11.2169266033059,13.4365599845077,4.31445728157045));
#84678=CARTESIAN_POINT('Ctrl Pts',(-11.1860867348378,13.4392347488967,4.35899583250288));
#84679=CARTESIAN_POINT('Ctrl Pts',(-11.1529218371365,13.4419159292845,4.4016390119544));
#84680=CARTESIAN_POINT('Ctrl Pts',(-11.119693539766,13.4446022351502,4.44436371023027));
#84681=CARTESIAN_POINT('Ctrl Pts',(-11.0841310338689,13.4472954693768,4.48518531569453));
#84682=CARTESIAN_POINT('Ctrl Pts',(-11.0464774039781,13.4500570205331,4.52381765057115));
#84683=CARTESIAN_POINT('Ctrl Pts',(-11.0149929368743,13.4523661197298,4.55612047184215));
#84684=CARTESIAN_POINT('Ctrl Pts',(-10.9820471053411,13.4547234711996,4.58689275186817));
#84685=CARTESIAN_POINT('Ctrl Pts',(-10.947806378907,13.457167717929,4.61598287146918));
#84686=CARTESIAN_POINT('Ctrl Pts',(-10.9477906510602,13.4571688406487,4.61599623347969));
#84687=CARTESIAN_POINT('Ctrl Pts',(-10.94777492294,13.4571699633867,4.61600959513598));
#84688=CARTESIAN_POINT('Ctrl Pts',(-10.9477591945465,13.4571710861431,4.61602295643805));
#84689=CARTESIAN_POINT('Ctrl Pts',(-10.9094872476417,13.4599030925948,4.64853505276661));
#84690=CARTESIAN_POINT('Ctrl Pts',(-10.869431407601,13.4627519499741,4.67908033928225));
#84691=CARTESIAN_POINT('Ctrl Pts',(-10.8278340982856,13.4656578568494,4.70748720938998));
#84692=CARTESIAN_POINT('Ctrl Pts',(-10.8237759029398,13.465941354459,4.71025855758433));
#84693=CARTESIAN_POINT('Ctrl Pts',(-10.8197030771707,13.4662253950528,4.71300955229469));
#84694=CARTESIAN_POINT('Ctrl Pts',(-10.815615872548,13.4665099231026,4.71574003452877));
#84695=CARTESIAN_POINT('Ctrl Pts',(-10.7697160879684,13.4697052062841,4.74640366845739));
#84696=CARTESIAN_POINT('Ctrl Pts',(-10.7219970544357,13.4729613189875,4.77448093742227));
#84697=CARTESIAN_POINT('Ctrl Pts',(-10.6727944195478,13.4762124530802,4.79979131982366));
#84698=CARTESIAN_POINT('Ctrl Pts',(-10.6236407645761,13.4794603507553,4.82507650641162));
#84699=CARTESIAN_POINT('Ctrl Pts',(-10.5730065714788,13.4827029317654,4.84760067203343));
#84700=CARTESIAN_POINT('Ctrl Pts',(-10.5212366024711,13.4858947597026,4.86722193790353));
#84701=CARTESIAN_POINT('Ctrl Pts',(-10.469497861905,13.48908466228,4.88683136792424));
#84702=CARTESIAN_POINT('Ctrl Pts',(-10.4166247401001,13.4922237292158,4.90354154255135));
#84703=CARTESIAN_POINT('Ctrl Pts',(-10.3629705797557,13.4952903731062,4.91724518846785));
#84704=CARTESIAN_POINT('Ctrl Pts',(-10.309327739629,13.498356369981,4.93094594312197));
#84705=CARTESIAN_POINT('Ctrl Pts',(-10.254904202352,13.5013499723776,4.94164140890122));
#84706=CARTESIAN_POINT('Ctrl Pts',(-10.2000620512057,13.504274428245,4.94925790984549));
#84707=CARTESIAN_POINT('Ctrl Pts',(-10.1451707659611,13.5072015041865,4.95688123455394));
#84708=CARTESIAN_POINT('Ctrl Pts',(-10.0898601359871,13.5100594326265,4.96141989310606));
#84709=CARTESIAN_POINT('Ctrl Pts',(-10.0345019800102,13.5128754485554,4.96283519573269));
#84710=CARTESIAN_POINT('Ctrl Pts',(-9.97911943547413,13.5156927051067,4.96425112188427));
#84711=CARTESIAN_POINT('Ctrl Pts',(-9.92368938023504,13.5184682986004,4.96254059815874));
#84712=CARTESIAN_POINT('Ctrl Pts',(-9.86859235972315,13.5212504641971,4.95770397676074));
#84713=CARTESIAN_POINT('Ctrl Pts',(-9.81339269079736,13.5240378131028,4.95285834450317));
#84714=CARTESIAN_POINT('Ctrl Pts',(-9.75852748088284,13.5268322697061,4.94487441448456));
#84715=CARTESIAN_POINT('Ctrl Pts',(-9.7043860069233,13.5296974670412,4.93379840192616));
#84716=CARTESIAN_POINT('Ctrl Pts',(-9.66259727071438,13.5319089505282,4.92524945537559));
#84717=CARTESIAN_POINT('Ctrl Pts',(-9.62123992915594,13.5341630234317,4.9148592385162));
#84718=CARTESIAN_POINT('Ctrl Pts',(-9.58049393286608,13.5364914585468,4.90267111986085));
#84719=CARTESIAN_POINT('Ctrl Pts',(-9.58047693404163,13.5364924299468,4.90266603509895));
#84720=CARTESIAN_POINT('Ctrl Pts',(-9.58045993532319,13.5364934013597,4.90266095002429));
#84721=CARTESIAN_POINT('Ctrl Pts',(-9.58044293671079,13.5364943727856,4.90265586463689));
#84722=CARTESIAN_POINT('Ctrl Pts',(-9.53202383501105,13.5392613967326,4.88817057112994));
#84723=CARTESIAN_POINT('Ctrl Pts',(-9.48429284608302,13.5421405845651,4.87108885568505));
#84724=CARTESIAN_POINT('Ctrl Pts',(-9.43753012185968,13.5450718499842,4.85152258524947));
#84725=CARTESIAN_POINT('Ctrl Pts',(-9.43327565767751,13.5453385359813,4.84974244950825));
#84726=CARTESIAN_POINT('Ctrl Pts',(-9.42902922831058,13.5456056530415,4.84794177767954));
#84727=CARTESIAN_POINT('Ctrl Pts',(-9.42479105634956,13.5458731559159,4.84612067190963));
#84728=CARTESIAN_POINT('Ctrl Pts',(-9.37405702481399,13.5490753618169,4.82432069814493));
#84729=CARTESIAN_POINT('Ctrl Pts',(-9.32450261137027,13.5523322309487,4.79958811715058));
#84730=CARTESIAN_POINT('Ctrl Pts',(-9.27646151112173,13.5555794400524,4.77210561834639));
#84731=CARTESIAN_POINT('Ctrl Pts',(-9.22846654423733,13.5588235308954,4.74464951069724));
#84732=CARTESIAN_POINT('Ctrl Pts',(-9.18198175759054,13.5620576470011,4.71444904085066));
#84733=CARTESIAN_POINT('Ctrl Pts',(-9.13731388703022,13.5652380057577,4.6817155957195));
#84734=CARTESIAN_POINT('Ctrl Pts',(-9.09267141884258,13.5684165558619,4.64900076591882));
#84735=CARTESIAN_POINT('Ctrl Pts',(-9.04984370571082,13.5715412748565,4.61375593455757));
#84736=CARTESIAN_POINT('Ctrl Pts',(-9.00911342310494,13.5745922292323,4.57621866854711));
#84737=CARTESIAN_POINT('Ctrl Pts',(-8.96839035491113,13.5776426432032,4.5386880513809));
#84738=CARTESIAN_POINT('Ctrl Pts',(-8.92976401327719,13.5806193232223,4.49886580285893));
#84739=CARTESIAN_POINT('Ctrl Pts',(-8.89349379236424,13.5835270645262,4.45701531701962));
#84740=CARTESIAN_POINT('Ctrl Pts',(-8.85718929406797,13.586437553808,4.41512528013517));
#84741=CARTESIAN_POINT('Ctrl Pts',(-8.82324554259782,13.5892791041831,4.37120308457584));
#84742=CARTESIAN_POINT('Ctrl Pts',(-8.79189791977439,13.5920803007864,4.32553960581249));
#84743=CARTESIAN_POINT('Ctrl Pts',(-8.76053561004683,13.5948828097989,4.2798547329186));
#84744=CARTESIAN_POINT('Ctrl Pts',(-8.73177218894977,13.597645223792,4.2324268041065));
#84745=CARTESIAN_POINT('Ctrl Pts',(-8.70581493137394,13.6004168019331,4.18357557404067));
#84746=CARTESIAN_POINT('Ctrl Pts',(-8.67980828609894,13.6031936534305,4.13463139695039));
#84747=CARTESIAN_POINT('Ctrl Pts',(-8.65661905923465,13.6059802289843,4.08425835729951));
#84748=CARTESIAN_POINT('Ctrl Pts',(-8.63642053376971,13.6088406852103,4.03280883998907));
#84749=CARTESIAN_POINT('Ctrl Pts',(-8.62090319297247,13.6110382057259,3.99328319761756));
#84750=CARTESIAN_POINT('Ctrl Pts',(-8.6071503804057,13.613279763713,3.9531228751966));
#84751=CARTESIAN_POINT('Ctrl Pts',(-8.59522272434344,13.6155966400574,3.91250036744496));
#84752=CARTESIAN_POINT('Ctrl Pts',(-8.59521747235296,13.6155976602254,3.91248248052545));
#84753=CARTESIAN_POINT('Ctrl Pts',(-8.59521222071596,13.6155986804079,3.91246459351607));
#84754=CARTESIAN_POINT('Ctrl Pts',(-8.59520696943243,13.6155997006051,3.91244670641683));
#84755=CARTESIAN_POINT('Ctrl Pts',(-8.58103522202286,13.6183529277781,3.86417442201071));
#84756=CARTESIAN_POINT('Ctrl Pts',(-8.56939194522168,13.6212198794063,3.81506537742746));
#84757=CARTESIAN_POINT('Ctrl Pts',(-8.56033681483484,13.6241402746798,3.76541254431727));
#84758=CARTESIAN_POINT('Ctrl Pts',(-8.55950142175534,13.6244096996241,3.76083175625723));
#84759=CARTESIAN_POINT('Ctrl Pts',(-8.55868804299287,13.6246795794397,3.75624637375511));
#84760=CARTESIAN_POINT('Ctrl Pts',(-8.55789671636854,13.624949866793,3.75165664722065));
#84761=CARTESIAN_POINT('Ctrl Pts',(-8.5485449206615,13.6281440877793,3.69741585260893));
#84762=CARTESIAN_POINT('Ctrl Pts',(-8.54227472254286,13.6313946029861,3.64256284387078));
#84763=CARTESIAN_POINT('Ctrl Pts',(-8.53911607976639,13.6346365187915,3.58747478516665));
#84764=CARTESIAN_POINT('Ctrl Pts',(-8.53596063262516,13.6378751547133,3.53244245968546));
#84765=CARTESIAN_POINT('Ctrl Pts',(-8.53591009395743,13.6411048750132,3.47717552279635));
#84766=CARTESIAN_POINT('Ctrl Pts',(-8.5389556392251,13.6442812733838,3.42204434808979));
#84767=CARTESIAN_POINT('Ctrl Pts',(-8.54199931682544,13.647455723842,3.36694698233559));
#84768=CARTESIAN_POINT('Ctrl Pts',(-8.54813515207398,13.6505767818087,3.31198518841675));
#84769=CARTESIAN_POINT('Ctrl Pts',(-8.55731922032615,13.6536238408607,3.25752355090235));
#84770=CARTESIAN_POINT('Ctrl Pts',(-8.5665013158374,13.6566702454034,3.20307361176588));
#84771=CARTESIAN_POINT('Ctrl Pts',(-8.57873036085231,13.6596426850592,3.14912364743867));
#84772=CARTESIAN_POINT('Ctrl Pts',(-8.59392807648934,13.6625452517985,3.09603284314746));
#84773=CARTESIAN_POINT('Ctrl Pts',(-8.60913971754387,13.6654504781121,3.0428933926233));
#84774=CARTESIAN_POINT('Ctrl Pts',(-8.62732563089968,13.6682858291034,2.99061477778822));
#84775=CARTESIAN_POINT('Ctrl Pts',(-8.6483714712423,13.6710792000015,2.93955100388496));
#84776=CARTESIAN_POINT('Ctrl Pts',(-8.66942672598226,13.6738738204532,2.88846438771693));
#84777=CARTESIAN_POINT('Ctrl Pts',(-8.69334475356521,13.6766267119448,2.83859389722841));
#84778=CARTESIAN_POINT('Ctrl Pts',(-8.71997185679439,13.6793865475947,2.79028566021711));
#84779=CARTESIAN_POINT('Ctrl Pts',(-8.74664989035071,13.6821516620514,2.74188502283116));
#84780=CARTESIAN_POINT('Ctrl Pts',(-8.77604778932435,13.6849242600086,2.6950530123612));
#84781=CARTESIAN_POINT('Ctrl Pts',(-8.80796629411427,13.6877681689548,2.65012506096888));
#84782=CARTESIAN_POINT('Ctrl Pts',(-8.83337919098557,13.6900324343155,2.61435429404583));
#84783=CARTESIAN_POINT('Ctrl Pts',(-8.86038912178864,13.6923423747132,2.57979044471691));
#84784=CARTESIAN_POINT('Ctrl Pts',(-8.88887257476405,13.6947328382195,2.54659367539854));
#84785=CARTESIAN_POINT('Ctrl Pts',(-8.88888491832562,13.6947338741484,2.54657928927878));
#84786=CARTESIAN_POINT('Ctrl Pts',(-8.88889726216392,13.6947349100925,2.54656490341523));
#84787=CARTESIAN_POINT('Ctrl Pts',(-8.88890960627894,13.6947359460517,2.54655051780791));
#84788=CARTESIAN_POINT('Ctrl Pts',(-8.92169834615637,13.6974876861723,2.50833911620758));
#84789=CARTESIAN_POINT('Ctrl Pts',(-8.9565677002468,13.7003535294571,2.4717973217811));
#84790=CARTESIAN_POINT('Ctrl Pts',(-8.99330384693746,13.7032733772355,2.43713445424665));
#84791=CARTESIAN_POINT('Ctrl Pts',(-8.99673080379003,13.703545757255,2.43390090467414));
#84792=CARTESIAN_POINT('Ctrl Pts',(-9.00017396903045,13.7038186072335,2.43068371265036));
#84793=CARTESIAN_POINT('Ctrl Pts',(-9.00363314629963,13.7040918783833,2.42748305164184));
#84794=CARTESIAN_POINT('Ctrl Pts',(-9.04410156576257,13.7072888384287,2.39003897688877));
#84795=CARTESIAN_POINT('Ctrl Pts',(-9.08676704561797,13.7105428120646,2.35485586819792));
#84796=CARTESIAN_POINT('Ctrl Pts',(-9.13132804186191,13.7137888296548,2.32216441714941));
#84797=CARTESIAN_POINT('Ctrl Pts',(-9.1758447733736,13.7170316228086,2.28950544020269));
#84798=CARTESIAN_POINT('Ctrl Pts',(-9.22225309481509,13.7202661384793,2.25933284974102));
#84799=CARTESIAN_POINT('Ctrl Pts',(-9.27023617413474,13.7234478790248,2.23184096100257));
#84800=CARTESIAN_POINT('Ctrl Pts',(-9.31819053906954,13.72662771553,2.20436552416102));
#84801=CARTESIAN_POINT('Ctrl Pts',(-9.36771772897977,13.7297547023749,2.17956745466027));
#84802=CARTESIAN_POINT('Ctrl Pts',(-9.41848677567056,13.7328081680564,2.15760840596674));
#84803=CARTESIAN_POINT('Ctrl Pts',(-9.46924548951519,13.7358610122767,2.13565382652143));
#84804=CARTESIAN_POINT('Ctrl Pts',(-9.52124554430092,13.7388403670468,2.11653714951301));
#84805=CARTESIAN_POINT('Ctrl Pts',(-9.57414187350395,13.7417503029817,2.10038825685897));
#84806=CARTESIAN_POINT('Ctrl Pts',(-9.62708678578948,13.7446629115721,2.08422453211741));
#84807=CARTESIAN_POINT('Ctrl Pts',(-9.68092962567542,13.7475061000111,2.07103423323377));
#84808=CARTESIAN_POINT('Ctrl Pts',(-9.7353100624131,13.7503077856434,2.06091417345501));
#84809=CARTESIAN_POINT('Ctrl Pts',(-9.78971504058485,13.753110735653,2.05078954657831));
#84810=CARTESIAN_POINT('Ctrl Pts',(-9.84465809458332,13.7558724357173,2.04373828028838));
#84811=CARTESIAN_POINT('Ctrl Pts',(-9.89976404808854,13.7586416089291,2.03981988639053));
#84812=CARTESIAN_POINT('Ctrl Pts',(-9.95497449508993,13.7614160331269,2.03589406232132));
#84813=CARTESIAN_POINT('Ctrl Pts',(-10.0103483599692,13.7641984746339,2.03511356918302));
#84814=CARTESIAN_POINT('Ctrl Pts',(-10.0654945829337,13.7670528007821,2.03749383091482));
#84815=CARTESIAN_POINT('Ctrl Pts',(-10.1086033050148,13.7692840751295,2.03935452120257));
#84816=CARTESIAN_POINT('Ctrl Pts',(-10.1515725545089,13.7715597302384,2.0431459448033));
#84817=CARTESIAN_POINT('Ctrl Pts',(-10.1942109485973,13.7739127461963,2.0488527094524));
#84818=CARTESIAN_POINT('Ctrl Pts',(-10.1942293142312,13.7739137597107,2.04885516752692));
#84819=CARTESIAN_POINT('Ctrl Pts',(-10.1942476798041,13.7739147732396,2.04885762595655));
#84820=CARTESIAN_POINT('Ctrl Pts',(-10.194266045316,13.7739157867827,2.04886008474125));
#84821=CARTESIAN_POINT('Ctrl Pts',(-10.2442097744667,13.7766720468016,2.05554657832052));
#84822=CARTESIAN_POINT('Ctrl Pts',(-10.2938863219672,13.7795417787078,2.06489100340673));
#84823=CARTESIAN_POINT('Ctrl Pts',(-10.3430031029192,13.7824648329367,2.07682795496787));
#84824=CARTESIAN_POINT('Ctrl Pts',(-10.3475396640703,13.7827348142751,2.07793048468714));
#84825=CARTESIAN_POINT('Ctrl Pts',(-10.3520714246654,13.7830052504997,2.07905510426859));
#84826=CARTESIAN_POINT('Ctrl Pts',(-10.3565981392177,13.7832760942166,2.08020174555158));
#84827=CARTESIAN_POINT('Ctrl Pts',(-10.4100398314226,13.7864736332674,2.09373881527563));
#84828=CARTESIAN_POINT('Ctrl Pts',(-10.4627825400434,13.7897273418425,2.11034907458777));
#84829=CARTESIAN_POINT('Ctrl Pts',(-10.5144686863502,13.7929724463404,2.12990545839473));
#84830=CARTESIAN_POINT('Ctrl Pts',(-10.5661036608873,13.7962143380289,2.14944248044155));
#84831=CARTESIAN_POINT('Ctrl Pts',(-10.6166843450709,13.7994473075797,2.17191948587805));
#84832=CARTESIAN_POINT('Ctrl Pts',(-10.6658752612794,13.8026270766391,2.19717677960584));
#84833=CARTESIAN_POINT('Ctrl Pts',(-10.7150369120028,13.805804953937,2.22241904684071));
#84834=CARTESIAN_POINT('Ctrl Pts',(-10.7628105260939,13.8089295576144,2.25043818611738));
#84835=CARTESIAN_POINT('Ctrl Pts',(-10.8088802671553,13.8119804340562,2.28104483930439));
#84836=CARTESIAN_POINT('Ctrl Pts',(-10.8549408012514,13.8150307007851,2.31164537579989));
#84837=CARTESIAN_POINT('Ctrl Pts',(-10.8992981051754,13.8180072724059,2.34483240405891));
#84838=CARTESIAN_POINT('Ctrl Pts',(-10.9416552807271,13.8209144210495,2.38038740919537));
#84839=CARTESIAN_POINT('Ctrl Pts',(-10.9840516323039,13.8238242585062,2.41597529904989));
#84840=CARTESIAN_POINT('Ctrl Pts',(-11.0244439990362,13.8266646716509,2.45393565561274));
#84841=CARTESIAN_POINT('Ctrl Pts',(-11.0625548888345,13.829463751375,2.49401911485619));
#84842=CARTESIAN_POINT('Ctrl Pts',(-11.1006831095188,13.8322641039775,2.53412080200948));
#84843=CARTESIAN_POINT('Ctrl Pts',(-11.1365274799243,13.8350233770792,2.57634770869379));
#84844=CARTESIAN_POINT('Ctrl Pts',(-11.1698337107885,13.8377904239016,2.62041766331957));
#84845=CARTESIAN_POINT('Ctrl Pts',(-11.2032033178711,13.840562735954,2.66457147573996));
#84846=CARTESIAN_POINT('Ctrl Pts',(-11.2340245862339,13.8433433687054,2.71057558109447));
#84847=CARTESIAN_POINT('Ctrl Pts',(-11.2620715734637,13.8461962565836,2.75811042793408));
#84848=CARTESIAN_POINT('Ctrl Pts',(-11.2840139973899,13.8484281995272,2.795299083959));
#84849=CARTESIAN_POINT('Ctrl Pts',(-11.3042588076683,13.8507048203907,2.83342394002852));
#84850=CARTESIAN_POINT('Ctrl Pts',(-11.3227144771106,13.8530591735347,2.87231568712075));
#84851=CARTESIAN_POINT('Ctrl Pts',(-11.3227224883573,13.8530601955135,2.87233256927086));
#84852=CARTESIAN_POINT('Ctrl Pts',(-11.3227304992674,13.853061217507,2.87234945156567));
#84853=CARTESIAN_POINT('Ctrl Pts',(-11.3227385098408,13.8530622395152,2.87236633400517));
#84854=CARTESIAN_POINT('Ctrl Pts',(-11.3451309243512,13.8559191174301,2.91955878397471));
#84855=CARTESIAN_POINT('Ctrl Pts',(-11.3649563316523,13.8588965713256,2.96803084211943));
#84856=CARTESIAN_POINT('Ctrl Pts',(-11.3821167642417,13.8619287665913,3.01749211161235));
#84857=CARTESIAN_POINT('Ctrl Pts',(-11.3844554623751,13.8623420073048,3.02423290780344));
#84858=CARTESIAN_POINT('Ctrl Pts',(-11.3867446659438,13.8627562647528,3.03099199785369));
#84859=CARTESIAN_POINT('Ctrl Pts',(-11.3889841324662,13.8631713722903,3.03776857201318));
#84860=CARTESIAN_POINT('Ctrl Pts',(-11.4076065058816,13.8666232156173,3.09411944540883));
#84861=CARTESIAN_POINT('Ctrl Pts',(-11.4227902001525,13.8701330513621,3.15168650924206));
#84862=CARTESIAN_POINT('Ctrl Pts',(-11.4344372945637,13.8736242312343,3.21004616268316));
#84863=CARTESIAN_POINT('Ctrl Pts',(-11.4460380654213,13.8771015257672,3.26817370445484));
#84864=CARTESIAN_POINT('Ctrl Pts',(-11.4541308043979,13.8805599316602,3.32708788606901));
#84865=CARTESIAN_POINT('Ctrl Pts',(-11.4586520317584,13.8839512986877,3.38637061734034));
#84866=CARTESIAN_POINT('Ctrl Pts',(-11.4615197102294,13.886102340747,3.42397186996851));
#84867=CARTESIAN_POINT('Ctrl Pts',(-11.4629511893303,13.8882270014167,3.46172138259162));
#84868=CARTESIAN_POINT('Ctrl Pts',(-11.4629363565808,13.890319544931,3.49951158075118));
#84869=CARTESIAN_POINT('Origin',(-10.,13.2,3.5));
#84870=CARTESIAN_POINT('',(-11.4635,14.4604121156607,3.50000000573507));
#84871=CARTESIAN_POINT('',(-11.4635,14.3893209889657,3.49999999993469));
#84872=CARTESIAN_POINT('',(-11.4635,13.2,3.5));
#84873=CARTESIAN_POINT('Ctrl Pts',(-11.4635,14.4604121156607,3.50000000573456));
#84874=CARTESIAN_POINT('Ctrl Pts',(-11.4635000000723,14.4593041116426,3.48153842462835));
#84875=CARTESIAN_POINT('Ctrl Pts',(-11.4631506697053,14.458199281557,3.46307658818486));
#84876=CARTESIAN_POINT('Ctrl Pts',(-11.4593750689781,14.4522573821589,3.36336413420576));
#84877=CARTESIAN_POINT('Ctrl Pts',(-11.4495305890919,14.4475406793002,3.28249266876787));
#84878=CARTESIAN_POINT('Ctrl Pts',(-11.4306966054332,14.4424045849979,3.19166596886317));
#84879=CARTESIAN_POINT('Ctrl Pts',(-11.4282471587374,14.4417764267522,3.18051179128755));
#84880=CARTESIAN_POINT('Ctrl Pts',(-11.4243039418189,14.4408226099513,3.16350786520779));
#84881=CARTESIAN_POINT('Ctrl Pts',(-11.4229041527754,14.4404939788765,3.15763696315542));
#84882=CARTESIAN_POINT('Ctrl Pts',(-11.4202855199202,14.4398968440649,3.14694760675266));
#84883=CARTESIAN_POINT('Ctrl Pts',(-11.4190783767436,14.4396279717479,3.14212640223678));
#84884=CARTESIAN_POINT('Ctrl Pts',(-11.4164112600126,14.4390474464297,3.13169993002671));
#84885=CARTESIAN_POINT('Ctrl Pts',(-11.4149425184964,14.4387360790542,3.12609697820713));
#84886=CARTESIAN_POINT('Ctrl Pts',(-11.4108455316339,14.4378896327043,3.11083771440092));
#84887=CARTESIAN_POINT('Ctrl Pts',(-11.4081514169898,14.437356672603,3.10119930773066));
#84888=CARTESIAN_POINT('Ctrl Pts',(-11.3940034093553,14.4346723632037,3.05251543149943));
#84889=CARTESIAN_POINT('Ctrl Pts',(-11.381023052222,14.4325707387485,3.01393039613512));
#84890=CARTESIAN_POINT('Ctrl Pts',(-11.3614207471332,14.429798355418,2.96281930929373));
#84891=CARTESIAN_POINT('Ctrl Pts',(-11.3562023154256,14.4290918920926,2.9497774653871));
#84892=CARTESIAN_POINT('Ctrl Pts',(-11.312271596917,14.4233842111193,2.84441027958009));
#84893=CARTESIAN_POINT('Ctrl Pts',(-11.2643688016554,14.4186275547095,2.75620865429596));
#84894=CARTESIAN_POINT('Ctrl Pts',(-11.1779740760711,14.4110757507415,2.62993879687574));
#84895=CARTESIAN_POINT('Ctrl Pts',(-11.1457674738151,14.4084146233724,2.58794447189866));
#84896=CARTESIAN_POINT('Ctrl Pts',(-11.1046319578082,14.4050700608973,2.53993359604392));
#84897=CARTESIAN_POINT('Ctrl Pts',(-11.0978183953659,14.404517680338,2.53214979417164));
#84898=CARTESIAN_POINT('Ctrl Pts',(-11.0881965508677,14.4037387819038,2.52139014577647));
#84899=CARTESIAN_POINT('Ctrl Pts',(-11.0854572798457,14.4035171625098,2.5183526738616));
#84900=CARTESIAN_POINT('Ctrl Pts',(-11.0807757792988,14.4031385439883,2.51320509243872));
#84901=CARTESIAN_POINT('Ctrl Pts',(-11.0788399906273,14.4029820250326,2.51108910956974));
#84902=CARTESIAN_POINT('Ctrl Pts',(-11.0751141359171,14.4026808144987,2.50704039131262));
#84903=CARTESIAN_POINT('Ctrl Pts',(-11.0733250565243,14.4025362010696,2.50510678334688));
#84904=CARTESIAN_POINT('Ctrl Pts',(-11.0685520457656,14.4021504766622,2.49997604976387));
#84905=CARTESIAN_POINT('Ctrl Pts',(-11.065559012149,14.4019086852552,2.49678747706412));
#84906=CARTESIAN_POINT('Ctrl Pts',(-11.0547640675646,14.4010370882455,2.48539009139971));
#84907=CARTESIAN_POINT('Ctrl Pts',(-11.046881426683,14.4004015089416,2.4772586997586));
#84908=CARTESIAN_POINT('Ctrl Pts',(-10.9849167805197,14.3954179257212,2.41480560462796));
#84909=CARTESIAN_POINT('Ctrl Pts',(-10.9267410402003,14.390818790509,2.3647216474997));
#84910=CARTESIAN_POINT('Ctrl Pts',(-10.813409908893,14.382359907193,2.28169232073399));
#84911=CARTESIAN_POINT('Ctrl Pts',(-10.7594852277375,14.3785129710107,2.24736587046793));
#84912=CARTESIAN_POINT('Ctrl Pts',(-10.6522677466764,14.3713144477356,2.18859197029449));
#84913=CARTESIAN_POINT('Ctrl Pts',(-10.5994074769879,14.3679545248946,2.16360327873566));
#84914=CARTESIAN_POINT('Ctrl Pts',(-10.5316946259927,14.3638918354729,2.13642215873947));
#84915=CARTESIAN_POINT('Ctrl Pts',(-10.5181195003967,14.3630888227772,2.1312064037073));
#84916=CARTESIAN_POINT('Ctrl Pts',(-10.4982265693755,14.3619283884958,2.12390162001956));
#84917=CARTESIAN_POINT('Ctrl Pts',(-10.4919689813092,14.3615656815066,2.12165207973847));
#84918=CARTESIAN_POINT('Ctrl Pts',(-10.4809471897867,14.3609308432514,2.11777447743404));
#84919=CARTESIAN_POINT('Ctrl Pts',(-10.4761895443317,14.3606581166207,2.11612821643571));
#84920=CARTESIAN_POINT('Ctrl Pts',(-10.4662884453787,14.3600932220642,2.11275930104501));
#84921=CARTESIAN_POINT('Ctrl Pts',(-10.4611437132677,14.3598011878942,2.11104062408813));
#84922=CARTESIAN_POINT('Ctrl Pts',(-10.4478121336516,14.3590482286469,2.10666924179509));
#84923=CARTESIAN_POINT('Ctrl Pts',(-10.439611165235,14.3585887263669,2.10406005269817));
#84924=CARTESIAN_POINT('Ctrl Pts',(-10.4067988717358,14.3567644649578,2.09393845776422));
#84925=CARTESIAN_POINT('Ctrl Pts',(-10.382013560085,14.3554183583217,2.08700313939953));
#84926=CARTESIAN_POINT('Ctrl Pts',(-10.2012158785516,14.3458001169739,2.04151857700132));
#84927=CARTESIAN_POINT('Ctrl Pts',(-10.040010019301,14.3384410370629,2.02825113933093));
#84928=CARTESIAN_POINT('Ctrl Pts',(-9.84889906581922,14.328685004098,2.04398917552953));
#84929=CARTESIAN_POINT('Ctrl Pts',(-9.81800246202222,14.3270703464246,2.04752774949459));
#84930=CARTESIAN_POINT('Ctrl Pts',(-9.78133457163267,14.3250851291321,2.05291556606619));
#84931=CARTESIAN_POINT('Ctrl Pts',(-9.7754303517248,14.3247633253456,2.05382006682907));
#84932=CARTESIAN_POINT('Ctrl Pts',(-9.76629517217275,14.3242618679235,2.05527682703097));
#84933=CARTESIAN_POINT('Ctrl Pts',(-9.76306018316681,14.3240835981042,2.05580385133066));
#84934=CARTESIAN_POINT('Ctrl Pts',(-9.75707903677028,14.323752671754,2.05679889964672));
#84935=CARTESIAN_POINT('Ctrl Pts',(-9.75433243001706,14.3236001854758,2.05726389969384));
#84936=CARTESIAN_POINT('Ctrl Pts',(-9.74812293381212,14.3232542711549,2.05833341218179));
#84937=CARTESIAN_POINT('Ctrl Pts',(-9.74466090271375,14.3230605871653,2.0589425577836));
#84938=CARTESIAN_POINT('Ctrl Pts',(-9.73419980421892,14.3224729178724,2.06082207252783));
#84939=CARTESIAN_POINT('Ctrl Pts',(-9.72720787881597,14.3220768539564,2.06213098460307));
#84940=CARTESIAN_POINT('Ctrl Pts',(-9.63917112801196,14.3170509184235,2.07927699437777));
#84941=CARTESIAN_POINT('Ctrl Pts',(-9.55960573488289,14.3120988818137,2.1018936082228));
#84942=CARTESIAN_POINT('Ctrl Pts',(-9.43248107653116,14.3039162305376,2.14996276278858));
#84943=CARTESIAN_POINT('Ctrl Pts',(-9.38364848795247,14.3007006231604,2.17154621806499));
#84944=CARTESIAN_POINT('Ctrl Pts',(-9.27582037802258,14.2935248006285,2.22643350815974));
#84945=CARTESIAN_POINT('Ctrl Pts',(-9.21773281225691,14.289606747387,2.2612636563679));
#84946=CARTESIAN_POINT('Ctrl Pts',(-9.14938252960827,14.284956436793,2.308979971233));
#84947=CARTESIAN_POINT('Ctrl Pts',(-9.13665303863318,14.2840882342111,2.31817478400478));
#84948=CARTESIAN_POINT('Ctrl Pts',(-9.11857968692033,14.2828520658595,2.33167747931422));
#84949=CARTESIAN_POINT('Ctrl Pts',(-9.1131146053878,14.2824777971522,2.3358206410879));
#84950=CARTESIAN_POINT('Ctrl Pts',(-9.1036620244799,14.2818295638375,2.34309198064149));
#84951=CARTESIAN_POINT('Ctrl Pts',(-9.0996613084195,14.281554925281,2.3462027158307));
#84952=CARTESIAN_POINT('Ctrl Pts',(-9.09197729478612,14.2810268637449,2.35224168197554));
#84953=CARTESIAN_POINT('Ctrl Pts',(-9.08829180814358,14.2807733315566,2.35516701506633));
#84954=CARTESIAN_POINT('Ctrl Pts',(-9.07959407567654,14.2801743476316,2.36213942657337));
#84955=CARTESIAN_POINT('Ctrl Pts',(-9.07459429367989,14.2798295139788,2.36620194452444));
#84956=CARTESIAN_POINT('Ctrl Pts',(-9.05704701702705,14.2786172998891,2.38065319013408));
#84957=CARTESIAN_POINT('Ctrl Pts',(-9.0446460575153,14.2777570112564,2.3912184699568));
#84958=CARTESIAN_POINT('Ctrl Pts',(-8.94219975033353,14.2706121335422,2.48149498262767));
#84959=CARTESIAN_POINT('Ctrl Pts',(-8.8621202607452,14.2648278457553,2.57181574140944));
#84960=CARTESIAN_POINT('Ctrl Pts',(-8.76104575217004,14.2561345912015,2.71884301775442));
#84961=CARTESIAN_POINT('Ctrl Pts',(-8.73099024637538,14.2532817982974,2.76868119677067));
#84962=CARTESIAN_POINT('Ctrl Pts',(-8.691768093299,14.2489538794105,2.8434539025698));
#84963=CARTESIAN_POINT('Ctrl Pts',(-8.68018540558855,14.2475807272606,2.86706021964633));
#84964=CARTESIAN_POINT('Ctrl Pts',(-8.66687557727843,14.2458658947284,2.89614243831849));
#84965=CARTESIAN_POINT('Ctrl Pts',(-8.66453595075689,14.245558865472,2.90133444036668));
#84966=CARTESIAN_POINT('Ctrl Pts',(-8.66092215901931,14.2450755645916,2.90948062211416));
#84967=CARTESIAN_POINT('Ctrl Pts',(-8.65962730586755,14.2449005210417,2.91242563000101));
#84968=CARTESIAN_POINT('Ctrl Pts',(-8.65722659710088,14.2445724165034,2.9179350229826));
#84969=CARTESIAN_POINT('Ctrl Pts',(-8.65611836551723,14.2444195009755,2.9204983165843));
#84970=CARTESIAN_POINT('Ctrl Pts',(-8.65359824961482,14.244068431326,2.92637334657593));
#84971=CARTESIAN_POINT('Ctrl Pts',(-8.65219124804487,14.2438699886391,2.92968712223823));
#84972=CARTESIAN_POINT('Ctrl Pts',(-8.64853515355139,14.2433479558743,2.93838706551633));
#84973=CARTESIAN_POINT('Ctrl Pts',(-8.64630605418791,14.2430232221022,2.94378150145911));
#84974=CARTESIAN_POINT('Ctrl Pts',(-8.63120570142131,14.2407791398923,2.98095292475122));
#84975=CARTESIAN_POINT('Ctrl Pts',(-8.61942319928684,14.2388028061162,3.01315810216131));
#84976=CARTESIAN_POINT('Ctrl Pts',(-8.57994651878173,14.2313411382223,3.13406060561002));
#84977=CARTESIAN_POINT('Ctrl Pts',(-8.55958516690778,14.2256660998844,3.22492048356303));
#84978=CARTESIAN_POINT('Ctrl Pts',(-8.53747870968423,14.2151179001388,3.40041897465775));
#84979=CARTESIAN_POINT('Ctrl Pts',(-8.53417314536208,14.2102385235977,3.4844989329429));
#84980=CARTESIAN_POINT('Ctrl Pts',(-8.53863613806729,14.2049513135456,3.57987238998724));
#84981=CARTESIAN_POINT('Ctrl Pts',(-8.5393073571228,14.2043200220066,3.5913287974092));
#84982=CARTESIAN_POINT('Ctrl Pts',(-8.54053792892943,14.2033624602404,3.60880845367943));
#84983=CARTESIAN_POINT('Ctrl Pts',(-8.54099997587137,14.2030331813313,3.61483791887953));
#84984=CARTESIAN_POINT('Ctrl Pts',(-8.5419098691852,14.2024353712951,3.62581782556946));
#84985=CARTESIAN_POINT('Ctrl Pts',(-8.54234558864907,14.2021664672428,3.63076915815563));
#84986=CARTESIAN_POINT('Ctrl Pts',(-8.54334274581042,14.2015864358263,3.64147553885085));
#84987=CARTESIAN_POINT('Ctrl Pts',(-8.54391308471256,14.2012755903013,3.64722968695282));
#84988=CARTESIAN_POINT('Ctrl Pts',(-8.54555909817605,14.2004319464622,3.66289015307856));
#84989=CARTESIAN_POINT('Ctrl Pts',(-8.54670187663079,14.1999012434357,3.67278920700273));
#84990=CARTESIAN_POINT('Ctrl Pts',(-8.55295386310655,14.1972490157889,3.72248497802612));
#84991=CARTESIAN_POINT('Ctrl Pts',(-8.5595972268523,14.1951757575384,3.76207310117166));
#84992=CARTESIAN_POINT('Ctrl Pts',(-8.57074962514721,14.1924309214968,3.81507557120897));
#84993=CARTESIAN_POINT('Ctrl Pts',(-8.57383710547414,14.1917245635973,3.82876839979471));
#84994=CARTESIAN_POINT('Ctrl Pts',(-8.60074421906827,14.1859714656528,3.94057884016097));
#84995=CARTESIAN_POINT('Ctrl Pts',(-8.63446083964771,14.1811758330106,4.03603044944025));
#84996=CARTESIAN_POINT('Ctrl Pts',(-8.70032732407648,14.173589203107,4.17487939151635));
#84997=CARTESIAN_POINT('Ctrl Pts',(-8.7254762972443,14.1709362075542,4.22124861622847));
#84998=CARTESIAN_POINT('Ctrl Pts',(-8.75847528992601,14.1676015012024,4.27495503357835));
#84999=CARTESIAN_POINT('Ctrl Pts',(-8.76397473460302,14.1670500146294,4.28369665117282));
#85000=CARTESIAN_POINT('Ctrl Pts',(-8.77177917179701,14.1662721731516,4.29581565388331));
#85001=CARTESIAN_POINT('Ctrl Pts',(-8.77400662646717,14.1660506992169,4.29924289489074));
#85002=CARTESIAN_POINT('Ctrl Pts',(-8.7778209710577,14.1656722564136,4.3050583163535));
#85003=CARTESIAN_POINT('Ctrl Pts',(-8.77940059498354,14.1655157666566,4.30745127646895));
#85004=CARTESIAN_POINT('Ctrl Pts',(-8.78244527250804,14.165214554503,4.31203428387048));
#85005=CARTESIAN_POINT('Ctrl Pts',(-8.78390921989145,14.165069909931,4.31422503457328));
#85006=CARTESIAN_POINT('Ctrl Pts',(-8.78782036820243,14.16468398684,4.32004386596956));
#85007=CARTESIAN_POINT('Ctrl Pts',(-8.79027792011034,14.1644420265999,4.32366491383094));
#85008=CARTESIAN_POINT('Ctrl Pts',(-8.79916403914265,14.1635691984649,4.33663249379929));
#85009=CARTESIAN_POINT('Ctrl Pts',(-8.80568481958957,14.1629325359026,4.34591498877244));
#85010=CARTESIAN_POINT('Ctrl Pts',(-8.85927799269935,14.157736591395,4.42035120979246));
#85011=CARTESIAN_POINT('Ctrl Pts',(-8.91153357123456,14.1529018032807,4.48159650099979));
#85012=CARTESIAN_POINT('Ctrl Pts',(-9.02020076115273,14.1436770663582,4.58955370693775));
#85013=CARTESIAN_POINT('Ctrl Pts',(-9.07561640786214,14.139300727543,4.63694779045571));
#85014=CARTESIAN_POINT('Ctrl Pts',(-9.16222252812138,14.1330397108026,4.70048223279547));
#85015=CARTESIAN_POINT('Ctrl Pts',(-9.19083006085732,14.1310538033954,4.71994793299115));
#85016=CARTESIAN_POINT('Ctrl Pts',(-9.23887587363222,14.1278533088287,4.75020580317848));
#85017=CARTESIAN_POINT('Ctrl Pts',(-9.25791662228319,14.1266178564323,4.76160089664236));
#85018=CARTESIAN_POINT('Ctrl Pts',(-9.28426967129974,14.1249515490318,4.77656894295486));
#85019=CARTESIAN_POINT('Ctrl Pts',(-9.29136281270442,14.124507258797,4.7805200154813));
#85020=CARTESIAN_POINT('Ctrl Pts',(-9.30268925421853,14.1238043842731,4.7867062148745));
#85021=CARTESIAN_POINT('Ctrl Pts',(-9.30690120376539,14.1235444379114,4.78897991411648));
#85022=CARTESIAN_POINT('Ctrl Pts',(-9.31555654150454,14.1230131585737,4.79359755667895));
#85023=CARTESIAN_POINT('Ctrl Pts',(-9.32000099905483,14.122741903112,4.79593936822146));
#85024=CARTESIAN_POINT('Ctrl Pts',(-9.3302909592772,14.1221174183178,4.80129370023385));
#85025=CARTESIAN_POINT('Ctrl Pts',(-9.33614490914258,14.1217647659493,4.80428981202847));
#85026=CARTESIAN_POINT('Ctrl Pts',(-9.35465419980878,14.1206578072834,4.81360616054434));
#85027=CARTESIAN_POINT('Ctrl Pts',(-9.36738129726038,14.1199084800202,4.81978253598129));
#85028=CARTESIAN_POINT('Ctrl Pts',(-9.43041675037628,14.1162522247754,4.84925182961821));
#85029=CARTESIAN_POINT('Ctrl Pts',(-9.48193329907797,14.1134371534019,4.86985886809654));
#85030=CARTESIAN_POINT('Ctrl Pts',(-9.63117826927043,14.1056128422882,4.91993018253081));
#85031=CARTESIAN_POINT('Ctrl Pts',(-9.73097715768316,14.1007816779589,4.94217076653062));
#85032=CARTESIAN_POINT('Ctrl Pts',(-9.84580858331721,14.0950306734715,4.95541845802973));
#85033=CARTESIAN_POINT('Ctrl Pts',(-9.85936435064441,14.094348422177,4.95679081582959));
#85034=CARTESIAN_POINT('Ctrl Pts',(-9.90854990123835,14.0918548999297,4.96107735538652));
#85035=CARTESIAN_POINT('Ctrl Pts',(-9.94426186570979,14.0900102745399,4.96287491830589));
#85036=CARTESIAN_POINT('Ctrl Pts',(-9.9859160960748,14.0877831684182,4.96344418748409));
#85037=CARTESIAN_POINT('Ctrl Pts',(-9.99183164097463,14.0874651081145,4.96348916011669));
#85038=CARTESIAN_POINT('Ctrl Pts',(-10.0013323907847,14.0869512015507,4.96350378489108));
#85039=CARTESIAN_POINT('Ctrl Pts',(-10.0049175553373,14.0867565712009,4.96349612939262));
#85040=CARTESIAN_POINT('Ctrl Pts',(-10.011300111432,14.086408766205,4.96345904750473));
#85041=CARTESIAN_POINT('Ctrl Pts',(-10.0140974866146,14.0862558784797,4.96343477374512));
#85042=CARTESIAN_POINT('Ctrl Pts',(-10.0200833735656,14.0859277446791,4.96336566732801));
#85043=CARTESIAN_POINT('Ctrl Pts',(-10.0232717637088,14.0857523731999,4.96331843520849));
#85044=CARTESIAN_POINT('Ctrl Pts',(-10.0320239643193,14.0852694011451,4.96316017037511));
#85045=CARTESIAN_POINT('Ctrl Pts',(-10.0375872760037,14.0849606554884,4.96302782376296));
#85046=CARTESIAN_POINT('Ctrl Pts',(-10.0674965618524,14.0832918933654,4.96214559951987));
#85047=CARTESIAN_POINT('Ctrl Pts',(-10.0918203738008,14.0819031115467,4.96081977528727));
#85048=CARTESIAN_POINT('Ctrl Pts',(-10.1671359390982,14.0775276505674,4.95482616566594));
#85049=CARTESIAN_POINT('Ctrl Pts',(-10.217922462486,14.0744708450747,4.94808935210492));
#85050=CARTESIAN_POINT('Ctrl Pts',(-10.3969462058607,14.0635248014939,4.91471019988736));
#85051=CARTESIAN_POINT('Ctrl Pts',(-10.5218715913884,14.0556387861717,4.87354798843426));
#85052=CARTESIAN_POINT('Ctrl Pts',(-10.6533726533742,14.0474842713034,4.80964450075971));
#85053=CARTESIAN_POINT('Ctrl Pts',(-10.6669763424547,14.0466415041869,4.80276902244779));
#85054=CARTESIAN_POINT('Ctrl Pts',(-10.6860154999664,14.0454628042309,4.79276997609644));
#85055=CARTESIAN_POINT('Ctrl Pts',(-10.6915417865954,14.0451207705642,4.78982224992127));
#85056=CARTESIAN_POINT('Ctrl Pts',(-10.7011469979569,14.0445264032371,4.78461934356134));
#85057=CARTESIAN_POINT('Ctrl Pts',(-10.7052343606598,14.0442735165954,4.78238000134131));
#85058=CARTESIAN_POINT('Ctrl Pts',(-10.7137746384088,14.0437451797012,4.77764786107218));
#85059=CARTESIAN_POINT('Ctrl Pts',(-10.7182253585414,14.0434698703348,4.77515121714888));
#85060=CARTESIAN_POINT('Ctrl Pts',(-10.7288002525965,14.0428157644681,4.76914626961165));
#85061=CARTESIAN_POINT('Ctrl Pts',(-10.7349123175732,14.042437728101,4.7656168257832));
#85062=CARTESIAN_POINT('Ctrl Pts',(-10.7555463406542,14.0411613810557,4.75350172289471));
#85063=CARTESIAN_POINT('Ctrl Pts',(-10.7699455910349,14.040270518108,4.74470906642126));
#85064=CARTESIAN_POINT('Ctrl Pts',(-10.8040071821918,14.0381604219844,4.7230926336885));
#85065=CARTESIAN_POINT('Ctrl Pts',(-10.823519553052,14.0369494307768,4.71004080914583));
#85066=CARTESIAN_POINT('Ctrl Pts',(-10.9373481063402,14.0298510092092,4.62987156839359));
#85067=CARTESIAN_POINT('Ctrl Pts',(-11.023739952332,14.024361667009,4.552229863221));
#85068=CARTESIAN_POINT('Ctrl Pts',(-11.1413359322687,14.0155933574891,4.41820311469097));
#85069=CARTESIAN_POINT('Ctrl Pts',(-11.1795280376052,14.0124578945094,4.36859459021663));
#85070=CARTESIAN_POINT('Ctrl Pts',(-11.2184677304692,14.0087352368312,4.31069174116087));
#85071=CARTESIAN_POINT('Ctrl Pts',(-11.2224648458871,14.0083461749696,4.30465172940805));
#85072=CARTESIAN_POINT('Ctrl Pts',(-11.2283491213237,14.0077625971509,4.29561499816345));
#85073=CARTESIAN_POINT('Ctrl Pts',(-11.2302705649923,14.007570278141,4.29264060300603));
#85074=CARTESIAN_POINT('Ctrl Pts',(-11.2336851923166,14.007225290817,4.28731243232751));
#85075=CARTESIAN_POINT('Ctrl Pts',(-11.2351824645837,14.0070728948977,4.2849613359059));
#85076=CARTESIAN_POINT('Ctrl Pts',(-11.2384151521333,14.0067414044978,4.27985304665037));
#85077=CARTESIAN_POINT('Ctrl Pts',(-11.2401480564084,14.0065621557493,4.27709437082169));
#85078=CARTESIAN_POINT('Ctrl Pts',(-11.2449842294291,14.0060575873514,4.26933810823639));
#85079=CARTESIAN_POINT('Ctrl Pts',(-11.2480665611999,14.0057309504855,4.26432762132821));
#85080=CARTESIAN_POINT('Ctrl Pts',(-11.2663870047416,14.003759559667,4.2341404967701));
#85081=CARTESIAN_POINT('Ctrl Pts',(-11.2808921145457,14.0020726540537,4.20852908496264));
#85082=CARTESIAN_POINT('Ctrl Pts',(-11.3570099687491,13.9925563484428,4.06414330473809));
#85083=CARTESIAN_POINT('Ctrl Pts',(-11.4028839154276,13.9842775844866,3.93778639184374));
#85084=CARTESIAN_POINT('Ctrl Pts',(-11.4414821788112,13.9735635673457,3.7578430097127));
#85085=CARTESIAN_POINT('Ctrl Pts',(-11.4494808128266,13.9707064496622,3.70823090366372));
#85086=CARTESIAN_POINT('Ctrl Pts',(-11.4559646310173,13.9673914050103,3.64863948814271));
#85087=CARTESIAN_POINT('Ctrl Pts',(-11.4569196210957,13.9668569242536,3.63896736410953));
#85088=CARTESIAN_POINT('Ctrl Pts',(-11.4583294345449,13.9659842211894,3.62307089487082));
#85089=CARTESIAN_POINT('Ctrl Pts',(-11.4588409097876,13.9656442457038,3.61685198518387));
#85090=CARTESIAN_POINT('Ctrl Pts',(-11.4596892954621,13.9650349902647,3.60566098155111));
#85091=CARTESIAN_POINT('Ctrl Pts',(-11.4600406111535,13.9647652662042,3.60069010350523));
#85092=CARTESIAN_POINT('Ctrl Pts',(-11.4607353402448,13.9641920063239,3.59009058643531));
#85093=CARTESIAN_POINT('Ctrl Pts',(-11.4610716257979,13.9638886962335,3.58446155050797));
#85094=CARTESIAN_POINT('Ctrl Pts',(-11.4618914662117,13.9630727341222,3.56926321728734));
#85095=CARTESIAN_POINT('Ctrl Pts',(-11.4623136008877,13.9625619925752,3.55969079303546));
#85096=CARTESIAN_POINT('Ctrl Pts',(-11.4632139046721,13.9611683106935,3.53341466330243));
#85097=CARTESIAN_POINT('Ctrl Pts',(-11.4634999999312,13.9602913597298,3.51670731772259));
#85098=CARTESIAN_POINT('Ctrl Pts',(-11.4635,13.9594225818479,3.50000000603013));
#85099=CARTESIAN_POINT('Ctrl Pts',(-11.4634999124217,13.8906444325997,3.49949369805951));
#85100=CARTESIAN_POINT('Ctrl Pts',(-11.4635032710664,13.8911858909132,3.50920208713336));
#85101=CARTESIAN_POINT('Ctrl Pts',(-11.4634100262615,13.8917243994204,3.51891046394916));
#85102=CARTESIAN_POINT('Ctrl Pts',(-11.4630599651482,13.8927118813261,3.5368092430745));
#85103=CARTESIAN_POINT('Ctrl Pts',(-11.4628309580255,13.8931616918135,3.54499971198327));
#85104=CARTESIAN_POINT('Ctrl Pts',(-11.4623552135967,13.8938769137533,3.55808147343423));
#85105=CARTESIAN_POINT('Ctrl Pts',(-11.4621526902116,13.8941436923484,3.56297411859369));
#85106=CARTESIAN_POINT('Ctrl Pts',(-11.4617040830429,13.8946692244319,3.57263776807771));
#85107=CARTESIAN_POINT('Ctrl Pts',(-11.4614591871489,13.894928011513,3.57740876427155));
#85108=CARTESIAN_POINT('Ctrl Pts',(-11.4608882362896,13.8954772699635,3.58756066605114));
#85109=CARTESIAN_POINT('Ctrl Pts',(-11.4605558026249,13.8957675389846,3.59294115158493));
#85110=CARTESIAN_POINT('Ctrl Pts',(-11.4596250734639,13.8965111611674,3.60676385876572));
#85111=CARTESIAN_POINT('Ctrl Pts',(-11.4589832576214,13.8969631558713,3.61520301501556));
#85112=CARTESIAN_POINT('Ctrl Pts',(-11.456177683201,13.8987280206099,3.64829428153379));
#85113=CARTESIAN_POINT('Ctrl Pts',(-11.4534619514906,13.9000237246107,3.67289617978589));
#85114=CARTESIAN_POINT('Ctrl Pts',(-11.4336082383893,13.9076269398112,3.81873030306006));
#85115=CARTESIAN_POINT('Ctrl Pts',(-11.4019376940631,13.9134477571552,3.93748498438483));
#85116=CARTESIAN_POINT('Ctrl Pts',(-11.3377899299475,13.9217963971866,4.09535860170369));
#85117=CARTESIAN_POINT('Ctrl Pts',(-11.3175574215204,13.9241757404651,4.1388862213477));
#85118=CARTESIAN_POINT('Ctrl Pts',(-11.284335208419,13.9278510626477,4.20204169542735));
#85119=CARTESIAN_POINT('Ctrl Pts',(-11.2729504157475,13.9290771281436,4.2224794705723));
#85120=CARTESIAN_POINT('Ctrl Pts',(-11.2582943219294,13.9306267833715,4.24736725694616));
#85121=CARTESIAN_POINT('Ctrl Pts',(-11.2554806555111,13.9309230561008,4.25208426327092));
#85122=CARTESIAN_POINT('Ctrl Pts',(-11.2510007026186,13.9313930442305,4.25949953820821));
#85123=CARTESIAN_POINT('Ctrl Pts',(-11.249352054374,13.9315656380569,4.26220846907503));
#85124=CARTESIAN_POINT('Ctrl Pts',(-11.2462308447665,13.931891750029,4.26729966453415));
#85125=CARTESIAN_POINT('Ctrl Pts',(-11.2447602418358,13.9320451420336,4.26968307342567));
#85126=CARTESIAN_POINT('Ctrl Pts',(-11.2413778284302,13.9323973386053,4.27512990957486));
#85127=CARTESIAN_POINT('Ctrl Pts',(-11.2394615138154,13.9325964344036,4.27819049392208));
#85128=CARTESIAN_POINT('Ctrl Pts',(-11.2343305451963,13.9331282804365,4.28631823418877));
#85129=CARTESIAN_POINT('Ctrl Pts',(-11.2310960534466,13.9334622731247,4.2913727092182));
#85130=CARTESIAN_POINT('Ctrl Pts',(-11.2072295451169,13.9359166505887,4.32816800062603));
#85131=CARTESIAN_POINT('Ctrl Pts',(-11.185405460241,13.9381063904024,4.35911514716666));
#85132=CARTESIAN_POINT('Ctrl Pts',(-11.1061530438012,13.9457875977111,4.46272048388466));
#85133=CARTESIAN_POINT('Ctrl Pts',(-11.0430462057516,13.9514431051591,4.53075715632658));
#85134=CARTESIAN_POINT('Ctrl Pts',(-10.9231761460071,13.9610020037966,4.6376301220376));
#85135=CARTESIAN_POINT('Ctrl Pts',(-10.8693218313548,13.9649640960408,4.67929553407391));
#85136=CARTESIAN_POINT('Ctrl Pts',(-10.8015697887803,13.9695387882705,4.72454038346953));
#85137=CARTESIAN_POINT('Ctrl Pts',(-10.7902779621024,13.9702887020011,4.73185796119353));
#85138=CARTESIAN_POINT('Ctrl Pts',(-10.7723084958512,13.971462694586,4.74315413680451));
#85139=CARTESIAN_POINT('Ctrl Pts',(-10.7656975193451,13.9718905446668,4.74723691925821));
#85140=CARTESIAN_POINT('Ctrl Pts',(-10.753138277802,13.9726957864608,4.75485571390308));
#85141=CARTESIAN_POINT('Ctrl Pts',(-10.7471968583926,13.9730735640408,4.75840255296829));
#85142=CARTESIAN_POINT('Ctrl Pts',(-10.7369039082363,13.9737226624015,4.76444851905635));
#85143=CARTESIAN_POINT('Ctrl Pts',(-10.7325643033987,13.9739946998868,4.76696762767455));
#85144=CARTESIAN_POINT('Ctrl Pts',(-10.7241787170347,13.9745172714312,4.77177791058589));
#85145=CARTESIAN_POINT('Ctrl Pts',(-10.7201346097001,13.9747679153383,4.77407221642244));
#85146=CARTESIAN_POINT('Ctrl Pts',(-10.7106646635601,13.9753516683393,4.77938521835069));
#85147=CARTESIAN_POINT('Ctrl Pts',(-10.7052303885801,13.9756842366191,4.78238874823704));
#85148=CARTESIAN_POINT('Ctrl Pts',(-10.6863698495434,13.9768302803127,4.79265684254898));
#85149=CARTESIAN_POINT('Ctrl Pts',(-10.6728488964784,13.9776375945381,4.79974600155214));
#85150=CARTESIAN_POINT('Ctrl Pts',(-10.5422131558147,13.9853087273094,4.86565454267108));
#85151=CARTESIAN_POINT('Ctrl Pts',(-10.4178144227959,13.9915594092099,4.90870166175729));
#85152=CARTESIAN_POINT('Ctrl Pts',(-10.2392156905274,14.0004685511921,4.94472238624106));
#85153=CARTESIAN_POINT('Ctrl Pts',(-10.1885989004517,14.0029960243115,4.95219719251997));
#85154=CARTESIAN_POINT('Ctrl Pts',(-10.1134650391501,14.0068770226795,4.95929792903287));
#85155=CARTESIAN_POINT('Ctrl Pts',(-10.0891794962779,14.0081513906661,4.9609831075946));
#85156=CARTESIAN_POINT('Ctrl Pts',(-10.0593030301201,14.0097555814205,4.9623085835812));
#85157=CARTESIAN_POINT('Ctrl Pts',(-10.0537400927606,14.0100558291128,4.96252358730388));
#85158=CARTESIAN_POINT('Ctrl Pts',(-10.044986850254,14.0105308914473,4.96281188674444));
#85159=CARTESIAN_POINT('Ctrl Pts',(-10.0417972420909,14.0107045482622,4.96290649832834));
#85160=CARTESIAN_POINT('Ctrl Pts',(-10.0358088613235,14.0110316536179,4.96306452783837));
#85161=CARTESIAN_POINT('Ctrl Pts',(-10.033010203,14.011184968555,4.9631303473121));
#85162=CARTESIAN_POINT('Ctrl Pts',(-10.0266238685112,14.0115358213642,4.96326221005647));
#85163=CARTESIAN_POINT('Ctrl Pts',(-10.0230361319911,14.0117336408742,4.96332308866219));
#85164=CARTESIAN_POINT('Ctrl Pts',(-10.0135256133057,14.0122598616147,4.96344948377995));
#85165=CARTESIAN_POINT('Ctrl Pts',(-10.0076026573392,14.0125894649278,4.96349223809736));
#85166=CARTESIAN_POINT('Ctrl Pts',(-9.96568245246635,14.0149348095153,4.96354035136587));
#85167=CARTESIAN_POINT('Ctrl Pts',(-9.92969865646566,14.0170133029548,4.96225352223029));
#85168=CARTESIAN_POINT('Ctrl Pts',(-9.88394151331369,14.0197097919931,4.95892440558378));
#85169=CARTESIAN_POINT('Ctrl Pts',(-9.87408870873401,14.0202936117471,4.95810710666906));
#85170=CARTESIAN_POINT('Ctrl Pts',(-9.77548719422565,14.0261637115097,4.94892118096201));
#85171=CARTESIAN_POINT('Ctrl Pts',(-9.687670053473,14.0316009288096,4.9325604251217));
#85172=CARTESIAN_POINT('Ctrl Pts',(-9.53535740836338,14.0409980668464,4.88950320621494));
#85173=CARTESIAN_POINT('Ctrl Pts',(-9.47023960214507,14.0450070400785,4.86600435201072));
#85174=CARTESIAN_POINT('Ctrl Pts',(-9.39250012515686,14.0497521247001,4.83155112284302));
#85175=CARTESIAN_POINT('Ctrl Pts',(-9.37808546408041,14.0506304836527,4.82487992989306));
#85176=CARTESIAN_POINT('Ctrl Pts',(-9.35757621043408,14.0518784705054,4.81497962268128));
#85177=CARTESIAN_POINT('Ctrl Pts',(-9.35139174446376,14.0522545665639,4.81194019169793));
#85178=CARTESIAN_POINT('Ctrl Pts',(-9.34069043955313,14.0529050090987,4.806586738772));
#85179=CARTESIAN_POINT('Ctrl Pts',(-9.33616377888516,14.0531800416248,4.80429271057883));
#85180=CARTESIAN_POINT('Ctrl Pts',(-9.32746828180742,14.0537081951419,4.79982899771809));
#85181=CARTESIAN_POINT('Ctrl Pts',(-9.32329779055664,14.0539614293269,4.79766268950284));
#85182=CARTESIAN_POINT('Ctrl Pts',(-9.31345917862181,14.0545586894861,4.79249181978395));
#85183=CARTESIAN_POINT('Ctrl Pts',(-9.30780020957477,14.0549021066307,4.78946999016714));
#85184=CARTESIAN_POINT('Ctrl Pts',(-9.28798913417361,14.0561040985067,4.77872308555758));
#85185=CARTESIAN_POINT('Ctrl Pts',(-9.27394470261818,14.0569557413303,4.77080129636367));
#85186=CARTESIAN_POINT('Ctrl Pts',(-9.15456093815374,14.0641982457844,4.70083729320009));
#85187=CARTESIAN_POINT('Ctrl Pts',(-9.05725069768205,14.0700690851717,4.62605664361488));
#85188=CARTESIAN_POINT('Ctrl Pts',(-8.92997519251147,14.0787997333249,4.50005475628076));
#85189=CARTESIAN_POINT('Ctrl Pts',(-8.89195061040829,14.081591714299,4.45775168258011));
#85190=CARTESIAN_POINT('Ctrl Pts',(-8.84029492113772,14.0858366818902,4.39307858175174));
#85191=CARTESIAN_POINT('Ctrl Pts',(-8.82464786221086,14.0871921305771,4.37238317896592));
#85192=CARTESIAN_POINT('Ctrl Pts',(-8.80626008658573,14.0888871728448,4.3466696246112));
#85193=CARTESIAN_POINT('Ctrl Pts',(-8.80298708656365,14.08919304817,4.34203593573131));
#85194=CARTESIAN_POINT('Ctrl Pts',(-8.79790284446138,14.08967495651,4.33474846570885));
#85195=CARTESIAN_POINT('Ctrl Pts',(-8.79607322454802,14.0898497733384,4.33210749984603));
#85196=CARTESIAN_POINT('Ctrl Pts',(-8.79266873726176,14.0901777323262,4.3271585573484));
#85197=CARTESIAN_POINT('Ctrl Pts',(-8.79109177519245,14.0903307310507,4.32485208404071));
#85198=CARTESIAN_POINT('Ctrl Pts',(-8.78749317068819,14.0906823651433,4.31955625925411));
#85199=CARTESIAN_POINT('Ctrl Pts',(-8.7854759788767,14.0908812922157,4.3165639440667));
#85200=CARTESIAN_POINT('Ctrl Pts',(-8.78020990389279,14.0914053458062,4.30868953355507));
#85201=CARTESIAN_POINT('Ctrl Pts',(-8.77697929491117,14.0917316298276,4.30379536750177));
#85202=CARTESIAN_POINT('Ctrl Pts',(-8.75476657696193,14.0940078564958,4.26970057258097));
#85203=CARTESIAN_POINT('Ctrl Pts',(-8.73680406952355,14.0960165956496,4.23985195342664));
#85204=CARTESIAN_POINT('Ctrl Pts',(-8.6976050923087,14.1007638637677,4.16911880973339));
#85205=CARTESIAN_POINT('Ctrl Pts',(-8.67719957349552,14.1035259533372,4.12781459708676));
#85206=CARTESIAN_POINT('Ctrl Pts',(-8.60931610861705,14.1137367789869,3.97234335341583));
#85207=CARTESIAN_POINT('Ctrl Pts',(-8.57439636355503,14.1211479511917,3.85323508322942));
#85208=CARTESIAN_POINT('Ctrl Pts',(-8.55237215857691,14.1289287233202,3.71553564884653));
#85209=CARTESIAN_POINT('Ctrl Pts',(-8.55012914148257,14.129802627925,3.69989123127804));
#85210=CARTESIAN_POINT('Ctrl Pts',(-8.54727434022999,14.1310454328642,3.67739135523392));
#85211=CARTESIAN_POINT('Ctrl Pts',(-8.54645687123336,14.1314207296773,3.67056350882363));
#85212=CARTESIAN_POINT('Ctrl Pts',(-8.54512015145841,14.1320702057688,3.65869025793949));
#85213=CARTESIAN_POINT('Ctrl Pts',(-8.54457895347306,14.1323450659023,3.65364748577135));
#85214=CARTESIAN_POINT('Ctrl Pts',(-8.54358653583629,14.132873178244,3.64392421824097));
#85215=CARTESIAN_POINT('Ctrl Pts',(-8.54313163891788,14.1331265419234,3.6392441682159));
#85216=CARTESIAN_POINT('Ctrl Pts',(-8.54210838049684,14.1337245519092,3.62816232078356));
#85217=CARTESIAN_POINT('Ctrl Pts',(-8.54155961536221,14.1340685852731,3.62175878174878));
#85218=CARTESIAN_POINT('Ctrl Pts',(-8.53977649447696,14.1352750360525,3.5992062115059));
#85219=CARTESIAN_POINT('Ctrl Pts',(-8.53876801501689,14.1361304509997,3.58304018311448));
#85220=CARTESIAN_POINT('Ctrl Pts',(-8.53248259780247,14.1433304939431,3.44560282877686));
#85221=CARTESIAN_POINT('Ctrl Pts',(-8.54204308505491,14.1491636747077,3.32412945788826));
#85222=CARTESIAN_POINT('Ctrl Pts',(-8.57805434608823,14.15787729412,3.1490059559888));
#85223=CARTESIAN_POINT('Ctrl Pts',(-8.59291071834515,14.1606950199935,3.09352106106201));
#85224=CARTESIAN_POINT('Ctrl Pts',(-8.61920250345888,14.1649751413803,3.01429303644262));
#85225=CARTESIAN_POINT('Ctrl Pts',(-8.62808030387407,14.1663381251565,2.98975578271803));
#85226=CARTESIAN_POINT('Ctrl Pts',(-8.63968409872609,14.1680416071993,2.96018040847446));
#85227=CARTESIAN_POINT('Ctrl Pts',(-8.64179039701179,14.1683479887029,2.95490256387294));
#85228=CARTESIAN_POINT('Ctrl Pts',(-8.64513632337104,14.168830515243,2.94665833060462));
#85229=CARTESIAN_POINT('Ctrl Pts',(-8.64635510246021,14.1690054388122,2.94368347472463));
#85230=CARTESIAN_POINT('Ctrl Pts',(-8.64865142077304,14.1693334992296,2.93813073226279));
#85231=CARTESIAN_POINT('Ctrl Pts',(-8.64972654561636,14.1694864918822,2.93555190268197));
#85232=CARTESIAN_POINT('Ctrl Pts',(-8.65220620303712,14.1698379696396,2.92965174255666));
#85233=CARTESIAN_POINT('Ctrl Pts',(-8.65361562770511,14.1700367453811,2.92633252195491));
#85234=CARTESIAN_POINT('Ctrl Pts',(-8.65734537343156,14.1705600907946,2.91763836169766));
#85235=CARTESIAN_POINT('Ctrl Pts',(-8.65968568084542,14.1708858126703,2.91227213138819));
#85236=CARTESIAN_POINT('Ctrl Pts',(-8.67608519559245,14.1731493982531,2.8752761024063));
#85237=CARTESIAN_POINT('Ctrl Pts',(-8.69122949671118,14.1751453328076,2.84414196965002));
#85238=CARTESIAN_POINT('Ctrl Pts',(-8.71494682760646,14.178113061807,2.7994821412635));
#85239=CARTESIAN_POINT('Ctrl Pts',(-8.72266172865886,14.1790569898152,2.78551148116026));
#85240=CARTESIAN_POINT('Ctrl Pts',(-8.77642708612927,14.1854820287117,2.69180454241418));
#85241=CARTESIAN_POINT('Ctrl Pts',(-8.82968620171524,14.1910977721433,2.61644040014841));
#85242=CARTESIAN_POINT('Ctrl Pts',(-8.93058345149162,14.2002493353626,2.49893892311125));
#85243=CARTESIAN_POINT('Ctrl Pts',(-8.9745170527604,14.2038732225143,2.45397832813544));
#85244=CARTESIAN_POINT('Ctrl Pts',(-9.03243913592683,14.2082154081896,2.4018713935886));
#85245=CARTESIAN_POINT('Ctrl Pts',(-9.04382609879661,14.2090501680802,2.39194225934966));
#85246=CARTESIAN_POINT('Ctrl Pts',(-9.06052367029214,14.2102476589927,2.37783152260777));
#85247=CARTESIAN_POINT('Ctrl Pts',(-9.06571244959343,14.2106161593746,2.3735078158146));
#85248=CARTESIAN_POINT('Ctrl Pts',(-9.0748346356763,14.2112577718285,2.36601286457413));
#85249=CARTESIAN_POINT('Ctrl Pts',(-9.0787548505221,14.2115315179099,2.36282580485295));
#85250=CARTESIAN_POINT('Ctrl Pts',(-9.0863811381315,14.2120602621776,2.35669109711661));
#85251=CARTESIAN_POINT('Ctrl Pts',(-9.09008516347825,14.2123153555749,2.35374101391647));
#85252=CARTESIAN_POINT('Ctrl Pts',(-9.0989491470618,14.2129217796122,2.34675130489529));
#85253=CARTESIAN_POINT('Ctrl Pts',(-9.10412207261081,14.2132724554158,2.34272823699314));
#85254=CARTESIAN_POINT('Ctrl Pts',(-9.12277459649179,14.2145255735667,2.32842188481019));
#85255=CARTESIAN_POINT('Ctrl Pts',(-9.13640591385913,14.2154202717952,2.31833804566199));
#85256=CARTESIAN_POINT('Ctrl Pts',(-9.23892428091119,14.2220019485415,2.24522130191374));
#85257=CARTESIAN_POINT('Ctrl Pts',(-9.33442725608668,14.2272907522713,2.19205449586917));
#85258=CARTESIAN_POINT('Ctrl Pts',(-9.4960128214411,14.2358090642966,2.12442366659073));
#85259=CARTESIAN_POINT('Ctrl Pts',(-9.558729519278,14.2390309998275,2.10304169936223));
#85260=CARTESIAN_POINT('Ctrl Pts',(-9.65002929994171,14.2438589385648,2.0786786318));
#85261=CARTESIAN_POINT('Ctrl Pts',(-9.67759021020195,14.2453341119206,2.07217450623295));
#85262=CARTESIAN_POINT('Ctrl Pts',(-9.7110222790235,14.2471633097302,2.06530211867285));
#85263=CARTESIAN_POINT('Ctrl Pts',(-9.71673089268684,14.2474770376255,2.06416409556601));
#85264=CARTESIAN_POINT('Ctrl Pts',(-9.72563267694309,14.2479686213699,2.0624446600172));
#85265=CARTESIAN_POINT('Ctrl Pts',(-9.72882131420717,14.2481451799787,2.06183975043562));
#85266=CARTESIAN_POINT('Ctrl Pts',(-9.73475495769333,14.2484746541843,2.0607345266009));
#85267=CARTESIAN_POINT('Ctrl Pts',(-9.73749939668629,14.2486274130061,2.06023145323678));
#85268=CARTESIAN_POINT('Ctrl Pts',(-9.74375075003085,14.2489762053549,2.05910400788803));
#85269=CARTESIAN_POINT('Ctrl Pts',(-9.74725850233021,14.2491725124807,2.05848459148154));
#85270=CARTESIAN_POINT('Ctrl Pts',(-9.75639311946363,14.2496851998631,2.05690592140658));
#85271=CARTESIAN_POINT('Ctrl Pts',(-9.76202334215519,14.2500026593933,2.0559667801384));
#85272=CARTESIAN_POINT('Ctrl Pts',(-9.79892082977262,14.252092015672,2.05003379366724));
#85273=CARTESIAN_POINT('Ctrl Pts',(-9.8303355587873,14.2539125479754,2.04602320605826));
#85274=CARTESIAN_POINT('Ctrl Pts',(-9.87327476152129,14.2564355497007,2.04195178757122));
#85275=CARTESIAN_POINT('Ctrl Pts',(-9.88470849612051,14.257110708452,2.04100317505609));
#85276=CARTESIAN_POINT('Ctrl Pts',(-9.98805535957383,14.2632370996351,2.03365128649823));
#85277=CARTESIAN_POINT('Ctrl Pts',(-10.0803708557154,14.2688627528796,2.03580652673169));
#85278=CARTESIAN_POINT('Ctrl Pts',(-10.2226423370278,14.2773691824545,2.05263128331906));
#85279=CARTESIAN_POINT('Ctrl Pts',(-10.2730654554302,14.2803548821478,2.06129160435795));
#85280=CARTESIAN_POINT('Ctrl Pts',(-10.3520953055363,14.2849657170242,2.07917103588605));
#85281=CARTESIAN_POINT('Ctrl Pts',(-10.3810472216457,14.2866402884213,2.08666025011202));
#85282=CARTESIAN_POINT('Ctrl Pts',(-10.4181580309301,14.2887688950394,2.09748340421269));
#85283=CARTESIAN_POINT('Ctrl Pts',(-10.4265430364494,14.2892486649193,2.10001072038826));
#85284=CARTESIAN_POINT('Ctrl Pts',(-10.4401170826114,14.2900235277542,2.10423533468347));
#85285=CARTESIAN_POINT('Ctrl Pts',(-10.445320114575,14.290320104036,2.10588664591674));
#85286=CARTESIAN_POINT('Ctrl Pts',(-10.4552950013835,14.2908878815622,2.10911396433005));
#85287=CARTESIAN_POINT('Ctrl Pts',(-10.46006820856,14.2911592232891,2.11068551189828));
#85288=CARTESIAN_POINT('Ctrl Pts',(-10.4709653296392,14.2917779229859,2.11433563609061));
#85289=CARTESIAN_POINT('Ctrl Pts',(-10.4770837747838,14.2921247498063,2.11643028914363));
#85290=CARTESIAN_POINT('Ctrl Pts',(-10.4932879215678,14.2930419221006,2.1220980586177));
#85291=CARTESIAN_POINT('Ctrl Pts',(-10.5033487668819,14.2936099615852,2.12574137784267));
#85292=CARTESIAN_POINT('Ctrl Pts',(-10.5898977075677,14.2984862620739,2.15816120114442));
#85293=CARTESIAN_POINT('Ctrl Pts',(-10.6638946856737,14.3025741231933,2.19318833173846));
#85294=CARTESIAN_POINT('Ctrl Pts',(-10.7883826980132,14.3096251898686,2.26543387012209));
#85295=CARTESIAN_POINT('Ctrl Pts',(-10.8401319481357,14.3126196953081,2.30005043258246));
#85296=CARTESIAN_POINT('Ctrl Pts',(-10.9370757284407,14.3186125422779,2.37425242145927));
#85297=CARTESIAN_POINT('Ctrl Pts',(-10.9823467030928,14.3216019416517,2.4135322903232));
#85298=CARTESIAN_POINT('Ctrl Pts',(-11.0329370496065,14.3253455418522,2.46318058809871));
#85299=CARTESIAN_POINT('Ctrl Pts',(-11.0407066954874,14.3259327124718,2.47097959162656));
#85300=CARTESIAN_POINT('Ctrl Pts',(-11.0513131777703,14.3267526058414,2.48186914603582));
#85301=CARTESIAN_POINT('Ctrl Pts',(-11.0542260102086,14.3269797202769,2.48488554730696));
#85302=CARTESIAN_POINT('Ctrl Pts',(-11.0591235563383,14.3273649751488,2.49000104575627));
#85303=CARTESIAN_POINT('Ctrl Pts',(-11.0611151159603,14.3275225944139,2.49209360272408));
#85304=CARTESIAN_POINT('Ctrl Pts',(-11.0648971291998,14.3278237772223,2.49609104571092));
#85305=CARTESIAN_POINT('Ctrl Pts',(-11.0666886947265,14.3279672506064,2.4979948540056));
#85306=CARTESIAN_POINT('Ctrl Pts',(-11.0713889883588,14.3283457509564,2.50301651597053));
#85307=CARTESIAN_POINT('Ctrl Pts',(-11.0742891851997,14.3285814125397,2.50614227505617));
#85308=CARTESIAN_POINT('Ctrl Pts',(-11.0843897913738,14.329409457747,2.51712432224812));
#85309=CARTESIAN_POINT('Ctrl Pts',(-11.091517839206,14.3300069039825,2.52504635456808));
#85310=CARTESIAN_POINT('Ctrl Pts',(-11.1665083321774,14.3364266309579,2.6102431518381));
#85311=CARTESIAN_POINT('Ctrl Pts',(-11.2261270538426,14.3426982024485,2.69438294245455));
#85312=CARTESIAN_POINT('Ctrl Pts',(-11.3199836244461,14.3542205076847,2.86171960095103));
#85313=CARTESIAN_POINT('Ctrl Pts',(-11.3563652307633,14.3594728738015,2.94319116259341));
#85314=CARTESIAN_POINT('Ctrl Pts',(-11.3916613937173,14.3656142093642,3.04665519222934));
#85315=CARTESIAN_POINT('Ctrl Pts',(-11.3978057672359,14.3667399744873,3.06596999585366));
#85316=CARTESIAN_POINT('Ctrl Pts',(-11.4056964885964,14.3682693235905,3.0926829342911));
#85317=CARTESIAN_POINT('Ctrl Pts',(-11.4077891700488,14.3686840492858,3.09997566848611));
#85318=CARTESIAN_POINT('Ctrl Pts',(-11.4112223426029,14.3693803230517,3.11230055014877));
#85319=CARTESIAN_POINT('Ctrl Pts',(-11.4125928418872,14.3696628335035,3.11732412187163));
#85320=CARTESIAN_POINT('Ctrl Pts',(-11.4152529747908,14.3702204300546,3.12728389497237));
#85321=CARTESIAN_POINT('Ctrl Pts',(-11.4165436652269,14.3704955467296,3.13221973541871));
#85322=CARTESIAN_POINT('Ctrl Pts',(-11.4196226872878,14.3711632534436,3.14425118461895));
#85323=CARTESIAN_POINT('Ctrl Pts',(-11.4213836741099,14.3715549643808,3.15135369280404));
#85324=CARTESIAN_POINT('Ctrl Pts',(-11.4270978726473,14.3728601218171,3.1751636286099));
#85325=CARTESIAN_POINT('Ctrl Pts',(-11.4308104332278,14.3737659223643,3.1919276983659));
#85326=CARTESIAN_POINT('Ctrl Pts',(-11.4536926321944,14.3797737405633,3.30460989540102));
#85327=CARTESIAN_POINT('Ctrl Pts',(-11.4634999999956,14.3845638431022,3.40217672343184));
#85328=CARTESIAN_POINT('Ctrl Pts',(-11.4635,14.3893209889657,3.49999999993469));
#85329=CARTESIAN_POINT('Origin',(-10.,13.2,3.5));
#85330=CARTESIAN_POINT('',(-11.4635,14.961903098074,3.50000000001399));
#85331=CARTESIAN_POINT('',(-11.4635,14.8882344353249,3.49999999998375));
#85332=CARTESIAN_POINT('',(-11.4635,13.2,3.5));
#85333=CARTESIAN_POINT('',(-11.4634998863947,14.9618714498257,3.49938784807456));
#85334=CARTESIAN_POINT('Ctrl Pts',(-11.4635,14.961903098074,3.50000000001399));
#85335=CARTESIAN_POINT('Ctrl Pts',(-11.4635,14.9618925647885,3.49979609515158));
#85336=CARTESIAN_POINT('Ctrl Pts',(-11.4634999573859,14.961882029762,3.49959218904603));
#85337=CARTESIAN_POINT('Ctrl Pts',(-11.463499872156,14.9618714929895,3.49938828171059));
#85338=CARTESIAN_POINT('Ctrl Pts',(-11.4634998719743,14.9618714705267,3.4993878470109));
#85339=CARTESIAN_POINT('Ctrl Pts',(-11.4634941562415,14.9611653489416,3.48572300442809));
#85340=CARTESIAN_POINT('Ctrl Pts',(-11.463297055919,14.9604517338739,3.47205933875743));
#85341=CARTESIAN_POINT('Ctrl Pts',(-11.462675813711,14.9592958685541,3.45021222867011));
#85342=CARTESIAN_POINT('Ctrl Pts',(-11.462374217243,14.9588594130255,3.44202585900509));
#85343=CARTESIAN_POINT('Ctrl Pts',(-11.4618314016375,14.9582144209366,3.43003024009514));
#85344=CARTESIAN_POINT('Ctrl Pts',(-11.4616439768593,14.9580086649302,3.42621857699805));
#85345=CARTESIAN_POINT('Ctrl Pts',(-11.4612918956356,14.9576492267382,3.41958716663405));
#85346=CARTESIAN_POINT('Ctrl Pts',(-11.4611339795133,14.9574959074667,3.41676706385665));
#85347=CARTESIAN_POINT('Ctrl Pts',(-11.4608126232754,14.9571983649139,3.41131119760458));
#85348=CARTESIAN_POINT('Ctrl Pts',(-11.4606502101068,14.9570541982038,3.408675372308));
#85349=CARTESIAN_POINT('Ctrl Pts',(-11.460311369411,14.9567652687256,3.40340855334878));
#85350=CARTESIAN_POINT('Ctrl Pts',(-11.4601349648237,14.9566205107315,3.40077758585935));
#85351=CARTESIAN_POINT('Ctrl Pts',(-11.4596963723103,14.9562736108224,3.39449083336596));
#85352=CARTESIAN_POINT('Ctrl Pts',(-11.4594275607889,14.9560711072967,3.39083554702266));
#85353=CARTESIAN_POINT('Ctrl Pts',(-11.4584155458281,14.955343182091,3.37774660656628));
#85354=CARTESIAN_POINT('Ctrl Pts',(-11.4575945969423,14.9548136966491,3.36831940949505));
#85355=CARTESIAN_POINT('Ctrl Pts',(-11.4546921843024,14.953115600815,3.33835537049578));
#85356=CARTESIAN_POINT('Ctrl Pts',(-11.4522676952669,14.9519311692878,3.31785501242865));
#85357=CARTESIAN_POINT('Ctrl Pts',(-11.4324365182466,14.94360707134,3.17597209312809));
#85358=CARTESIAN_POINT('Ctrl Pts',(-11.40026788733,14.9360397509419,3.05714430200627));
#85359=CARTESIAN_POINT('Ctrl Pts',(-11.3314871629945,14.9253872985827,2.88977453303682));
#85360=CARTESIAN_POINT('Ctrl Pts',(-11.3061142940837,14.9220330636867,2.83720295945621));
#85361=CARTESIAN_POINT('Ctrl Pts',(-11.2705831372885,14.9179764225479,2.77359664460495));
#85362=CARTESIAN_POINT('Ctrl Pts',(-11.2633089494245,14.9171741070723,2.76101836071715));
#85363=CARTESIAN_POINT('Ctrl Pts',(-11.2524353858916,14.9160144861728,2.74284609249837));
#85364=CARTESIAN_POINT('Ctrl Pts',(-11.2489834406885,14.9156519057848,2.7371652850024));
#85365=CARTESIAN_POINT('Ctrl Pts',(-11.242849486914,14.9150172127121,2.72722400135307));
#85366=CARTESIAN_POINT('Ctrl Pts',(-11.2401839941528,14.9147445055185,2.7229535067101));
#85367=CARTESIAN_POINT('Ctrl Pts',(-11.2346002556836,14.9141795787947,2.71410949211253));
#85368=CARTESIAN_POINT('Ctrl Pts',(-11.2316785034138,14.9138874934652,2.70953826971854));
#85369=CARTESIAN_POINT('Ctrl Pts',(-11.2240540772426,14.913134248671,2.69775440114759));
#85370=CARTESIAN_POINT('Ctrl Pts',(-11.2193130126363,14.9126745140809,2.69056676224568));
#85371=CARTESIAN_POINT('Ctrl Pts',(-11.2001320945518,14.9108482125492,2.662038719991));
#85372=CARTESIAN_POINT('Ctrl Pts',(-11.1851927706987,14.9095003519492,2.64103879399989));
#85373=CARTESIAN_POINT('Ctrl Pts',(-11.097529470527,14.9019754130674,2.52445698764153));
#85374=CARTESIAN_POINT('Ctrl Pts',(-11.0138163647713,14.8962586810473,2.43772302821349));
#85375=CARTESIAN_POINT('Ctrl Pts',(-10.882616825591,14.8879939319066,2.33158776942962));
#85376=CARTESIAN_POINT('Ctrl Pts',(-10.8432890537668,14.8855824008541,2.30289409147578));
#85377=CARTESIAN_POINT('Ctrl Pts',(-10.7894771440365,14.882268982896,2.26760205810116));
#85378=CARTESIAN_POINT('Ctrl Pts',(-10.7762085480918,14.8814508715331,2.25920223126527));
#85379=CARTESIAN_POINT('Ctrl Pts',(-10.7565976213906,14.8802362588672,2.24722498349501));
#85380=CARTESIAN_POINT('Ctrl Pts',(-10.7503593125465,14.8798490938724,2.24347857135356));
#85381=CARTESIAN_POINT('Ctrl Pts',(-10.7404526528811,14.8792325985728,2.23762921635464));
#85382=CARTESIAN_POINT('Ctrl Pts',(-10.736802605289,14.8790051010416,2.23549533550374));
#85383=CARTESIAN_POINT('Ctrl Pts',(-10.7298979823834,14.8785739913863,2.23149881872907));
#85384=CARTESIAN_POINT('Ctrl Pts',(-10.7266453868623,14.8783705889706,2.22963281186522));
#85385=CARTESIAN_POINT('Ctrl Pts',(-10.7209755863483,14.8780154118914,2.22640895870506));
#85386=CARTESIAN_POINT('Ctrl Pts',(-10.7185616064974,14.8778639980089,2.22504543054102));
#85387=CARTESIAN_POINT('Ctrl Pts',(-10.7134640906307,14.8775438308677,2.2221851923121));
#85388=CARTESIAN_POINT('Ctrl Pts',(-10.7107797177237,14.8773749825155,2.22069007512704));
#85389=CARTESIAN_POINT('Ctrl Pts',(-10.7036775305322,14.8769276414606,2.21676361817231));
#85390=CARTESIAN_POINT('Ctrl Pts',(-10.699251864399,14.8766482637709,2.21434666133254));
#85391=CARTESIAN_POINT('Ctrl Pts',(-10.6805588544942,14.8754659157775,2.20426305490482));
#85392=CARTESIAN_POINT('Ctrl Pts',(-10.6661777738268,14.8745506408534,2.19681094465549));
#85393=CARTESIAN_POINT('Ctrl Pts',(-10.5079179185524,14.8644412056483,2.11810658127842));
#85394=CARTESIAN_POINT('Ctrl Pts',(-10.353367839915,14.8543869381076,2.0707500682976));
#85395=CARTESIAN_POINT('Ctrl Pts',(-10.1541503836348,14.8428101526799,2.04408044742302));
#85396=CARTESIAN_POINT('Ctrl Pts',(-10.1139044482114,14.8405295819394,2.04038008045864));
#85397=CARTESIAN_POINT('Ctrl Pts',(-10.0639048801985,14.8377673890358,2.03786397441423));
#85398=CARTESIAN_POINT('Ctrl Pts',(-10.0542510453968,14.8372373001573,2.03747395873035));
#85399=CARTESIAN_POINT('Ctrl Pts',(-10.038939492813,14.836401534841,2.03700718804892));
#85400=CARTESIAN_POINT('Ctrl Pts',(-10.0332840893871,14.8360939178519,2.03686759909809));
#85401=CARTESIAN_POINT('Ctrl Pts',(-10.0226473009366,14.8355173312904,2.03666676194556));
#85402=CARTESIAN_POINT('Ctrl Pts',(-10.0176661497447,14.8352481372942,2.03659815025506));
#85403=CARTESIAN_POINT('Ctrl Pts',(-10.0064704090983,14.8346448923091,2.0365011089357));
#85404=CARTESIAN_POINT('Ctrl Pts',(-10.0002557719555,14.834311284629,2.03648682734015));
#85405=CARTESIAN_POINT('Ctrl Pts',(-9.98440626561432,14.8334635532542,2.03655136123908));
#85406=CARTESIAN_POINT('Ctrl Pts',(-9.97477183965166,14.83295115272,2.03668573823459));
#85407=CARTESIAN_POINT('Ctrl Pts',(-9.91651883599945,14.8298696133236,2.03807372433107));
#85408=CARTESIAN_POINT('Ctrl Pts',(-9.86798379163357,14.827373575416,2.04165508579084));
#85409=CARTESIAN_POINT('Ctrl Pts',(-9.68532041755657,14.8181295829508,2.06432982740108));
#85410=CARTESIAN_POINT('Ctrl Pts',(-9.55391115244006,14.8118460513211,2.0995821566756));
#85411=CARTESIAN_POINT('Ctrl Pts',(-9.40201905512112,14.8034343129593,2.16391449073052));
#85412=CARTESIAN_POINT('Ctrl Pts',(-9.37516234655413,14.801896781624,2.1762615931939));
#85413=CARTESIAN_POINT('Ctrl Pts',(-9.34342490366024,14.7999978699034,2.19203360609857));
#85414=CARTESIAN_POINT('Ctrl Pts',(-9.33816607903672,14.7996804672609,2.1946867029691));
#85415=CARTESIAN_POINT('Ctrl Pts',(-9.33002211141636,14.7991844151925,2.19885723131609));
#85416=CARTESIAN_POINT('Ctrl Pts',(-9.32712572041076,14.7990071023433,2.20035270971994));
#85417=CARTESIAN_POINT('Ctrl Pts',(-9.32176191953072,14.7986770355272,2.20314490947861));
#85418=CARTESIAN_POINT('Ctrl Pts',(-9.31929320483483,14.7985244445488,2.20443901021965));
#85419=CARTESIAN_POINT('Ctrl Pts',(-9.31369845472581,14.7981771027566,2.20739218497442));
#85420=CARTESIAN_POINT('Ctrl Pts',(-9.31057474484624,14.7979820868382,2.20905554281994));
#85421=CARTESIAN_POINT('Ctrl Pts',(-9.30108543529763,14.7973864246472,2.21415281076305));
#85422=CARTESIAN_POINT('Ctrl Pts',(-9.29473933011607,14.7969836176409,2.21762254154762));
#85423=CARTESIAN_POINT('Ctrl Pts',(-9.23588990555423,14.7932085338717,2.25036739460156));
#85424=CARTESIAN_POINT('Ctrl Pts',(-9.18521625643155,14.7896639527778,2.28280163359406));
#85425=CARTESIAN_POINT('Ctrl Pts',(-9.13221996427978,14.7857368314953,2.32151765106432));
#85426=CARTESIAN_POINT('Ctrl Pts',(-9.12777269944645,14.7854054802587,2.32480538938953));
#85427=CARTESIAN_POINT('Ctrl Pts',(-9.03275776395706,14.7782888873674,2.39588371630588));
#85428=CARTESIAN_POINT('Ctrl Pts',(-8.95031998660529,14.7714252403453,2.47393537866975));
#85429=CARTESIAN_POINT('Ctrl Pts',(-8.85512799931429,14.7629320992061,2.58767513568424));
#85430=CARTESIAN_POINT('Ctrl Pts',(-8.83353907418968,14.7609546478014,2.61544487879821));
#85431=CARTESIAN_POINT('Ctrl Pts',(-8.80756116954138,14.7585064027503,2.65146750378906));
#85432=CARTESIAN_POINT('Ctrl Pts',(-8.80222338109642,14.7579993708997,2.65901906190863));
#85433=CARTESIAN_POINT('Ctrl Pts',(-8.79378808640856,14.7571915267414,2.67119601435724));
#85434=CARTESIAN_POINT('Ctrl Pts',(-8.79064483046342,14.7568889892139,2.67578928530601));
#85435=CARTESIAN_POINT('Ctrl Pts',(-8.78472983009452,14.7563167443723,2.68453962333893));
#85436=CARTESIAN_POINT('Ctrl Pts',(-8.78195302762407,14.7560468498355,2.6886931618011));
#85437=CARTESIAN_POINT('Ctrl Pts',(-8.77568902705632,14.7554351020333,2.69816749795127));
#85438=CARTESIAN_POINT('Ctrl Pts',(-8.77221512965469,14.7550937462624,2.7034969970504));
#85439=CARTESIAN_POINT('Ctrl Pts',(-8.76330652822853,14.7542127817259,2.71736095461726));
#85440=CARTESIAN_POINT('Ctrl Pts',(-8.75792532962948,14.7536751391083,2.72592950027572));
#85441=CARTESIAN_POINT('Ctrl Pts',(-8.72212342038124,14.750059002665,2.78427204559509));
#85442=CARTESIAN_POINT('Ctrl Pts',(-8.69461165083842,14.7470877696307,2.83577313663909));
#85443=CARTESIAN_POINT('Ctrl Pts',(-8.63112667196301,14.7395221303334,2.97389023531073));
#85444=CARTESIAN_POINT('Ctrl Pts',(-8.60026970582796,14.7350612777493,3.06255254069402));
#85445=CARTESIAN_POINT('Ctrl Pts',(-8.56538816939235,14.727793208853,3.20571536017011));
#85446=CARTESIAN_POINT('Ctrl Pts',(-8.55556012721204,14.7250943646727,3.25853170470827));
#85447=CARTESIAN_POINT('Ctrl Pts',(-8.54731548323043,14.7217040720922,3.32209950573827));
#85448=CARTESIAN_POINT('Ctrl Pts',(-8.54608535369498,14.7211475789637,3.33244976865544));
#85449=CARTESIAN_POINT('Ctrl Pts',(-8.54452527851898,14.7203638287484,3.3468908354331));
#85450=CARTESIAN_POINT('Ctrl Pts',(-8.54410179740904,14.7201415515894,3.35097146578372));
#85451=CARTESIAN_POINT('Ctrl Pts',(-8.54341121256805,14.7197621457897,3.35790991350719));
#85452=CARTESIAN_POINT('Ctrl Pts',(-8.54313534472277,14.7196055022068,3.36076687021167));
#85453=CARTESIAN_POINT('Ctrl Pts',(-8.54262265748319,14.7193043191511,3.3662447871321));
#85454=CARTESIAN_POINT('Ctrl Pts',(-8.54238450078552,14.7191598593208,3.3688655969126));
#85455=CARTESIAN_POINT('Ctrl Pts',(-8.54177063406256,14.7187750777326,3.37582927838293));
#85456=CARTESIAN_POINT('Ctrl Pts',(-8.54140725941812,14.7185340815292,3.38017317532311));
#85457=CARTESIAN_POINT('Ctrl Pts',(-8.54017657920275,14.717668181767,3.39572099613764));
#85458=CARTESIAN_POINT('Ctrl Pts',(-8.5394189400394,14.7170376001372,3.40693291616243));
#85459=CARTESIAN_POINT('Ctrl Pts',(-8.53387118612173,14.7114194994315,3.50597552797113));
#85460=CARTESIAN_POINT('Ctrl Pts',(-8.53687993494716,14.7061029330103,3.59405664850519));
#85461=CARTESIAN_POINT('Ctrl Pts',(-8.56047688999091,14.6946357609698,3.78304220603267));
#85462=CARTESIAN_POINT('Ctrl Pts',(-8.58383037462774,14.6885362444489,3.8831570149342));
#85463=CARTESIAN_POINT('Ctrl Pts',(-8.62425892384568,14.6816071550057,3.99959809355428));
#85464=CARTESIAN_POINT('Ctrl Pts',(-8.63147184563165,14.6804553979283,4.01903036166328));
#85465=CARTESIAN_POINT('Ctrl Pts',(-8.64190962845576,14.6788970395135,4.04541849489856));
#85466=CARTESIAN_POINT('Ctrl Pts',(-8.64477970049039,14.6784787354355,4.05251129832242));
#85467=CARTESIAN_POINT('Ctrl Pts',(-8.64970087862084,14.6777782311501,4.0644039086174));
#85468=CARTESIAN_POINT('Ctrl Pts',(-8.65172225469562,14.6774950414398,4.06921578663917));
#85469=CARTESIAN_POINT('Ctrl Pts',(-8.6557652324437,14.6769374529482,4.07869770536841));
#85470=CARTESIAN_POINT('Ctrl Pts',(-8.65778553535971,14.6766630153595,4.08336821675354));
#85471=CARTESIAN_POINT('Ctrl Pts',(-8.66228946418074,14.676060286359,4.09363308185138));
#85472=CARTESIAN_POINT('Ctrl Pts',(-8.66478391611111,14.675732366568,4.09922260002691));
#85473=CARTESIAN_POINT('Ctrl Pts',(-8.67366700950775,14.6745848799438,4.11879675816106));
#85474=CARTESIAN_POINT('Ctrl Pts',(-8.68024100620505,14.6737716208157,4.13269649240202));
#85475=CARTESIAN_POINT('Ctrl Pts',(-8.745295869381,14.6660497120382,4.2648173837534));
#85476=CARTESIAN_POINT('Ctrl Pts',(-8.81928232218055,14.6597637678889,4.37472030649176));
#85477=CARTESIAN_POINT('Ctrl Pts',(-8.94071397065072,14.6508331496625,4.51109654883778));
#85478=CARTESIAN_POINT('Ctrl Pts',(-8.97637506673069,14.6483259141703,4.54718405369752));
#85479=CARTESIAN_POINT('Ctrl Pts',(-9.03172376523995,14.6444729715065,4.5976609731145));
#85480=CARTESIAN_POINT('Ctrl Pts',(-9.05001466538014,14.6432051955157,4.6135287185643));
#85481=CARTESIAN_POINT('Ctrl Pts',(-9.0729741613783,14.6416085773171,4.63246907011735));
#85482=CARTESIAN_POINT('Ctrl Pts',(-9.07727873014917,14.6413090137971,4.63597911794853));
#85483=CARTESIAN_POINT('Ctrl Pts',(-9.08408386574832,14.6408348998374,4.64146398850898));
#85484=CARTESIAN_POINT('Ctrl Pts',(-9.08657112509848,14.6406615018767,4.64345533019182));
#85485=CARTESIAN_POINT('Ctrl Pts',(-9.09125463080724,14.6403347450532,4.64717999105758));
#85486=CARTESIAN_POINT('Ctrl Pts',(-9.09344935536209,14.6401815186307,4.64891514315538));
#85487=CARTESIAN_POINT('Ctrl Pts',(-9.09847051712793,14.6398307332045,4.65286153541031));
#85488=CARTESIAN_POINT('Ctrl Pts',(-9.10130011847474,14.6396328916599,4.65506867791382));
#85489=CARTESIAN_POINT('Ctrl Pts',(-9.10882500576555,14.6391064010243,4.66089384338185));
#85490=CARTESIAN_POINT('Ctrl Pts',(-9.11353415460382,14.6387765470279,4.66449374771605));
#85491=CARTESIAN_POINT('Ctrl Pts',(-9.14690316320284,14.6364373787969,4.68968295130505));
#85492=CARTESIAN_POINT('Ctrl Pts',(-9.17632455243358,14.6343657221275,4.71023885503368));
#85493=CARTESIAN_POINT('Ctrl Pts',(-9.21777709636512,14.6314663595144,4.73698856277608));
#85494=CARTESIAN_POINT('Ctrl Pts',(-9.22918519330165,14.6306703442032,4.74412937238147));
#85495=CARTESIAN_POINT('Ctrl Pts',(-9.32786375717238,14.6238106622919,4.8040182128677));
#85496=CARTESIAN_POINT('Ctrl Pts',(-9.42033762718389,14.6175790371933,4.84767379449155));
#85497=CARTESIAN_POINT('Ctrl Pts',(-9.56892749650163,14.6083352996318,4.899672259121));
#85498=CARTESIAN_POINT('Ctrl Pts',(-9.62225897527975,14.6051535840508,4.91499779604537));
#85499=CARTESIAN_POINT('Ctrl Pts',(-9.69013264525586,14.6012810005489,4.93038966265702));
#85500=CARTESIAN_POINT('Ctrl Pts',(-9.70397350472048,14.600500173755,4.93331807301127));
#85501=CARTESIAN_POINT('Ctrl Pts',(-9.72430774509668,14.5993656696688,4.93731321423341));
#85502=CARTESIAN_POINT('Ctrl Pts',(-9.73076903411243,14.5990070340954,4.93853751574538));
#85503=CARTESIAN_POINT('Ctrl Pts',(-9.74218042512871,14.5983768589851,4.94062019757165));
#85504=CARTESIAN_POINT('Ctrl Pts',(-9.74712707289918,14.5981047514563,4.94149671191149));
#85505=CARTESIAN_POINT('Ctrl Pts',(-9.75745562822386,14.5975387741943,4.94327206341733));
#85506=CARTESIAN_POINT('Ctrl Pts',(-9.7628382534342,14.5972450527911,4.94416630911928));
#85507=CARTESIAN_POINT('Ctrl Pts',(-9.77686728426921,14.5964826533297,4.94641648132642));
#85508=CARTESIAN_POINT('Ctrl Pts',(-9.78552114552896,14.5960154674733,4.94772499866229));
#85509=CARTESIAN_POINT('Ctrl Pts',(-9.82081154011209,14.5941224376476,4.95273774277879));
#85510=CARTESIAN_POINT('Ctrl Pts',(-9.84753689645598,14.5927171097038,4.95578520920637));
#85511=CARTESIAN_POINT('Ctrl Pts',(-10.0330484797189,14.5831260044657,4.97177376483858));
#85512=CARTESIAN_POINT('Ctrl Pts',(-10.1929050688574,14.5758260786432,4.95944774436787));
#85513=CARTESIAN_POINT('Ctrl Pts',(-10.3777597628051,14.5661432464801,4.91424628419051));
#85514=CARTESIAN_POINT('Ctrl Pts',(-10.4076557724205,14.5645318296078,4.90592015866132));
#85515=CARTESIAN_POINT('Ctrl Pts',(-10.4429594830149,14.5625502388016,4.89486729993801));
#85516=CARTESIAN_POINT('Ctrl Pts',(-10.4486454937222,14.5622286148242,4.89304885288785));
#85517=CARTESIAN_POINT('Ctrl Pts',(-10.4574351501718,14.5617273783574,4.8901784315798));
#85518=CARTESIAN_POINT('Ctrl Pts',(-10.4605467225262,14.5615491477444,4.88915071327117));
#85519=CARTESIAN_POINT('Ctrl Pts',(-10.4662970800943,14.5612182581444,4.88722998949425));
#85520=CARTESIAN_POINT('Ctrl Pts',(-10.4689367818223,14.5610657691221,4.88633989517037));
#85521=CARTESIAN_POINT('Ctrl Pts',(-10.4749025318789,14.5607198018598,4.88430928569167));
#85522=CARTESIAN_POINT('Ctrl Pts',(-10.4782270037585,14.5605260673192,4.88316432341943));
#85523=CARTESIAN_POINT('Ctrl Pts',(-10.4882689873286,14.5599380892001,4.87966529015015));
#85524=CARTESIAN_POINT('Ctrl Pts',(-10.4949733790469,14.5595417638173,4.87727421622463));
#85525=CARTESIAN_POINT('Ctrl Pts',(-10.5503824953309,14.5562365618224,4.85705612065294));
#85526=CARTESIAN_POINT('Ctrl Pts',(-10.5981211042744,14.5531989649412,4.83670202615643));
#85527=CARTESIAN_POINT('Ctrl Pts',(-10.7190833218266,14.5451739064173,4.77734929979471));
#85528=CARTESIAN_POINT('Ctrl Pts',(-10.7902575079625,14.5401292070343,4.73458328875718));
#85529=CARTESIAN_POINT('Ctrl Pts',(-10.8984476366941,14.5322059267931,4.6563674968305));
#85530=CARTESIAN_POINT('Ctrl Pts',(-10.9379013757492,14.5292514279283,4.62460469095677));
#85531=CARTESIAN_POINT('Ctrl Pts',(-10.9977635808065,14.5246825017653,4.57106564858843));
#85532=CARTESIAN_POINT('Ctrl Pts',(-11.0192878954463,14.5230197356274,4.55060275724091));
#85533=CARTESIAN_POINT('Ctrl Pts',(-11.0463201506024,14.5209038332795,4.52329012630722));
#85534=CARTESIAN_POINT('Ctrl Pts',(-11.0524087671256,14.5204253354726,4.51702720301684));
#85535=CARTESIAN_POINT('Ctrl Pts',(-11.0622065758544,14.5196520797133,4.50676669070671));
#85536=CARTESIAN_POINT('Ctrl Pts',(-11.0659500750907,14.5193558489495,4.5028022825268));
#85537=CARTESIAN_POINT('Ctrl Pts',(-11.0731007537442,14.5187884381013,4.4951443470398));
#85538=CARTESIAN_POINT('Ctrl Pts',(-11.0765112316097,14.5185171195869,4.49145401719912));
#85539=CARTESIAN_POINT('Ctrl Pts',(-11.0842721149211,14.5178980674495,4.48296904516542));
#85540=CARTESIAN_POINT('Ctrl Pts',(-11.0886098646393,14.5175508679945,4.47816293499361));
#85541=CARTESIAN_POINT('Ctrl Pts',(-11.1000503119783,14.5166318433307,4.46531686273832));
#85542=CARTESIAN_POINT('Ctrl Pts',(-11.1070968146649,14.5160623401602,4.45722723815051));
#85543=CARTESIAN_POINT('Ctrl Pts',(-11.170713829191,14.5108867113263,4.3825504771167));
#85544=CARTESIAN_POINT('Ctrl Pts',(-11.2213066435107,14.506535428348,4.31109729997014));
#85545=CARTESIAN_POINT('Ctrl Pts',(-11.3242138073556,14.49653038765,4.1340854782053));
#85546=CARTESIAN_POINT('Ctrl Pts',(-11.3707728072551,14.4909846397861,4.02590946919204));
#85547=CARTESIAN_POINT('Ctrl Pts',(-11.40684118657,14.4842295579097,3.90340756888663));
#85548=CARTESIAN_POINT('Ctrl Pts',(-11.409664275351,14.4836758391506,3.89342903996408));
#85549=CARTESIAN_POINT('Ctrl Pts',(-11.4134536590065,14.4828953613382,3.87947037684506));
#85550=CARTESIAN_POINT('Ctrl Pts',(-11.4145097163728,14.4826735271771,3.87551467950928));
#85551=CARTESIAN_POINT('Ctrl Pts',(-11.4162774447946,14.4822946514273,3.86877998664128));
#85552=CARTESIAN_POINT('Ctrl Pts',(-11.4169975781294,14.4821380916016,3.86600320030713));
#85553=CARTESIAN_POINT('Ctrl Pts',(-11.4183631342146,14.4818368898653,3.86067326567109));
#85554=CARTESIAN_POINT('Ctrl Pts',(-11.4190098353259,14.481692326592,3.85812047147511));
#85555=CARTESIAN_POINT('Ctrl Pts',(-11.4207110255185,14.4813069103332,3.85132821837439));
#85556=CARTESIAN_POINT('Ctrl Pts',(-11.4217534193583,14.4810653788785,3.84708579428408));
#85557=CARTESIAN_POINT('Ctrl Pts',(-11.4254230419094,14.480195650896,3.83185690700463));
#85558=CARTESIAN_POINT('Ctrl Pts',(-11.4279419759509,14.4795617121576,3.82084505990614));
#85559=CARTESIAN_POINT('Ctrl Pts',(-11.4483457461069,14.4741021535261,3.72664341749088));
#85560=CARTESIAN_POINT('Ctrl Pts',(-11.4590698476733,14.4689683731578,3.642075580809));
#85561=CARTESIAN_POINT('Ctrl Pts',(-11.4631290190957,14.4626991343197,3.53804989860196));
#85562=CARTESIAN_POINT('Ctrl Pts',(-11.4634999999255,14.4615539391712,3.51902508777929));
#85563=CARTESIAN_POINT('Ctrl Pts',(-11.4635,14.4604121156607,3.50000000573456));
#85564=CARTESIAN_POINT('',(-11.4634998779574,14.8881996490159,3.4994023223159));
#85565=CARTESIAN_POINT('Ctrl Pts',(-11.4635,14.3893209889657,3.49999999993469));
#85566=CARTESIAN_POINT('Ctrl Pts',(-11.4635,14.389342318194,3.5004386022108));
#85567=CARTESIAN_POINT('Ctrl Pts',(-11.4634998028312,14.3893636472093,3.50087720962041));
#85568=CARTESIAN_POINT('Ctrl Pts',(-11.4634121584128,14.394103948603,3.59835813830859));
#85569=CARTESIAN_POINT('Ctrl Pts',(-11.4536730819326,14.3987763817662,3.69513925308056));
#85570=CARTESIAN_POINT('Ctrl Pts',(-11.4322738321971,14.4044740470969,3.80090277700886));
#85571=CARTESIAN_POINT('Ctrl Pts',(-11.4299955115346,14.4050546072532,3.81155037255397));
#85572=CARTESIAN_POINT('Ctrl Pts',(-11.4266513225759,14.4058735549096,3.82636907495734));
#85573=CARTESIAN_POINT('Ctrl Pts',(-11.4256854829067,14.4061065411713,3.83056265998381));
#85574=CARTESIAN_POINT('Ctrl Pts',(-11.4241015176665,14.4064831443729,3.83730400286495));
#85575=CARTESIAN_POINT('Ctrl Pts',(-11.4234950096157,14.4066261048282,3.83985449878406));
#85576=CARTESIAN_POINT('Ctrl Pts',(-11.4222075191619,14.4069270270035,3.84520475792863));
#85577=CARTESIAN_POINT('Ctrl Pts',(-11.4215251191904,14.4070850717748,3.8480041487153));
#85578=CARTESIAN_POINT('Ctrl Pts',(-11.419838318364,14.407472206315,3.8548361176531));
#85579=CARTESIAN_POINT('Ctrl Pts',(-11.4188250028883,14.4077017985899,3.85886645287101));
#85580=CARTESIAN_POINT('Ctrl Pts',(-11.4151261661451,14.4085292398004,3.87331754375532));
#85581=CARTESIAN_POINT('Ctrl Pts',(-11.4123429586264,14.4091323342623,3.88371266315544));
#85582=CARTESIAN_POINT('Ctrl Pts',(-11.394041990626,14.4129756672591,3.94916762015689));
#85583=CARTESIAN_POINT('Ctrl Pts',(-11.3754229631227,14.4163584040188,4.0033041915881));
#85584=CARTESIAN_POINT('Ctrl Pts',(-11.3269812635271,14.423992657982,4.12120070912478));
#85585=CARTESIAN_POINT('Ctrl Pts',(-11.2956291761927,14.4282537359137,4.18418942620265));
#85586=CARTESIAN_POINT('Ctrl Pts',(-11.2207994271709,14.4369918740804,4.31078836588991));
#85587=CARTESIAN_POINT('Ctrl Pts',(-11.1765794246168,14.4414367664753,4.37372350413566));
#85588=CARTESIAN_POINT('Ctrl Pts',(-11.120844864374,14.4462815274992,4.44109081668099));
#85589=CARTESIAN_POINT('Ctrl Pts',(-11.1139830792076,14.4468666758097,4.449203267402));
#85590=CARTESIAN_POINT('Ctrl Pts',(-11.1028179259459,14.4478010115508,4.46211559070526));
#85591=CARTESIAN_POINT('Ctrl Pts',(-11.0985702194774,14.4481524517087,4.46696290642563));
#85592=CARTESIAN_POINT('Ctrl Pts',(-11.0909558831337,14.4487753865979,4.47553715049023));
#85593=CARTESIAN_POINT('Ctrl Pts',(-11.0876018488371,14.4490473956288,4.47927508403406));
#85594=CARTESIAN_POINT('Ctrl Pts',(-11.0805550178097,14.449613963184,4.487047626402));
#85595=CARTESIAN_POINT('Ctrl Pts',(-11.0768587060985,14.4499083683507,4.49107895321984));
#85596=CARTESIAN_POINT('Ctrl Pts',(-11.0671528554002,14.4506742767163,4.50154608719232));
#85597=CARTESIAN_POINT('Ctrl Pts',(-11.0611076307184,14.4511442625555,4.5079486009497));
#85598=CARTESIAN_POINT('Ctrl Pts',(-11.0339565160482,14.4532245601372,4.53618942178855));
#85599=CARTESIAN_POINT('Ctrl Pts',(-11.0122309001124,14.4548079929299,4.55742298544379));
#85600=CARTESIAN_POINT('Ctrl Pts',(-10.9513225714017,14.4590511195217,4.61335300566082));
#85601=CARTESIAN_POINT('Ctrl Pts',(-10.9109143426204,14.4616573752491,4.64664954367225));
#85602=CARTESIAN_POINT('Ctrl Pts',(-10.8129423107516,14.4676355668168,4.71892428685838));
#85603=CARTESIAN_POINT('Ctrl Pts',(-10.7542167048291,14.4709700364914,4.75610849349001));
#85604=CARTESIAN_POINT('Ctrl Pts',(-10.637943889477,14.4774618487418,4.81862731034578));
#85605=CARTESIAN_POINT('Ctrl Pts',(-10.5809737447922,14.480599439223,4.84470003270051));
#85606=CARTESIAN_POINT('Ctrl Pts',(-10.5157496791872,14.4843246169107,4.86963024443279));
#85607=CARTESIAN_POINT('Ctrl Pts',(-10.5089633353008,14.4847137833371,4.87216655587092));
#85608=CARTESIAN_POINT('Ctrl Pts',(-10.4988314715312,14.4852975254021,4.87586771160278));
#85609=CARTESIAN_POINT('Ctrl Pts',(-10.4954999970626,14.4854899029261,4.8770710036859));
#85610=CARTESIAN_POINT('Ctrl Pts',(-10.4895381110456,14.4858350080482,4.8791999360828));
#85611=CARTESIAN_POINT('Ctrl Pts',(-10.4869093906532,14.4859874631704,4.88013016451039));
#85612=CARTESIAN_POINT('Ctrl Pts',(-10.4812020876988,14.4863191069529,4.88213147902669));
#85613=CARTESIAN_POINT('Ctrl Pts',(-10.4781226231971,14.486498450168,4.88319977996017));
#85614=CARTESIAN_POINT('Ctrl Pts',(-10.4694721152723,14.4870033100668,4.8861683991773));
#85615=CARTESIAN_POINT('Ctrl Pts',(-10.4638932035743,14.4873301454291,4.88804538512558));
#85616=CARTESIAN_POINT('Ctrl Pts',(-10.4303269589742,14.4893033684728,4.8991135510081));
#85617=CARTESIAN_POINT('Ctrl Pts',(-10.402080427348,14.4909919828032,4.90749106858268));
#85618=CARTESIAN_POINT('Ctrl Pts',(-10.2439044071077,14.5005304652491,4.94925399066714));
#85619=CARTESIAN_POINT('Ctrl Pts',(-10.11011020097,14.5088311459879,4.96550634083251));
#85620=CARTESIAN_POINT('Ctrl Pts',(-9.92610919725075,14.5195409137585,4.96248360021393));
#85621=CARTESIAN_POINT('Ctrl Pts',(-9.87632817384542,14.5223770220857,4.95911762376294));
#85622=CARTESIAN_POINT('Ctrl Pts',(-9.81717708968965,14.525671299234,4.95206824098857));
#85623=CARTESIAN_POINT('Ctrl Pts',(-9.8075540342621,14.5262048853686,4.95082423114348));
#85624=CARTESIAN_POINT('Ctrl Pts',(-9.79176722072903,14.5270765139875,4.94862357163731));
#85625=CARTESIAN_POINT('Ctrl Pts',(-9.78559604731992,14.5274163009371,4.9477230706959));
#85626=CARTESIAN_POINT('Ctrl Pts',(-9.77450270460006,14.528025463329,4.94603183570263));
#85627=CARTESIAN_POINT('Ctrl Pts',(-9.7695784877446,14.5282952809169,4.94525535032436));
#85628=CARTESIAN_POINT('Ctrl Pts',(-9.75908595454679,14.528868999375,4.94354582466448));
#85629=CARTESIAN_POINT('Ctrl Pts',(-9.75351886525646,14.5291726726454,4.9426056899389));
#85630=CARTESIAN_POINT('Ctrl Pts',(-9.73849591853881,14.5299902478676,4.93997920795611));
#85631=CARTESIAN_POINT('Ctrl Pts',(-9.72905090307435,14.5305022276834,4.93823193426739));
#85632=CARTESIAN_POINT('Ctrl Pts',(-9.68075406032457,14.5331105805803,4.92880463579633));
#85633=CARTESIAN_POINT('Ctrl Pts',(-9.64220661203632,14.5351597143119,4.9196425286188));
#85634=CARTESIAN_POINT('Ctrl Pts',(-9.46031577036151,14.5447476923221,4.86852919701771));
#85635=CARTESIAN_POINT('Ctrl Pts',(-9.32360851419405,14.5516141937201,4.80637523549079));
#85636=CARTESIAN_POINT('Ctrl Pts',(-9.17648226743139,14.5606161694766,4.71010516029549));
#85637=CARTESIAN_POINT('Ctrl Pts',(-9.15468495970759,14.5620000084049,4.69498044499086));
#85638=CARTESIAN_POINT('Ctrl Pts',(-9.12895134599161,14.5637104750145,4.67606793141302));
#85639=CARTESIAN_POINT('Ctrl Pts',(-9.12460849974417,14.5640018424251,4.67283897292114));
#85640=CARTESIAN_POINT('Ctrl Pts',(-9.11750917138189,14.5644827846558,4.66749913952317));
#85641=CARTESIAN_POINT('Ctrl Pts',(-9.11474207678029,14.5646714087241,4.66540238211958));
#85642=CARTESIAN_POINT('Ctrl Pts',(-9.10976940707364,14.5650125416893,4.6616064278575));
#85643=CARTESIAN_POINT('Ctrl Pts',(-9.10756119813874,14.5651648048303,4.6599107666315));
#85644=CARTESIAN_POINT('Ctrl Pts',(-9.10273451029718,14.565499334031,4.65618245910433));
#85645=CARTESIAN_POINT('Ctrl Pts',(-9.10011812531457,14.5656817770791,4.65414723883737));
#85646=CARTESIAN_POINT('Ctrl Pts',(-9.09267302128851,14.5662040394351,4.64831517295536));
#85647=CARTESIAN_POINT('Ctrl Pts',(-9.08786132198781,14.5665453235079,4.64449683795408));
#85648=CARTESIAN_POINT('Ctrl Pts',(-9.05614154474927,14.5688192997372,4.61899845294539));
#85649=CARTESIAN_POINT('Ctrl Pts',(-9.02998643967149,14.5708101362053,4.59640304686016));
#85650=CARTESIAN_POINT('Ctrl Pts',(-8.93229728227649,14.5786255458622,4.50577606571329));
#85651=CARTESIAN_POINT('Ctrl Pts',(-8.86691415133092,14.5846662181041,4.431499639084));
#85652=CARTESIAN_POINT('Ctrl Pts',(-8.76419674668663,14.5951667291323,4.28783929512394));
#85653=CARTESIAN_POINT('Ctrl Pts',(-8.72401580447861,14.5996789223421,4.22094922021483));
#85654=CARTESIAN_POINT('Ctrl Pts',(-8.68461007668905,14.6045865336568,4.14163458794331));
#85655=CARTESIAN_POINT('Ctrl Pts',(-8.67997718897416,14.6051728912806,4.13204855951779));
#85656=CARTESIAN_POINT('Ctrl Pts',(-8.67270556135671,14.6061087742783,4.11657387403076));
#85657=CARTESIAN_POINT('Ctrl Pts',(-8.67000050096529,14.6064605643365,4.11071695851973));
#85658=CARTESIAN_POINT('Ctrl Pts',(-8.66525833512971,14.6070838970414,4.10026841300552));
#85659=CARTESIAN_POINT('Ctrl Pts',(-8.66320598738009,14.6073559562996,4.09568384927746));
#85660=CARTESIAN_POINT('Ctrl Pts',(-8.65896955319943,14.6079224076401,4.08608827804928));
#85661=CARTESIAN_POINT('Ctrl Pts',(-8.65678985375869,14.6082166477332,4.0810754108215));
#85662=CARTESIAN_POINT('Ctrl Pts',(-8.65117797699607,14.6089816451301,4.06796891145177));
#85663=CARTESIAN_POINT('Ctrl Pts',(-8.64779052234515,14.6094508918143,4.05985629156161));
#85664=CARTESIAN_POINT('Ctrl Pts',(-8.63307985704552,14.6115231092877,4.02371315852638));
#85665=CARTESIAN_POINT('Ctrl Pts',(-8.62255324408652,14.6130994633753,3.99536527170792));
#85666=CARTESIAN_POINT('Ctrl Pts',(-8.59633988427138,14.6173180459498,3.91745774302727));
#85667=CARTESIAN_POINT('Ctrl Pts',(-8.58240226533197,14.6199076461924,3.86735528846226));
#85668=CARTESIAN_POINT('Ctrl Pts',(-8.54827221938631,14.6276564855475,3.71333093641444));
#85669=CARTESIAN_POINT('Ctrl Pts',(-8.53665383458155,14.6326599237121,3.60787967298341));
#85670=CARTESIAN_POINT('Ctrl Pts',(-8.5364603238373,14.6395172610135,3.47350180698756));
#85671=CARTESIAN_POINT('Ctrl Pts',(-8.53725783843772,14.6410057726106,3.44490287714756));
#85672=CARTESIAN_POINT('Ctrl Pts',(-8.53920929031795,14.6428334658408,3.41081799661619));
#85673=CARTESIAN_POINT('Ctrl Pts',(-8.53955726092556,14.6431315613034,3.40529027951902));
#85674=CARTESIAN_POINT('Ctrl Pts',(-8.54017703797334,14.6436213635055,3.39626237895485));
#85675=CARTESIAN_POINT('Ctrl Pts',(-8.54043007975871,14.643812058964,3.39276091252988));
#85676=CARTESIAN_POINT('Ctrl Pts',(-8.54090654845293,14.6441553686145,3.38648210185648));
#85677=CARTESIAN_POINT('Ctrl Pts',(-8.5411253105693,14.6443077222738,3.3837044544901));
#85678=CARTESIAN_POINT('Ctrl Pts',(-8.54161914373234,14.6446405906303,3.37765496188581));
#85679=CARTESIAN_POINT('Ctrl Pts',(-8.54189728981065,14.6448212696088,3.37438345498683));
#85680=CARTESIAN_POINT('Ctrl Pts',(-8.54271451798922,14.6453336015689,3.36513996407526));
#85681=CARTESIAN_POINT('Ctrl Pts',(-8.54327929111791,14.6456666350909,3.35917038967585));
#85682=CARTESIAN_POINT('Ctrl Pts',(-8.5470416019305,14.6477614652763,3.32185061091354));
#85683=CARTESIAN_POINT('Ctrl Pts',(-8.55121413370243,14.6495716108706,3.29060913552611));
#85684=CARTESIAN_POINT('Ctrl Pts',(-8.58450789119584,14.6614149673323,3.09073812546877));
#85685=CARTESIAN_POINT('Ctrl Pts',(-8.64200738318631,14.6720532122382,2.92816398274606));
#85686=CARTESIAN_POINT('Ctrl Pts',(-8.73496465313359,14.6826184803685,2.76391215063134));
#85687=CARTESIAN_POINT('Ctrl Pts',(-8.74387545889991,14.6835905392957,2.74880699841342));
#85688=CARTESIAN_POINT('Ctrl Pts',(-8.75691862071611,14.6849577868378,2.72757823647388));
#85689=CARTESIAN_POINT('Ctrl Pts',(-8.76082891077137,14.6853609614944,2.72132053404061));
#85690=CARTESIAN_POINT('Ctrl Pts',(-8.76727969667483,14.6860153229084,2.71116889282431));
#85691=CARTESIAN_POINT('Ctrl Pts',(-8.76979168302489,14.6862675491686,2.70725706599327));
#85692=CARTESIAN_POINT('Ctrl Pts',(-8.77510744121103,14.6867959317582,2.6990651408183));
#85693=CARTESIAN_POINT('Ctrl Pts',(-8.777915109139,14.6870719393491,2.69478763690839));
#85694=CARTESIAN_POINT('Ctrl Pts',(-8.78468621927589,14.687730325603,2.68458879476031));
#85695=CARTESIAN_POINT('Ctrl Pts',(-8.78867060660366,14.6881119180431,2.67868147325002));
#85696=CARTESIAN_POINT('Ctrl Pts',(-8.80246001185854,14.6894130192345,2.65855569364177));
#85697=CARTESIAN_POINT('Ctrl Pts',(-8.81247369874298,14.6903246759255,2.64448152507192));
#85698=CARTESIAN_POINT('Ctrl Pts',(-8.83710747201905,14.6924921958117,2.61112510054536));
#85699=CARTESIAN_POINT('Ctrl Pts',(-8.85196134733785,14.693739186876,2.59202150273576));
#85700=CARTESIAN_POINT('Ctrl Pts',(-8.91167032814787,14.6985404741856,2.51903889311095));
#85701=CARTESIAN_POINT('Ctrl Pts',(-8.95990081226546,14.7019723429171,2.46804033037075));
#85702=CARTESIAN_POINT('Ctrl Pts',(-9.08653934581786,14.7103271899521,2.35206849377786));
#85703=CARTESIAN_POINT('Ctrl Pts',(-9.16840958621896,14.7151992592941,2.29144334789854));
#85704=CARTESIAN_POINT('Ctrl Pts',(-9.2650789484952,14.7211301026905,2.23436287598538));
#85705=CARTESIAN_POINT('Ctrl Pts',(-9.27433305141891,14.7216996731456,2.22903432455242));
#85706=CARTESIAN_POINT('Ctrl Pts',(-9.28736587405346,14.722505504595,2.22171870624835));
#85707=CARTESIAN_POINT('Ctrl Pts',(-9.29109645596594,14.7227365883625,2.21964605372261));
#85708=CARTESIAN_POINT('Ctrl Pts',(-9.29712740604751,14.7231109231526,2.21632979127867));
#85709=CARTESIAN_POINT('Ctrl Pts',(-9.29942216390929,14.7232535326876,2.21507596199455));
#85710=CARTESIAN_POINT('Ctrl Pts',(-9.30425847568518,14.7235544853693,2.21245026390786));
#85711=CARTESIAN_POINT('Ctrl Pts',(-9.30680073996476,14.7237129157286,2.21107976312565));
#85712=CARTESIAN_POINT('Ctrl Pts',(-9.31304096385428,14.7241023321206,2.20773954346345));
#85713=CARTESIAN_POINT('Ctrl Pts',(-9.31674334226656,14.724333834119,2.20577817062005));
#85714=CARTESIAN_POINT('Ctrl Pts',(-9.33018360487602,14.7251757378988,2.19873179903315));
#85715=CARTESIAN_POINT('Ctrl Pts',(-9.3399699972636,14.725791624287,2.19374071688748));
#85716=CARTESIAN_POINT('Ctrl Pts',(-9.40323453775983,14.7297868550527,2.16236809436687));
#85717=CARTESIAN_POINT('Ctrl Pts',(-9.45822239713232,14.7333203086661,2.13916794981007));
#85718=CARTESIAN_POINT('Ctrl Pts',(-9.57533236702496,14.7407639914435,2.0979826844455));
#85719=CARTESIAN_POINT('Ctrl Pts',(-9.637549589396,14.7446721582833,2.08062505308544));
#85720=CARTESIAN_POINT('Ctrl Pts',(-9.7787372410444,14.7532570106408,2.05112833336713));
#85721=CARTESIAN_POINT('Ctrl Pts',(-9.85797479411013,14.7578795224073,2.04122710117559));
#85722=CARTESIAN_POINT('Ctrl Pts',(-9.9483013197222,14.7628896489768,2.03737445817805));
#85723=CARTESIAN_POINT('Ctrl Pts',(-9.95897257273528,14.7634776719302,2.03703623153573));
#85724=CARTESIAN_POINT('Ctrl Pts',(-9.97610540086514,14.7644156886124,2.03668081748006));
#85725=CARTESIAN_POINT('Ctrl Pts',(-9.98256491375617,14.7647679634693,2.03658959910783));
#85726=CARTESIAN_POINT('Ctrl Pts',(-9.99404893751969,14.7653918519988,2.03650347547258));
#85727=CARTESIAN_POINT('Ctrl Pts',(-9.99907318599637,14.7656639854529,2.03649166919401));
#85728=CARTESIAN_POINT('Ctrl Pts',(-10.0095594164535,14.7662302908705,2.03652102817245));
#85729=CARTESIAN_POINT('Ctrl Pts',(-10.015021314684,14.7665243127017,2.03656689779099));
#85730=CARTESIAN_POINT('Ctrl Pts',(-10.0292542554504,14.7672880893945,2.03676611895257));
#85731=CARTESIAN_POINT('Ctrl Pts',(-10.0380244745551,14.7677563427297,2.03696775635065));
#85732=CARTESIAN_POINT('Ctrl Pts',(-10.0768206162417,14.7698177023062,2.0382088198072));
#85733=CARTESIAN_POINT('Ctrl Pts',(-10.1068132628365,14.7713845428022,2.04009385450433));
#85734=CARTESIAN_POINT('Ctrl Pts',(-10.1879956941611,14.7755702437649,2.04771167493886));
#85735=CARTESIAN_POINT('Ctrl Pts',(-10.2389760149104,14.7781375505845,2.05522501010984));
#85736=CARTESIAN_POINT('Ctrl Pts',(-10.3938242997306,14.7858996734032,2.08646871710028));
#85737=CARTESIAN_POINT('Ctrl Pts',(-10.4955722327321,14.7909329752407,2.11885092764405));
#85738=CARTESIAN_POINT('Ctrl Pts',(-10.6190668988083,14.7978257449656,2.17357334855364));
#85739=CARTESIAN_POINT('Ctrl Pts',(-10.6448877105855,14.7993150899003,2.18593336794324));
#85740=CARTESIAN_POINT('Ctrl Pts',(-10.67525222424,14.8011437163814,2.20157889277397));
#85741=CARTESIAN_POINT('Ctrl Pts',(-10.6801621210611,14.8014418635582,2.2041441341138));
#85742=CARTESIAN_POINT('Ctrl Pts',(-10.6881597827738,14.8019317339091,2.20838059400114));
#85743=CARTESIAN_POINT('Ctrl Pts',(-10.6912563513537,14.8021224453322,2.21003518157764));
#85744=CARTESIAN_POINT('Ctrl Pts',(-10.6966618203515,14.8024572339183,2.21294853500151));
#85745=CARTESIAN_POINT('Ctrl Pts',(-10.6989733159429,14.8026010018738,2.21420239968839));
#85746=CARTESIAN_POINT('Ctrl Pts',(-10.701290635301,14.802745745833,2.21546751892041));
#85747=CARTESIAN_POINT('Ctrl Pts',(-10.7012998170609,14.802746319352,2.2154725317457));
#85748=CARTESIAN_POINT('Ctrl Pts',(-10.7013179991876,14.8027474550787,2.21548245861698));
#85749=CARTESIAN_POINT('Ctrl Pts',(-10.7013269995107,14.8027480172833,2.21548737263408));
#85750=CARTESIAN_POINT('Ctrl Pts',(-10.7013442395075,14.8027490941964,2.21549678560237));
#85751=CARTESIAN_POINT('Ctrl Pts',(-10.7013524792389,14.8027496089069,2.21550128456522));
#85752=CARTESIAN_POINT('Ctrl Pts',(-10.7013689210014,14.8027506359884,2.2155102621116));
#85753=CARTESIAN_POINT('Ctrl Pts',(-10.7013771231267,14.8027511483653,2.2155147407456));
#85754=CARTESIAN_POINT('Ctrl Pts',(-10.7013934902058,14.8027521708122,2.21552367792028));
#85755=CARTESIAN_POINT('Ctrl Pts',(-10.7014016550708,14.8027526808767,2.21552813641152));
#85756=CARTESIAN_POINT('Ctrl Pts',(-10.7014179476104,14.8027536986975,2.21553703328753));
#85757=CARTESIAN_POINT('Ctrl Pts',(-10.7014260753742,14.8027542064594,2.21554147172013));
#85758=CARTESIAN_POINT('Ctrl Pts',(-10.7014422938674,14.8027552196846,2.21555032856131));
#85759=CARTESIAN_POINT('Ctrl Pts',(-10.701450384669,14.8027557251524,2.21555474700838));
#85760=CARTESIAN_POINT('Ctrl Pts',(-10.701466529898,14.8027567338304,2.21556356423642));
#85761=CARTESIAN_POINT('Ctrl Pts',(-10.701474584129,14.8027572370283,2.21556796290921));
#85762=CARTESIAN_POINT('Ctrl Pts',(-10.7014906560814,14.8027582411579,2.21557674051193));
#85763=CARTESIAN_POINT('Ctrl Pts',(-10.7014986738488,14.8027587420924,2.21558111946614));
#85764=CARTESIAN_POINT('Ctrl Pts',(-10.70151467328,14.8027597417204,2.21558985785088));
#85765=CARTESIAN_POINT('Ctrl Pts',(-10.7015226548932,14.8027602404107,2.21559421725288));
#85766=CARTESIAN_POINT('Ctrl Pts',(-10.7043322685578,14.8029357873097,2.21712880762796));
#85767=CARTESIAN_POINT('Ctrl Pts',(-10.707128858977,14.8031114175166,2.2186681861633));
#85768=CARTESIAN_POINT('Ctrl Pts',(-10.7148740617645,14.8036002729374,2.22296459877992));
#85769=CARTESIAN_POINT('Ctrl Pts',(-10.7198116819565,14.8039147013131,2.22574120347394));
#85770=CARTESIAN_POINT('Ctrl Pts',(-10.7308711094175,14.8046250161681,2.23204511538023));
#85771=CARTESIAN_POINT('Ctrl Pts',(-10.7369837093925,14.8050218117944,2.23558820939854));
#85772=CARTESIAN_POINT('Ctrl Pts',(-10.7560473149775,14.8062719456654,2.24682339508197));
#85773=CARTESIAN_POINT('Ctrl Pts',(-10.7689050272972,14.8071335218242,2.25467105880305));
#85774=CARTESIAN_POINT('Ctrl Pts',(-10.820134098984,14.8106340253724,2.28703437677541));
#85775=CARTESIAN_POINT('Ctrl Pts',(-10.8574712183705,14.8133399085539,2.31313516009308));
#85776=CARTESIAN_POINT('Ctrl Pts',(-10.9439649612743,14.8198886711239,2.37981340534427));
#85777=CARTESIAN_POINT('Ctrl Pts',(-10.9918112571779,14.8237457275513,2.42194682535507));
#85778=CARTESIAN_POINT('Ctrl Pts',(-11.0935244932582,14.8323265126232,2.52403663086385));
#85779=CARTESIAN_POINT('Ctrl Pts',(-11.1455012830883,14.8369923758831,2.58559832503061));
#85780=CARTESIAN_POINT('Ctrl Pts',(-11.1983594793626,14.8420425957085,2.6598327609473));
#85781=CARTESIAN_POINT('Ctrl Pts',(-11.2044620066647,14.8426311485935,2.66860495889492));
#85782=CARTESIAN_POINT('Ctrl Pts',(-11.2141004248147,14.843569844042,2.68278878118939));
#85783=CARTESIAN_POINT('Ctrl Pts',(-11.2176974137151,14.8439222729796,2.6881582492922));
#85784=CARTESIAN_POINT('Ctrl Pts',(-11.2240275146196,14.8445463381623,2.6977443425));
#85785=CARTESIAN_POINT('Ctrl Pts',(-11.2267746837641,14.8448184951978,2.70195152234554));
#85786=CARTESIAN_POINT('Ctrl Pts',(-11.2324621204086,14.8453847544427,2.71076037176514));
#85787=CARTESIAN_POINT('Ctrl Pts',(-11.2353984131859,14.8456787071084,2.71536452359918));
#85788=CARTESIAN_POINT('Ctrl Pts',(-11.2429811246269,14.8464420973229,2.72740241976261));
#85789=CARTESIAN_POINT('Ctrl Pts',(-11.2475866815155,14.8469100362181,2.73486172898027));
#85790=CARTESIAN_POINT('Ctrl Pts',(-11.2676476485209,14.8489679732402,2.76801587532363));
#85791=CARTESIAN_POINT('Ctrl Pts',(-11.282378854405,14.8505318156998,2.79414168728199));
#85792=CARTESIAN_POINT('Ctrl Pts',(-11.3201296659054,14.8547071820405,2.86618128859346));
#85793=CARTESIAN_POINT('Ctrl Pts',(-11.3415529291829,14.8572674871752,2.91288435927259));
#85794=CARTESIAN_POINT('Ctrl Pts',(-11.3975992591731,14.8647407067194,3.05424982825733));
#85795=CARTESIAN_POINT('Ctrl Pts',(-11.4249527831082,14.869514882211,3.15145474985847));
#85796=CARTESIAN_POINT('Ctrl Pts',(-11.4456619666599,14.8756690960264,3.2712449825051));
#85797=CARTESIAN_POINT('Ctrl Pts',(-11.4487754533726,14.8767390071556,3.29187264875632));
#85798=CARTESIAN_POINT('Ctrl Pts',(-11.4534716577475,14.878653668477,3.32823763046049));
#85799=CARTESIAN_POINT('Ctrl Pts',(-11.4552421594919,14.8794901011025,3.34394748275528));
#85800=CARTESIAN_POINT('Ctrl Pts',(-11.4572368589926,14.8806084314415,3.36465615721395));
#85801=CARTESIAN_POINT('Ctrl Pts',(-11.4576904684699,14.880878356399,3.36963238265516));
#85802=CARTESIAN_POINT('Ctrl Pts',(-11.4583810221683,14.881316004209,3.37766265046703));
#85803=CARTESIAN_POINT('Ctrl Pts',(-11.4586338812994,14.8814828548404,3.380715328387));
#85804=CARTESIAN_POINT('Ctrl Pts',(-11.459089437443,14.8817963158792,3.38643324368223));
#85805=CARTESIAN_POINT('Ctrl Pts',(-11.4592944182874,14.8819427981857,3.38909826453622));
#85806=CARTESIAN_POINT('Ctrl Pts',(-11.4596981435806,14.8822427915594,3.39454222776246));
#85807=CARTESIAN_POINT('Ctrl Pts',(-11.4598962559606,14.8823963365641,3.39732121121951));
#85808=CARTESIAN_POINT('Ctrl Pts',(-11.4603396224605,14.8827552963578,3.40380127201299));
#85809=CARTESIAN_POINT('Ctrl Pts',(-11.4605787425555,14.8829610378778,3.40750273309786));
#85810=CARTESIAN_POINT('Ctrl Pts',(-11.4614403784447,14.8837515254349,3.42167787003378));
#85811=CARTESIAN_POINT('Ctrl Pts',(-11.4619643106131,14.8843412870754,3.43215696343751));
#85812=CARTESIAN_POINT('Ctrl Pts',(-11.4631173255255,14.8860090843852,3.46155296687572));
#85813=CARTESIAN_POINT('Ctrl Pts',(-11.4634921491228,14.887098285449,3.48047715784938));
#85814=CARTESIAN_POINT('Ctrl Pts',(-11.4634998779574,14.8881996490159,3.4994023223159));
#85815=CARTESIAN_POINT('Ctrl Pts',(-11.4634998771631,14.8881995360101,3.49940038049047));
#85816=CARTESIAN_POINT('Ctrl Pts',(-11.4634999590548,14.8882111678261,3.49960025472328));
#85817=CARTESIAN_POINT('Ctrl Pts',(-11.4635,14.8882228009326,3.49980012789184));
#85818=CARTESIAN_POINT('Ctrl Pts',(-11.4635,14.8882344353249,3.49999999998375));
#85819=CARTESIAN_POINT('Origin',(-10.,13.2,3.5));
#85820=CARTESIAN_POINT('',(-11.4635,15.4596442608852,3.50000000000481));
#85821=CARTESIAN_POINT('',(-11.4635,15.3905155741067,3.49999999999573));
#85822=CARTESIAN_POINT('',(-11.4635,13.2,3.5));
#85823=CARTESIAN_POINT('Ctrl Pts',(-11.4635,15.4596442608852,3.50000000000481));
#85824=CARTESIAN_POINT('Ctrl Pts',(-11.4635,15.4596305239997,3.49972896597656));
#85825=CARTESIAN_POINT('Ctrl Pts',(-11.4634999247368,15.4596167888801,3.49945793106095));
#85826=CARTESIAN_POINT('Ctrl Pts',(-11.4634551756689,15.4555356919543,3.41891492979269));
#85827=CARTESIAN_POINT('Ctrl Pts',(-11.4568063299427,15.4516448954757,3.33877945007402));
#85828=CARTESIAN_POINT('Ctrl Pts',(-11.429541796671,15.4435734829384,3.1750591932718));
#85829=CARTESIAN_POINT('Ctrl Pts',(-11.4080682176578,15.4394039263173,3.09193536609401));
#85830=CARTESIAN_POINT('Ctrl Pts',(-11.37568177232,15.434289074522,3.00054101620579));
#85831=CARTESIAN_POINT('Ctrl Pts',(-11.3717894747857,15.4336877512384,2.98994780994598));
#85832=CARTESIAN_POINT('Ctrl Pts',(-11.3662217651065,15.4328442173318,2.97531970819412));
#85833=CARTESIAN_POINT('Ctrl Pts',(-11.3646501139149,15.4326078451764,2.97124543911044));
#85834=CARTESIAN_POINT('Ctrl Pts',(-11.3621016207484,15.4322272241544,2.96472590376175));
#85835=CARTESIAN_POINT('Ctrl Pts',(-11.3611363604048,15.4320836588598,2.9622761010461));
#85836=CARTESIAN_POINT('Ctrl Pts',(-11.3591055783895,15.4317828303336,2.9571625401835));
#85837=CARTESIAN_POINT('Ctrl Pts',(-11.3580388329525,15.4316254914923,2.95449930457078));
#85838=CARTESIAN_POINT('Ctrl Pts',(-11.3554301908,15.4312424058033,2.94804164728486));
#85839=CARTESIAN_POINT('Ctrl Pts',(-11.3538801878438,15.4310161798071,2.94425054080497));
#85840=CARTESIAN_POINT('Ctrl Pts',(-11.3483458887013,15.4302134501606,2.93087492388027));
#85841=CARTESIAN_POINT('Ctrl Pts',(-11.3442756572806,15.4296320953399,2.92132657522915));
#85842=CARTESIAN_POINT('Ctrl Pts',(-11.3187058276955,15.4260374273143,2.86306823339446));
#85843=CARTESIAN_POINT('Ctrl Pts',(-11.2946644573736,15.4228997181584,2.81552205115584));
#85844=CARTESIAN_POINT('Ctrl Pts',(-11.2192978538469,15.4138764482001,2.68471034206742));
#85845=CARTESIAN_POINT('Ctrl Pts',(-11.1621408427373,15.4079255343839,2.60511683750367));
#85846=CARTESIAN_POINT('Ctrl Pts',(-11.0851725098982,15.4011224105358,2.51787034808266));
#85847=CARTESIAN_POINT('Ctrl Pts',(-11.0726058361066,15.4000433637595,2.50416126398622));
#85848=CARTESIAN_POINT('Ctrl Pts',(-11.033286241938,15.396764042071,2.46287527300432));
#85849=CARTESIAN_POINT('Ctrl Pts',(-11.0057048751487,15.3945963352812,2.43610797192771));
#85850=CARTESIAN_POINT('Ctrl Pts',(-10.9697798968078,15.3919322525683,2.40389056994274));
#85851=CARTESIAN_POINT('Ctrl Pts',(-10.9623936073968,15.3913924841453,2.39739967259808));
#85852=CARTESIAN_POINT('Ctrl Pts',(-10.9505835215266,15.3905418282193,2.38723034516482));
#85853=CARTESIAN_POINT('Ctrl Pts',(-10.9462025773107,15.3902289291237,2.38350278991417));
#85854=CARTESIAN_POINT('Ctrl Pts',(-10.9379937718405,15.3896475099769,2.37660129152837));
#85855=CARTESIAN_POINT('Ctrl Pts',(-10.9341715026429,15.3893787281474,2.37342085111512));
#85856=CARTESIAN_POINT('Ctrl Pts',(-10.925636172017,15.3887827925637,2.36639206592505));
#85857=CARTESIAN_POINT('Ctrl Pts',(-10.9209151557293,15.3884560341586,2.36255349636957));
#85858=CARTESIAN_POINT('Ctrl Pts',(-10.9070813967356,15.387506751398,2.35144811435346));
#85859=CARTESIAN_POINT('Ctrl Pts',(-10.89790550092,15.3868873677109,2.34426048947077));
#85860=CARTESIAN_POINT('Ctrl Pts',(-10.8132001998544,15.3812600682219,2.27952725110197));
#85861=CARTESIAN_POINT('Ctrl Pts',(-10.7323215298924,15.3765576184053,2.22934803547161));
#85862=CARTESIAN_POINT('Ctrl Pts',(-10.5479634960048,15.3665388088277,2.13845841619453));
#85863=CARTESIAN_POINT('Ctrl Pts',(-10.4435765171853,15.3612785158233,2.100967244196));
#85864=CARTESIAN_POINT('Ctrl Pts',(-10.3263507817662,15.3549030713687,2.07331666067449));
#85865=CARTESIAN_POINT('Ctrl Pts',(-10.3166964270464,15.3543745127806,2.07114257325522));
#85866=CARTESIAN_POINT('Ctrl Pts',(-10.3033768970087,15.353639578052,2.06828473521485));
#85867=CARTESIAN_POINT('Ctrl Pts',(-10.2997298299482,15.3534377554188,2.06751678213002));
#85868=CARTESIAN_POINT('Ctrl Pts',(-10.2934814295339,15.3530909135124,2.06622597988029));
#85869=CARTESIAN_POINT('Ctrl Pts',(-10.2908815155282,15.3529462798142,2.06569625464344));
#85870=CARTESIAN_POINT('Ctrl Pts',(-10.2854832094401,15.3526452905358,2.06461164625534));
#85871=CARTESIAN_POINT('Ctrl Pts',(-10.2826846335496,15.3524888706417,2.06405787498233));
#85872=CARTESIAN_POINT('Ctrl Pts',(-10.2759485397135,15.35211148098,2.06274541807741));
#85873=CARTESIAN_POINT('Ctrl Pts',(-10.2720094993891,15.3518900654938,2.06199472835211));
#85874=CARTESIAN_POINT('Ctrl Pts',(-10.2583896584571,15.3511220838221,2.05945706557036));
#85875=CARTESIAN_POINT('Ctrl Pts',(-10.2486941629726,15.3505711954585,2.05775162885507));
#85876=CARTESIAN_POINT('Ctrl Pts',(-10.1916598651684,15.347308968388,2.04831149121491));
#85877=CARTESIAN_POINT('Ctrl Pts',(-10.1439846718586,15.344495683007,2.04281070402325));
#85878=CARTESIAN_POINT('Ctrl Pts',(-10.0323325874114,15.3378307286899,2.03546095386668));
#85879=CARTESIAN_POINT('Ctrl Pts',(-9.9683288415689,15.3339543821337,2.03544649937339));
#85880=CARTESIAN_POINT('Ctrl Pts',(-9.87845763787296,15.3285593939951,2.04132171322294));
#85881=CARTESIAN_POINT('Ctrl Pts',(-9.85243560626152,15.3270024443801,2.04372402732658));
#85882=CARTESIAN_POINT('Ctrl Pts',(-9.75910427968921,15.3214500859481,2.05486774481952));
#85883=CARTESIAN_POINT('Ctrl Pts',(-9.69235238273318,15.3175439678568,2.06759190439752));
#85884=CARTESIAN_POINT('Ctrl Pts',(-9.61665193514905,15.313207843049,2.08756066769791));
#85885=CARTESIAN_POINT('Ctrl Pts',(-9.60661523569978,15.3126347443779,2.09032307199516));
#85886=CARTESIAN_POINT('Ctrl Pts',(-9.59040907124544,15.3117121451861,2.09497006566845));
#85887=CARTESIAN_POINT('Ctrl Pts',(-9.5842212169069,15.3113605369858,2.09678873626285));
#85888=CARTESIAN_POINT('Ctrl Pts',(-9.5732514801817,15.3107383317008,2.10009178253024));
#85889=CARTESIAN_POINT('Ctrl Pts',(-9.56846484210033,15.3104672135685,2.10155989585975));
#85890=CARTESIAN_POINT('Ctrl Pts',(-9.55841883704447,15.309898968704,2.10469760499573));
#85891=CARTESIAN_POINT('Ctrl Pts',(-9.55316118094456,15.3096020172258,2.10637244289861));
#85892=CARTESIAN_POINT('Ctrl Pts',(-9.53932394352627,15.3088215991895,2.11086668152395));
#85893=CARTESIAN_POINT('Ctrl Pts',(-9.53076069456945,15.308339760734,2.11373585321252));
#85894=CARTESIAN_POINT('Ctrl Pts',(-9.49128545836975,15.3061232001782,2.12736998012011));
#85895=CARTESIAN_POINT('Ctrl Pts',(-9.46071237375714,15.3044200112537,2.13909121415465));
#85896=CARTESIAN_POINT('Ctrl Pts',(-9.37662266987157,15.299749904531,2.17460920139484));
#85897=CARTESIAN_POINT('Ctrl Pts',(-9.32410197594008,15.2968518055122,2.20060682245706));
#85898=CARTESIAN_POINT('Ctrl Pts',(-9.20092772125547,15.2899143146875,2.27107227533048));
#85899=CARTESIAN_POINT('Ctrl Pts',(-9.13225019822145,15.2859278471301,2.31856495182274));
#85900=CARTESIAN_POINT('Ctrl Pts',(-9.03683473424141,15.2797146079092,2.39737676550485));
#85901=CARTESIAN_POINT('Ctrl Pts',(-9.00675942091175,15.2776402540572,2.4243895072629));
#85902=CARTESIAN_POINT('Ctrl Pts',(-8.97348035787536,15.2751558438626,2.45686681993499));
#85903=CARTESIAN_POINT('Ctrl Pts',(-8.96914456549895,15.2748282671382,2.46115136925395));
#85904=CARTESIAN_POINT('Ctrl Pts',(-8.9622641443726,15.2743019371378,2.46803596080709));
#85905=CARTESIAN_POINT('Ctrl Pts',(-8.95970217885161,15.2741044955695,2.47061866785246));
#85906=CARTESIAN_POINT('Ctrl Pts',(-8.9551826617476,15.2737535400496,2.47520887897217));
#85907=CARTESIAN_POINT('Ctrl Pts',(-8.95322121749009,15.2736003325114,2.47721248910089));
#85908=CARTESIAN_POINT('Ctrl Pts',(-8.94906370896963,15.2732736631797,2.48148386010979));
#85909=CARTESIAN_POINT('Ctrl Pts',(-8.94686925549387,15.273100089598,2.48375305677801));
#85910=CARTESIAN_POINT('Ctrl Pts',(-8.94092642347853,15.2726269485331,2.48993822228083));
#85911=CARTESIAN_POINT('Ctrl Pts',(-8.93719247159222,15.2723263103039,2.4938679058073));
#85912=CARTESIAN_POINT('Ctrl Pts',(-8.91813409800759,15.2707749253096,2.51414978148589));
#85913=CARTESIAN_POINT('Ctrl Pts',(-8.90316569275912,15.2694998891367,2.53083083402208));
#85914=CARTESIAN_POINT('Ctrl Pts',(-8.8594285966054,15.2656176851472,2.5818835794357));
#85915=CARTESIAN_POINT('Ctrl Pts',(-8.83185067574945,15.2629560089545,2.61723867634104));
#85916=CARTESIAN_POINT('Ctrl Pts',(-8.76571477293374,15.2560998208935,2.7105621294741));
#85917=CARTESIAN_POINT('Ctrl Pts',(-8.72958644884635,15.2518828934182,2.77012182467499));
#85918=CARTESIAN_POINT('Ctrl Pts',(-8.66329139191361,15.2432582374766,2.89935937343006));
#85919=CARTESIAN_POINT('Ctrl Pts',(-8.63402223335021,15.2388809762397,2.96927730756257));
#85920=CARTESIAN_POINT('Ctrl Pts',(-8.60696726604364,15.2340997210999,3.0512190044596));
#85921=CARTESIAN_POINT('Ctrl Pts',(-8.60375370267395,15.2335160378211,3.06131917599875));
#85922=CARTESIAN_POINT('Ctrl Pts',(-8.59876543850539,15.2325836435224,3.07760755540805));
#85923=CARTESIAN_POINT('Ctrl Pts',(-8.59692139169167,15.2322326936642,3.08377398647471));
#85924=CARTESIAN_POINT('Ctrl Pts',(-8.59371173635364,15.2316103979543,3.09477072777387));
#85925=CARTESIAN_POINT('Ctrl Pts',(-8.59233019510439,15.231338540544,3.09959624777577));
#85926=CARTESIAN_POINT('Ctrl Pts',(-8.58949485627215,15.2307720609224,3.10969573881254));
#85927=CARTESIAN_POINT('Ctrl Pts',(-8.58804574758886,15.2304775933667,3.11497095304563));
#85928=CARTESIAN_POINT('Ctrl Pts',(-8.58433856725694,15.2297110266837,3.12876868738873));
#85929=CARTESIAN_POINT('Ctrl Pts',(-8.58212785014757,15.2292404507844,3.13730377603917));
#85930=CARTESIAN_POINT('Ctrl Pts',(-8.57261337882318,15.2271526046165,3.17545406619381));
#85931=CARTESIAN_POINT('Ctrl Pts',(-8.56615913515251,15.2255624648734,3.20527440513749));
#85932=CARTESIAN_POINT('Ctrl Pts',(-8.55111580171925,15.2212957506551,3.28706814570617));
#85933=CARTESIAN_POINT('Ctrl Pts',(-8.54439223253082,15.2186734097962,3.33933888104768));
#85934=CARTESIAN_POINT('Ctrl Pts',(-8.53271469506209,15.2109152816151,3.49694491628077));
#85935=CARTESIAN_POINT('Ctrl Pts',(-8.53630096204094,15.2059294778514,3.60255235812155));
#85936=CARTESIAN_POINT('Ctrl Pts',(-8.55515876038345,15.1991151490045,3.73463556914109));
#85937=CARTESIAN_POINT('Ctrl Pts',(-8.55992412777462,15.1976536733168,3.76230009026063));
#85938=CARTESIAN_POINT('Ctrl Pts',(-8.5665717899392,15.1958563169162,3.79520523106249));
#85939=CARTESIAN_POINT('Ctrl Pts',(-8.56769246332606,15.1955599743587,3.80059554273705));
#85940=CARTESIAN_POINT('Ctrl Pts',(-8.56957524666501,15.195072512928,3.80940188176442));
#85941=CARTESIAN_POINT('Ctrl Pts',(-8.57031925367067,15.1948823896445,3.81282177425315));
#85942=CARTESIAN_POINT('Ctrl Pts',(-8.57167725771477,15.1945397342874,3.81895791075269));
#85943=CARTESIAN_POINT('Ctrl Pts',(-8.57228674636658,15.1943874589618,3.82167510033378));
#85944=CARTESIAN_POINT('Ctrl Pts',(-8.57363314941225,15.1940543189583,3.82759835020923));
#85945=CARTESIAN_POINT('Ctrl Pts',(-8.57437310994154,15.1938732871037,3.83080362969389));
#85946=CARTESIAN_POINT('Ctrl Pts',(-8.5764997290435,15.1933588017598,3.83987581880031));
#85947=CARTESIAN_POINT('Ctrl Pts',(-8.57791182445659,15.1930239490981,3.84573662232813));
#85948=CARTESIAN_POINT('Ctrl Pts',(-8.58709103329239,15.1908898132808,3.88282643978772));
#85949=CARTESIAN_POINT('Ctrl Pts',(-8.59584967683019,15.1890401039775,3.91379873525406));
#85950=CARTESIAN_POINT('Ctrl Pts',(-8.62968671575224,15.1825226835892,4.01995498778359));
#85951=CARTESIAN_POINT('Ctrl Pts',(-8.65984367379001,15.1777083807406,4.09337346073131));
#85952=CARTESIAN_POINT('Ctrl Pts',(-8.74113151012844,15.1669527749925,4.25303920240693));
#85953=CARTESIAN_POINT('Ctrl Pts',(-8.79547653613902,15.1610858880768,4.33722594648556));
#85954=CARTESIAN_POINT('Ctrl Pts',(-8.86464691593975,15.1549567769307,4.42353614521159));
#85955=CARTESIAN_POINT('Ctrl Pts',(-8.87139665549476,15.1543703086505,4.43177257750891));
#85956=CARTESIAN_POINT('Ctrl Pts',(-8.88237880792422,15.1534343455758,4.44487921608996));
#85957=CARTESIAN_POINT('Ctrl Pts',(-8.88655449133425,15.1530825845425,4.44979627450981));
#85958=CARTESIAN_POINT('Ctrl Pts',(-8.8940382259944,15.1524593604496,4.45849153317498));
#85959=CARTESIAN_POINT('Ctrl Pts',(-8.89733344966403,15.1521873805266,4.46228059544641));
#85960=CARTESIAN_POINT('Ctrl Pts',(-8.90425456370589,15.1516211520048,4.47015670816005));
#85961=CARTESIAN_POINT('Ctrl Pts',(-8.90788397529257,15.151327054929,4.4742405705148));
#85962=CARTESIAN_POINT('Ctrl Pts',(-8.91740831308821,15.15056255699,4.48483737510305));
#85963=CARTESIAN_POINT('Ctrl Pts',(-8.92333920827098,15.1500936639218,4.4913177896407));
#85964=CARTESIAN_POINT('Ctrl Pts',(-8.94990532124871,15.148024324217,4.51982567745601));
#85965=CARTESIAN_POINT('Ctrl Pts',(-8.97116145693098,15.1464504051846,4.5412658961279));
#85966=CARTESIAN_POINT('Ctrl Pts',(-9.03069252501514,15.1422399951761,4.59770834599292));
#85967=CARTESIAN_POINT('Ctrl Pts',(-9.07018946038228,15.1396558716182,4.63135914252011));
#85968=CARTESIAN_POINT('Ctrl Pts',(-9.19486868036149,15.1319477799415,4.72663505465746));
#85969=CARTESIAN_POINT('Ctrl Pts',(-9.28496457063728,15.1269772920335,4.78124582763346));
#85970=CARTESIAN_POINT('Ctrl Pts',(-9.4067730171197,15.1201240747427,4.83820014783875));
#85971=CARTESIAN_POINT('Ctrl Pts',(-9.43379323321419,15.1185945897375,4.84985464223194));
#85972=CARTESIAN_POINT('Ctrl Pts',(-9.46633703910955,15.1167210616185,4.86274256060889));
#85973=CARTESIAN_POINT('Ctrl Pts',(-9.47154133525394,15.116420512928,4.86476916728659));
#85974=CARTESIAN_POINT('Ctrl Pts',(-9.48004818434357,15.1159275165333,4.86802586915334));
#85975=CARTESIAN_POINT('Ctrl Pts',(-9.48334385371099,15.1157361028238,4.8692739299524));
#85976=CARTESIAN_POINT('Ctrl Pts',(-9.48925323858479,15.1153920784687,4.87148742584891));
#85977=CARTESIAN_POINT('Ctrl Pts',(-9.49186523334213,15.1152397337505,4.87245731165007));
#85978=CARTESIAN_POINT('Ctrl Pts',(-9.49754953501219,15.1149075697124,4.87454955480878));
#85979=CARTESIAN_POINT('Ctrl Pts',(-9.5006227984139,15.1147275908429,4.87566905849327));
#85980=CARTESIAN_POINT('Ctrl Pts',(-9.50928928780186,15.1142190081,4.87879314969508));
#85981=CARTESIAN_POINT('Ctrl Pts',(-9.51489093931473,15.1138890543297,4.88077396755631));
#85982=CARTESIAN_POINT('Ctrl Pts',(-9.54931690174186,15.1118544377,4.8927120971759));
#85983=CARTESIAN_POINT('Ctrl Pts',(-9.57843268625854,15.1101045038807,4.90179990534415));
#85984=CARTESIAN_POINT('Ctrl Pts',(-9.75160576131538,15.0996110617689,4.94996894629137));
#85985=CARTESIAN_POINT('Ctrl Pts',(-9.90068412272485,15.0903494570182,4.96773943994467));
#85986=CARTESIAN_POINT('Ctrl Pts',(-10.0854962516892,15.0797468876945,4.96143470858105));
#85987=CARTESIAN_POINT('Ctrl Pts',(-10.1210410043669,15.0777412714519,4.9589209714033));
#85988=CARTESIAN_POINT('Ctrl Pts',(-10.1660972810273,15.075240820453,4.95407629656318));
#85989=CARTESIAN_POINT('Ctrl Pts',(-10.1757232652197,15.074709027742,4.95294443231735));
#85990=CARTESIAN_POINT('Ctrl Pts',(-10.1909556123931,15.0738712008915,4.95099975264291));
#85991=CARTESIAN_POINT('Ctrl Pts',(-10.1965696060167,15.073563209881,4.95024988168364));
#85992=CARTESIAN_POINT('Ctrl Pts',(-10.207065141767,15.0729888615243,4.94878591045955));
#85993=CARTESIAN_POINT('Ctrl Pts',(-10.2119476860737,15.0727222620452,4.94807968236347));
#85994=CARTESIAN_POINT('Ctrl Pts',(-10.2229399456884,15.072123346253,4.94643293735704));
#85995=CARTESIAN_POINT('Ctrl Pts',(-10.229047482265,15.071791475386,4.94547836861207));
#85996=CARTESIAN_POINT('Ctrl Pts',(-10.2471186793039,15.070812082335,4.942536544441));
#85997=CARTESIAN_POINT('Ctrl Pts',(-10.2590640514646,15.0701680188861,4.94043922214755));
#85998=CARTESIAN_POINT('Ctrl Pts',(-10.3686230803753,15.0642885205211,4.91979627920464));
#85999=CARTESIAN_POINT('Ctrl Pts',(-10.4641395082695,15.059389569775,4.89150352424864));
#86000=CARTESIAN_POINT('Ctrl Pts',(-10.6037619261951,15.0520418276346,4.83415254617049));
#86001=CARTESIAN_POINT('Ctrl Pts',(-10.6503924129982,15.0495482740272,4.81205219940654));
#86002=CARTESIAN_POINT('Ctrl Pts',(-10.7467881196453,15.0441421405985,4.75996199431381));
#86003=CARTESIAN_POINT('Ctrl Pts',(-10.7961285062314,15.0412206506213,4.72937980734762));
#86004=CARTESIAN_POINT('Ctrl Pts',(-10.8493986491535,15.0377424432373,4.69180785200379));
#86005=CARTESIAN_POINT('Ctrl Pts',(-10.8552477198228,15.0373559014095,4.68761751199154));
#86006=CARTESIAN_POINT('Ctrl Pts',(-10.8639211302505,15.0367753855477,4.68130648117454));
#86007=CARTESIAN_POINT('Ctrl Pts',(-10.8667691663875,15.0365835749731,4.6792183569735));
#86008=CARTESIAN_POINT('Ctrl Pts',(-10.8717822395187,15.0362437936472,4.67551489719724));
#86009=CARTESIAN_POINT('Ctrl Pts',(-10.8739503922626,15.0360961185289,4.67390385398586));
#86010=CARTESIAN_POINT('Ctrl Pts',(-10.8761257756508,15.0359472199628,4.67227807087424));
#86011=CARTESIAN_POINT('Ctrl Pts',(-10.8761374461992,15.0359464211272,4.67226934856275));
#86012=CARTESIAN_POINT('Ctrl Pts',(-10.8761606415294,15.0359448333915,4.67225201234286));
#86013=CARTESIAN_POINT('Ctrl Pts',(-10.8761721662952,15.0359440444931,4.67224339845296));
#86014=CARTESIAN_POINT('Ctrl Pts',(-10.876195072934,15.0359424764368,4.67222627694832));
#86015=CARTESIAN_POINT('Ctrl Pts',(-10.8762064547431,15.0359416972838,4.67221776938775));
#86016=CARTESIAN_POINT('Ctrl Pts',(-10.8762290780093,15.0359401485458,4.67220085866198));
#86017=CARTESIAN_POINT('Ctrl Pts',(-10.8762403195403,15.0359393789562,4.67219245544786));
#86018=CARTESIAN_POINT('Ctrl Pts',(-10.8762626646925,15.0359378491795,4.67217575160816));
#86019=CARTESIAN_POINT('Ctrl Pts',(-10.8762737684747,15.0359370889817,4.67216745086838));
#86020=CARTESIAN_POINT('Ctrl Pts',(-10.8762958409873,15.0359355777943,4.67215094985926));
#86021=CARTESIAN_POINT('Ctrl Pts',(-10.8763068096672,15.0359348268085,4.67214274963351));
#86022=CARTESIAN_POINT('Ctrl Pts',(-10.8763286144016,15.0359333338804,4.6721264478562));
#86023=CARTESIAN_POINT('Ctrl Pts',(-10.8763394504403,15.0359325919395,4.67211834632221));
#86024=CARTESIAN_POINT('Ctrl Pts',(-10.876360992492,15.0359311169245,4.67210224000176));
#86025=CARTESIAN_POINT('Ctrl Pts',(-10.8763716984013,15.0359303838578,4.67209423529848));
#86026=CARTESIAN_POINT('Ctrl Pts',(-10.8763929823846,15.0359289264425,4.67207832101846));
#86027=CARTESIAN_POINT('Ctrl Pts',(-10.8764035604791,15.0359282020929,4.67207041143181));
#86028=CARTESIAN_POINT('Ctrl Pts',(-10.87642459128,15.0359267619452,4.67205468557145));
#86029=CARTESIAN_POINT('Ctrl Pts',(-10.8764350439283,15.0359260461517,4.6720468693464));
#86030=CARTESIAN_POINT('Ctrl Pts',(-10.87645582608,15.0359246229638,4.67203132854752));
#86031=CARTESIAN_POINT('Ctrl Pts',(-10.8764661555771,15.0359239155703,4.67202360398344));
#86032=CARTESIAN_POINT('Ctrl Pts',(-10.8764866934039,15.0359225090484,4.67200824504284));
#86033=CARTESIAN_POINT('Ctrl Pts',(-10.8764969018557,15.035921809912,4.67200061057998));
#86034=CARTESIAN_POINT('Ctrl Pts',(-10.8790948178505,15.0357438848339,4.67005768780813));
#86035=CARTESIAN_POINT('Ctrl Pts',(-10.8816760830758,15.0355660632671,4.66811385390571));
#86036=CARTESIAN_POINT('Ctrl Pts',(-10.8870281543534,15.0351952399179,4.66405560500789));
#86037=CARTESIAN_POINT('Ctrl Pts',(-10.8897978843546,15.0350021453055,4.66193981025642));
#86038=CARTESIAN_POINT('Ctrl Pts',(-10.8968822653561,15.0345052447549,4.65648787208356));
#86039=CARTESIAN_POINT('Ctrl Pts',(-10.9011858352736,15.0342005137745,4.65313749598288));
#86040=CARTESIAN_POINT('Ctrl Pts',(-10.9136945416134,15.0333066007085,4.64328654167272));
#86041=CARTESIAN_POINT('Ctrl Pts',(-10.9218486271412,15.0327135089199,4.63672201020118));
#86042=CARTESIAN_POINT('Ctrl Pts',(-10.9502818532888,15.0306106923727,4.61332440552044));
#86043=CARTESIAN_POINT('Ctrl Pts',(-10.9701752541397,15.0290764114008,4.59603223683043));
#86044=CARTESIAN_POINT('Ctrl Pts',(-11.0934145911177,15.0192189751559,4.48292253295863));
#86045=CARTESIAN_POINT('Ctrl Pts',(-11.1829560351067,15.0105232002911,4.37310861173191));
#86046=CARTESIAN_POINT('Ctrl Pts',(-11.2732444225819,15.0004615697204,4.22241629916845));
#86047=CARTESIAN_POINT('Ctrl Pts',(-11.2900177844434,14.9985088288786,4.19201955965918));
#86048=CARTESIAN_POINT('Ctrl Pts',(-11.310034610839,14.9960640539962,4.15248283331175));
#86049=CARTESIAN_POINT('Ctrl Pts',(-11.3142892568767,14.9955370342598,4.14386977317137));
#86050=CARTESIAN_POINT('Ctrl Pts',(-11.320908966445,14.9947049830729,4.1301298415765));
#86051=CARTESIAN_POINT('Ctrl Pts',(-11.3233296496965,14.9943980403267,4.12503020275846));
#86052=CARTESIAN_POINT('Ctrl Pts',(-11.327620482344,14.9938490564419,4.1158540559587));
#86053=CARTESIAN_POINT('Ctrl Pts',(-11.3295015040351,14.9936066450047,4.11178273493822));
#86054=CARTESIAN_POINT('Ctrl Pts',(-11.3338552306561,14.9930414167458,4.10224452974898));
#86055=CARTESIAN_POINT('Ctrl Pts',(-11.3363131003484,14.9927191086675,4.09677093533924));
#86056=CARTESIAN_POINT('Ctrl Pts',(-11.3432828386302,14.9917956881457,4.08099057461121));
#86057=CARTESIAN_POINT('Ctrl Pts',(-11.3477096635691,14.9911974552448,4.07064656705221));
#86058=CARTESIAN_POINT('Ctrl Pts',(-11.3805409257206,14.9866669468822,3.99141723359833));
#86059=CARTESIAN_POINT('Ctrl Pts',(-11.4037681826831,14.9829153079701,3.92050074532737));
#86060=CARTESIAN_POINT('Ctrl Pts',(-11.4494005048327,14.97347487253,3.7341661659573));
#86061=CARTESIAN_POINT('Ctrl Pts',(-11.4634999999989,14.9679620217355,3.6172895195206));
#86062=CARTESIAN_POINT('Ctrl Pts',(-11.4635,14.961903098074,3.50000000001399));
#86063=CARTESIAN_POINT('Ctrl Pts',(-11.4635,14.8882344353249,3.49999999998375));
#86064=CARTESIAN_POINT('Ctrl Pts',(-11.4635000000011,14.8942398463545,3.60316946844975));
#86065=CARTESIAN_POINT('Ctrl Pts',(-11.4525909842708,14.9005631074229,3.70605351707629));
#86066=CARTESIAN_POINT('Ctrl Pts',(-11.4139418140341,14.9115352747244,3.88623554115491));
#86067=CARTESIAN_POINT('Ctrl Pts',(-11.3903693881249,14.9162386267349,3.96398890181075));
#86068=CARTESIAN_POINT('Ctrl Pts',(-11.3562631000691,14.9213624430335,4.05001182474101));
#86069=CARTESIAN_POINT('Ctrl Pts',(-11.3519309330338,14.9219904851051,4.06057592407899));
#86070=CARTESIAN_POINT('Ctrl Pts',(-11.3451200584314,14.9229442315386,4.07664609054269));
#86071=CARTESIAN_POINT('Ctrl Pts',(-11.3427302335125,14.9232729065917,4.08218915042296));
#86072=CARTESIAN_POINT('Ctrl Pts',(-11.3383096329501,14.9238701753104,4.09227045635291));
#86073=CARTESIAN_POINT('Ctrl Pts',(-11.3362899035378,14.9241391373364,4.09681342282491));
#86074=CARTESIAN_POINT('Ctrl Pts',(-11.3318657990193,14.9247199180101,4.1066294819829));
#86075=CARTESIAN_POINT('Ctrl Pts',(-11.3294531674705,14.9250314504131,4.11189877580763));
#86076=CARTESIAN_POINT('Ctrl Pts',(-11.3227856777081,14.9258785004376,4.12623527163765));
#86077=CARTESIAN_POINT('Ctrl Pts',(-11.3184688953993,14.9264118950679,4.13527343965763));
#86078=CARTESIAN_POINT('Ctrl Pts',(-11.2961109676347,14.9291009078496,4.18087512597888));
#86079=CARTESIAN_POINT('Ctrl Pts',(-11.276639515071,14.9312065918726,4.21671927176488));
#86080=CARTESIAN_POINT('Ctrl Pts',(-11.2485836215971,14.9339726899913,4.26358555172696));
#86081=CARTESIAN_POINT('Ctrl Pts',(-11.2413036116069,14.9346690809629,4.27536398611937));
#86082=CARTESIAN_POINT('Ctrl Pts',(-11.1799430085759,14.9403743632802,4.37156046142418));
#86083=CARTESIAN_POINT('Ctrl Pts',(-11.1174888547309,14.9451375093534,4.45031637052945));
#86084=CARTESIAN_POINT('Ctrl Pts',(-11.0196089356964,14.9520556001033,4.55062939020628));
#86085=CARTESIAN_POINT('Ctrl Pts',(-10.9905869972881,14.954054528487,4.57803594963648));
#86086=CARTESIAN_POINT('Ctrl Pts',(-10.9500432617639,14.9568351377534,4.61330208036142));
#86087=CARTESIAN_POINT('Ctrl Pts',(-10.9394749762753,14.9575589466431,4.6222345857603));
#86088=CARTESIAN_POINT('Ctrl Pts',(-10.9236417963749,14.9586445506031,4.63523668057777));
#86089=CARTESIAN_POINT('Ctrl Pts',(-10.9184729937097,14.9589991370126,4.63942259306721));
#86090=CARTESIAN_POINT('Ctrl Pts',(-10.9091064979989,14.959642388092,4.64690282800226));
#86091=CARTESIAN_POINT('Ctrl Pts',(-10.9049189505992,14.9599302188324,4.65020972551071));
#86092=CARTESIAN_POINT('Ctrl Pts',(-10.898231985169,14.9603904047423,4.65543128885926));
#86093=CARTESIAN_POINT('Ctrl Pts',(-10.8957442696172,14.9605617268526,4.65736094867607));
#86094=CARTESIAN_POINT('Ctrl Pts',(-10.8911614439799,14.9608775956956,4.66089210741686));
#86095=CARTESIAN_POINT('Ctrl Pts',(-10.8890682196649,14.961021973266,4.66249598052491));
#86096=CARTESIAN_POINT('Ctrl Pts',(-10.8841668262038,14.9613602744784,4.66623055142004));
#86097=CARTESIAN_POINT('Ctrl Pts',(-10.8813552987281,14.9615545049822,4.66835675736992));
#86098=CARTESIAN_POINT('Ctrl Pts',(-10.8729956394954,14.9621324679079,4.67463136969499));
#86099=CARTESIAN_POINT('Ctrl Pts',(-10.8674257840841,14.9625181327696,4.67875050222272));
#86100=CARTESIAN_POINT('Ctrl Pts',(-10.8230534053649,14.965593722231,4.71108086177603));
#86101=CARTESIAN_POINT('Ctrl Pts',(-10.7829175560504,14.9683940614871,4.73740575378498));
#86102=CARTESIAN_POINT('Ctrl Pts',(-10.6648471168658,14.9765290500929,4.80680127348856));
#86103=CARTESIAN_POINT('Ctrl Pts',(-10.5841749258098,14.9819549150823,4.84480179992673));
#86104=CARTESIAN_POINT('Ctrl Pts',(-10.4376851436043,14.9911954356943,4.89811987002947));
#86105=CARTESIAN_POINT('Ctrl Pts',(-10.3733221161449,14.9950681815391,4.91666507748371));
#86106=CARTESIAN_POINT('Ctrl Pts',(-10.2926446318109,14.9996713321233,4.9340275980174));
#86107=CARTESIAN_POINT('Ctrl Pts',(-10.2773285912516,15.0005345839328,4.9370681651998));
#86108=CARTESIAN_POINT('Ctrl Pts',(-10.2552331436454,15.0017650987034,4.94108817557133));
#86109=CARTESIAN_POINT('Ctrl Pts',(-10.2484913042628,15.0021385838179,4.9422659814753));
#86110=CARTESIAN_POINT('Ctrl Pts',(-10.236744327441,15.0027859739623,4.94423337597208));
#86111=CARTESIAN_POINT('Ctrl Pts',(-10.2317429300737,15.0030605471564,4.94504433707251));
#86112=CARTESIAN_POINT('Ctrl Pts',(-10.222083272515,15.0035888442992,4.94655918076951));
#86113=CARTESIAN_POINT('Ctrl Pts',(-10.2174256332924,15.0038426754045,4.94726657465079));
#86114=CARTESIAN_POINT('Ctrl Pts',(-10.2063729698559,15.0044429241842,4.94889067310962));
#86115=CARTESIAN_POINT('Ctrl Pts',(-10.1999751014081,15.0047887180051,4.94978755200362));
#86116=CARTESIAN_POINT('Ctrl Pts',(-10.1773247131694,15.0060072159816,4.95280998481098));
#86117=CARTESIAN_POINT('Ctrl Pts',(-10.1610423161494,15.0068727314364,4.9547048864692));
#86118=CARTESIAN_POINT('Ctrl Pts',(-10.0263100253444,15.0139561778449,4.96809471160317));
#86119=CARTESIAN_POINT('Ctrl Pts',(-9.90689796821671,15.0196859228711,4.96537668725338));
#86120=CARTESIAN_POINT('Ctrl Pts',(-9.73074272871516,15.0283567719625,4.93972689016283));
#86121=CARTESIAN_POINT('Ctrl Pts',(-9.67293178081447,15.0312485904662,4.92770390335595));
#86122=CARTESIAN_POINT('Ctrl Pts',(-9.59042092525551,15.0356297987794,4.90526878823164));
#86123=CARTESIAN_POINT('Ctrl Pts',(-9.56502861172117,15.0370143228863,4.89761765242205));
#86124=CARTESIAN_POINT('Ctrl Pts',(-9.53443880959041,15.0387419692196,4.88748608588831));
#86125=CARTESIAN_POINT('Ctrl Pts',(-9.52902848969315,15.0390498334634,4.88565893886861));
#86126=CARTESIAN_POINT('Ctrl Pts',(-9.52058328674959,15.0395341974786,4.88275169186861));
#86127=CARTESIAN_POINT('Ctrl Pts',(-9.5175409817214,15.03970946082,4.88169313582316));
#86128=CARTESIAN_POINT('Ctrl Pts',(-9.51186717425911,15.0400378145127,4.87969793670759));
#86129=CARTESIAN_POINT('Ctrl Pts',(-9.50923484536701,15.0401907580668,4.87876379945913));
#86130=CARTESIAN_POINT('Ctrl Pts',(-9.50321882364958,15.0405416790484,4.87660947657419));
#86131=CARTESIAN_POINT('Ctrl Pts',(-9.49983695386807,15.0407399435442,4.8753843516939));
#86132=CARTESIAN_POINT('Ctrl Pts',(-9.49099111631437,15.0412610848098,4.872142895987));
#86133=CARTESIAN_POINT('Ctrl Pts',(-9.48553466333627,15.0415850985818,4.87010641402269));
#86134=CARTESIAN_POINT('Ctrl Pts',(-9.44831571681395,15.0438120040533,4.85596171357128));
#86135=CARTESIAN_POINT('Ctrl Pts',(-9.41697351941511,15.0457709147941,4.84278348446731));
#86136=CARTESIAN_POINT('Ctrl Pts',(-9.29484981178013,15.053661090066,4.786353200698));
#86137=CARTESIAN_POINT('Ctrl Pts',(-9.2081681221159,15.0598180118331,4.73488636195495));
#86138=CARTESIAN_POINT('Ctrl Pts',(-9.08610674666367,15.0688484644349,4.64423894864798));
#86139=CARTESIAN_POINT('Ctrl Pts',(-9.04641399966737,15.0718567349263,4.61137670636658));
#86140=CARTESIAN_POINT('Ctrl Pts',(-8.98643462371903,15.0764977565217,4.55613449917588));
#86141=CARTESIAN_POINT('Ctrl Pts',(-8.96496696949253,15.0781807497666,4.53510466383559));
#86142=CARTESIAN_POINT('Ctrl Pts',(-8.93808624996012,15.0803183400619,4.50709899690486));
#86143=CARTESIAN_POINT('Ctrl Pts',(-8.93206868824645,15.0807989404787,4.50071570396994));
#86144=CARTESIAN_POINT('Ctrl Pts',(-8.92239799450001,15.081574810741,4.49027067066547));
#86145=CARTESIAN_POINT('Ctrl Pts',(-8.91870963101484,15.0818715710564,4.48624196955192));
#86146=CARTESIAN_POINT('Ctrl Pts',(-8.91167201039257,15.0824394809647,4.47846802681584));
#86147=CARTESIAN_POINT('Ctrl Pts',(-8.90831932194101,15.0827107725056,4.47472600790505));
#86148=CARTESIAN_POINT('Ctrl Pts',(-8.90070000759502,15.0833290554933,4.46613327679684));
#86149=CARTESIAN_POINT('Ctrl Pts',(-8.89644607895447,15.0836755183138,4.461271411728));
#86150=CARTESIAN_POINT('Ctrl Pts',(-8.88524770984574,15.0845910819654,4.44830035377643));
#86151=CARTESIAN_POINT('Ctrl Pts',(-8.87835950325239,15.0851578899332,4.44014298563865));
#86152=CARTESIAN_POINT('Ctrl Pts',(-8.81071966705183,15.0907626790732,4.35823876962812));
#86153=CARTESIAN_POINT('Ctrl Pts',(-8.75723664950791,15.0954906074507,4.27878347640379));
#86154=CARTESIAN_POINT('Ctrl Pts',(-8.67257484173989,15.1041820835112,4.12179602815909));
#86155=CARTESIAN_POINT('Ctrl Pts',(-8.63953134981396,15.1081543712008,4.04572072778805));
#86156=CARTESIAN_POINT('Ctrl Pts',(-8.60259495352467,15.1140247168365,3.93608911931097));
#86157=CARTESIAN_POINT('Ctrl Pts',(-8.59314601981413,15.1157295742275,3.90456908694282));
#86158=CARTESIAN_POINT('Ctrl Pts',(-8.58322291074366,15.1178157959694,3.86689469457777));
#86159=CARTESIAN_POINT('Ctrl Pts',(-8.5817145619884,15.1181424879712,3.8610200150951));
#86160=CARTESIAN_POINT('Ctrl Pts',(-8.57944245509655,15.118649981678,3.8519366273158));
#86161=CARTESIAN_POINT('Ctrl Pts',(-8.57865293632641,15.1188293464862,3.84873435760762));
#86162=CARTESIAN_POINT('Ctrl Pts',(-8.57721666971745,15.1191613315591,3.84282299014518));
#86163=CARTESIAN_POINT('Ctrl Pts',(-8.57656682681676,15.1193137736565,3.84011469922855));
#86164=CARTESIAN_POINT('Ctrl Pts',(-8.57511966607134,15.1196583456021,3.83400670283099));
#86165=CARTESIAN_POINT('Ctrl Pts',(-8.57432678731008,15.1198507221023,3.83060600969835));
#86166=CARTESIAN_POINT('Ctrl Pts',(-8.57232147347091,15.1203465770944,3.82186375578899));
#86167=CARTESIAN_POINT('Ctrl Pts',(-8.57112685318125,15.1206510241418,3.81651821555197));
#86168=CARTESIAN_POINT('Ctrl Pts',(-8.56409799375259,15.1224977955142,3.78421543125748));
#86169=CARTESIAN_POINT('Ctrl Pts',(-8.55899712432177,15.1240770293036,3.75710599878659));
#86170=CARTESIAN_POINT('Ctrl Pts',(-8.53796603708125,15.1318701327016,3.62487089865659));
#86171=CARTESIAN_POINT('Ctrl Pts',(-8.53275795637476,15.1383937334468,3.51836579631194));
#86172=CARTESIAN_POINT('Ctrl Pts',(-8.5422747562762,15.1478266647474,3.35995562693801));
#86173=CARTESIAN_POINT('Ctrl Pts',(-8.54821990518427,15.1508889964035,3.30787842699104));
#86174=CARTESIAN_POINT('Ctrl Pts',(-8.56200742495591,15.1556021272015,3.22626056100973));
#86175=CARTESIAN_POINT('Ctrl Pts',(-8.56800225099869,15.1573051241657,3.19645664774875));
#86176=CARTESIAN_POINT('Ctrl Pts',(-8.57692604473056,15.1594640281688,3.15828324986426));
#86177=CARTESIAN_POINT('Ctrl Pts',(-8.57900829327314,15.1599465821011,3.14972525973881));
#86178=CARTESIAN_POINT('Ctrl Pts',(-8.58250874671746,15.1607248206277,3.13588365186717));
#86179=CARTESIAN_POINT('Ctrl Pts',(-8.58387952145032,15.1610220125585,3.13058836039581));
#86180=CARTESIAN_POINT('Ctrl Pts',(-8.5865657045988,15.1615902331718,3.12044636543015));
#86181=CARTESIAN_POINT('Ctrl Pts',(-8.58787643387499,15.161861407242,3.11559851223665));
#86182=CARTESIAN_POINT('Ctrl Pts',(-8.59092596060797,15.1624787167359,3.10454567252207));
#86183=CARTESIAN_POINT('Ctrl Pts',(-8.5926808455952,15.1628243294063,3.09834520659373));
#86184=CARTESIAN_POINT('Ctrl Pts',(-8.59743651468287,15.1637361433772,3.08195606861809));
#86185=CARTESIAN_POINT('Ctrl Pts',(-8.60050738803506,15.1643000822078,3.07178802462116));
#86186=CARTESIAN_POINT('Ctrl Pts',(-8.62663584487003,15.1689034814842,2.98855818020661));
#86187=CARTESIAN_POINT('Ctrl Pts',(-8.65528821930903,15.1727511726298,2.91737318651635));
#86188=CARTESIAN_POINT('Ctrl Pts',(-8.71979843770249,15.1798725818493,2.78754861217136));
#86189=CARTESIAN_POINT('Ctrl Pts',(-8.75445983502587,15.183156754937,2.72855166315073));
#86190=CARTESIAN_POINT('Ctrl Pts',(-8.81857046839752,15.1887237550825,2.6350828894891));
#86191=CARTESIAN_POINT('Ctrl Pts',(-8.84572121775919,15.190963756061,2.59916853803295));
#86192=CARTESIAN_POINT('Ctrl Pts',(-8.88884382868792,15.1944443208247,2.54728328637657));
#86193=CARTESIAN_POINT('Ctrl Pts',(-8.90360178069876,15.1956234681499,2.5303361365475));
#86194=CARTESIAN_POINT('Ctrl Pts',(-8.92240025110593,15.1971205180982,2.50972706789437));
#86195=CARTESIAN_POINT('Ctrl Pts',(-8.92607954657268,15.1974133001321,2.50573818502168));
#86196=CARTESIAN_POINT('Ctrl Pts',(-8.931935389935,15.1978791013175,2.49946003768659));
#86197=CARTESIAN_POINT('Ctrl Pts',(-8.93409734858696,15.1980510351194,2.49715715848275));
#86198=CARTESIAN_POINT('Ctrl Pts',(-8.93819303292104,15.1983767204283,2.49282271608833));
#86199=CARTESIAN_POINT('Ctrl Pts',(-8.94012515282852,15.1985303517351,2.49078970257424));
#86200=CARTESIAN_POINT('Ctrl Pts',(-8.94457665313866,15.1988842745235,2.48613263101965));
#86201=CARTESIAN_POINT('Ctrl Pts',(-8.94709998197698,15.1990848666479,2.48351240320294));
#86202=CARTESIAN_POINT('Ctrl Pts',(-8.95387576549448,15.1996233624182,2.47652872085102));
#86203=CARTESIAN_POINT('Ctrl Pts',(-8.95814569798557,15.1999625572352,2.47218241695962));
#86204=CARTESIAN_POINT('Ctrl Pts',(-8.99086001091462,15.2025592526505,2.43929630025795));
#86205=CARTESIAN_POINT('Ctrl Pts',(-9.02044280829839,15.2048952455832,2.41191773726276));
#86206=CARTESIAN_POINT('Ctrl Pts',(-9.12762148620842,15.2132045294412,2.32064147821887));
#86207=CARTESIAN_POINT('Ctrl Pts',(-9.21063609141853,15.2193546353876,2.26353858448475));
#86208=CARTESIAN_POINT('Ctrl Pts',(-9.35504210098213,15.2290851614235,2.18472066462419));
#86209=CARTESIAN_POINT('Ctrl Pts',(-9.41319061678508,15.2327831895614,2.1577679644304));
#86210=CARTESIAN_POINT('Ctrl Pts',(-9.48715955031423,15.2372033364255,2.12921198571385));
#86211=CARTESIAN_POINT('Ctrl Pts',(-9.50148064875236,15.2380466929788,2.12393910448444));
#86212=CARTESIAN_POINT('Ctrl Pts',(-9.52228131036886,15.2392541508225,2.11664788048163));
#86213=CARTESIAN_POINT('Ctrl Pts',(-9.52869621747294,15.239624156737,2.11444921430426));
#86214=CARTESIAN_POINT('Ctrl Pts',(-9.53992068113804,15.2402675002265,2.11068907853604));
#86215=CARTESIAN_POINT('Ctrl Pts',(-9.54472344343061,15.2405414821885,2.10910781364137));
#86216=CARTESIAN_POINT('Ctrl Pts',(-9.55403218860354,15.2410700484772,2.10609637742144));
#86217=CARTESIAN_POINT('Ctrl Pts',(-9.55853709014672,15.2413247317102,2.10466308807332));
#86218=CARTESIAN_POINT('Ctrl Pts',(-9.56927498891296,15.2419291881029,2.10130390264339));
#86219=CARTESIAN_POINT('Ctrl Pts',(-9.57551410401955,15.2422783162133,2.09939779597486));
#86220=CARTESIAN_POINT('Ctrl Pts',(-9.5978395194634,15.2435203394882,2.0927400602162));
#86221=CARTESIAN_POINT('Ctrl Pts',(-9.61399483812844,15.2444056707068,2.08822323447989));
#86222=CARTESIAN_POINT('Ctrl Pts',(-9.73956200821279,15.251190923548,2.05543287596522));
#86223=CARTESIAN_POINT('Ctrl Pts',(-9.85183739388462,15.2566579178559,2.03963955576761));
#86224=CARTESIAN_POINT('Ctrl Pts',(-10.0507956081288,15.2663404534831,2.03485561460626));
#86225=CARTESIAN_POINT('Ctrl Pts',(-10.136775493678,15.2705381222922,2.0403709239744));
#86226=CARTESIAN_POINT('Ctrl Pts',(-10.2305116623212,15.2755742466312,2.05474051074436));
#86227=CARTESIAN_POINT('Ctrl Pts',(-10.239249431601,15.2760482308405,2.05616125570871));
#86228=CARTESIAN_POINT('Ctrl Pts',(-10.2517606175828,15.276734097112,2.05831223658529));
#86229=CARTESIAN_POINT('Ctrl Pts',(-10.2555450554805,15.2769425073409,2.05897823067048));
#86230=CARTESIAN_POINT('Ctrl Pts',(-10.2621071076818,15.2773055924583,2.06015969812805));
#86231=CARTESIAN_POINT('Ctrl Pts',(-10.2648859575046,15.2774598833904,2.06066832861743));
#86232=CARTESIAN_POINT('Ctrl Pts',(-10.270320301903,15.2777626858669,2.06167928186661));
#86233=CARTESIAN_POINT('Ctrl Pts',(-10.2729758814471,15.2779111523883,2.0621809148104));
#86234=CARTESIAN_POINT('Ctrl Pts',(-10.2802635831982,15.2783199255853,2.06357846254583));
#86235=CARTESIAN_POINT('Ctrl Pts',(-10.2848927434349,15.2785810635875,2.06448941738199));
#86236=CARTESIAN_POINT('Ctrl Pts',(-10.3029047561696,15.2796027175856,2.06812448837272));
#86237=CARTESIAN_POINT('Ctrl Pts',(-10.3162531984437,15.2803718408089,2.07101341540137));
#86238=CARTESIAN_POINT('Ctrl Pts',(-10.3548769649107,15.2826283341168,2.07994019741264));
#86239=CARTESIAN_POINT('Ctrl Pts',(-10.380033541817,15.2841368213591,2.08646476304541));
#86240=CARTESIAN_POINT('Ctrl Pts',(-10.4146769176456,15.2862563404977,2.09644142347499));
#86241=CARTESIAN_POINT('Ctrl Pts',(-10.4243230089417,15.2868511053106,2.0993274466112));
#86242=CARTESIAN_POINT('Ctrl Pts',(-10.5125573669318,15.2923296385583,2.12672146906737));
#86243=CARTESIAN_POINT('Ctrl Pts',(-10.5889765547282,15.2973426361053,2.15771986660788));
#86244=CARTESIAN_POINT('Ctrl Pts',(-10.7117423426112,15.3055455699722,2.22003170265305));
#86245=CARTESIAN_POINT('Ctrl Pts',(-10.7596421104052,15.308790722422,2.24786549118916));
#86246=CARTESIAN_POINT('Ctrl Pts',(-10.832183641133,15.3137458524652,2.29571698768956));
#86247=CARTESIAN_POINT('Ctrl Pts',(-10.8579466149676,15.315514915319,2.31393296639621));
#86248=CARTESIAN_POINT('Ctrl Pts',(-10.8902155388229,15.3177439931508,2.33835112129689));
#86249=CARTESIAN_POINT('Ctrl Pts',(-10.8972796084536,15.3182328340307,2.3437988357749));
#86250=CARTESIAN_POINT('Ctrl Pts',(-10.9086137858932,15.3190186944345,2.35270604041413));
#86251=CARTESIAN_POINT('Ctrl Pts',(-10.9129149172011,15.319317276063,2.35612553279761));
#86252=CARTESIAN_POINT('Ctrl Pts',(-10.9211044943868,15.3198865224981,2.36271203801644));
#86253=CARTESIAN_POINT('Ctrl Pts',(-10.9249961123888,15.3201573436389,2.36587496677694));
#86254=CARTESIAN_POINT('Ctrl Pts',(-10.9338122744345,15.3207716391897,2.37311590402879));
#86255=CARTESIAN_POINT('Ctrl Pts',(-10.9387265249153,15.3211146090705,2.37720632223563));
#86256=CARTESIAN_POINT('Ctrl Pts',(-10.9516023477294,15.3220147981336,2.38806724864338));
#86257=CARTESIAN_POINT('Ctrl Pts',(-10.9595185540679,15.3225698478196,2.39489112587574));
#86258=CARTESIAN_POINT('Ctrl Pts',(-11.0193993321717,15.3267824026093,2.44763771282057));
#86259=CARTESIAN_POINT('Ctrl Pts',(-11.0681165806546,15.3302849749552,2.49711919994953));
#86260=CARTESIAN_POINT('Ctrl Pts',(-11.1288964898801,15.3349052785255,2.56832753106945));
#86261=CARTESIAN_POINT('Ctrl Pts',(-11.1441863649272,15.3360927912822,2.58717007640934));
#86262=CARTESIAN_POINT('Ctrl Pts',(-11.1978185158371,15.3403758920866,2.65672985655768));
#86263=CARTESIAN_POINT('Ctrl Pts',(-11.2333132507234,15.3434382683448,2.70954967388866));
#86264=CARTESIAN_POINT('Ctrl Pts',(-11.2896613205186,15.3489951677788,2.80648476672443));
#86265=CARTESIAN_POINT('Ctrl Pts',(-11.3119561216286,15.3514505166937,2.84964624668677));
#86266=CARTESIAN_POINT('Ctrl Pts',(-11.3361664199632,15.3545460996965,2.90284868204695));
#86267=CARTESIAN_POINT('Ctrl Pts',(-11.3401780258813,15.3550755149608,2.91190711053269));
#86268=CARTESIAN_POINT('Ctrl Pts',(-11.345688046681,15.3558273118416,2.92469825358599));
#86269=CARTESIAN_POINT('Ctrl Pts',(-11.3472636007124,15.3560452380944,2.92839768385424));
#86270=CARTESIAN_POINT('Ctrl Pts',(-11.3499319561595,15.3564194958149,2.9347353556276));
#86271=CARTESIAN_POINT('Ctrl Pts',(-11.3510323313652,15.3565753745971,2.93737042030137));
#86272=CARTESIAN_POINT('Ctrl Pts',(-11.3531397029463,15.3568769281393,2.94245876668105));
#86273=CARTESIAN_POINT('Ctrl Pts',(-11.3541477497147,15.3570225335151,2.94491157979048));
#86274=CARTESIAN_POINT('Ctrl Pts',(-11.3565536419067,15.3573733112104,2.95081123337625));
#86275=CARTESIAN_POINT('Ctrl Pts',(-11.3579450170331,15.3575788627272,2.95426067133729));
#86276=CARTESIAN_POINT('Ctrl Pts',(-11.3629671215119,15.3583305848348,2.96684937917546));
#86277=CARTESIAN_POINT('Ctrl Pts',(-11.3665187740726,15.3588811721961,2.97601966810231));
#86278=CARTESIAN_POINT('Ctrl Pts',(-11.4090758996143,15.3657117135496,3.08927747424932));
#86279=CARTESIAN_POINT('Ctrl Pts',(-11.4361902494202,15.3725209920055,3.1974391301335));
#86280=CARTESIAN_POINT('Ctrl Pts',(-11.4592203408166,15.3830179682979,3.37111649555571));
#86281=CARTESIAN_POINT('Ctrl Pts',(-11.4634632343829,15.3868013572218,3.43510224584699));
#86282=CARTESIAN_POINT('Ctrl Pts',(-11.463499920781,15.390483742019,3.49944368928866));
#86283=CARTESIAN_POINT('Ctrl Pts',(-11.4635,15.390499659156,3.49972184492555));
#86284=CARTESIAN_POINT('Ctrl Pts',(-11.4635,15.3905155741067,3.49999999999573));
#86285=CARTESIAN_POINT('Origin',(-10.,13.2,3.5));
#86286=CARTESIAN_POINT('',(-11.4635,15.960023863236,3.50000000002449));
#86287=CARTESIAN_POINT('',(-11.4635,15.8897282898296,3.49999999995642));
#86288=CARTESIAN_POINT('',(-11.4635,13.2,3.5));
#86289=CARTESIAN_POINT('Ctrl Pts',(-11.4635,15.960023863236,3.50000000002449));
#86290=CARTESIAN_POINT('Ctrl Pts',(-11.4635000000009,15.9568962036078,3.4473044483025));
#86291=CARTESIAN_POINT('Ctrl Pts',(-11.4606539605496,15.9538221865891,3.39464321866628));
#86292=CARTESIAN_POINT('Ctrl Pts',(-11.4524341116655,15.949492807175,3.31883138145111));
#86293=CARTESIAN_POINT('Ctrl Pts',(-11.4493305376893,15.94817231534,3.29548105321944));
#86294=CARTESIAN_POINT('Ctrl Pts',(-11.4444430278596,15.9464349894388,3.26446191623883));
#86295=CARTESIAN_POINT('Ctrl Pts',(-11.4431590851417,15.9460027149928,3.2567188704753));
#86296=CARTESIAN_POINT('Ctrl Pts',(-11.4408759777639,15.9452728985708,3.24360478451572));
#86297=CARTESIAN_POINT('Ctrl Pts',(-11.4399089253907,15.9449743550825,3.23822838668932));
#86298=CARTESIAN_POINT('Ctrl Pts',(-11.4380600356207,15.9444225574881,3.22826969776994));
#86299=CARTESIAN_POINT('Ctrl Pts',(-11.4371863438578,15.9441690501085,3.22368598129795));
#86300=CARTESIAN_POINT('Ctrl Pts',(-11.4353318059959,15.9436455428288,3.21420318655391));
#86301=CARTESIAN_POINT('Ctrl Pts',(-11.4343477638558,15.9433756477469,3.20930479010235));
#86302=CARTESIAN_POINT('Ctrl Pts',(-11.4320537526297,15.9427638936236,3.19818089726335));
#86303=CARTESIAN_POINT('Ctrl Pts',(-11.4307282314604,15.9424225321171,3.19195868678954));
#86304=CARTESIAN_POINT('Ctrl Pts',(-11.4271895258137,15.9415415427226,3.17586317207036));
#86305=CARTESIAN_POINT('Ctrl Pts',(-11.424914427742,15.9410038811709,3.16600373315612));
#86306=CARTESIAN_POINT('Ctrl Pts',(-11.4088297519592,15.9373871195153,3.09945645373874));
#86307=CARTESIAN_POINT('Ctrl Pts',(-11.3917424850724,15.9344153251949,3.04361171257661));
#86308=CARTESIAN_POINT('Ctrl Pts',(-11.3578169515657,15.9295801403371,2.95257833349419));
#86309=CARTESIAN_POINT('Ctrl Pts',(-11.3428286530943,15.9276802664013,2.91677730844212));
#86310=CARTESIAN_POINT('Ctrl Pts',(-11.3093019978364,15.9238144313663,2.8448628590834));
#86311=CARTESIAN_POINT('Ctrl Pts',(-11.2906490496529,15.9218510559634,2.80884055088164));
#86312=CARTESIAN_POINT('Ctrl Pts',(-11.2451776863909,15.9173713458771,2.72930361279366));
#86313=CARTESIAN_POINT('Ctrl Pts',(-11.2175290223151,15.9148470324123,2.686327594106));
#86314=CARTESIAN_POINT('Ctrl Pts',(-11.1734834653787,15.9109704456013,2.62515130329857));
#86315=CARTESIAN_POINT('Ctrl Pts',(-11.1587848611077,15.9096972211357,2.60577341015681));
#86316=CARTESIAN_POINT('Ctrl Pts',(-11.1401405818136,15.9080944848471,2.58242567694317));
#86317=CARTESIAN_POINT('Ctrl Pts',(-11.136645254541,15.9077945179989,2.57809938281918));
#86318=CARTESIAN_POINT('Ctrl Pts',(-11.1311078783804,15.9073199075609,2.57132493294089));
#86319=CARTESIAN_POINT('Ctrl Pts',(-11.1290823085488,15.9071464204813,2.56886330067195));
#86320=CARTESIAN_POINT('Ctrl Pts',(-11.1252641384612,15.9068195922635,2.56425393675488));
#86321=CARTESIAN_POINT('Ctrl Pts',(-11.1234734142915,15.9066663842771,2.56210471633554));
#86322=CARTESIAN_POINT('Ctrl Pts',(-11.1193731955624,15.9063157656869,2.55721224114234));
#86323=CARTESIAN_POINT('Ctrl Pts',(-11.1170597755381,15.9061180735414,2.55447233435166));
#86324=CARTESIAN_POINT('Ctrl Pts',(-11.1109015035602,15.9055922390507,2.54723290984417));
#86325=CARTESIAN_POINT('Ctrl Pts',(-11.1070394269122,15.905262896463,2.54274821309016));
#86326=CARTESIAN_POINT('Ctrl Pts',(-11.0796365625771,15.9029298540553,2.5113152563544));
#86327=CARTESIAN_POINT('Ctrl Pts',(-11.0551432960583,15.9008641439903,2.48521684638434));
#86328=CARTESIAN_POINT('Ctrl Pts',(-11.0286256443926,15.8986712425415,2.45896017953603));
#86329=CARTESIAN_POINT('Ctrl Pts',(-11.0275290443621,15.8985806323488,2.45787779648239));
#86330=CARTESIAN_POINT('Ctrl Pts',(-10.9598782297139,15.8929954259981,2.3913146389042));
#86331=CARTESIAN_POINT('Ctrl Pts',(-10.8872128595198,15.8872911306016,2.33235142091044));
#86332=CARTESIAN_POINT('Ctrl Pts',(-10.7528600822203,15.8776929951419,2.24316127912962));
#86333=CARTESIAN_POINT('Ctrl Pts',(-10.6937457625153,15.8737373947097,2.20958898227639));
#86334=CARTESIAN_POINT('Ctrl Pts',(-10.6203798978882,15.8691691504059,2.17442771387024));
#86335=CARTESIAN_POINT('Ctrl Pts',(-10.6081727485223,15.8684196027385,2.16878287709968));
#86336=CARTESIAN_POINT('Ctrl Pts',(-10.5860688537917,15.8670810305065,2.15892910173817));
#86337=CARTESIAN_POINT('Ctrl Pts',(-10.5762003501307,15.8664899957783,2.1546595149432));
#86338=CARTESIAN_POINT('Ctrl Pts',(-10.5608730483858,15.8655819890449,2.14822778301719));
#86339=CARTESIAN_POINT('Ctrl Pts',(-10.5554469274014,15.8652624498807,2.1459891376893));
#86340=CARTESIAN_POINT('Ctrl Pts',(-10.5454468052684,15.8646770124106,2.14193363464437));
#86341=CARTESIAN_POINT('Ctrl Pts',(-10.5408768431749,15.8644107927743,2.14010709560459));
#86342=CARTESIAN_POINT('Ctrl Pts',(-10.5308881787346,15.8638317490648,2.13617310706793));
#86343=CARTESIAN_POINT('Ctrl Pts',(-10.5254659420733,15.8635192338782,2.13407482003494));
#86344=CARTESIAN_POINT('Ctrl Pts',(-10.5105878570213,15.8626665910351,2.12841903056188));
#86345=CARTESIAN_POINT('Ctrl Pts',(-10.5011073518067,15.8621286349723,2.12492700401845));
#86346=CARTESIAN_POINT('Ctrl Pts',(-10.452098283955,15.8593742363972,2.1074493008723));
#86347=CARTESIAN_POINT('Ctrl Pts',(-10.412016324378,15.8572107798683,2.09506823084163));
#86348=CARTESIAN_POINT('Ctrl Pts',(-10.2685440591714,15.8497088616215,2.05742025816476));
#86349=CARTESIAN_POINT('Ctrl Pts',(-10.1629989675784,15.8446493263694,2.04171898007317));
#86350=CARTESIAN_POINT('Ctrl Pts',(-9.998198904247,15.8365456077858,2.03533123189213));
#86351=CARTESIAN_POINT('Ctrl Pts',(-9.93963629123927,15.8336194918298,2.03657499629506));
#86352=CARTESIAN_POINT('Ctrl Pts',(-9.87046466678711,15.8299530480189,2.04220327667502));
#86353=CARTESIAN_POINT('Ctrl Pts',(-9.85962804380893,15.8293724589847,2.04320681323338));
#86354=CARTESIAN_POINT('Ctrl Pts',(-9.84465279962538,15.828560341094,2.0447622478619));
#86355=CARTESIAN_POINT('Ctrl Pts',(-9.84050356944017,15.8283342828381,2.04521116457326));
#86356=CARTESIAN_POINT('Ctrl Pts',(-9.83349028378045,15.8279503370411,2.04600031538899));
#86357=CARTESIAN_POINT('Ctrl Pts',(-9.830625175024,15.8277929628939,2.04633128363261));
#86358=CARTESIAN_POINT('Ctrl Pts',(-9.82516233083524,15.8274918736265,2.04697870360727));
#86359=CARTESIAN_POINT('Ctrl Pts',(-9.8225644379796,15.8273482465037,2.04729365684715));
#86360=CARTESIAN_POINT('Ctrl Pts',(-9.81571838593965,15.8269686153677,2.04814226989608));
#86361=CARTESIAN_POINT('Ctrl Pts',(-9.81147173317666,15.8267319693174,2.04868760309712));
#86362=CARTESIAN_POINT('Ctrl Pts',(-9.79655585326278,15.8258968520576,2.05066959393247));
#86363=CARTESIAN_POINT('Ctrl Pts',(-9.78590040412202,15.8252932053556,2.05220529910829));
#86364=CARTESIAN_POINT('Ctrl Pts',(-9.67593669752432,15.8189972581231,2.06929414552402));
#86365=CARTESIAN_POINT('Ctrl Pts',(-9.57847180934187,15.8128756980523,2.09492075553681));
#86366=CARTESIAN_POINT('Ctrl Pts',(-9.46293814267093,15.8054576958196,2.1384115302824));
#86367=CARTESIAN_POINT('Ctrl Pts',(-9.44165941195558,15.8040832986414,2.1469979961773));
#86368=CARTESIAN_POINT('Ctrl Pts',(-9.34602539713028,15.7978822039627,2.18822906870028));
#86369=CARTESIAN_POINT('Ctrl Pts',(-9.27425634679107,15.7931727072006,2.22653020878963));
#86370=CARTESIAN_POINT('Ctrl Pts',(-9.19643616550276,15.7880433249029,2.27678793494339));
#86371=CARTESIAN_POINT('Ctrl Pts',(-9.18691820226508,15.7874153118116,2.28309384388545));
#86372=CARTESIAN_POINT('Ctrl Pts',(-9.17248329593104,15.7864616682631,2.29290233474315));
#86373=CARTESIAN_POINT('Ctrl Pts',(-9.16751275903493,15.7861330669625,2.29632493415501));
#86374=CARTESIAN_POINT('Ctrl Pts',(-9.15848761219643,15.7855359627809,2.30262209327246));
#86375=CARTESIAN_POINT('Ctrl Pts',(-9.15442622108853,15.7852670915221,2.30548673694756));
#86376=CARTESIAN_POINT('Ctrl Pts',(-9.14566292629698,15.7846865421063,2.31173489110296));
#86377=CARTESIAN_POINT('Ctrl Pts',(-9.14096634810732,15.7843751497534,2.31512574896586));
#86378=CARTESIAN_POINT('Ctrl Pts',(-9.12820952531143,15.7835285703457,2.32445169910644));
#86379=CARTESIAN_POINT('Ctrl Pts',(-9.12018975802617,15.7829955032797,2.33044179953527));
#86380=CARTESIAN_POINT('Ctrl Pts',(-9.07986165475805,15.7803096684735,2.36121311616388));
#86381=CARTESIAN_POINT('Ctrl Pts',(-9.04853465282346,15.7782066954236,2.38725374804408));
#86382=CARTESIAN_POINT('Ctrl Pts',(-9.00796215401531,15.7754362564872,2.42394764518034));
#86383=CARTESIAN_POINT('Ctrl Pts',(-8.9977266200889,15.7747329971335,2.43347487479258));
#86384=CARTESIAN_POINT('Ctrl Pts',(-8.89320424434621,15.7674961138958,2.53359804027025));
#86385=CARTESIAN_POINT('Ctrl Pts',(-8.81133853057874,15.7614121856562,2.63628283444366));
#86386=CARTESIAN_POINT('Ctrl Pts',(-8.72921938640003,15.7532528099632,2.77350127820991));
#86387=CARTESIAN_POINT('Ctrl Pts',(-8.71498772646282,15.7517340391825,2.79898146248846));
#86388=CARTESIAN_POINT('Ctrl Pts',(-8.69882054194111,15.7498561243616,2.83007558931542));
#86389=CARTESIAN_POINT('Ctrl Pts',(-8.69614437558332,15.7495398348578,2.83529916019225));
#86390=CARTESIAN_POINT('Ctrl Pts',(-8.6920329564605,15.7490451503653,2.84344454990599));
#86391=CARTESIAN_POINT('Ctrl Pts',(-8.69057587913687,15.7488680801191,2.84635535853742));
#86392=CARTESIAN_POINT('Ctrl Pts',(-8.68788894169534,15.7485382280867,2.85176810250996));
#86393=CARTESIAN_POINT('Ctrl Pts',(-8.68665651284523,15.7483856074345,2.85426870402017));
#86394=CARTESIAN_POINT('Ctrl Pts',(-8.68387306936121,15.7480378900271,2.8599572506615));
#86395=CARTESIAN_POINT('Ctrl Pts',(-8.68232649555938,15.7478425257776,2.86314730613535));
#86396=CARTESIAN_POINT('Ctrl Pts',(-8.67764637786537,15.7472447653868,2.87289082668586));
#86397=CARTESIAN_POINT('Ctrl Pts',(-8.67455007117627,15.7468401867075,2.87946192786984));
#86398=CARTESIAN_POINT('Ctrl Pts',(-8.6420825631744,15.7425014250007,2.94971746834774));
#86399=CARTESIAN_POINT('Ctrl Pts',(-8.61727924527846,15.7383338052031,3.01540542703653));
#86400=CARTESIAN_POINT('Ctrl Pts',(-8.56926998273027,15.7282226414929,3.17674960448337));
#86401=CARTESIAN_POINT('Ctrl Pts',(-8.55080292236035,15.7222761674507,3.27348119612623));
#86402=CARTESIAN_POINT('Ctrl Pts',(-8.53827691825814,15.7140364184731,3.41541070628096));
#86403=CARTESIAN_POINT('Ctrl Pts',(-8.53638758214428,15.7115318489563,3.459639220784));
#86404=CARTESIAN_POINT('Ctrl Pts',(-8.53653154490704,15.7085410112187,3.51381550444179));
#86405=CARTESIAN_POINT('Ctrl Pts',(-8.53665891683797,15.7079961426061,3.52374170104145));
#86406=CARTESIAN_POINT('Ctrl Pts',(-8.53701874578127,15.7071425046438,3.53937973832679));
#86407=CARTESIAN_POINT('Ctrl Pts',(-8.53718368776214,15.7068316512991,3.54509270374045));
#86408=CARTESIAN_POINT('Ctrl Pts',(-8.53755480722251,15.706252137337,3.5557768902552));
#86409=CARTESIAN_POINT('Ctrl Pts',(-8.53775287697131,15.7059832292774,3.56074829549104));
#86410=CARTESIAN_POINT('Ctrl Pts',(-8.53825167439652,15.7053846242354,3.57184489901904));
#86411=CARTESIAN_POINT('Ctrl Pts',(-8.53856555871815,15.7050553403103,3.57796943195846));
#86412=CARTESIAN_POINT('Ctrl Pts',(-8.53945622958422,15.7042260163666,3.59344468708322));
#86413=CARTESIAN_POINT('Ctrl Pts',(-8.54008432683518,15.7037275712682,3.60279225428986));
#86414=CARTESIAN_POINT('Ctrl Pts',(-8.54421004905313,15.7008782099779,3.6564805458821));
#86415=CARTESIAN_POINT('Ctrl Pts',(-8.54963799199644,15.6985878862357,3.70065164209107));
#86416=CARTESIAN_POINT('Ctrl Pts',(-8.58042128618632,15.6892946397258,3.88231352972219));
#86417=CARTESIAN_POINT('Ctrl Pts',(-8.62338799325155,15.6828257351684,4.01604217549472));
#86418=CARTESIAN_POINT('Ctrl Pts',(-8.69775304316821,15.67418039309,4.16848909254152));
#86419=CARTESIAN_POINT('Ctrl Pts',(-8.71166958822675,15.6726267268869,4.19493115536883));
#86420=CARTESIAN_POINT('Ctrl Pts',(-8.72929477232807,15.6707097584033,4.22606843950203));
#86421=CARTESIAN_POINT('Ctrl Pts',(-8.73223613823896,15.6703914120714,4.2311921381551));
#86422=CARTESIAN_POINT('Ctrl Pts',(-8.73685031861745,15.669894200767,4.23911824714436));
#86423=CARTESIAN_POINT('Ctrl Pts',(-8.73850165447372,15.6697166824403,4.24193316723761));
#86424=CARTESIAN_POINT('Ctrl Pts',(-8.74158062575843,15.6693864328612,4.24714168401531));
#86425=CARTESIAN_POINT('Ctrl Pts',(-8.74300569057353,15.6692338661648,4.24953673902448));
#86426=CARTESIAN_POINT('Ctrl Pts',(-8.74625320548167,15.6688868386015,4.2549594114311));
#86427=CARTESIAN_POINT('Ctrl Pts',(-8.74807977706318,15.6686921146338,4.25798449359756));
#86428=CARTESIAN_POINT('Ctrl Pts',(-8.75366458833495,15.6680982076117,4.26715854031814));
#86429=CARTESIAN_POINT('Ctrl Pts',(-8.75745724829173,15.6676968819776,4.27328629251207));
#86430=CARTESIAN_POINT('Ctrl Pts',(-8.79269555816046,15.663988039685,4.32929177949537));
#86431=CARTESIAN_POINT('Ctrl Pts',(-8.82708051377024,15.6605146009096,4.37724987258664));
#86432=CARTESIAN_POINT('Ctrl Pts',(-8.90792462825394,15.65284891439,4.47672775812324));
#86433=CARTESIAN_POINT('Ctrl Pts',(-8.9553488470132,15.6486486352057,4.52729259636271));
#86434=CARTESIAN_POINT('Ctrl Pts',(-9.06058626698526,15.6401093348475,4.62464592604532));
#86435=CARTESIAN_POINT('Ctrl Pts',(-9.11874923704675,15.6357952075521,4.67078018011592));
#86436=CARTESIAN_POINT('Ctrl Pts',(-9.19380005005272,15.6307346876338,4.72153380011897));
#86437=CARTESIAN_POINT('Ctrl Pts',(-9.20758996838148,15.6298238015158,4.73052409851194));
#86438=CARTESIAN_POINT('Ctrl Pts',(-9.22744690372434,15.628538410048,4.74299750751416));
#86439=CARTESIAN_POINT('Ctrl Pts',(-9.23339139889537,15.6281568898385,4.74667250925717));
#86440=CARTESIAN_POINT('Ctrl Pts',(-9.24371087512879,15.6275001662113,4.75295048634648));
#86441=CARTESIAN_POINT('Ctrl Pts',(-9.2480734976975,15.6272242387452,4.75557345371734));
#86442=CARTESIAN_POINT('Ctrl Pts',(-9.25646864039173,15.6266964931476,4.7605614703379));
#86443=CARTESIAN_POINT('Ctrl Pts',(-9.26049897486578,15.6264445493617,4.76293006051219));
#86444=CARTESIAN_POINT('Ctrl Pts',(-9.2710495673999,15.6257886593534,4.76906272396085));
#86445=CARTESIAN_POINT('Ctrl Pts',(-9.27758769070849,15.6253858234389,4.772795894396));
#86446=CARTESIAN_POINT('Ctrl Pts',(-9.30025764662855,15.624001229463,4.78550914255081));
#86447=CARTESIAN_POINT('Ctrl Pts',(-9.3165307659428,15.6230284784064,4.79423450852946));
#86448=CARTESIAN_POINT('Ctrl Pts',(-9.44652115950057,15.6154132737831,4.86079738618215));
#86449=CARTESIAN_POINT('Ctrl Pts',(-9.56718702467038,15.6093343751655,4.90384570117857));
#86450=CARTESIAN_POINT('Ctrl Pts',(-9.74106357654327,15.6006332533548,4.94128835746997));
#86451=CARTESIAN_POINT('Ctrl Pts',(-9.79072531439699,15.5981458523097,4.94933213674936));
#86452=CARTESIAN_POINT('Ctrl Pts',(-9.86464256444154,15.5943203931647,4.95742608584392));
#86453=CARTESIAN_POINT('Ctrl Pts',(-9.88864611261351,15.5930589774026,4.95945627174356));
#86454=CARTESIAN_POINT('Ctrl Pts',(-9.91822290140941,15.5914695019034,4.96122397583003));
#86455=CARTESIAN_POINT('Ctrl Pts',(-9.92376016404684,15.5911704115556,4.96152334460419));
#86456=CARTESIAN_POINT('Ctrl Pts',(-9.93247945188097,15.5906968799903,4.96194506228082));
#86457=CARTESIAN_POINT('Ctrl Pts',(-9.93566046174225,15.5905235865287,4.96208851064688));
#86458=CARTESIAN_POINT('Ctrl Pts',(-9.94163765026828,15.5901969129296,4.96233850941591));
#86459=CARTESIAN_POINT('Ctrl Pts',(-9.94443367996392,15.5900436643959,4.96244742251341));
#86460=CARTESIAN_POINT('Ctrl Pts',(-9.95081944450417,15.5896926813833,4.96267782642178));
#86461=CARTESIAN_POINT('Ctrl Pts',(-9.95440932271794,15.5894946631836,4.96279412103113));
#86462=CARTESIAN_POINT('Ctrl Pts',(-9.96393536875779,15.5889673968527,4.96306761816576));
#86463=CARTESIAN_POINT('Ctrl Pts',(-9.96987206483511,15.5886369382967,4.96320190610689));
#86464=CARTESIAN_POINT('Ctrl Pts',(-10.0121984731203,15.5862684104015,4.96390162932665));
#86465=CARTESIAN_POINT('Ctrl Pts',(-10.0485946349193,15.5841661930598,4.9631455567877));
#86466=CARTESIAN_POINT('Ctrl Pts',(-10.0972051187587,15.5813030802851,4.96032010489185));
#86467=CARTESIAN_POINT('Ctrl Pts',(-10.109478904138,15.5805753972936,4.95945126767905));
#86468=CARTESIAN_POINT('Ctrl Pts',(-10.2112193692979,15.574510864254,4.95095863657535));
#86469=CARTESIAN_POINT('Ctrl Pts',(-10.2998223154583,15.5690352706318,4.93527077762637));
#86470=CARTESIAN_POINT('Ctrl Pts',(-10.450266348908,15.5597943973382,4.89408490209033));
#86471=CARTESIAN_POINT('Ctrl Pts',(-10.5128477234004,15.5559650170763,4.87229790641708));
#86472=CARTESIAN_POINT('Ctrl Pts',(-10.588027787757,15.551407305756,4.84025989483278));
#86473=CARTESIAN_POINT('Ctrl Pts',(-10.6022123035343,15.5505490530019,4.8339466377807));
#86474=CARTESIAN_POINT('Ctrl Pts',(-10.622485995773,15.5493244021479,4.82453389515986));
#86475=CARTESIAN_POINT('Ctrl Pts',(-10.6286577948156,15.5489518617864,4.8216157662461));
#86476=CARTESIAN_POINT('Ctrl Pts',(-10.6393704267743,15.548305645153,4.81645863425174));
#86477=CARTESIAN_POINT('Ctrl Pts',(-10.6439204444234,15.548031306755,4.8142390728015));
#86478=CARTESIAN_POINT('Ctrl Pts',(-10.6526840809335,15.5475031353315,4.80990761268122));
#86479=CARTESIAN_POINT('Ctrl Pts',(-10.656899188971,15.5472491971318,4.80779888343309));
#86480=CARTESIAN_POINT('Ctrl Pts',(-10.6680054172211,15.5465803298333,4.80217543051707));
#86481=CARTESIAN_POINT('Ctrl Pts',(-10.6748790368415,15.5461665998545,4.79862634272655));
#86482=CARTESIAN_POINT('Ctrl Pts',(-10.6991563963623,15.5447058687563,4.78584628620261));
#86483=CARTESIAN_POINT('Ctrl Pts',(-10.7164019496999,15.5436692704866,4.77631839031584));
#86484=CARTESIAN_POINT('Ctrl Pts',(-10.8426883036775,15.5360741976743,4.70318075718056));
#86485=CARTESIAN_POINT('Ctrl Pts',(-10.9432777160316,15.5300605192592,4.62605329344906));
#86486=CARTESIAN_POINT('Ctrl Pts',(-11.0681557927213,15.5214370382806,4.50168644538353));
#86487=CARTESIAN_POINT('Ctrl Pts',(-11.1017517380528,15.5189625191717,4.46461131243999));
#86488=CARTESIAN_POINT('Ctrl Pts',(-11.1485692807684,15.5151549232385,4.40730210538272));
#86489=CARTESIAN_POINT('Ctrl Pts',(-11.1632958109638,15.5138976571113,4.38834184125282));
#86490=CARTESIAN_POINT('Ctrl Pts',(-11.1808379498359,15.5123128423391,4.36457195935395));
#86491=CARTESIAN_POINT('Ctrl Pts',(-11.184101962443,15.5120140622116,4.36009620231301));
#86492=CARTESIAN_POINT('Ctrl Pts',(-11.1892012894379,15.511540912511,4.35301973866309));
#86493=CARTESIAN_POINT('Ctrl Pts',(-11.1910536976845,15.5113676876021,4.35043134360479));
#86494=CARTESIAN_POINT('Ctrl Pts',(-11.1945188348553,15.5110410685088,4.34555593223225));
#86495=CARTESIAN_POINT('Ctrl Pts',(-11.1961334560194,15.5108878053789,4.34327032219734));
#86496=CARTESIAN_POINT('Ctrl Pts',(-11.1998066678057,15.5105366922791,4.33803885693779));
#86497=CARTESIAN_POINT('Ctrl Pts',(-11.2018609677618,15.5103385578114,4.3350900427211));
#86498=CARTESIAN_POINT('Ctrl Pts',(-11.2072848170796,15.5098107805893,4.32724299162193));
#86499=CARTESIAN_POINT('Ctrl Pts',(-11.2106353797506,15.5094799237671,4.32233178923502));
#86500=CARTESIAN_POINT('Ctrl Pts',(-11.2343754024269,15.507101677208,4.28707447836635));
#86501=CARTESIAN_POINT('Ctrl Pts',(-11.2536498382057,15.504989558406,4.25599637727083));
#86502=CARTESIAN_POINT('Ctrl Pts',(-11.3168208868424,15.4974822733556,4.14506910678062));
#86503=CARTESIAN_POINT('Ctrl Pts',(-11.3544123653171,15.4919203340701,4.06187075066631));
#86504=CARTESIAN_POINT('Ctrl Pts',(-11.4111113944972,15.4815221562677,3.8969137613648));
#86505=CARTESIAN_POINT('Ctrl Pts',(-11.4314211491093,15.4766826516192,3.81593204748348));
#86506=CARTESIAN_POINT('Ctrl Pts',(-11.4465582022554,15.4714323971834,3.7223353357576));
#86507=CARTESIAN_POINT('Ctrl Pts',(-11.4482552171472,15.470801840148,3.71099874538706));
#86508=CARTESIAN_POINT('Ctrl Pts',(-11.4506434433598,15.4698451534468,3.69365532327172));
#86509=CARTESIAN_POINT('Ctrl Pts',(-11.4514308860396,15.4695160236494,3.68766237922612));
#86510=CARTESIAN_POINT('Ctrl Pts',(-11.452798157936,15.4689183658172,3.67673275499461));
#86511=CARTESIAN_POINT('Ctrl Pts',(-11.4533900055018,15.4686494658813,3.67179769248364));
#86512=CARTESIAN_POINT('Ctrl Pts',(-11.4546162371738,15.4680693105584,3.66111273916939));
#86513=CARTESIAN_POINT('Ctrl Pts',(-11.4552416964148,15.4677583379078,3.65536189528));
#86514=CARTESIAN_POINT('Ctrl Pts',(-11.4568527151101,15.4669140224848,3.63968503918302));
#86515=CARTESIAN_POINT('Ctrl Pts',(-11.4577709306515,15.4663827805759,3.62975231805008));
#86516=CARTESIAN_POINT('Ctrl Pts',(-11.4618609702844,15.4637373491525,3.57995981190155));
#86517=CARTESIAN_POINT('Ctrl Pts',(-11.4634999999999,15.4616710633252,3.53998959100317));
#86518=CARTESIAN_POINT('Ctrl Pts',(-11.4635,15.4596442608852,3.50000000000481));
#86519=CARTESIAN_POINT('Ctrl Pts',(-11.4635,15.3905155741067,3.49999999999573));
#86520=CARTESIAN_POINT('Ctrl Pts',(-11.4635,15.3924479265974,3.53377287519692));
#86521=CARTESIAN_POINT('Ctrl Pts',(-11.4623309559757,15.3943469930721,3.56753745619958));
#86522=CARTESIAN_POINT('Ctrl Pts',(-11.4593343437384,15.3967366095462,3.61075474225848));
#86523=CARTESIAN_POINT('Ctrl Pts',(-11.4585810250861,15.3972601693145,3.62026944362245));
#86524=CARTESIAN_POINT('Ctrl Pts',(-11.4572352147539,15.3980880983137,3.63538649531933));
#86525=CARTESIAN_POINT('Ctrl Pts',(-11.4567033698223,15.3983943456444,3.64099385738379));
#86526=CARTESIAN_POINT('Ctrl Pts',(-11.4556895848887,15.398942808918,3.65106364886));
#86527=CARTESIAN_POINT('Ctrl Pts',(-11.4552194652323,15.3991853897264,3.65552717508704));
#86528=CARTESIAN_POINT('Ctrl Pts',(-11.4540705446105,15.3997519316809,3.66597397536798));
#86529=CARTESIAN_POINT('Ctrl Pts',(-11.4533753318413,15.4000753767965,3.67195538805569));
#86530=CARTESIAN_POINT('Ctrl Pts',(-11.4512635768085,15.4010050542376,3.68919579279601));
#86531=CARTESIAN_POINT('Ctrl Pts',(-11.4497529607197,15.4016083459921,3.70044295928912));
#86532=CARTESIAN_POINT('Ctrl Pts',(-11.4368121949794,15.406333954281,3.7889747726702));
#86533=CARTESIAN_POINT('Ctrl Pts',(-11.4193406955769,15.4102562796685,3.86525297622746));
#86534=CARTESIAN_POINT('Ctrl Pts',(-11.3638911721045,15.4193170126255,4.041249878645));
#86535=CARTESIAN_POINT('Ctrl Pts',(-11.3209561715124,15.4243479523232,4.13892219510135));
#86536=CARTESIAN_POINT('Ctrl Pts',(-11.2540427537917,15.4311945194401,4.25496342070717));
#86537=CARTESIAN_POINT('Ctrl Pts',(-11.239592920001,15.4326315102702,4.27846142762621));
#86538=CARTESIAN_POINT('Ctrl Pts',(-11.2214889166481,15.4344015119695,4.30611852669048));
#86539=CARTESIAN_POINT('Ctrl Pts',(-11.2184633412356,15.4346963623763,4.31068448655606));
#86540=CARTESIAN_POINT('Ctrl Pts',(-11.2134670953802,15.4351818928509,4.31813327277118));
#86541=CARTESIAN_POINT('Ctrl Pts',(-11.2115115850846,15.4353715910389,4.32102626162252));
#86542=CARTESIAN_POINT('Ctrl Pts',(-11.2079777548484,15.4357138482009,4.32621410738476));
#86543=CARTESIAN_POINT('Ctrl Pts',(-11.2064032212908,15.435866153749,4.32851148146362));
#86544=CARTESIAN_POINT('Ctrl Pts',(-11.2029497958787,15.4361998010226,4.33351959580938));
#86545=CARTESIAN_POINT('Ctrl Pts',(-11.2010683191604,15.4363813130443,4.33622844980883));
#86546=CARTESIAN_POINT('Ctrl Pts',(-11.1957008974664,15.4368983250465,4.34390070573417));
#86547=CARTESIAN_POINT('Ctrl Pts',(-11.1921932740865,15.4372352449728,4.34884876859077));
#86548=CARTESIAN_POINT('Ctrl Pts',(-11.1694627667194,15.4394117895475,4.3804949739973));
#86549=CARTESIAN_POINT('Ctrl Pts',(-11.1493763375795,15.4413041163679,4.40655847569105));
#86550=CARTESIAN_POINT('Ctrl Pts',(-11.075710044139,15.4480767624132,4.49575841135937));
#86551=CARTESIAN_POINT('Ctrl Pts',(-11.0176691443843,15.4531145791447,4.55500516851086));
#86552=CARTESIAN_POINT('Ctrl Pts',(-10.8825252638254,15.4638053838747,4.67137149085821));
#86553=CARTESIAN_POINT('Ctrl Pts',(-10.804177403668,15.469400059251,4.72648527052344));
#86554=CARTESIAN_POINT('Ctrl Pts',(-10.71171615676,15.4752880042463,4.77883003245339));
#86555=CARTESIAN_POINT('Ctrl Pts',(-10.702371809612,15.475875792682,4.78398597704378));
#86556=CARTESIAN_POINT('Ctrl Pts',(-10.6872828738873,15.4768135090254,4.79209760358683));
#86557=CARTESIAN_POINT('Ctrl Pts',(-10.6815737793313,15.4771657157405,4.79511819967667));
#86558=CARTESIAN_POINT('Ctrl Pts',(-10.6713885960845,15.4777895262364,4.80042102555505));
#86559=CARTESIAN_POINT('Ctrl Pts',(-10.6669204265679,15.4780616493522,4.80271817219173));
#86560=CARTESIAN_POINT('Ctrl Pts',(-10.6575695297175,15.4786279755011,4.80746487655657));
#86561=CARTESIAN_POINT('Ctrl Pts',(-10.6526847320212,15.4789220281408,4.80991019980008));
#86562=CARTESIAN_POINT('Ctrl Pts',(-10.6399178175918,15.4796859766753,4.81621215444183));
#86563=CARTESIAN_POINT('Ctrl Pts',(-10.6320144393242,15.4801543697673,4.82002537921713));
#86564=CARTESIAN_POINT('Ctrl Pts',(-10.5968783948047,15.4822172516288,4.83658992258273));
#86565=CARTESIAN_POINT('Ctrl Pts',(-10.5692898427104,15.4837854256293,4.84857171850007));
#86566=CARTESIAN_POINT('Ctrl Pts',(-10.4934484355024,15.4879757278688,4.87876728120516));
#86567=CARTESIAN_POINT('Ctrl Pts',(-10.444569961316,15.4905461529664,4.895295191772));
#86568=CARTESIAN_POINT('Ctrl Pts',(-10.2969866506334,15.4980769237978,4.9366541124906));
#86569=CARTESIAN_POINT('Ctrl Pts',(-10.1964688735872,15.5028957923717,4.95381334171361));
#86570=CARTESIAN_POINT('Ctrl Pts',(-10.0622136362668,15.5097181210195,4.96254597188032));
#86571=CARTESIAN_POINT('Ctrl Pts',(-10.029374494844,15.5114188551345,4.96357373684852));
#86572=CARTESIAN_POINT('Ctrl Pts',(-9.99076287140086,15.513484179312,4.9634822165618));
#86573=CARTESIAN_POINT('Ctrl Pts',(-9.98499486145552,15.5137944321807,4.96343444211142));
#86574=CARTESIAN_POINT('Ctrl Pts',(-9.97564757487826,15.5143002157791,4.96330175527143));
#86575=CARTESIAN_POINT('Ctrl Pts',(-9.97206800674776,15.5144946217253,4.96323780390823));
#86576=CARTESIAN_POINT('Ctrl Pts',(-9.96569774405163,15.5148419181339,4.96310061122072));
#86577=CARTESIAN_POINT('Ctrl Pts',(-9.96290698694573,15.5149945217354,4.96303251896967));
#86578=CARTESIAN_POINT('Ctrl Pts',(-9.95688505362365,15.5153248107346,4.96286834702902));
#86579=CARTESIAN_POINT('Ctrl Pts',(-9.95365404315212,15.5155026395728,4.96276954822251));
#86580=CARTESIAN_POINT('Ctrl Pts',(-9.94466440782513,15.5159990746492,4.96246484626167));
#86581=CARTESIAN_POINT('Ctrl Pts',(-9.93890669713507,15.516318931364,4.96223563778122));
#86582=CARTESIAN_POINT('Ctrl Pts',(-9.90583520968154,15.5181664669529,4.96072342770647));
#86583=CARTESIAN_POINT('Ctrl Pts',(-9.8785619372936,15.5197304924079,4.95870920324859));
#86584=CARTESIAN_POINT('Ctrl Pts',(-9.78946400237685,15.524938313691,4.94961314248932));
#86585=CARTESIAN_POINT('Ctrl Pts',(-9.72803416839514,15.528682294912,4.93935313746615));
#86586=CARTESIAN_POINT('Ctrl Pts',(-9.55605141058428,15.5393178488581,4.89922355911073));
#86587=CARTESIAN_POINT('Ctrl Pts',(-9.44806758836559,15.5461457541195,4.86025589123931));
#86588=CARTESIAN_POINT('Ctrl Pts',(-9.33077783421074,15.5534764736581,4.80163464799671));
#86589=CARTESIAN_POINT('Ctrl Pts',(-9.31597017330557,15.5544012729764,4.79391432973713));
#86590=CARTESIAN_POINT('Ctrl Pts',(-9.29557609920256,15.5556744198301,4.7828334323548));
#86591=CARTESIAN_POINT('Ctrl Pts',(-9.28987551343262,15.5560302344369,4.77968662674915));
#86592=CARTESIAN_POINT('Ctrl Pts',(-9.28007552885593,15.5566418724905,4.77419124288742));
#86593=CARTESIAN_POINT('Ctrl Pts',(-9.275966183373,15.5568983305095,4.77186068447477));
#86594=CARTESIAN_POINT('Ctrl Pts',(-9.26748039705959,15.5574279114339,4.76699363342391));
#86595=CARTESIAN_POINT('Ctrl Pts',(-9.26310567267965,15.5577009269031,4.7644542645264));
#86596=CARTESIAN_POINT('Ctrl Pts',(-9.25288692263474,15.5583386904326,4.75845160609522));
#86597=CARTESIAN_POINT('Ctrl Pts',(-9.24705364275756,15.5587027803744,4.75497019107539));
#86598=CARTESIAN_POINT('Ctrl Pts',(-9.22813877838497,15.5598836274135,4.74350207582798));
#86599=CARTESIAN_POINT('Ctrl Pts',(-9.21515813779132,15.5606943945906,4.73535032794443));
#86600=CARTESIAN_POINT('Ctrl Pts',(-9.14818165004608,15.5648834933773,4.69180769531754));
#86601=CARTESIAN_POINT('Ctrl Pts',(-9.09644055774671,15.5681351977014,4.65307486203232));
#86602=CARTESIAN_POINT('Ctrl Pts',(-8.97104608087096,15.5762814416564,4.54556556398651));
#86603=CARTESIAN_POINT('Ctrl Pts',(-8.90163085381228,15.5810477380525,4.47238705418304));
#86604=CARTESIAN_POINT('Ctrl Pts',(-8.8161201283604,15.588093134494,4.3612947554924));
#86605=CARTESIAN_POINT('Ctrl Pts',(-8.79325274604905,15.5901275494179,4.32895159931876));
#86606=CARTESIAN_POINT('Ctrl Pts',(-8.76842762291223,15.5925672241003,4.29063173842885));
#86607=CARTESIAN_POINT('Ctrl Pts',(-8.76516034514825,15.5928933171649,4.28551899409216));
#86608=CARTESIAN_POINT('Ctrl Pts',(-8.75998919636404,15.5934177458523,4.2773150173647));
#86609=CARTESIAN_POINT('Ctrl Pts',(-8.75806483644245,15.5936147851654,4.27423670688957));
#86610=CARTESIAN_POINT('Ctrl Pts',(-8.75467460677688,15.5939653306117,4.26876835006387));
#86611=CARTESIAN_POINT('Ctrl Pts',(-8.75320412777754,15.5941185333728,4.26638121322627));
#86612=CARTESIAN_POINT('Ctrl Pts',(-8.75008932403682,15.5944455449542,4.26129203105642));
#86613=CARTESIAN_POINT('Ctrl Pts',(-8.74844692272374,15.5946194678516,4.25858891951134));
#86614=CARTESIAN_POINT('Ctrl Pts',(-8.74400053585063,15.5950943599629,4.25121718204668));
#86615=CARTESIAN_POINT('Ctrl Pts',(-8.74121385538734,15.5953964125454,4.24653824333437));
#86616=CARTESIAN_POINT('Ctrl Pts',(-8.72693573011277,15.5969666892207,4.22225750245936));
#86617=CARTESIAN_POINT('Ctrl Pts',(-8.71587640171128,15.5982598931284,4.20240657852535));
#86618=CARTESIAN_POINT('Ctrl Pts',(-8.68393366634153,15.6022183756158,4.14179349206602));
#86619=CARTESIAN_POINT('Ctrl Pts',(-8.664497682262,15.6049404550471,4.100302032205));
#86620=CARTESIAN_POINT('Ctrl Pts',(-8.62396026863709,15.6113170174828,4.00200742882423));
#86621=CARTESIAN_POINT('Ctrl Pts',(-8.60437453957507,15.6149819432937,3.94466464749764));
#86622=CARTESIAN_POINT('Ctrl Pts',(-8.56644434643042,15.6235512380044,3.80605199561006));
#86623=CARTESIAN_POINT('Ctrl Pts',(-8.55136816441418,15.6283846408657,3.72409612057871));
#86624=CARTESIAN_POINT('Ctrl Pts',(-8.54230231722548,15.6335888365207,3.63063094936023));
#86625=CARTESIAN_POINT('Ctrl Pts',(-8.54138527165353,15.6341788230113,3.61995858504686));
#86626=CARTESIAN_POINT('Ctrl Pts',(-8.54010233182435,15.6351193544361,3.60282467234005));
#86627=CARTESIAN_POINT('Ctrl Pts',(-8.53966199526193,15.635472199962,3.59636923049541));
#86628=CARTESIAN_POINT('Ctrl Pts',(-8.53895572271467,15.6360967430292,3.5848948022735));
#86629=CARTESIAN_POINT('Ctrl Pts',(-8.53867280400491,15.6363689640888,3.57987699769955));
#86630=CARTESIAN_POINT('Ctrl Pts',(-8.53813660442161,15.6369350998103,3.56940780191909));
#86631=CARTESIAN_POINT('Ctrl Pts',(-8.53788795564795,15.6372288665142,3.56395624417164));
#86632=CARTESIAN_POINT('Ctrl Pts',(-8.53732001545623,15.6379912173924,3.54976020611194));
#86633=CARTESIAN_POINT('Ctrl Pts',(-8.53704864221797,15.6384583106285,3.54101395546865));
#86634=CARTESIAN_POINT('Ctrl Pts',(-8.53619814278807,15.6405070733441,3.50244653962598));
#86635=CARTESIAN_POINT('Ctrl Pts',(-8.53645226202916,15.642062880952,3.47261308286535));
#86636=CARTESIAN_POINT('Ctrl Pts',(-8.53960900223283,15.6462106101044,3.39189791822188));
#86637=CARTESIAN_POINT('Ctrl Pts',(-8.54425711986274,15.6487522018452,3.34112543266745));
#86638=CARTESIAN_POINT('Ctrl Pts',(-8.56406109833577,15.6555595437033,3.20407496090257));
#86639=CARTESIAN_POINT('Ctrl Pts',(-8.58432221753983,15.6597325453229,3.11875539523684));
#86640=CARTESIAN_POINT('Ctrl Pts',(-8.61552706984217,15.664635148724,3.02546354358181));
#86641=CARTESIAN_POINT('Ctrl Pts',(-8.61908574053981,15.6651791804299,3.01520525611983));
#86642=CARTESIAN_POINT('Ctrl Pts',(-8.63517257446305,15.66757819518,2.97044786416266));
#86643=CARTESIAN_POINT('Ctrl Pts',(-8.64888097643546,15.6694700723622,2.93638991456549));
#86644=CARTESIAN_POINT('Ctrl Pts',(-8.66628237545294,15.6717499116966,2.89745126097008));
#86645=CARTESIAN_POINT('Ctrl Pts',(-8.66874420616607,15.6720699277985,2.89203150253327));
#86646=CARTESIAN_POINT('Ctrl Pts',(-8.67274640548649,15.6725864221828,2.88336146576302));
#86647=CARTESIAN_POINT('Ctrl Pts',(-8.67426583702232,15.6727816653516,2.88010152879236));
#86648=CARTESIAN_POINT('Ctrl Pts',(-8.67698930800257,15.6731301932463,2.87431413907305));
#86649=CARTESIAN_POINT('Ctrl Pts',(-8.67818860014775,15.6732831870255,2.87178450287929));
#86650=CARTESIAN_POINT('Ctrl Pts',(-8.6807670514305,15.6736111148596,2.86638591400915));
#86651=CARTESIAN_POINT('Ctrl Pts',(-8.68214829265891,15.6737861716274,2.86351806025893));
#86652=CARTESIAN_POINT('Ctrl Pts',(-8.68595792046577,15.6742672926443,2.85567374288215));
#86653=CARTESIAN_POINT('Ctrl Pts',(-8.68840518630778,15.6745744875118,2.85070657243267));
#86654=CARTESIAN_POINT('Ctrl Pts',(-8.70159037638528,15.6762192293733,2.82432356741786));
#86655=CARTESIAN_POINT('Ctrl Pts',(-8.71282418329001,15.6775845926265,2.80316108573879));
#86656=CARTESIAN_POINT('Ctrl Pts',(-8.74901075838211,15.6818554277292,2.73885506361895));
#86657=CARTESIAN_POINT('Ctrl Pts',(-8.77565088384762,15.6848275664704,2.69670407498942));
#86658=CARTESIAN_POINT('Ctrl Pts',(-8.87668053444641,15.6953525156578,2.55358571325118));
#86659=CARTESIAN_POINT('Ctrl Pts',(-8.96184800919518,15.7029216242198,2.46086687780801));
#86660=CARTESIAN_POINT('Ctrl Pts',(-9.07348741503224,15.7111253482019,2.36693918181937));
#86661=CARTESIAN_POINT('Ctrl Pts',(-9.08944786051499,15.7122649183693,2.35407362846749));
#86662=CARTESIAN_POINT('Ctrl Pts',(-9.1118960180913,15.713823116112,2.3367436415362));
#86663=CARTESIAN_POINT('Ctrl Pts',(-9.11815681938413,15.7142530423524,2.33199030553167));
#86664=CARTESIAN_POINT('Ctrl Pts',(-9.12825215470888,15.7149389476004,2.3244531522515));
#86665=CARTESIAN_POINT('Ctrl Pts',(-9.13206238094477,15.7151961723969,2.32163715809377));
#86666=CARTESIAN_POINT('Ctrl Pts',(-9.13996213077413,15.7157261023629,2.31585785579372));
#86667=CARTESIAN_POINT('Ctrl Pts',(-9.14405345692767,15.7159987068053,2.3128971104097));
#86668=CARTESIAN_POINT('Ctrl Pts',(-9.15364304932451,15.7166333996662,2.30603281916753));
#86669=CARTESIAN_POINT('Ctrl Pts',(-9.15915315594597,15.716994848937,2.30214595890034));
#86670=CARTESIAN_POINT('Ctrl Pts',(-9.17704522828503,15.7181582626773,2.28970908349303));
#86671=CARTESIAN_POINT('Ctrl Pts',(-9.18953246270674,15.7189544850009,2.28131174944742));
#86672=CARTESIAN_POINT('Ctrl Pts',(-9.25439424112042,15.7230135807754,2.2391318698669));
#86673=CARTESIAN_POINT('Ctrl Pts',(-9.3087607640867,15.7261589077104,2.20852571380866));
#86674=CARTESIAN_POINT('Ctrl Pts',(-9.44100944242262,15.7334112402951,2.1448265891744));
#86675=CARTESIAN_POINT('Ctrl Pts',(-9.52012820983936,15.7374455024037,2.11483286518537));
#86676=CARTESIAN_POINT('Ctrl Pts',(-9.65683569730927,15.7444576959922,2.07613518234008));
#86677=CARTESIAN_POINT('Ctrl Pts',(-9.71315402196966,15.7473611747843,2.0637302645995));
#86678=CARTESIAN_POINT('Ctrl Pts',(-9.7771544582214,15.7508190292898,2.05354783613727));
#86679=CARTESIAN_POINT('Ctrl Pts',(-9.784266795475,15.7512054847457,2.05246997334373));
#86680=CARTESIAN_POINT('Ctrl Pts',(-9.79488250863763,15.7517859345523,2.05094115396298));
#86681=CARTESIAN_POINT('Ctrl Pts',(-9.79838014731786,15.7519777668717,2.0504503599358));
#86682=CARTESIAN_POINT('Ctrl Pts',(-9.80464157527021,15.7523222867186,2.04959484714745));
#86683=CARTESIAN_POINT('Ctrl Pts',(-9.80740466244638,15.7524747056307,2.04922535956782));
#86684=CARTESIAN_POINT('Ctrl Pts',(-9.81340828430043,15.7528067325372,2.04843999253055));
#86685=CARTESIAN_POINT('Ctrl Pts',(-9.81664911696382,15.7529864981792,2.04802707431856));
#86686=CARTESIAN_POINT('Ctrl Pts',(-9.82576724769338,15.7534937177388,2.04689633677292));
#86687=CARTESIAN_POINT('Ctrl Pts',(-9.83164748933168,15.7538225097363,2.04620333685724));
#86688=CARTESIAN_POINT('Ctrl Pts',(-9.8674332102233,15.7558330458244,2.04220592855481));
#86689=CARTESIAN_POINT('Ctrl Pts',(-9.89742860693153,15.757558849874,2.03978893259091));
#86690=CARTESIAN_POINT('Ctrl Pts',(-10.0700758681224,15.7676452210945,2.03122271221597));
#86691=CARTESIAN_POINT('Ctrl Pts',(-10.2129520125314,15.7764955200935,2.04505024830482));
#86692=CARTESIAN_POINT('Ctrl Pts',(-10.391949115939,15.7871380350668,2.08934854924332));
#86693=CARTESIAN_POINT('Ctrl Pts',(-10.4318753627286,15.7894898873021,2.10105547516521));
#86694=CARTESIAN_POINT('Ctrl Pts',(-10.4807950875598,15.7923440815215,2.11769397573293));
#86695=CARTESIAN_POINT('Ctrl Pts',(-10.4903047977213,15.7928976528069,2.12103840755994));
#86696=CARTESIAN_POINT('Ctrl Pts',(-10.5052401058005,15.793765195711,2.12646498340331));
#86697=CARTESIAN_POINT('Ctrl Pts',(-10.5106890359732,15.7940813136363,2.12848160193782));
#86698=CARTESIAN_POINT('Ctrl Pts',(-10.5207328809838,15.7946633199977,2.13226692811116));
#86699=CARTESIAN_POINT('Ctrl Pts',(-10.5253311411677,15.7949295069913,2.13402647089481));
#86700=CARTESIAN_POINT('Ctrl Pts',(-10.5353999501252,15.7955118265018,2.1379377038491));
#86701=CARTESIAN_POINT('Ctrl Pts',(-10.5408666057631,15.7958276268652,2.1400992237151));
#86702=CARTESIAN_POINT('Ctrl Pts',(-10.5563099272839,15.7967188357942,2.14631337864954));
#86703=CARTESIAN_POINT('Ctrl Pts',(-10.5662552114978,15.797291656807,2.15044331436572));
#86704=CARTESIAN_POINT('Ctrl Pts',(-10.5885494183519,15.7985737529293,2.15999117406386));
#86705=CARTESIAN_POINT('Ctrl Pts',(-10.6008709390954,15.7992809450882,2.16547079409635));
#86706=CARTESIAN_POINT('Ctrl Pts',(-10.6783705440249,15.8037235931014,2.20122736371009));
#86707=CARTESIAN_POINT('Ctrl Pts',(-10.7413235716121,15.8073011911491,2.23610216141011));
#86708=CARTESIAN_POINT('Ctrl Pts',(-10.8576563601416,15.8141059563843,2.31224239230292));
#86709=CARTESIAN_POINT('Ctrl Pts',(-10.9112497687661,15.8173341225055,2.35284434744152));
#86710=CARTESIAN_POINT('Ctrl Pts',(-11.0059088938757,15.8235288414033,2.43538991877264));
#86711=CARTESIAN_POINT('Ctrl Pts',(-11.0476087806386,15.8264708651137,2.47639767023548));
#86712=CARTESIAN_POINT('Ctrl Pts',(-11.0915652211292,15.8299725518948,2.52513103943536));
#86713=CARTESIAN_POINT('Ctrl Pts',(-11.096349464391,15.8303594643826,2.53051458497907));
#86714=CARTESIAN_POINT('Ctrl Pts',(-11.1034214378828,15.8309404690736,2.5385917271441));
#86715=CARTESIAN_POINT('Ctrl Pts',(-11.1057395363231,15.8311323931747,2.54125873460491));
#86716=CARTESIAN_POINT('Ctrl Pts',(-11.1098691707229,15.8314770111753,2.54604484062238));
#86717=CARTESIAN_POINT('Ctrl Pts',(-11.1116843322156,15.8316294358075,2.54816074489119));
#86718=CARTESIAN_POINT('Ctrl Pts',(-11.1156127399841,15.8319613968301,2.55276659178419));
#86719=CARTESIAN_POINT('Ctrl Pts',(-11.1177236723323,15.8321410903424,2.5552583913402));
#86720=CARTESIAN_POINT('Ctrl Pts',(-11.123634503141,15.8326479068886,2.56228322976308));
#86721=CARTESIAN_POINT('Ctrl Pts',(-11.1274152406231,15.8329763646806,2.56683221733516));
#86722=CARTESIAN_POINT('Ctrl Pts',(-11.1501898824591,15.8349804605761,2.59457512067511));
#86723=CARTESIAN_POINT('Ctrl Pts',(-11.1684937796426,15.8366998393674,2.61832374942014));
#86724=CARTESIAN_POINT('Ctrl Pts',(-11.2185616993983,15.8416859341888,2.68758472845355));
#86725=CARTESIAN_POINT('Ctrl Pts',(-11.2484838545116,15.845018768198,2.73436388773581));
#86726=CARTESIAN_POINT('Ctrl Pts',(-11.3027327595979,15.851683454617,2.83084593066268));
#86727=CARTESIAN_POINT('Ctrl Pts',(-11.3270457184486,15.855009783153,2.88045991990366));
#86728=CARTESIAN_POINT('Ctrl Pts',(-11.376122882885,15.8624873419584,2.99683760341718));
#86729=CARTESIAN_POINT('Ctrl Pts',(-11.3989404602103,15.8665876788832,3.06427704862729));
#86730=CARTESIAN_POINT('Ctrl Pts',(-11.4193979278188,15.8711082217035,3.14327613881463));
#86731=CARTESIAN_POINT('Ctrl Pts',(-11.421919545259,15.8716860968864,3.15346399102705));
#86732=CARTESIAN_POINT('Ctrl Pts',(-11.4258036988268,15.8726111054585,3.16991348426326));
#86733=CARTESIAN_POINT('Ctrl Pts',(-11.4272350504583,15.8729604205542,3.17615835964278));
#86734=CARTESIAN_POINT('Ctrl Pts',(-11.4297139884825,15.8735809263,3.18730953459525));
#86735=CARTESIAN_POINT('Ctrl Pts',(-11.4307774355492,15.8738526173816,3.19221217241253));
#86736=CARTESIAN_POINT('Ctrl Pts',(-11.4329514603583,15.8744198620266,3.20248952673352));
#86737=CARTESIAN_POINT('Ctrl Pts',(-11.4340570573443,15.8747152539228,3.20786522484543));
#86738=CARTESIAN_POINT('Ctrl Pts',(-11.4362376801581,15.8753123374117,3.21877873985698));
#86739=CARTESIAN_POINT('Ctrl Pts',(-11.4373109791141,15.8756139702687,3.22431680938647));
#86740=CARTESIAN_POINT('Ctrl Pts',(-11.4398810488931,15.8763560180534,3.23800111863998));
#86741=CARTESIAN_POINT('Ctrl Pts',(-11.4413407475178,15.8767952712872,3.24615417657465));
#86742=CARTESIAN_POINT('Ctrl Pts',(-11.4565520095823,15.8815777959073,3.3354805338014));
#86743=CARTESIAN_POINT('Ctrl Pts',(-11.4634999999975,15.8856953222076,3.417663599478));
#86744=CARTESIAN_POINT('Ctrl Pts',(-11.4635,15.8897282898296,3.49999999995642));
#86745=CARTESIAN_POINT('Origin',(-10.,13.2,3.5));
#86746=CARTESIAN_POINT('',(-11.4635,16.4620214545711,3.5));
#86747=CARTESIAN_POINT('',(-11.4635,16.3880240412435,3.49999999999906));
#86748=CARTESIAN_POINT('',(-11.4635,13.2,3.5));
#86749=CARTESIAN_POINT('',(-11.463499289286,15.9600992933965,3.50126593704094));
#86750=CARTESIAN_POINT('Ctrl Pts',(-11.4635,16.4620214545711,3.5));
#86751=CARTESIAN_POINT('Ctrl Pts',(-11.4635,16.4620179317433,3.49993469539802));
#86752=CARTESIAN_POINT('Ctrl Pts',(-11.4634999956977,16.462014408645,3.49986939079802));
#86753=CARTESIAN_POINT('Ctrl Pts',(-11.4634994890769,16.4618102356802,3.49608502007503));
#86754=CARTESIAN_POINT('Ctrl Pts',(-11.4634848147942,16.4616088403519,3.49236602360626));
#86755=CARTESIAN_POINT('Ctrl Pts',(-11.4634353993144,16.4612625415967,3.48599603852318));
#86756=CARTESIAN_POINT('Ctrl Pts',(-11.463407629272,16.4611180209993,3.48334499291789));
#86757=CARTESIAN_POINT('Ctrl Pts',(-11.4633350012376,16.4608170560929,3.47783985432014));
#86758=CARTESIAN_POINT('Ctrl Pts',(-11.4632889967301,16.4606605463131,3.47498581479545));
#86759=CARTESIAN_POINT('Ctrl Pts',(-11.463158122383,16.4602825890147,3.46811414699329));
#86760=CARTESIAN_POINT('Ctrl Pts',(-11.4630650538143,16.4600606924473,3.46409670993799));
#86761=CARTESIAN_POINT('Ctrl Pts',(-11.4626854793201,16.4592892876604,3.45018645982909));
#86762=CARTESIAN_POINT('Ctrl Pts',(-11.4623151756252,16.4587354065625,3.44029642890958));
#86763=CARTESIAN_POINT('Ctrl Pts',(-11.4595398677968,16.4554413791121,3.38199583243003));
#86764=CARTESIAN_POINT('Ctrl Pts',(-11.4548314994578,16.4525972279559,3.33372884426687));
#86765=CARTESIAN_POINT('Ctrl Pts',(-11.4384257364983,16.4459184976122,3.22285099501531));
#86766=CARTESIAN_POINT('Ctrl Pts',(-11.4250190844743,16.4420613096008,3.16058757473446));
#86767=CARTESIAN_POINT('Ctrl Pts',(-11.4009291195383,16.4367900833161,3.07594297823236));
#86768=CARTESIAN_POINT('Ctrl Pts',(-11.3936697060786,16.4353367821147,3.05266169272317));
#86769=CARTESIAN_POINT('Ctrl Pts',(-11.3635631087754,16.4297985780481,2.96397077459831));
#86770=CARTESIAN_POINT('Ctrl Pts',(-11.336662434992,16.4258075901989,2.90002719525077));
#86771=CARTESIAN_POINT('Ctrl Pts',(-11.3006048313447,16.4213907872111,2.82890502969825));
#86772=CARTESIAN_POINT('Ctrl Pts',(-11.2957811785397,16.4208155954075,2.81963794066478));
#86773=CARTESIAN_POINT('Ctrl Pts',(-11.287847105386,16.4198940916472,2.80478569275871));
#86774=CARTESIAN_POINT('Ctrl Pts',(-11.2847986595119,16.4195456234819,2.79916799004742));
#86775=CARTESIAN_POINT('Ctrl Pts',(-11.2792936892484,16.4189261587787,2.78918002476904));
#86776=CARTESIAN_POINT('Ctrl Pts',(-11.2768513401937,16.418654666886,2.78480209979895));
#86777=CARTESIAN_POINT('Ctrl Pts',(-11.2716858400344,16.4180873727025,2.77565371153268));
#86778=CARTESIAN_POINT('Ctrl Pts',(-11.2689582253679,16.4177917348561,2.77088584929266));
#86779=CARTESIAN_POINT('Ctrl Pts',(-11.2617321592159,16.4170186387257,2.75841808933737));
#86780=CARTESIAN_POINT('Ctrl Pts',(-11.257190023555,16.4165427527707,2.75074368789045));
#86781=CARTESIAN_POINT('Ctrl Pts',(-11.2362697761007,16.4143952990966,2.71612269784851));
#86782=CARTESIAN_POINT('Ctrl Pts',(-11.2190929269557,16.4127528550993,2.68966722315921));
#86783=CARTESIAN_POINT('Ctrl Pts',(-11.1694580243537,16.4083019652555,2.6183754425417));
#86784=CARTESIAN_POINT('Ctrl Pts',(-11.1352908501064,16.4055541438616,2.57479232064836));
#86785=CARTESIAN_POINT('Ctrl Pts',(-11.0447416938529,16.3988386025747,2.47188127322583));
#86786=CARTESIAN_POINT('Ctrl Pts',(-10.9857041528785,16.3949302280811,2.41514994773822));
#86787=CARTESIAN_POINT('Ctrl Pts',(-10.9142041731137,16.3903380178101,2.35712198631516));
#86788=CARTESIAN_POINT('Ctrl Pts',(-10.9060969531774,16.3898190609612,2.3506837991595));
#86789=CARTESIAN_POINT('Ctrl Pts',(-10.8690422571964,16.3874517000272,2.32189331356306));
#86790=CARTESIAN_POINT('Ctrl Pts',(-10.8393335014563,16.3855662582615,2.30054651405468));
#86791=CARTESIAN_POINT('Ctrl Pts',(-10.8039038317721,16.3832937003946,2.27705019215995));
#86792=CARTESIAN_POINT('Ctrl Pts',(-10.7989287268348,16.382974047527,2.27379427081977));
#86793=CARTESIAN_POINT('Ctrl Pts',(-10.7909148008438,16.3824580617593,2.26861909028466));
#86794=CARTESIAN_POINT('Ctrl Pts',(-10.7878884581149,16.3822629606058,2.26668051827097));
#86795=CARTESIAN_POINT('Ctrl Pts',(-10.7824930416615,16.3819146366548,2.26325236159538));
#86796=CARTESIAN_POINT('Ctrl Pts',(-10.7801268017806,16.3817617040863,2.26175840225348));
#86797=CARTESIAN_POINT('Ctrl Pts',(-10.7750600384494,16.381433852987,2.25857971761627));
#86798=CARTESIAN_POINT('Ctrl Pts',(-10.7723583421704,16.3812588114774,2.25689703902055));
#86799=CARTESIAN_POINT('Ctrl Pts',(-10.7649399320901,16.3807776087937,2.2523102020271));
#86800=CARTESIAN_POINT('Ctrl Pts',(-10.7602122360716,16.3804703158602,2.24942401838785));
#86801=CARTESIAN_POINT('Ctrl Pts',(-10.7349140701712,16.3788231297274,2.23417635065422));
#86802=CARTESIAN_POINT('Ctrl Pts',(-10.7140593631872,16.3774553200107,2.22229608662211));
#86803=CARTESIAN_POINT('Ctrl Pts',(-10.6488993641576,16.3731733040815,2.1872700244556));
#86804=CARTESIAN_POINT('Ctrl Pts',(-10.6036945206132,16.3701920530025,2.16587755407076));
#86805=CARTESIAN_POINT('Ctrl Pts',(-10.4408851413988,16.3596124567826,2.09880183488542));
#86806=CARTESIAN_POINT('Ctrl Pts',(-10.318538352263,16.3519998236053,2.0660264360505));
#86807=CARTESIAN_POINT('Ctrl Pts',(-10.1738690257786,16.3438014829121,2.04672998035304));
#86808=CARTESIAN_POINT('Ctrl Pts',(-10.1541936720739,16.3427015642797,2.04451088852681));
#86809=CARTESIAN_POINT('Ctrl Pts',(-10.1267614028325,16.3411883230858,2.04197947212793));
#86810=CARTESIAN_POINT('Ctrl Pts',(-10.1190385259674,16.3407645344016,2.04132863690242));
#86811=CARTESIAN_POINT('Ctrl Pts',(-10.1066085881601,16.3400859506714,2.04038049554464));
#86812=CARTESIAN_POINT('Ctrl Pts',(-10.1019046949798,16.3398299579214,2.04004454769256));
#86813=CARTESIAN_POINT('Ctrl Pts',(-10.0921496980776,16.3393007188954,2.03939523011893));
#86814=CARTESIAN_POINT('Ctrl Pts',(-10.0870984223888,16.3390275833443,2.03908531174441));
#86815=CARTESIAN_POINT('Ctrl Pts',(-10.0752401007136,16.3383884698882,2.03841947261312));
#86816=CARTESIAN_POINT('Ctrl Pts',(-10.0684319420465,16.3380231593388,2.03808489225956));
#86817=CARTESIAN_POINT('Ctrl Pts',(-10.0461702080909,16.336833773342,2.03714671553428));
#86818=CARTESIAN_POINT('Ctrl Pts',(-10.0307090852649,16.336015812855,2.03674048914706));
#86819=CARTESIAN_POINT('Ctrl Pts',(-9.94954887933745,16.3317606611936,2.03589506695001));
#86820=CARTESIAN_POINT('Ctrl Pts',(-9.88387891043051,16.3284548725228,2.03963506899745));
#86821=CARTESIAN_POINT('Ctrl Pts',(-9.73520018917126,16.321071487501,2.05819894108525));
#86822=CARTESIAN_POINT('Ctrl Pts',(-9.652780758381,16.3170541075319,2.07579939509915));
#86823=CARTESIAN_POINT('Ctrl Pts',(-9.56459615244761,16.3124896895882,2.10274513186083));
#86824=CARTESIAN_POINT('Ctrl Pts',(-9.55688032600002,16.312087933008,2.10517290351569));
#86825=CARTESIAN_POINT('Ctrl Pts',(-9.53938282946858,16.3111706480171,2.11083829965606));
#86826=CARTESIAN_POINT('Ctrl Pts',(-9.52961449251298,16.3106541154168,2.11411548977361));
#86827=CARTESIAN_POINT('Ctrl Pts',(-9.48537506647408,16.3082913394211,2.12947902541361));
#86828=CARTESIAN_POINT('Ctrl Pts',(-9.45133178171022,16.306408091368,2.14274934747207));
#86829=CARTESIAN_POINT('Ctrl Pts',(-9.41236987114795,16.3041379917954,2.15964243110291));
#86830=CARTESIAN_POINT('Ctrl Pts',(-9.40693098154697,16.3038184386072,2.16204009111253));
#86831=CARTESIAN_POINT('Ctrl Pts',(-9.39822769070095,16.3033025830735,2.16594031213614));
#86832=CARTESIAN_POINT('Ctrl Pts',(-9.39495389919815,16.3031075114832,2.16742190534092));
#86833=CARTESIAN_POINT('Ctrl Pts',(-9.38914043862299,16.3027592205662,2.17007869508921));
#86834=CARTESIAN_POINT('Ctrl Pts',(-9.38659864629389,16.3026062912644,2.17124913540923));
#86835=CARTESIAN_POINT('Ctrl Pts',(-9.38117261180963,16.3022784242984,2.17376659425047));
#86836=CARTESIAN_POINT('Ctrl Pts',(-9.37828944818641,16.3021033635097,2.17511571363189));
#86837=CARTESIAN_POINT('Ctrl Pts',(-9.37040000459547,16.3016220547435,2.17883884604856));
#86838=CARTESIAN_POINT('Ctrl Pts',(-9.36540282217486,16.3013146741941,2.18123187451134));
#86839=CARTESIAN_POINT('Ctrl Pts',(-9.33881394923839,16.2996661800116,2.1941507544183));
#86840=CARTESIAN_POINT('Ctrl Pts',(-9.31747143916905,16.2982970985201,2.20517805399805));
#86841=CARTESIAN_POINT('Ctrl Pts',(-9.25252076616979,16.294009446776,2.24078893600373));
#86842=CARTESIAN_POINT('Ctrl Pts',(-9.20989621405615,16.2910236468348,2.26708754727458));
#86843=CARTESIAN_POINT('Ctrl Pts',(-9.06462463035638,16.2804181739965,2.36734913690631));
#86844=CARTESIAN_POINT('Ctrl Pts',(-8.97027201716319,16.2727852334712,2.45238540821475));
#86845=CARTESIAN_POINT('Ctrl Pts',(-8.87537049755298,16.2645899009743,2.56329325711897));
#86846=CARTESIAN_POINT('Ctrl Pts',(-8.86301278039784,16.2635089363818,2.57833240606659));
#86847=CARTESIAN_POINT('Ctrl Pts',(-8.84619017626691,16.2620171027929,2.59965872419743));
#86848=CARTESIAN_POINT('Ctrl Pts',(-8.84146977695941,16.2615961564136,2.60574095043141));
#86849=CARTESIAN_POINT('Ctrl Pts',(-8.83394151563374,16.2609209312797,2.61560076352859));
#86850=CARTESIAN_POINT('Ctrl Pts',(-8.83110353972844,16.2606654770197,2.61935508613345));
#86851=CARTESIAN_POINT('Ctrl Pts',(-8.82524773647433,16.2601364499133,2.62717983307557));
#86852=CARTESIAN_POINT('Ctrl Pts',(-8.82223283630973,16.2598629926943,2.63125237642151));
#86853=CARTESIAN_POINT('Ctrl Pts',(-8.81518970577999,16.2592215558686,2.64087032810612));
#86854=CARTESIAN_POINT('Ctrl Pts',(-8.81117914081665,16.2588542579799,2.64642856575206));
#86855=CARTESIAN_POINT('Ctrl Pts',(-8.79812279846009,16.2576515654163,2.66479386861437));
#86856=CARTESIAN_POINT('Ctrl Pts',(-8.78924360533658,16.2568224806806,2.6777183771426));
#86857=CARTESIAN_POINT('Ctrl Pts',(-8.71392253688211,16.2496834800432,2.79122136553634));
#86858=CARTESIAN_POINT('Ctrl Pts',(-8.65993569976571,16.2438796416924,2.89950628501159));
#86859=CARTESIAN_POINT('Ctrl Pts',(-8.59428367651107,16.2342658107381,3.08563890367132));
#86860=CARTESIAN_POINT('Ctrl Pts',(-8.57447743871951,16.2304963190294,3.15997599735643));
#86861=CARTESIAN_POINT('Ctrl Pts',(-8.55855094319861,16.2258479950539,3.2466521879023));
#86862=CARTESIAN_POINT('Ctrl Pts',(-8.55663375107693,16.2252446330111,3.25781339201078));
#86863=CARTESIAN_POINT('Ctrl Pts',(-8.55415604709014,16.22439868045,3.27331378734267));
#86864=CARTESIAN_POINT('Ctrl Pts',(-8.5534851274375,16.22416197217,3.27763521493868));
#86865=CARTESIAN_POINT('Ctrl Pts',(-8.55244111713695,16.2237809484068,3.28456446353685));
#86866=CARTESIAN_POINT('Ctrl Pts',(-8.55205567625175,16.2236373191879,3.28717043244637));
#86867=CARTESIAN_POINT('Ctrl Pts',(-8.55126531727836,16.2233364856879,3.29261558865705));
#86868=CARTESIAN_POINT('Ctrl Pts',(-8.55086170798363,16.2231792064975,3.29545493129895));
#86869=CARTESIAN_POINT('Ctrl Pts',(-8.54990271148155,16.2227964839828,3.30234668109798));
#86870=CARTESIAN_POINT('Ctrl Pts',(-8.54935596451256,16.222570563643,3.30640025279708));
#86871=CARTESIAN_POINT('Ctrl Pts',(-8.54748639373319,16.2217700767385,3.32071393335293));
#86872=CARTESIAN_POINT('Ctrl Pts',(-8.54625540448858,16.2211906941084,3.33098547792107));
#86873=CARTESIAN_POINT('Ctrl Pts',(-8.53444038804317,16.2150364135262,3.43927725404014));
#86874=CARTESIAN_POINT('Ctrl Pts',(-8.53367898396677,16.2090418751038,3.53810789670551));
#86875=CARTESIAN_POINT('Ctrl Pts',(-8.55195412443037,16.1972392174759,3.73354512733723));
#86876=CARTESIAN_POINT('Ctrl Pts',(-8.57077330088434,16.1914637974433,3.82969179931078));
#86877=CARTESIAN_POINT('Ctrl Pts',(-8.60400844990076,16.1850342483103,3.9396986070818));
#86878=CARTESIAN_POINT('Ctrl Pts',(-8.60926517271683,16.1840824675942,3.9560525721009));
#86879=CARTESIAN_POINT('Ctrl Pts',(-8.61717022482973,16.1827385453827,3.9792364820915));
#86880=CARTESIAN_POINT('Ctrl Pts',(-8.61958365138434,16.1823387822354,3.98614452590325));
#86881=CARTESIAN_POINT('Ctrl Pts',(-8.62376711032751,16.1816632591698,3.99783661826078));
#86882=CARTESIAN_POINT('Ctrl Pts',(-8.62551051126551,16.1813866292381,4.00262999450132));
#86883=CARTESIAN_POINT('Ctrl Pts',(-8.62908353459874,16.1808293832529,4.01229618895413));
#86884=CARTESIAN_POINT('Ctrl Pts',(-8.63091416475779,16.1805488053774,4.01716855765677));
#86885=CARTESIAN_POINT('Ctrl Pts',(-8.63547517187958,16.1798616262582,4.02911409551682));
#86886=CARTESIAN_POINT('Ctrl Pts',(-8.63823461172387,16.1794559955694,4.03617605584134));
#86887=CARTESIAN_POINT('Ctrl Pts',(-8.64856174983524,16.1779740561627,4.06201120683181));
#86888=CARTESIAN_POINT('Ctrl Pts',(-8.6564639831058,16.1769089200978,4.08064874470118));
#86889=CARTESIAN_POINT('Ctrl Pts',(-8.70070815944155,16.17128535954,4.17925554893343));
#86890=CARTESIAN_POINT('Ctrl Pts',(-8.74380800449931,16.1669651217598,4.25599676670985));
#86891=CARTESIAN_POINT('Ctrl Pts',(-8.85254035705587,16.1576148606236,4.41434947636516));
#86892=CARTESIAN_POINT('Ctrl Pts',(-8.92055116027678,16.1526286195492,4.49372185123336));
#86893=CARTESIAN_POINT('Ctrl Pts',(-9.00407727240567,16.1465638859934,4.57241846764813));
#86894=CARTESIAN_POINT('Ctrl Pts',(-9.0118300820101,16.146001302206,4.57956641738272));
#86895=CARTESIAN_POINT('Ctrl Pts',(-9.02281070751389,16.1452038363584,4.5894729699752));
#86896=CARTESIAN_POINT('Ctrl Pts',(-9.02597449697489,16.1449739917627,4.59230242341602));
#86897=CARTESIAN_POINT('Ctrl Pts',(-9.03110355979625,16.1446011676901,4.59684946569989));
#86898=CARTESIAN_POINT('Ctrl Pts',(-9.03306122219504,16.1444588201883,4.59857565146943));
#86899=CARTESIAN_POINT('Ctrl Pts',(-9.03719735531448,16.1441579431562,4.60220310196241));
#86900=CARTESIAN_POINT('Ctrl Pts',(-9.03937685220175,16.1439993238997,4.60410315554556));
#86901=CARTESIAN_POINT('Ctrl Pts',(-9.04474327557044,16.1436086145669,4.60875360734033));
#86902=CARTESIAN_POINT('Ctrl Pts',(-9.04793645205105,16.1433760004452,4.61149672564652));
#86903=CARTESIAN_POINT('Ctrl Pts',(-9.05961028796306,16.1425252642291,4.62143799421912));
#86904=CARTESIAN_POINT('Ctrl Pts',(-9.06816088831363,16.1419015074982,4.62855298501033));
#86905=CARTESIAN_POINT('Ctrl Pts',(-9.12425789433248,16.1378099588156,4.67415937827377));
#86906=CARTESIAN_POINT('Ctrl Pts',(-9.17409310297747,16.1341804694032,4.70973175487258));
#86907=CARTESIAN_POINT('Ctrl Pts',(-9.26068684141239,16.1280586795754,4.76369240136407));
#86908=CARTESIAN_POINT('Ctrl Pts',(-9.29626162910709,16.1255907035297,4.7838437376221));
#86909=CARTESIAN_POINT('Ctrl Pts',(-9.42323571391089,16.1170215991625,4.84890294263922));
#86910=CARTESIAN_POINT('Ctrl Pts',(-9.51844802721915,16.1110380274387,4.88575263745446));
#86911=CARTESIAN_POINT('Ctrl Pts',(-9.62696029245809,16.1048081742526,4.91519822330876));
#86912=CARTESIAN_POINT('Ctrl Pts',(-9.63722150704141,16.1042243462223,4.91786332487408));
#86913=CARTESIAN_POINT('Ctrl Pts',(-9.65375835184062,16.1032917663985,4.92196708978953));
#86914=CARTESIAN_POINT('Ctrl Pts',(-9.66001596368178,16.1029407743462,4.92347621696547));
#86915=CARTESIAN_POINT('Ctrl Pts',(-9.67117058804314,16.1023184303823,4.9260885885756));
#86916=CARTESIAN_POINT('Ctrl Pts',(-9.6760636741292,16.1020465666363,4.9272080094669));
#86917=CARTESIAN_POINT('Ctrl Pts',(-9.68630107322397,16.1014801002587,4.92949472054757));
#86918=CARTESIAN_POINT('Ctrl Pts',(-9.69164637370049,16.1011856521189,4.93065726678272));
#86919=CARTESIAN_POINT('Ctrl Pts',(-9.70562188698924,16.1004191938273,4.93361482854274));
#86920=CARTESIAN_POINT('Ctrl Pts',(-9.71426209194547,16.0999487060933,4.93536190646082));
#86921=CARTESIAN_POINT('Ctrl Pts',(-9.75285162354715,16.0978618339913,4.94280257960455));
#86922=CARTESIAN_POINT('Ctrl Pts',(-9.78295981495007,16.0962725482274,4.94763784628891));
#86923=CARTESIAN_POINT('Ctrl Pts',(-9.86538591947739,16.0920088076565,4.9582454956842));
#86924=CARTESIAN_POINT('Ctrl Pts',(-9.91789988718294,16.0893884868907,4.96214261278699));
#86925=CARTESIAN_POINT('Ctrl Pts',(-10.076072460101,16.0816219120699,4.96533023130551));
#86926=CARTESIAN_POINT('Ctrl Pts',(-10.1815426907608,16.0766267479744,4.95602825698673));
#86927=CARTESIAN_POINT('Ctrl Pts',(-10.3124864034093,16.0698070056283,4.93002271748299));
#86928=CARTESIAN_POINT('Ctrl Pts',(-10.3397250450732,16.0683521183909,4.923797534166));
#86929=CARTESIAN_POINT('Ctrl Pts',(-10.3720893578367,16.0665621395121,4.915419367255));
#86930=CARTESIAN_POINT('Ctrl Pts',(-10.3774037891972,16.0662662131697,4.91401161713932));
#86931=CARTESIAN_POINT('Ctrl Pts',(-10.3860858884793,16.0657792996803,4.91165936731473));
#86932=CARTESIAN_POINT('Ctrl Pts',(-10.3894583734814,16.065589304357,4.91073266688461));
#86933=CARTESIAN_POINT('Ctrl Pts',(-10.3955099143621,16.0652467839791,4.90904645481509));
#86934=CARTESIAN_POINT('Ctrl Pts',(-10.3981901530613,16.065094514761,4.90829137823229));
#86935=CARTESIAN_POINT('Ctrl Pts',(-10.4040338899206,16.0647612744982,4.90662706496039));
#86936=CARTESIAN_POINT('Ctrl Pts',(-10.4071964406046,16.0645801355038,4.90571481545962));
#86937=CARTESIAN_POINT('Ctrl Pts',(-10.4161511030771,16.0640650481834,4.90309905569145));
#86938=CARTESIAN_POINT('Ctrl Pts',(-10.4219357183245,16.0637296956144,4.90137038204972));
#86939=CARTESIAN_POINT('Ctrl Pts',(-10.4586558640148,16.0615850171189,4.89014897378434));
#86940=CARTESIAN_POINT('Ctrl Pts',(-10.4892779789864,16.0597247022061,4.87966884348865));
#86941=CARTESIAN_POINT('Ctrl Pts',(-10.599490720058,16.0528272637606,4.8378189761102));
#86942=CARTESIAN_POINT('Ctrl Pts',(-10.6766381064648,16.0476175432362,4.80050341449727));
#86943=CARTESIAN_POINT('Ctrl Pts',(-10.8302563364765,16.0369015018342,4.70881113823773));
#86944=CARTESIAN_POINT('Ctrl Pts',(-10.9056763196231,16.0314418058153,4.65338866581849));
#86945=CARTESIAN_POINT('Ctrl Pts',(-10.9832768662898,16.0256738580968,4.58402631076947));
#86946=CARTESIAN_POINT('Ctrl Pts',(-10.9911658962252,16.0250852875304,4.57681781787796));
#86947=CARTESIAN_POINT('Ctrl Pts',(-11.0036976570844,16.0241466315328,4.56511267827738));
#86948=CARTESIAN_POINT('Ctrl Pts',(-11.0083906843494,16.0237942590809,4.56067065286819));
#86949=CARTESIAN_POINT('Ctrl Pts',(-11.0166792810886,16.0231703342717,4.55272062784796));
#86950=CARTESIAN_POINT('Ctrl Pts',(-11.0202864768818,16.0228982610496,4.54922494578488));
#86951=CARTESIAN_POINT('Ctrl Pts',(-11.0272037998889,16.0223754407541,4.54245206081779));
#86952=CARTESIAN_POINT('Ctrl Pts',(-11.0305164143292,16.0221245846215,4.53917749499192));
#86953=CARTESIAN_POINT('Ctrl Pts',(-11.0391298748392,16.0214709981277,4.53058127806441));
#86954=CARTESIAN_POINT('Ctrl Pts',(-11.0444055232095,16.0210693738379,4.52523449679433));
#86955=CARTESIAN_POINT('Ctrl Pts',(-11.064393955728,16.0195423835162,4.50466214659077));
#86956=CARTESIAN_POINT('Ctrl Pts',(-11.0788172630665,16.0184294428988,4.48915817483372));
#86957=CARTESIAN_POINT('Ctrl Pts',(-11.1140872974781,16.0156743811656,4.44955601892534));
#86958=CARTESIAN_POINT('Ctrl Pts',(-11.1344933423461,16.0140495041917,4.42507954587033));
#86959=CARTESIAN_POINT('Ctrl Pts',(-11.1889601940384,16.0095962030362,4.35523232626712));
#86960=CARTESIAN_POINT('Ctrl Pts',(-11.2212072728127,16.006823249415,4.30851834683157));
#86961=CARTESIAN_POINT('Ctrl Pts',(-11.3035648260366,15.9991071228051,4.17299882279297));
#86962=CARTESIAN_POINT('Ctrl Pts',(-11.3472271175272,15.9942241944666,4.08067411036933));
#86963=CARTESIAN_POINT('Ctrl Pts',(-11.3844896104899,15.9882791648054,3.97448419050778));
#86964=CARTESIAN_POINT('Ctrl Pts',(-11.3879213916615,15.9877084989882,3.96435000365024));
#86965=CARTESIAN_POINT('Ctrl Pts',(-11.3925669130381,15.9869014074386,3.95011984956479));
#86966=CARTESIAN_POINT('Ctrl Pts',(-11.3938743862061,15.986670181498,3.9460545715614));
#86967=CARTESIAN_POINT('Ctrl Pts',(-11.3959537263924,15.9862957116515,3.93949093412466));
#86968=CARTESIAN_POINT('Ctrl Pts',(-11.3967367325264,15.9861531105323,3.93699609517209));
#86969=CARTESIAN_POINT('Ctrl Pts',(-11.3983699690903,15.9858522682238,3.93174299126924));
#86970=CARTESIAN_POINT('Ctrl Pts',(-11.3992187290161,15.9856939403813,3.92898429913406));
#86971=CARTESIAN_POINT('Ctrl Pts',(-11.401277903736,15.985304940307,3.92222031469942));
#86972=CARTESIAN_POINT('Ctrl Pts',(-11.4024793078821,15.9850737541201,3.91821232373061));
#86973=CARTESIAN_POINT('Ctrl Pts',(-11.4067636723387,15.9842339406782,3.90369321139507));
#86974=CARTESIAN_POINT('Ctrl Pts',(-11.4097457076662,15.9836198624403,3.89315297758475));
#86975=CARTESIAN_POINT('Ctrl Pts',(-11.4281109509877,15.9796454487502,3.82534266659133));
#86976=CARTESIAN_POINT('Ctrl Pts',(-11.4401183079515,15.9761326038071,3.76722035944168));
#86977=CARTESIAN_POINT('Ctrl Pts',(-11.4584491247974,15.9684199590326,3.63988794984887));
#86978=CARTESIAN_POINT('Ctrl Pts',(-11.4634394420433,15.9642166244403,3.57062294632637));
#86979=CARTESIAN_POINT('Ctrl Pts',(-11.4634994521832,15.9600990306171,3.50126627775981));
#86980=CARTESIAN_POINT('Ctrl Pts',(-11.4634994524634,15.9600990113915,3.50126595392359));
#86981=CARTESIAN_POINT('Ctrl Pts',(-11.4634998174897,15.9600739587178,3.50084396715964));
#86982=CARTESIAN_POINT('Ctrl Pts',(-11.4635,15.9600489093257,3.5004219824875));
#86983=CARTESIAN_POINT('Ctrl Pts',(-11.4635,15.960023863236,3.50000000002449));
#86984=CARTESIAN_POINT('',(-11.4634993427279,15.8897888773263,3.50124168730561));
#86985=CARTESIAN_POINT('Ctrl Pts',(-11.4635,15.8897282898296,3.49999999995642));
#86986=CARTESIAN_POINT('Ctrl Pts',(-11.4635,15.8897485812173,3.50041426557451));
#86987=CARTESIAN_POINT('Ctrl Pts',(-11.4634998241039,15.8897688707616,3.50082853505967));
#86988=CARTESIAN_POINT('Ctrl Pts',(-11.4634994723018,15.8897891584897,3.50124280830086));
#86989=CARTESIAN_POINT('Ctrl Pts',(-11.4634994732626,15.8897891030564,3.50124167636007));
#86990=CARTESIAN_POINT('Ctrl Pts',(-11.4634429208337,15.8930533426711,3.56789708876401));
#86991=CARTESIAN_POINT('Ctrl Pts',(-11.4588327255218,15.8962578075281,3.63447116018265));
#86992=CARTESIAN_POINT('Ctrl Pts',(-11.4421263112084,15.9022646502392,3.75526584806839));
#86993=CARTESIAN_POINT('Ctrl Pts',(-11.4314552758207,15.9050388591201,3.80955386092396));
#86994=CARTESIAN_POINT('Ctrl Pts',(-11.4151159284091,15.908520678393,3.87335115221185));
#86995=CARTESIAN_POINT('Ctrl Pts',(-11.4123801444055,15.9090853631532,3.88357070858721));
#86996=CARTESIAN_POINT('Ctrl Pts',(-11.4084232940843,15.9098788134638,3.89773497866231));
#86997=CARTESIAN_POINT('Ctrl Pts',(-11.4072959005409,15.910102435243,3.9017057829439));
#86998=CARTESIAN_POINT('Ctrl Pts',(-11.4053545701882,15.9104834914579,3.90843488173125));
#86999=CARTESIAN_POINT('Ctrl Pts',(-11.4045492639391,15.9106404310371,3.91119567798628));
#87000=CARTESIAN_POINT('Ctrl Pts',(-11.402992647264,15.9109416752255,3.9164742311754));
#87001=CARTESIAN_POINT('Ctrl Pts',(-11.4022426872647,15.9110858972966,3.91899236185908));
#87002=CARTESIAN_POINT('Ctrl Pts',(-11.4002377046772,15.9114690429023,3.92565878815586));
#87003=CARTESIAN_POINT('Ctrl Pts',(-11.3989710390601,15.911708630159,3.92980351839303));
#87004=CARTESIAN_POINT('Ctrl Pts',(-11.3944013296108,15.9125641772583,3.94452210165846));
#87005=CARTESIAN_POINT('Ctrl Pts',(-11.3909967447944,15.9131856421364,3.95506374031328));
#87006=CARTESIAN_POINT('Ctrl Pts',(-11.3579082451518,15.9190743963223,4.05367372978732));
#87007=CARTESIAN_POINT('Ctrl Pts',(-11.3200204464006,15.9247087990548,4.13875886812837));
#87008=CARTESIAN_POINT('Ctrl Pts',(-11.2519856905339,15.9330344154156,4.25922858108924));
#87009=CARTESIAN_POINT('Ctrl Pts',(-11.2278145792619,15.9357563648387,4.29772669859862));
#87010=CARTESIAN_POINT('Ctrl Pts',(-11.1766541726618,15.9410446506838,4.37136301478326));
#87011=CARTESIAN_POINT('Ctrl Pts',(-11.149782361342,15.9436105400264,4.40652611322557));
#87012=CARTESIAN_POINT('Ctrl Pts',(-11.1040452423892,15.9476462548384,4.46106304122844));
#87013=CARTESIAN_POINT('Ctrl Pts',(-11.0861659919513,15.94915186665,4.48122456128071));
#87014=CARTESIAN_POINT('Ctrl Pts',(-11.0621089130142,15.9510876569649,4.50688861821555));
#87015=CARTESIAN_POINT('Ctrl Pts',(-11.0564277192387,15.9515385664006,4.51284772325852));
#87016=CARTESIAN_POINT('Ctrl Pts',(-11.0468965809449,15.9522848527628,4.52267766009709));
#87017=CARTESIAN_POINT('Ctrl Pts',(-11.0430747713931,15.9525814304796,4.52657540885455));
#87018=CARTESIAN_POINT('Ctrl Pts',(-11.0356929578405,15.9531492101371,4.53402011572748));
#87019=CARTESIAN_POINT('Ctrl Pts',(-11.0321363232207,15.9534205525647,4.53757029342998));
#87020=CARTESIAN_POINT('Ctrl Pts',(-11.0239610096179,15.9540392530456,4.54564713070572));
#87021=CARTESIAN_POINT('Ctrl Pts',(-11.0193304528417,15.9543860799559,4.55016165465651));
#87022=CARTESIAN_POINT('Ctrl Pts',(-11.0069595389834,15.955303250955,4.56206366097577));
#87023=CARTESIAN_POINT('Ctrl Pts',(-10.9991677539915,15.9558712890916,4.56939727910808));
#87024=CARTESIAN_POINT('Ctrl Pts',(-10.9238562523922,15.9612725878394,4.63873861597449));
#87025=CARTESIAN_POINT('Ctrl Pts',(-10.8507291257415,15.9658227499381,4.69436122111318));
#87026=CARTESIAN_POINT('Ctrl Pts',(-10.6990431484781,15.9745374131878,4.78869283537293));
#87027=CARTESIAN_POINT('Ctrl Pts',(-10.6212775259882,15.9786973168724,4.82793175916797));
#87028=CARTESIAN_POINT('Ctrl Pts',(-10.5101876583657,15.9847657175092,4.87208035112681));
#87029=CARTESIAN_POINT('Ctrl Pts',(-10.479487147089,15.9864563812095,4.88310798698696));
#87030=CARTESIAN_POINT('Ctrl Pts',(-10.4426859771268,15.9885267196702,4.8949544779082));
#87031=CARTESIAN_POINT('Ctrl Pts',(-10.4369143003977,15.9888526770867,4.89677298131441));
#87032=CARTESIAN_POINT('Ctrl Pts',(-10.4279826321461,15.9893592694767,4.89952633951154));
#87033=CARTESIAN_POINT('Ctrl Pts',(-10.4248304133642,15.9895384756237,4.90048642544233));
#87034=CARTESIAN_POINT('Ctrl Pts',(-10.4190077020568,15.9898703143651,4.90223840849455));
#87035=CARTESIAN_POINT('Ctrl Pts',(-10.4163381758478,15.9900227699838,4.90303333232577));
#87036=CARTESIAN_POINT('Ctrl Pts',(-10.4103133162295,15.9903675610151,4.90480868871112));
#87037=CARTESIAN_POINT('Ctrl Pts',(-10.4069567497967,15.9905601445081,4.90578471773755));
#87038=CARTESIAN_POINT('Ctrl Pts',(-10.3983201012654,15.9910568822568,4.90826257559364));
#87039=CARTESIAN_POINT('Ctrl Pts',(-10.3930350559108,15.9913620107424,4.90974672469049));
#87040=CARTESIAN_POINT('Ctrl Pts',(-10.3609543643755,15.9932206444829,4.91856122147095));
#87041=CARTESIAN_POINT('Ctrl Pts',(-10.3339644315741,15.9948115944618,4.92515667422241));
#87042=CARTESIAN_POINT('Ctrl Pts',(-10.1925609974508,16.0032307835444,4.95547387081249));
#87043=CARTESIAN_POINT('Ctrl Pts',(-10.0757948519613,16.0104263324791,4.96619953579029));
#87044=CARTESIAN_POINT('Ctrl Pts',(-9.89725550988873,16.0209714852411,4.96119477694553));
#87045=CARTESIAN_POINT('Ctrl Pts',(-9.83568554052009,16.0245330917125,4.95555792456925));
#87046=CARTESIAN_POINT('Ctrl Pts',(-9.75985238290576,16.0288095707521,4.94374015888907));
#87047=CARTESIAN_POINT('Ctrl Pts',(-9.74509109358632,16.0296369765581,4.94120713197345));
#87048=CARTESIAN_POINT('Ctrl Pts',(-9.72375600627072,16.0308259034913,4.93720798772075));
#87049=CARTESIAN_POINT('Ctrl Pts',(-9.71714968285501,16.0311930803273,4.93592243671084));
#87050=CARTESIAN_POINT('Ctrl Pts',(-9.70560396383945,16.0318331462646,4.93359293649683));
#87051=CARTESIAN_POINT('Ctrl Pts',(-9.70066070046152,16.0321066605158,4.93256892271181));
#87052=CARTESIAN_POINT('Ctrl Pts',(-9.69108495880993,16.0326355004478,4.93053354683056));
#87053=CARTESIAN_POINT('Ctrl Pts',(-9.68645190787305,16.032890918161,4.92952520996757));
#87054=CARTESIAN_POINT('Ctrl Pts',(-9.67413273278485,16.0335689049781,4.92678129414028));
#87055=CARTESIAN_POINT('Ctrl Pts',(-9.66645552592589,16.0339902121404,4.92500611375972));
#87056=CARTESIAN_POINT('Ctrl Pts',(-9.63874984763337,16.0355065531902,4.91836363247497));
#87057=CARTESIAN_POINT('Ctrl Pts',(-9.61880991556881,16.0365900912884,4.91313525239739));
#87058=CARTESIAN_POINT('Ctrl Pts',(-9.47853700597395,16.044170491937,4.87316945828526));
#87059=CARTESIAN_POINT('Ctrl Pts',(-9.36299600318659,16.0501362356306,4.82353511653231));
#87060=CARTESIAN_POINT('Ctrl Pts',(-9.21229589674631,16.0587032543091,4.73443774680789));
#87061=CARTESIAN_POINT('Ctrl Pts',(-9.1707355869757,16.0611692351423,4.70691101069027));
#87062=CARTESIAN_POINT('Ctrl Pts',(-9.11139368996741,16.0649650667623,4.66309277921341));
#87063=CARTESIAN_POINT('Ctrl Pts',(-9.09247801072464,16.0662196627082,4.64839439856228));
#87064=CARTESIAN_POINT('Ctrl Pts',(-9.06964509611192,16.0678015447531,4.6297356601552));
#87065=CARTESIAN_POINT('Ctrl Pts',(-9.06537754536843,16.0681001923612,4.6262076959144));
#87066=CARTESIAN_POINT('Ctrl Pts',(-9.0586884197408,16.0685732155084,4.62061362252977));
#87067=CARTESIAN_POINT('Ctrl Pts',(-9.05625334531319,16.0687464479391,4.61856364749642));
#87068=CARTESIAN_POINT('Ctrl Pts',(-9.05168916595467,16.0690731391413,4.61469576563487));
#87069=CARTESIAN_POINT('Ctrl Pts',(-9.04955857913786,16.069226467191,4.61287968484958));
#87070=CARTESIAN_POINT('Ctrl Pts',(-9.04470262790791,16.0695778073536,4.60871642799783));
#87071=CARTESIAN_POINT('Ctrl Pts',(-9.04198069870504,16.0697761047855,4.60636531246047));
#87072=CARTESIAN_POINT('Ctrl Pts',(-9.03477672331327,16.0703044809455,4.60009623010691));
#87073=CARTESIAN_POINT('Ctrl Pts',(-9.03030991636911,16.0706357775209,4.59616095013628));
#87074=CARTESIAN_POINT('Ctrl Pts',(-8.99846952057362,16.0730230317316,4.56776247925283));
#87075=CARTESIAN_POINT('Ctrl Pts',(-8.97200299837268,16.0751442511612,4.54230597422903));
#87076=CARTESIAN_POINT('Ctrl Pts',(-8.93876085809529,16.0779610509686,4.50783371557471));
#87077=CARTESIAN_POINT('Ctrl Pts',(-8.93109070596816,16.078622282335,4.49969506732024));
#87078=CARTESIAN_POINT('Ctrl Pts',(-8.86877152234954,16.0840835199847,4.43203218125015));
#87079=CARTESIAN_POINT('Ctrl Pts',(-8.81904498565561,16.0890020786102,4.36816328068427));
#87080=CARTESIAN_POINT('Ctrl Pts',(-8.72983646451623,16.0987189168368,4.23163327763754));
#87081=CARTESIAN_POINT('Ctrl Pts',(-8.69071312446134,16.103494498167,4.15907061112101));
#87082=CARTESIAN_POINT('Ctrl Pts',(-8.6533300188433,16.1086855463525,4.07309960405249));
#87083=CARTESIAN_POINT('Ctrl Pts',(-8.64889005481879,16.1093150311084,4.06255232716928));
#87084=CARTESIAN_POINT('Ctrl Pts',(-8.64229560467415,16.1102705034516,4.04635842217766));
#87085=CARTESIAN_POINT('Ctrl Pts',(-8.6400516945561,16.1105994783246,4.04074888684293));
#87086=CARTESIAN_POINT('Ctrl Pts',(-8.63602461295747,16.1111970608495,4.03049798576373));
#87087=CARTESIAN_POINT('Ctrl Pts',(-8.63423024252627,16.1114660388623,4.02586114115142));
#87088=CARTESIAN_POINT('Ctrl Pts',(-8.6303971989463,16.1120465946868,4.01580417767325));
#87089=CARTESIAN_POINT('Ctrl Pts',(-8.628366990728,16.1123578880008,4.01038090829862));
#87090=CARTESIAN_POINT('Ctrl Pts',(-8.62292016424368,16.1132036482661,3.99556361207068));
#87091=CARTESIAN_POINT('Ctrl Pts',(-8.61956748048885,16.1137360031373,3.98614630860418));
#87092=CARTESIAN_POINT('Ctrl Pts',(-8.60311707408465,16.1164101251813,3.93839622275472));
#87093=CARTESIAN_POINT('Ctrl Pts',(-8.59151780351218,16.1185026402088,3.89956406303697));
#87094=CARTESIAN_POINT('Ctrl Pts',(-8.57816805651377,16.1212494549363,3.84700751100414));
#87095=CARTESIAN_POINT('Ctrl Pts',(-8.57497904628135,16.1219393904434,3.83366986919692));
#87096=CARTESIAN_POINT('Ctrl Pts',(-8.54326091589608,16.1291889042777,3.69225331118162));
#87097=CARTESIAN_POINT('Ctrl Pts',(-8.53189627573499,16.1352925243252,3.56095357763328));
#87098=CARTESIAN_POINT('Ctrl Pts',(-8.53957869214876,16.1434768631266,3.40072422397946));
#87099=CARTESIAN_POINT('Ctrl Pts',(-8.54185180459172,16.1449976201787,3.37158782018656));
#87100=CARTESIAN_POINT('Ctrl Pts',(-8.54562708361405,16.146877830445,3.33670223282864));
#87101=CARTESIAN_POINT('Ctrl Pts',(-8.54629407971528,16.1471943124988,3.33086740212575));
#87102=CARTESIAN_POINT('Ctrl Pts',(-8.54738549816016,16.1476892704291,3.32180357851776));
#87103=CARTESIAN_POINT('Ctrl Pts',(-8.54778561828998,16.1478664197631,3.3185716540454));
#87104=CARTESIAN_POINT('Ctrl Pts',(-8.54854840002927,16.1481964022131,3.31257460039337));
#87105=CARTESIAN_POINT('Ctrl Pts',(-8.54890817981985,16.1483490739492,3.30980915770685));
#87106=CARTESIAN_POINT('Ctrl Pts',(-8.54974339221648,16.1486968891717,3.30352965587547));
#87107=CARTESIAN_POINT('Ctrl Pts',(-8.5502236917122,16.1488923001878,3.30001630086117));
#87108=CARTESIAN_POINT('Ctrl Pts',(-8.55172689033268,16.1494901434328,3.28931059280308));
#87109=CARTESIAN_POINT('Ctrl Pts',(-8.55279056299814,16.1498947583583,3.28212419249358));
#87110=CARTESIAN_POINT('Ctrl Pts',(-8.56480342041571,16.154274078806,3.20493510227587));
#87111=CARTESIAN_POINT('Ctrl Pts',(-8.58076801131875,16.1584869612585,3.1358146181308));
#87112=CARTESIAN_POINT('Ctrl Pts',(-8.63048308582169,16.1686084351147,2.97484491496365));
#87113=CARTESIAN_POINT('Ctrl Pts',(-8.66856005668425,16.1745172112687,2.88466609873806));
#87114=CARTESIAN_POINT('Ctrl Pts',(-8.7364704133736,16.182714673906,2.76022201798481));
#87115=CARTESIAN_POINT('Ctrl Pts',(-8.75934465406478,16.1852118328955,2.72246969672117));
#87116=CARTESIAN_POINT('Ctrl Pts',(-8.7894107158728,16.1881952752186,2.67756200700994));
#87117=CARTESIAN_POINT('Ctrl Pts',(-8.79501361774546,16.1887398065995,2.66937463766826));
#87118=CARTESIAN_POINT('Ctrl Pts',(-8.80397486928208,16.1895931032315,2.65656132444671));
#87119=CARTESIAN_POINT('Ctrl Pts',(-8.80727774006488,16.1899039487145,2.65189710254192));
#87120=CARTESIAN_POINT('Ctrl Pts',(-8.81350797086442,16.1904835566353,2.64320732546038));
#87121=CARTESIAN_POINT('Ctrl Pts',(-8.81642870056186,16.1907525658682,2.63917713649062));
#87122=CARTESIAN_POINT('Ctrl Pts',(-8.82299677265504,16.1913515347051,2.63021076099476));
#87123=CARTESIAN_POINT('Ctrl Pts',(-8.82665473277363,16.191681079925,2.62528244391914));
#87124=CARTESIAN_POINT('Ctrl Pts',(-8.83598179746578,16.1925113194784,2.6128800129419));
#87125=CARTESIAN_POINT('Ctrl Pts',(-8.84169200687672,16.1930104134511,2.60543706436782));
#87126=CARTESIAN_POINT('Ctrl Pts',(-8.87498455462523,16.1958688863119,2.56289532761114));
#87127=CARTESIAN_POINT('Ctrl Pts',(-8.90409099571932,16.1981672116393,2.52901654402643));
#87128=CARTESIAN_POINT('Ctrl Pts',(-9.03041662352791,16.2074580622841,2.39490902338277));
#87129=CARTESIAN_POINT('Ctrl Pts',(-9.14016098901583,16.2139194369629,2.3075287537668));
#87130=CARTESIAN_POINT('Ctrl Pts',(-9.28637719863801,16.2225553276027,2.22192854637982));
#87131=CARTESIAN_POINT('Ctrl Pts',(-9.31260406773908,16.2241084332452,2.20763366922292));
#87132=CARTESIAN_POINT('Ctrl Pts',(-9.34452021458465,16.226024847343,2.19148427036018));
#87133=CARTESIAN_POINT('Ctrl Pts',(-9.34980851256189,16.2263432356556,2.18884852473925));
#87134=CARTESIAN_POINT('Ctrl Pts',(-9.35804293527525,16.2268405354254,2.18480646540317));
#87135=CARTESIAN_POINT('Ctrl Pts',(-9.36097811017378,16.2270181000329,2.18337783313053));
#87136=CARTESIAN_POINT('Ctrl Pts',(-9.36642892284749,16.2273484509214,2.18074728985268));
#87137=CARTESIAN_POINT('Ctrl Pts',(-9.36894322876594,16.2275010726497,2.17954274051282));
#87138=CARTESIAN_POINT('Ctrl Pts',(-9.37465377131094,16.2278482485287,2.17682697887323));
#87139=CARTESIAN_POINT('Ctrl Pts',(-9.37785203684649,16.2280430661356,2.17532016661546));
#87140=CARTESIAN_POINT('Ctrl Pts',(-9.3875904262919,16.2286373380291,2.17077512500257));
#87141=CARTESIAN_POINT('Ctrl Pts',(-9.39414747397611,16.2290389379656,2.16777368039821));
#87142=CARTESIAN_POINT('Ctrl Pts',(-9.45478043447993,16.2327641506433,2.14055954988788));
#87143=CARTESIAN_POINT('Ctrl Pts',(-9.51025285169229,16.2362552698517,2.11960548517195));
#87144=CARTESIAN_POINT('Ctrl Pts',(-9.68009853672908,16.2468902324134,2.06697681170343));
#87145=CARTESIAN_POINT('Ctrl Pts',(-9.79722675141693,16.2541114709821,2.04577079682824));
#87146=CARTESIAN_POINT('Ctrl Pts',(-9.93935188967328,16.2622715656758,2.03756421962031));
#87147=CARTESIAN_POINT('Ctrl Pts',(-9.96309924542753,16.2636171255825,2.03677239305236));
#87148=CARTESIAN_POINT('Ctrl Pts',(-10.0038847294892,16.2658973367962,2.03640608498709));
#87149=CARTESIAN_POINT('Ctrl Pts',(-10.0209149585324,16.266840275943,2.03655036365255));
#87150=CARTESIAN_POINT('Ctrl Pts',(-10.0450222965302,16.2681625326108,2.03717552482123));
#87151=CARTESIAN_POINT('Ctrl Pts',(-10.0521039358916,16.2685494224825,2.03741064043745));
#87152=CARTESIAN_POINT('Ctrl Pts',(-10.0642886801084,16.2692125428466,2.03790379271605));
#87153=CARTESIAN_POINT('Ctrl Pts',(-10.0693926102124,16.269489534483,2.03813714038811));
#87154=CARTESIAN_POINT('Ctrl Pts',(-10.0791458761303,16.2700173969798,2.03863424676978));
#87155=CARTESIAN_POINT('Ctrl Pts',(-10.0837953716329,16.270268404979,2.03889347725565));
#87156=CARTESIAN_POINT('Ctrl Pts',(-10.0958524630101,16.2709177226534,2.03962345678638));
#87157=CARTESIAN_POINT('Ctrl Pts',(-10.1032579083141,16.271314967056,2.04012837901467));
#87158=CARTESIAN_POINT('Ctrl Pts',(-10.1284145960952,16.2726593326,2.04203600686002));
#87159=CARTESIAN_POINT('Ctrl Pts',(-10.1461443284622,16.2735981504402,2.04370635334587));
#87160=CARTESIAN_POINT('Ctrl Pts',(-10.2913206411272,16.281223938107,2.06006174105072));
#87161=CARTESIAN_POINT('Ctrl Pts',(-10.4163541484964,16.2873373706702,2.09112077805399));
#87162=CARTESIAN_POINT('Ctrl Pts',(-10.5826658290999,16.2960794534488,2.15654352199211));
#87163=CARTESIAN_POINT('Ctrl Pts',(-10.6286010439063,16.2985736002872,2.17741358091135));
#87164=CARTESIAN_POINT('Ctrl Pts',(-10.6947898098933,16.3024084913463,2.2117136588335));
#87165=CARTESIAN_POINT('Ctrl Pts',(-10.7159361502919,16.3036721631857,2.22334426289036));
#87166=CARTESIAN_POINT('Ctrl Pts',(-10.7415792734289,16.3052642392268,2.23828559812841));
#87167=CARTESIAN_POINT('Ctrl Pts',(-10.7463584901551,16.305563565692,2.24110681435914));
#87168=CARTESIAN_POINT('Ctrl Pts',(-10.753855772242,16.3060374244808,2.24559022854256));
#87169=CARTESIAN_POINT('Ctrl Pts',(-10.75658470394,16.3062108069295,2.24723426554002));
#87170=CARTESIAN_POINT('Ctrl Pts',(-10.7617010945485,16.3065376173573,2.25033943510618));
#87171=CARTESIAN_POINT('Ctrl Pts',(-10.7640897415579,16.3066909134119,2.25179851334627));
#87172=CARTESIAN_POINT('Ctrl Pts',(-10.7695343565603,16.3070419686624,2.25514578031875));
#87173=CARTESIAN_POINT('Ctrl Pts',(-10.7725875654661,16.3072400114752,2.25703837255318));
#87174=CARTESIAN_POINT('Ctrl Pts',(-10.7806689126119,16.307767268733,2.26208903606904));
#87175=CARTESIAN_POINT('Ctrl Pts',(-10.7856847992492,16.308097693042,2.26526646618435));
#87176=CARTESIAN_POINT('Ctrl Pts',(-10.8211400406343,16.3104551112773,2.28802992905568));
#87177=CARTESIAN_POINT('Ctrl Pts',(-10.850860656992,16.3125455457606,2.30870736443489));
#87178=CARTESIAN_POINT('Ctrl Pts',(-10.889983757823,16.3154236451108,2.33813764282156));
#87179=CARTESIAN_POINT('Ctrl Pts',(-10.9000846742633,16.3161786893833,2.34594506480466));
#87180=CARTESIAN_POINT('Ctrl Pts',(-10.9780404983675,16.3220927880081,2.40784644086944));
#87181=CARTESIAN_POINT('Ctrl Pts',(-11.0410654047166,16.3273812225013,2.46774700270536));
#87182=CARTESIAN_POINT('Ctrl Pts',(-11.1317960502074,16.3355291550366,2.57079504022169));
#87183=CARTESIAN_POINT('Ctrl Pts',(-11.1631953606938,16.3384777505339,2.61041500492246));
#87184=CARTESIAN_POINT('Ctrl Pts',(-11.2096758111024,16.3430388786693,2.67574516583451));
#87185=CARTESIAN_POINT('Ctrl Pts',(-11.2261291153938,16.3446995376021,2.70042563079732));
#87186=CARTESIAN_POINT('Ctrl Pts',(-11.2464428171441,16.3468132937864,2.73300012363092));
#87187=CARTESIAN_POINT('Ctrl Pts',(-11.2509972732995,16.3472916848312,2.74045123026959));
#87188=CARTESIAN_POINT('Ctrl Pts',(-11.2582871263826,16.3480648767564,2.75262091583309));
#87189=CARTESIAN_POINT('Ctrl Pts',(-11.2610632732097,16.3483611491176,2.75731473021593));
#87190=CARTESIAN_POINT('Ctrl Pts',(-11.2663479948344,16.3489287125397,2.76636502539326));
#87191=CARTESIAN_POINT('Ctrl Pts',(-11.2688604817851,16.3492001416362,2.77071912226983));
#87192=CARTESIAN_POINT('Ctrl Pts',(-11.2745595435021,16.3498195477933,2.7807141094843));
#87193=CARTESIAN_POINT('Ctrl Pts',(-11.2777312084153,16.350166989459,2.78636340963398));
#87194=CARTESIAN_POINT('Ctrl Pts',(-11.2860605156266,16.3510868765282,2.80143294007527));
#87195=CARTESIAN_POINT('Ctrl Pts',(-11.2911522098383,16.3516569937792,2.81088929318332));
#87196=CARTESIAN_POINT('Ctrl Pts',(-11.33866645321,16.3570551302457,2.90150903466805));
#87197=CARTESIAN_POINT('Ctrl Pts',(-11.3734885037713,16.3616007524379,2.98643268033429));
#87198=CARTESIAN_POINT('Ctrl Pts',(-11.4330550950195,16.3715860348141,3.18224110963936));
#87199=CARTESIAN_POINT('Ctrl Pts',(-11.4533113551798,16.3769507256209,3.293852749732));
#87200=CARTESIAN_POINT('Ctrl Pts',(-11.4611845277739,16.3834803001121,3.41705195689414));
#87201=CARTESIAN_POINT('Ctrl Pts',(-11.4617375201281,16.3840360648367,3.42744648870476));
#87202=CARTESIAN_POINT('Ctrl Pts',(-11.462353748965,16.3848190010061,3.44194327713486));
#87203=CARTESIAN_POINT('Ctrl Pts',(-11.4625107000311,16.385041207398,3.44604148212911));
#87204=CARTESIAN_POINT('Ctrl Pts',(-11.4627482229919,16.3854205677168,3.45300928691118));
#87205=CARTESIAN_POINT('Ctrl Pts',(-11.4628375825116,16.3855772373467,3.45587859872773));
#87206=CARTESIAN_POINT('Ctrl Pts',(-11.4629927204368,16.3858785321493,3.46138027023476));
#87207=CARTESIAN_POINT('Ctrl Pts',(-11.4630598374641,16.3860230779656,3.46401256677904));
#87208=CARTESIAN_POINT('Ctrl Pts',(-11.4632030117003,16.3863688545646,3.47029291813981));
#87209=CARTESIAN_POINT('Ctrl Pts',(-11.463272529837,16.3865704415006,3.47394108602005));
#87210=CARTESIAN_POINT('Ctrl Pts',(-11.4634418718914,16.3871835756994,3.4849985064854));
#87211=CARTESIAN_POINT('Ctrl Pts',(-11.4634990664671,16.3875973454599,3.49240817566415));
#87212=CARTESIAN_POINT('Ctrl Pts',(-11.4634999963152,16.3880172148887,3.4998785531803));
#87213=CARTESIAN_POINT('Ctrl Pts',(-11.4635,16.3880206279513,3.49993927663728));
#87214=CARTESIAN_POINT('Ctrl Pts',(-11.4635,16.3880240412434,3.49999999999839));
#87215=CARTESIAN_POINT('Origin',(-10.,13.2,3.5));
#87216=CARTESIAN_POINT('',(-11.4635,16.9599527886714,3.50000000001837));
#87217=CARTESIAN_POINT('',(-11.4635,16.8902616844768,3.4999999999813));
#87218=CARTESIAN_POINT('',(-11.4635,13.2,3.5));
#87219=CARTESIAN_POINT('',(-11.4634995966695,16.9598988801815,3.49891346965536));
#87220=CARTESIAN_POINT('Ctrl Pts',(-11.4635,16.9599527886714,3.50000000001837));
#87221=CARTESIAN_POINT('Ctrl Pts',(-11.4635,16.9599348168433,3.49963782541032));
#87222=CARTESIAN_POINT('Ctrl Pts',(-11.4634998655581,16.9599168473517,3.49927564859787));
#87223=CARTESIAN_POINT('Ctrl Pts',(-11.4634995966695,16.9598988801815,3.49891346965532));
#87224=CARTESIAN_POINT('Ctrl Pts',(-11.4634995979088,16.9598989630521,3.4989151401456));
#87225=CARTESIAN_POINT('Ctrl Pts',(-11.4634505510007,16.9566165950605,3.43274979180149));
#87226=CARTESIAN_POINT('Ctrl Pts',(-11.4589144860793,16.9534233256929,3.36666071639118));
#87227=CARTESIAN_POINT('Ctrl Pts',(-11.4420526131649,16.9473774955259,3.24374040176786));
#87228=CARTESIAN_POINT('Ctrl Pts',(-11.430786897264,16.9445362947727,3.18689830496202));
#87229=CARTESIAN_POINT('Ctrl Pts',(-11.4095708260853,16.9402241967998,3.1055002145385));
#87230=CARTESIAN_POINT('Ctrl Pts',(-11.4022758947889,16.9388544197586,3.0803070884726));
#87231=CARTESIAN_POINT('Ctrl Pts',(-11.392579590649,16.9371433711262,3.04990365950361));
#87232=CARTESIAN_POINT('Ctrl Pts',(-11.3908189862349,16.9368365715305,3.04449239588263));
#87233=CARTESIAN_POINT('Ctrl Pts',(-11.388014013278,16.9363535536954,3.03603912595516));
#87234=CARTESIAN_POINT('Ctrl Pts',(-11.3869910795332,16.9361785611847,3.03299000161903));
#87235=CARTESIAN_POINT('Ctrl Pts',(-11.3850610953427,16.935850498388,3.02729944777417));
#87236=CARTESIAN_POINT('Ctrl Pts',(-11.3841565302295,16.9356975731559,3.0246572296684));
#87237=CARTESIAN_POINT('Ctrl Pts',(-11.3820681126217,16.9353464110128,3.0186135089699));
#87238=CARTESIAN_POINT('Ctrl Pts',(-11.3808792660396,16.9351478849696,3.01521378554841));
#87239=CARTESIAN_POINT('Ctrl Pts',(-11.3777292503128,16.9346254963236,3.0063113439938));
#87240=CARTESIAN_POINT('Ctrl Pts',(-11.3757476815438,16.9343004875987,3.00081597517593));
#87241=CARTESIAN_POINT('Ctrl Pts',(-11.3618763629126,16.932050532595,2.9630574503832));
#87242=CARTESIAN_POINT('Ctrl Pts',(-11.3488865384744,16.9300682729349,2.93121245532271));
#87243=CARTESIAN_POINT('Ctrl Pts',(-11.293718808576,16.922174719466,2.80851293127426));
#87244=CARTESIAN_POINT('Ctrl Pts',(-11.2433816407423,16.9160426227228,2.72162635652017));
#87245=CARTESIAN_POINT('Ctrl Pts',(-11.1543378701479,16.907036750944,2.59889747505946));
#87246=CARTESIAN_POINT('Ctrl Pts',(-11.1219317177388,16.9040296668239,2.55885617874726));
#87247=CARTESIAN_POINT('Ctrl Pts',(-11.0741732928337,16.8999679898767,2.50582728916153));
#87248=CARTESIAN_POINT('Ctrl Pts',(-11.0605661263867,16.8988479581727,2.49132404247235));
#87249=CARTESIAN_POINT('Ctrl Pts',(-11.0363968235167,16.8969216271248,2.46659311391925));
#87250=CARTESIAN_POINT('Ctrl Pts',(-11.0259685650123,16.8961098616748,2.45623915874379));
#87251=CARTESIAN_POINT('Ctrl Pts',(-11.0106696827442,16.8949462177781,2.44150015165882));
#87252=CARTESIAN_POINT('Ctrl Pts',(-11.0059230055867,16.8945888710161,2.43698821956649));
#87253=CARTESIAN_POINT('Ctrl Pts',(-10.9974474697348,16.8939572515617,2.42903944613702));
#87254=CARTESIAN_POINT('Ctrl Pts',(-10.9937307562888,16.8936824374249,2.42558986056712));
#87255=CARTESIAN_POINT('Ctrl Pts',(-10.986534182009,16.8931544420089,2.4189798085762));
#87256=CARTESIAN_POINT('Ctrl Pts',(-10.9830568803333,16.8929011491501,2.41581665882687));
#87257=CARTESIAN_POINT('Ctrl Pts',(-10.9747914194238,16.8923033508257,2.40837038843208));
#87258=CARTESIAN_POINT('Ctrl Pts',(-10.9699901572121,16.8919594575289,2.40410191307195));
#87259=CARTESIAN_POINT('Ctrl Pts',(-10.9529945420396,16.8907537297291,2.38919146550323));
#87260=CARTESIAN_POINT('Ctrl Pts',(-10.9406516713332,16.8898988864544,2.37872008040215));
#87261=CARTESIAN_POINT('Ctrl Pts',(-10.8225067423732,16.8819019333641,2.28181297904141));
#87262=CARTESIAN_POINT('Ctrl Pts',(-10.7052728600729,16.8754302215461,2.21039232986514));
#87263=CARTESIAN_POINT('Ctrl Pts',(-10.537623296873,16.8664692659895,2.13805041288576));
#87264=CARTESIAN_POINT('Ctrl Pts',(-10.4945831035662,16.8641836797743,2.1218372742373));
#87265=CARTESIAN_POINT('Ctrl Pts',(-10.4291872197754,16.8606393198545,2.10066112810666));
#87266=CARTESIAN_POINT('Ctrl Pts',(-10.4073602879359,16.8594446526317,2.09415206032007));
#87267=CARTESIAN_POINT('Ctrl Pts',(-10.38013517239,16.8579302037356,2.08672041343235));
#87268=CARTESIAN_POINT('Ctrl Pts',(-10.3748708316213,16.8576362479258,2.08531494783818));
#87269=CARTESIAN_POINT('Ctrl Pts',(-10.3665384469342,16.857169037837,2.08314015476809));
#87270=CARTESIAN_POINT('Ctrl Pts',(-10.363475492954,16.856996880599,2.08235130594908));
#87271=CARTESIAN_POINT('Ctrl Pts',(-10.3576937785843,16.8566710936699,2.08088222294295));
#87272=CARTESIAN_POINT('Ctrl Pts',(-10.3549756081898,16.8565175864081,2.08019986564182));
#87273=CARTESIAN_POINT('Ctrl Pts',(-10.3487349485336,16.8561643729621,2.07865227961618));
#87274=CARTESIAN_POINT('Ctrl Pts',(-10.3452111910898,16.8559643698027,2.07779233600281));
#87275=CARTESIAN_POINT('Ctrl Pts',(-10.3357927334898,16.8554283587612,2.07553090523285));
#87276=CARTESIAN_POINT('Ctrl Pts',(-10.3298925294139,16.8550910773904,2.0741529260608));
#87277=CARTESIAN_POINT('Ctrl Pts',(-10.285557765369,16.8525463825345,2.06408855289314));
#87278=CARTESIAN_POINT('Ctrl Pts',(-10.2467979378014,16.8502638710549,2.05692163188722));
#87279=CARTESIAN_POINT('Ctrl Pts',(-10.1077261063655,16.8419782180728,2.03697295504369));
#87280=CARTESIAN_POINT('Ctrl Pts',(-10.0064338543024,16.8357892791638,2.03302588819919));
#87281=CARTESIAN_POINT('Ctrl Pts',(-9.84136043219604,16.8260031288557,2.04370265268689));
#87282=CARTESIAN_POINT('Ctrl Pts',(-9.77751885899916,16.8222871579585,2.05208000632784));
#87283=CARTESIAN_POINT('Ctrl Pts',(-9.69942826141916,16.8178482850114,2.06761639188507));
#87284=CARTESIAN_POINT('Ctrl Pts',(-9.68447511395744,16.8170029725733,2.07083582395915));
#87285=CARTESIAN_POINT('Ctrl Pts',(-9.66296407630395,16.8157933210572,2.07582125955562));
#87286=CARTESIAN_POINT('Ctrl Pts',(-9.65636404431078,16.8154230458648,2.07739934249798));
#87287=CARTESIAN_POINT('Ctrl Pts',(-9.64486632553198,16.8147794632248,2.08023315872866));
#87288=CARTESIAN_POINT('Ctrl Pts',(-9.63996376326172,16.8145055091208,2.08146846371276));
#87289=CARTESIAN_POINT('Ctrl Pts',(-9.63049308560946,16.8139771597648,2.083907063649));
#87290=CARTESIAN_POINT('Ctrl Pts',(-9.62592420726582,16.8137226647164,2.08510711847995));
#87291=CARTESIAN_POINT('Ctrl Pts',(-9.61383413929475,16.8130502276327,2.08834533300278));
#87292=CARTESIAN_POINT('Ctrl Pts',(-9.60632322247638,16.8126335094872,2.09042149248491));
#87293=CARTESIAN_POINT('Ctrl Pts',(-9.57951634167599,16.811149633807,2.09806240129607));
#87294=CARTESIAN_POINT('Ctrl Pts',(-9.5603183195409,16.8100933330598,2.10396432390656));
#87295=CARTESIAN_POINT('Ctrl Pts',(-9.42177424697449,16.8025046244441,2.14969767431031));
#87296=CARTESIAN_POINT('Ctrl Pts',(-9.30789043075783,16.7965112324549,2.20437387210448));
#87297=CARTESIAN_POINT('Ctrl Pts',(-9.16053025606825,16.7879112334743,2.30015983276175));
#87298=CARTESIAN_POINT('Ctrl Pts',(-9.12008474140615,16.7854398240238,2.32949824368207));
#87299=CARTESIAN_POINT('Ctrl Pts',(-9.06255077725626,16.7816365418002,2.37590191275258));
#87300=CARTESIAN_POINT('Ctrl Pts',(-9.04425504121095,16.780380279607,2.39141576928095));
#87301=CARTESIAN_POINT('Ctrl Pts',(-9.02221514660181,16.7787965924843,2.41105569405283));
#87302=CARTESIAN_POINT('Ctrl Pts',(-9.01810146243788,16.7784978875836,2.41476353685228));
#87303=CARTESIAN_POINT('Ctrl Pts',(-9.01165704475714,16.7780248304845,2.4206388082833));
#87304=CARTESIAN_POINT('Ctrl Pts',(-9.00931212431326,16.7778516222012,2.42279068332406));
#87305=CARTESIAN_POINT('Ctrl Pts',(-9.00491854616952,16.7775250163079,2.42684904047287));
#87306=CARTESIAN_POINT('Ctrl Pts',(-9.00286832750737,16.7773717496192,2.42875375895468));
#87307=CARTESIAN_POINT('Ctrl Pts',(-8.99819729805911,16.7770206048863,2.43311832152913));
#87308=CARTESIAN_POINT('Ctrl Pts',(-8.99558007992412,16.7768224421555,2.43558194629183));
#87309=CARTESIAN_POINT('Ctrl Pts',(-8.98865671149561,16.7762945407183,2.44214728344486));
#87310=CARTESIAN_POINT('Ctrl Pts',(-8.98436648736165,16.7759635870576,2.4462656014528));
#87311=CARTESIAN_POINT('Ctrl Pts',(-8.95385266558713,16.7735829679234,2.47591622289546));
#87312=CARTESIAN_POINT('Ctrl Pts',(-8.9285718478928,16.7714684311253,2.50239631510661));
#87313=CARTESIAN_POINT('Ctrl Pts',(-8.89656418863795,16.7686288758347,2.53854368063939));
#87314=CARTESIAN_POINT('Ctrl Pts',(-8.88892145670163,16.7679377470337,2.54738606703397));
#87315=CARTESIAN_POINT('Ctrl Pts',(-8.82539449770146,16.7620871529143,2.62268922950463));
#87316=CARTESIAN_POINT('Ctrl Pts',(-8.77542089830049,16.7567948256325,2.69391125049634));
#87317=CARTESIAN_POINT('Ctrl Pts',(-8.6975801841063,16.7475413175796,2.82895557027836));
#87318=CARTESIAN_POINT('Ctrl Pts',(-8.66737704869881,16.7435384840293,2.89113537144882));
#87319=CARTESIAN_POINT('Ctrl Pts',(-8.63576709211558,16.738799909474,2.96995035869295));
#87320=CARTESIAN_POINT('Ctrl Pts',(-8.63010004258949,16.7379223360277,2.98477365773653));
#87321=CARTESIAN_POINT('Ctrl Pts',(-8.62232066124691,16.7366753390207,3.0061586091418));
#87322=CARTESIAN_POINT('Ctrl Pts',(-8.62001197629201,16.7362994592426,3.01264721561729));
#87323=CARTESIAN_POINT('Ctrl Pts',(-8.61608249733157,16.7356493468252,3.02394293719634));
#87324=CARTESIAN_POINT('Ctrl Pts',(-8.61444074906282,16.7353744291465,3.02874259233389));
#87325=CARTESIAN_POINT('Ctrl Pts',(-8.61132658429202,16.7348464660836,3.03800382389259));
#87326=CARTESIAN_POINT('Ctrl Pts',(-8.60985063444537,16.7345933077595,3.04246413868554));
#87327=CARTESIAN_POINT('Ctrl Pts',(-8.60641052446307,16.7339961813672,3.05303046676262));
#87328=CARTESIAN_POINT('Ctrl Pts',(-8.60446496765342,16.7336528221063,3.05914246604871));
#87329=CARTESIAN_POINT('Ctrl Pts',(-8.5977698010131,16.7324508032018,3.08066394893246));
#87330=CARTESIAN_POINT('Ctrl Pts',(-8.59323463821695,16.7315990774522,3.09613925831642));
#87331=CARTESIAN_POINT('Ctrl Pts',(-8.55653952176319,16.7243605403908,3.22948115749335));
#87332=CARTESIAN_POINT('Ctrl Pts',(-8.53900015189412,16.7184929782355,3.35086770589383));
#87333=CARTESIAN_POINT('Ctrl Pts',(-8.53570058869568,16.7097645653421,3.52988618448959));
#87334=CARTESIAN_POINT('Ctrl Pts',(-8.53796740850145,16.7069711807532,3.58675126277679));
#87335=CARTESIAN_POINT('Ctrl Pts',(-8.54607741690219,16.7027244199626,3.66915863880108));
#87336=CARTESIAN_POINT('Ctrl Pts',(-8.54930487280592,16.7013686738462,3.69490768634974));
#87337=CARTESIAN_POINT('Ctrl Pts',(-8.5540696632921,16.6996733540424,3.72616341122331));
#87338=CARTESIAN_POINT('Ctrl Pts',(-8.55495711411148,16.6993675118403,3.73176600917943));
#87339=CARTESIAN_POINT('Ctrl Pts',(-8.55639808290768,16.6988856716973,3.74053289435875));
#87340=CARTESIAN_POINT('Ctrl Pts',(-8.55692949645908,16.6987108896822,3.74370082007357));
#87341=CARTESIAN_POINT('Ctrl Pts',(-8.55794253261088,16.6983830028226,3.74962033970232));
#87342=CARTESIAN_POINT('Ctrl Pts',(-8.55842160601236,16.6982300413816,3.75237231783145));
#87343=CARTESIAN_POINT('Ctrl Pts',(-8.55953745755101,16.697878506009,3.75867533535166));
#87344=CARTESIAN_POINT('Ctrl Pts',(-8.56017948779137,16.6976796406277,3.76222539420633));
#87345=CARTESIAN_POINT('Ctrl Pts',(-8.56189917038474,16.6971557817959,3.77153750492745));
#87346=CARTESIAN_POINT('Ctrl Pts',(-8.5629983166613,16.6968296320128,3.77729546057872));
#87347=CARTESIAN_POINT('Ctrl Pts',(-8.57086177896742,16.6945553387951,3.81718604933112));
#87348=CARTESIAN_POINT('Ctrl Pts',(-8.57880647809686,16.6925485101136,3.85107213138752));
#87349=CARTESIAN_POINT('Ctrl Pts',(-8.61416277230028,16.6846517604419,3.98086838599768));
#87350=CARTESIAN_POINT('Ctrl Pts',(-8.65014264478111,16.6785461257338,4.07416466700464));
#87351=CARTESIAN_POINT('Ctrl Pts',(-8.72690957835493,16.6684828595072,4.22521074513935));
#87352=CARTESIAN_POINT('Ctrl Pts',(-8.76288837434592,16.6644396541601,4.28501387943824));
#87353=CARTESIAN_POINT('Ctrl Pts',(-8.81217229757436,16.6596591360626,4.35507420532179));
#87354=CARTESIAN_POINT('Ctrl Pts',(-8.8215601090728,16.6587771451913,4.36796658865068));
#87355=CARTESIAN_POINT('Ctrl Pts',(-8.83530964021091,16.6575250471504,4.38621455276451));
#87356=CARTESIAN_POINT('Ctrl Pts',(-8.83950122630601,16.6571484109448,4.39169639802833));
#87357=CARTESIAN_POINT('Ctrl Pts',(-8.8468424935228,16.6564974140959,4.40115801623208));
#87358=CARTESIAN_POINT('Ctrl Pts',(-8.84997436962335,16.6562223632046,4.40515139912759));
#87359=CARTESIAN_POINT('Ctrl Pts',(-8.85604342268691,16.6556944388202,4.41280755952471));
#87360=CARTESIAN_POINT('Ctrl Pts',(-8.85897757295679,16.6554414506537,4.41647264727055));
#87361=CARTESIAN_POINT('Ctrl Pts',(-8.86595384655399,16.6548451758194,4.42510137117518));
#87362=CARTESIAN_POINT('Ctrl Pts',(-8.87001101784079,16.654502493703,4.43005275498897));
#87363=CARTESIAN_POINT('Ctrl Pts',(-8.88435319922937,16.6533051898675,4.4473236038106));
#87364=CARTESIAN_POINT('Ctrl Pts',(-8.89480844094996,16.6524574294324,4.45950061956521));
#87365=CARTESIAN_POINT('Ctrl Pts',(-8.98711689877095,16.6451783376181,4.56349931730929));
#87366=CARTESIAN_POINT('Ctrl Pts',(-9.08004075503841,16.6392746440423,4.64483200697732));
#87367=CARTESIAN_POINT('Ctrl Pts',(-9.22874769995715,16.6305304575254,4.74505958107827));
#87368=CARTESIAN_POINT('Ctrl Pts',(-9.27721961215285,16.6277626068333,4.77380969143141));
#87369=CARTESIAN_POINT('Ctrl Pts',(-9.35013386353142,16.6235507898639,4.81155319672937));
#87370=CARTESIAN_POINT('Ctrl Pts',(-9.37335249344405,16.6222026129317,4.82280403834688));
#87371=CARTESIAN_POINT('Ctrl Pts',(-9.4020142524743,16.6205157796641,4.83576845361831));
#87372=CARTESIAN_POINT('Ctrl Pts',(-9.40718708947211,16.6202104588071,4.83807218300337));
#87373=CARTESIAN_POINT('Ctrl Pts',(-9.41531301069147,16.619729260021,4.84163470401166));
#87374=CARTESIAN_POINT('Ctrl Pts',(-9.41825714495305,16.6195545926937,4.84291392303114));
#87375=CARTESIAN_POINT('Ctrl Pts',(-9.42377142700586,16.6192268012539,4.84528832849124));
#87376=CARTESIAN_POINT('Ctrl Pts',(-9.42634051475876,16.6190738196438,4.84638584724973));
#87377=CARTESIAN_POINT('Ctrl Pts',(-9.43223744858918,16.618722078918,4.84888508574561));
#87378=CARTESIAN_POINT('Ctrl Pts',(-9.43556734261051,16.6185230270796,4.85028184614459));
#87379=CARTESIAN_POINT('Ctrl Pts',(-9.44432662641474,16.6179983598569,4.85391796096234));
#87380=CARTESIAN_POINT('Ctrl Pts',(-9.44976433100091,16.6176715825077,4.85613695817576));
#87381=CARTESIAN_POINT('Ctrl Pts',(-9.48772140460113,16.6153838974898,4.87136046296472));
#87382=CARTESIAN_POINT('Ctrl Pts',(-9.520682759239,16.613363543386,4.88322575100979));
#87383=CARTESIAN_POINT('Ctrl Pts',(-9.64880703307678,16.605465073032,4.9242179803999));
#87384=CARTESIAN_POINT('Ctrl Pts',(-9.74642354967697,16.5993740197994,4.94479516224972));
#87385=CARTESIAN_POINT('Ctrl Pts',(-9.89652529098856,16.5904089066308,4.96074336300252));
#87386=CARTESIAN_POINT('Ctrl Pts',(-9.94793039616041,16.5874038992011,4.96347795868971));
#87387=CARTESIAN_POINT('Ctrl Pts',(-10.0293970093133,16.5827673594069,4.96351265151782));
#87388=CARTESIAN_POINT('Ctrl Pts',(-10.0594119368165,16.5810856962556,4.96260174813191));
#87389=CARTESIAN_POINT('Ctrl Pts',(-10.0981308889068,16.5789496295749,4.96023267207046));
#87390=CARTESIAN_POINT('Ctrl Pts',(-10.1068776691884,16.5784692638795,4.95961854484892));
#87391=CARTESIAN_POINT('Ctrl Pts',(-10.121061329657,16.5776937440279,4.95849450272809));
#87392=CARTESIAN_POINT('Ctrl Pts',(-10.1265017148023,16.5773971010036,4.95803270789957));
#87393=CARTESIAN_POINT('Ctrl Pts',(-10.136941519766,16.5768293977552,4.95708767615026));
#87394=CARTESIAN_POINT('Ctrl Pts',(-10.1419412774326,16.5765581957941,4.95660912754752));
#87395=CARTESIAN_POINT('Ctrl Pts',(-10.1533641933419,16.5759400936031,4.95545641775633));
#87396=CARTESIAN_POINT('Ctrl Pts',(-10.1597855765533,16.575593721823,4.95476545571316));
#87397=CARTESIAN_POINT('Ctrl Pts',(-10.1768073477316,16.5746783516421,4.9528197924749));
#87398=CARTESIAN_POINT('Ctrl Pts',(-10.1873990481804,16.5741116454794,4.951491575025));
#87399=CARTESIAN_POINT('Ctrl Pts',(-10.2950374637156,16.5683794873798,4.93679566764981));
#87400=CARTESIAN_POINT('Ctrl Pts',(-10.3905267454149,16.5635415900345,4.91383196217092));
#87401=CARTESIAN_POINT('Ctrl Pts',(-10.5593075488035,16.5548341843128,4.85482080836481));
#87402=CARTESIAN_POINT('Ctrl Pts',(-10.6332543843851,16.5509508837894,4.82187424852942));
#87403=CARTESIAN_POINT('Ctrl Pts',(-10.7325920023136,16.5451976834576,4.76735852213373));
#87404=CARTESIAN_POINT('Ctrl Pts',(-10.760554920684,16.5435125836994,4.75077758700944));
#87405=CARTESIAN_POINT('Ctrl Pts',(-10.7930342758906,16.5414485466426,4.73002659454609));
#87406=CARTESIAN_POINT('Ctrl Pts',(-10.7981076368049,16.541122956629,4.72674079721484));
#87407=CARTESIAN_POINT('Ctrl Pts',(-10.8059132472803,16.5406168521236,4.72161652409847));
#87408=CARTESIAN_POINT('Ctrl Pts',(-10.8086599508535,16.5404377626776,4.71980005637847));
#87409=CARTESIAN_POINT('Ctrl Pts',(-10.8137178574439,16.540106089571,4.71643053731557));
#87410=CARTESIAN_POINT('Ctrl Pts',(-10.8160307721753,16.5399536823543,4.71488015135012));
#87411=CARTESIAN_POINT('Ctrl Pts',(-10.8212373134589,16.5396089395748,4.71136854189779));
#87412=CARTESIAN_POINT('Ctrl Pts',(-10.8241283291991,16.5394163556338,4.70940355787654));
#87413=CARTESIAN_POINT('Ctrl Pts',(-10.8315429212018,16.5389195048439,4.70432502972887));
#87414=CARTESIAN_POINT('Ctrl Pts',(-10.8360560213095,16.5386142625798,4.70119637625286));
#87415=CARTESIAN_POINT('Ctrl Pts',(-10.8633364370759,16.5367525146598,4.68205632835596));
#87416=CARTESIAN_POINT('Ctrl Pts',(-10.8856593950103,16.5351584179006,4.66542447088776));
#87417=CARTESIAN_POINT('Ctrl Pts',(-10.9909613289468,16.5273438729891,4.58219552331111));
#87418=CARTESIAN_POINT('Ctrl Pts',(-11.0669859044227,16.5208156003626,4.50731975952143));
#87419=CARTESIAN_POINT('Ctrl Pts',(-11.1788159931942,16.5102991949617,4.37017500146768));
#87420=CARTESIAN_POINT('Ctrl Pts',(-11.2194003851939,16.5062029656009,4.31232787288269));
#87421=CARTESIAN_POINT('Ctrl Pts',(-11.2639003112585,16.5013674460147,4.23800123589068));
#87422=CARTESIAN_POINT('Ctrl Pts',(-11.2719175317066,16.5004796980069,4.224096431662));
#87423=CARTESIAN_POINT('Ctrl Pts',(-11.2830612488159,16.4992209563954,4.20401274424045));
#87424=CARTESIAN_POINT('Ctrl Pts',(-11.2863749560413,16.4988433382746,4.19793952964295));
#87425=CARTESIAN_POINT('Ctrl Pts',(-11.2920460416399,16.4981911923057,4.18736821447288));
#87426=CARTESIAN_POINT('Ctrl Pts',(-11.2944232839424,16.4979159674379,4.18288095512766));
#87427=CARTESIAN_POINT('Ctrl Pts',(-11.2989514209203,16.4973880887414,4.17422507988745));
#87428=CARTESIAN_POINT('Ctrl Pts',(-11.3011057203239,16.4971353180025,4.1700583239585));
#87429=CARTESIAN_POINT('Ctrl Pts',(-11.3061449502822,16.4965401341449,4.16019571572897));
#87430=CARTESIAN_POINT('Ctrl Pts',(-11.3090127270379,16.496198320132,4.15449117367747));
#87431=CARTESIAN_POINT('Ctrl Pts',(-11.3189139535921,16.4950070428047,4.13447037092822));
#87432=CARTESIAN_POINT('Ctrl Pts',(-11.3257507522875,16.4941643485673,4.12005776959551));
#87433=CARTESIAN_POINT('Ctrl Pts',(-11.383670451414,16.4868354722167,3.99261800050048));
#87434=CARTESIAN_POINT('Ctrl Pts',(-11.4204271278246,16.4808873786295,3.87363819008585));
#87435=CARTESIAN_POINT('Ctrl Pts',(-11.4448776580043,16.4739460446586,3.73344087256024));
#87436=CARTESIAN_POINT('Ctrl Pts',(-11.4476794056018,16.4730521087111,3.71538433178781));
#87437=CARTESIAN_POINT('Ctrl Pts',(-11.4576173709659,16.4694210514421,3.64233363242904));
#87438=CARTESIAN_POINT('Ctrl Pts',(-11.4619627599203,16.4666390583929,3.58701144672067));
#87439=CARTESIAN_POINT('Ctrl Pts',(-11.4633863975749,16.4631513064801,3.52105591908527));
#87440=CARTESIAN_POINT('Ctrl Pts',(-11.4635,16.4625893807927,3.51052796134199));
#87441=CARTESIAN_POINT('Ctrl Pts',(-11.4635,16.4620214545711,3.5));
#87442=CARTESIAN_POINT('',(-11.4634995813664,16.8901969352951,3.49889304900151));
#87443=CARTESIAN_POINT('Ctrl Pts',(-11.4635,16.3880240412434,3.49999999999839));
#87444=CARTESIAN_POINT('Ctrl Pts',(-11.4635,16.3931801882591,3.59172920727273));
#87445=CARTESIAN_POINT('Ctrl Pts',(-11.4548759495079,16.3987234838506,3.6832472985968));
#87446=CARTESIAN_POINT('Ctrl Pts',(-11.4176111906088,16.4107369833002,3.87925201809585));
#87447=CARTESIAN_POINT('Ctrl Pts',(-11.3858332866077,16.4171472519497,3.98262500487411));
#87448=CARTESIAN_POINT('Ctrl Pts',(-11.3362257707668,16.424129631001,4.09717824540646));
#87449=CARTESIAN_POINT('Ctrl Pts',(-11.3291996942818,16.4250713372376,4.11265763212551));
#87450=CARTESIAN_POINT('Ctrl Pts',(-11.3190904515954,16.4263637814336,4.13393663748888));
#87451=CARTESIAN_POINT('Ctrl Pts',(-11.3162357366293,16.4267222847214,4.13984276773713));
#87452=CARTESIAN_POINT('Ctrl Pts',(-11.3112514155487,16.4273373012125,4.14998031660428));
#87453=CARTESIAN_POINT('Ctrl Pts',(-11.3091408143689,16.4275944652624,4.15422092265529));
#87454=CARTESIAN_POINT('Ctrl Pts',(-11.3047372189894,16.4281243663789,4.16296195200507));
#87455=CARTESIAN_POINT('Ctrl Pts',(-11.3024414382342,16.4283970021939,4.16746090617847));
#87456=CARTESIAN_POINT('Ctrl Pts',(-11.2970246869188,16.4290319323183,4.17794153931007));
#87457=CARTESIAN_POINT('Ctrl Pts',(-11.2938855373527,16.4293935860143,4.18391372811532));
#87458=CARTESIAN_POINT('Ctrl Pts',(-11.2836022134155,16.4305583430662,4.20315337255562));
#87459=CARTESIAN_POINT('Ctrl Pts',(-11.27629427864,16.4313556853812,4.2163324955626));
#87460=CARTESIAN_POINT('Ctrl Pts',(-11.2376377263323,16.4354247081208,4.28357547800333));
#87461=CARTESIAN_POINT('Ctrl Pts',(-11.2030517617731,16.4385781624238,4.33570644424629));
#87462=CARTESIAN_POINT('Ctrl Pts',(-11.1110468408351,16.4460900895755,4.45678035221242));
#87463=CARTESIAN_POINT('Ctrl Pts',(-11.0504290663564,16.4503573169292,4.52296220127521));
#87464=CARTESIAN_POINT('Ctrl Pts',(-10.945338350377,16.4573958303877,4.61844384484336));
#87465=CARTESIAN_POINT('Ctrl Pts',(-10.9046695933794,16.4600521107499,4.65158719627362));
#87466=CARTESIAN_POINT('Ctrl Pts',(-10.8565577731584,16.463229992384,4.68667257769171));
#87467=CARTESIAN_POINT('Ctrl Pts',(-10.8507699136273,16.4636128562546,4.69082894462523));
#87468=CARTESIAN_POINT('Ctrl Pts',(-10.8420793077374,16.4641889438487,4.69697413023724));
#87469=CARTESIAN_POINT('Ctrl Pts',(-10.83919927963,16.4643800529696,4.69899507818673));
#87470=CARTESIAN_POINT('Ctrl Pts',(-10.8340250536535,16.4647238017809,4.70259811500445));
#87471=CARTESIAN_POINT('Ctrl Pts',(-10.8317335986452,16.4648761779959,4.7041840544719));
#87472=CARTESIAN_POINT('Ctrl Pts',(-10.8267374314621,16.4652087347354,4.70762088849826));
#87473=CARTESIAN_POINT('Ctrl Pts',(-10.8240310633824,16.4653890771003,4.7094692212142));
#87474=CARTESIAN_POINT('Ctrl Pts',(-10.8163785367876,16.4658995230326,4.71465795910971));
#87475=CARTESIAN_POINT('Ctrl Pts',(-10.8114181785268,16.4662309914072,4.71797717959226));
#87476=CARTESIAN_POINT('Ctrl Pts',(-10.7805880623926,16.4682941525806,4.73833521069324));
#87477=CARTESIAN_POINT('Ctrl Pts',(-10.7542047482493,16.4700725589853,4.75457831055091));
#87478=CARTESIAN_POINT('Ctrl Pts',(-10.590082747963,16.4811202693212,4.84857300899681));
#87479=CARTESIAN_POINT('Ctrl Pts',(-10.4409930404533,16.490944853355,4.90441804275674));
#87480=CARTESIAN_POINT('Ctrl Pts',(-10.2585434265272,16.5015105828399,4.94075022572236));
#87481=CARTESIAN_POINT('Ctrl Pts',(-10.2311136817078,16.5030670935772,4.94540393353071));
#87482=CARTESIAN_POINT('Ctrl Pts',(-10.1947869504817,16.5050875314302,4.95050642755518));
#87483=CARTESIAN_POINT('Ctrl Pts',(-10.1859961768655,16.5055733367188,4.95165983601738));
#87484=CARTESIAN_POINT('Ctrl Pts',(-10.1717530185874,16.5063555169609,4.95339712741371));
#87485=CARTESIAN_POINT('Ctrl Pts',(-10.1663069730138,16.5066534274817,4.95403036461971));
#87486=CARTESIAN_POINT('Ctrl Pts',(-10.1558697446845,16.5072221737813,4.95518454295686));
#87487=CARTESIAN_POINT('Ctrl Pts',(-10.1508791982187,16.5074931606319,4.95571044503378));
#87488=CARTESIAN_POINT('Ctrl Pts',(-10.1393924158685,16.5081147301189,4.9568612131095));
#87489=CARTESIAN_POINT('Ctrl Pts',(-10.132894480934,16.508464754818,4.95746831824342));
#87490=CARTESIAN_POINT('Ctrl Pts',(-10.112570897897,16.5095546983652,4.95923011167431));
#87491=CARTESIAN_POINT('Ctrl Pts',(-10.0987325304649,16.5102898588875,4.96023170447868));
#87492=CARTESIAN_POINT('Ctrl Pts',(-10.0666348602718,16.5119800662877,4.96209647969414));
#87493=CARTESIAN_POINT('Ctrl Pts',(-10.0483693056904,16.512930681251,4.96281467305182));
#87494=CARTESIAN_POINT('Ctrl Pts',(-9.98472315620391,16.5162092832952,4.96412373234447));
#87495=CARTESIAN_POINT('Ctrl Pts',(-9.93933088742377,16.5184868547295,4.96294612254834));
#87496=CARTESIAN_POINT('Ctrl Pts',(-9.80857053458222,16.5249660434233,4.95345612520352));
#87497=CARTESIAN_POINT('Ctrl Pts',(-9.72379001921425,16.5290582179531,4.93975256620771));
#87498=CARTESIAN_POINT('Ctrl Pts',(-9.62381203559086,16.5341517004134,4.91443214209929));
#87499=CARTESIAN_POINT('Ctrl Pts',(-9.60700426248252,16.5350177910798,4.90985460029978));
#87500=CARTESIAN_POINT('Ctrl Pts',(-9.5518288556204,16.5379045404512,4.89376443966103));
#87501=CARTESIAN_POINT('Ctrl Pts',(-9.51385482115936,16.5399614332783,4.88097755935368));
#87502=CARTESIAN_POINT('Ctrl Pts',(-9.47077463775093,16.5424263247385,4.86447417897149));
#87503=CARTESIAN_POINT('Ctrl Pts',(-9.46510666962518,16.542753302647,4.86226223308327));
#87504=CARTESIAN_POINT('Ctrl Pts',(-9.45607458405374,16.5432788857912,4.8586723691638));
#87505=CARTESIAN_POINT('Ctrl Pts',(-9.45270146195518,16.5434761856947,4.85731712378299));
#87506=CARTESIAN_POINT('Ctrl Pts',(-9.44673516066509,16.5438270253892,4.85489414057631));
#87507=CARTESIAN_POINT('Ctrl Pts',(-9.44413995893464,16.5439802600057,4.85383149958612));
#87508=CARTESIAN_POINT('Ctrl Pts',(-9.43862675233822,16.5443071456383,4.85155551619068));
#87509=CARTESIAN_POINT('Ctrl Pts',(-9.43570966501676,16.544480909512,4.85034019935334));
#87510=CARTESIAN_POINT('Ctrl Pts',(-9.42778804029564,16.5449549294327,4.84700974106772));
#87511=CARTESIAN_POINT('Ctrl Pts',(-9.42279136023704,16.5452562623008,4.84487618524535));
#87512=CARTESIAN_POINT('Ctrl Pts',(-9.39711345763482,16.546816440524,4.83374239841065));
#87513=CARTESIAN_POINT('Ctrl Pts',(-9.37663148297218,16.5480998932401,4.82429322462625));
#87514=CARTESIAN_POINT('Ctrl Pts',(-9.3157234456813,16.5520171710776,4.79446779811624));
#87515=CARTESIAN_POINT('Ctrl Pts',(-9.27601749540531,16.5547065480505,4.77268618166388));
#87516=CARTESIAN_POINT('Ctrl Pts',(-9.18080049301202,16.5613952172425,4.71455343493635));
#87517=CARTESIAN_POINT('Ctrl Pts',(-9.12662471568174,16.5654120816084,4.67619893687998));
#87518=CARTESIAN_POINT('Ctrl Pts',(-9.01460132407091,16.5740074643417,4.58486954158093));
#87519=CARTESIAN_POINT('Ctrl Pts',(-8.95802159746886,16.578539913458,4.53064859576869));
#87520=CARTESIAN_POINT('Ctrl Pts',(-8.8989656985755,16.5834663997762,4.46419354430413));
#87521=CARTESIAN_POINT('Ctrl Pts',(-8.89197666623584,16.5840530964361,4.45615376590983));
#87522=CARTESIAN_POINT('Ctrl Pts',(-8.88089568501535,16.5849894141752,4.44312216822952));
#87523=CARTESIAN_POINT('Ctrl Pts',(-8.87674798086112,16.5853413032756,4.43817844538799));
#87524=CARTESIAN_POINT('Ctrl Pts',(-8.86943001400414,16.5859647498678,4.42933793048835));
#87525=CARTESIAN_POINT('Ctrl Pts',(-8.86624688001899,16.5862368246155,4.42545196854624));
#87526=CARTESIAN_POINT('Ctrl Pts',(-8.85964233623009,16.5868032470903,4.41730394004426));
#87527=CARTESIAN_POINT('Ctrl Pts',(-8.85622466260814,16.587097443206,4.41303893587688));
#87528=CARTESIAN_POINT('Ctrl Pts',(-8.84737448651616,16.587862193174,4.40186689280143));
#87529=CARTESIAN_POINT('Ctrl Pts',(-8.84198011378171,16.5883312382589,4.39492983765594));
#87530=CARTESIAN_POINT('Ctrl Pts',(-8.81832982760106,16.5904012420737,4.36394412148767));
#87531=CARTESIAN_POINT('Ctrl Pts',(-8.80075753444055,16.5919756559307,4.33938162819158));
#87532=CARTESIAN_POINT('Ctrl Pts',(-8.75509688571016,16.5961875208373,4.27119315531665));
#87533=CARTESIAN_POINT('Ctrl Pts',(-8.7285472486907,16.5987725644281,4.22658867551589));
#87534=CARTESIAN_POINT('Ctrl Pts',(-8.65549313553559,16.6064882822691,4.08753758299332));
#87535=CARTESIAN_POINT('Ctrl Pts',(-8.61675383388309,16.6114650354277,3.98941360058881));
#87536=CARTESIAN_POINT('Ctrl Pts',(-8.5811102198745,16.6183188830102,3.85977826741604));
#87537=CARTESIAN_POINT('Ctrl Pts',(-8.57420057649422,16.6198404290076,3.83133726956228));
#87538=CARTESIAN_POINT('Ctrl Pts',(-8.56699488810879,16.6217051353892,3.79725360452117));
#87539=CARTESIAN_POINT('Ctrl Pts',(-8.5658725030529,16.6220052749347,3.79179046697166));
#87540=CARTESIAN_POINT('Ctrl Pts',(-8.56409226819519,16.6224977668794,3.78286682885399));
#87541=CARTESIAN_POINT('Ctrl Pts',(-8.56341562646414,16.6226890892882,3.77941008268206));
#87542=CARTESIAN_POINT('Ctrl Pts',(-8.56222595806813,16.6230330650534,3.77321387624022));
#87543=CARTESIAN_POINT('Ctrl Pts',(-8.56170827151446,16.6231854534177,3.77047536194942));
#87544=CARTESIAN_POINT('Ctrl Pts',(-8.56059940163914,16.6235178519028,3.7645163290109));
#87545=CARTESIAN_POINT('Ctrl Pts',(-8.56001121040862,16.6236980226177,3.76129534303752));
#87546=CARTESIAN_POINT('Ctrl Pts',(-8.5583838549246,16.624207507531,3.75221140825435));
#87547=CARTESIAN_POINT('Ctrl Pts',(-8.5573696678812,16.6245381785504,3.74634412223357));
#87548=CARTESIAN_POINT('Ctrl Pts',(-8.55134556880129,16.6265854626481,3.71017990810905));
#87549=CARTESIAN_POINT('Ctrl Pts',(-8.54725479528341,16.6283479803188,3.67973968361974));
#87550=CARTESIAN_POINT('Ctrl Pts',(-8.5285311135885,16.639072922007,3.49703100312817));
#87551=CARTESIAN_POINT('Ctrl Pts',(-8.53688494605726,16.6485691405206,3.34335109958162));
#87552=CARTESIAN_POINT('Ctrl Pts',(-8.57566707559699,16.659153265462,3.16213651885384));
#87553=CARTESIAN_POINT('Ctrl Pts',(-8.58347270923564,16.660967740492,3.13077557289536));
#87554=CARTESIAN_POINT('Ctrl Pts',(-8.59487270734675,16.6632658523272,3.09068681023922));
#87555=CARTESIAN_POINT('Ctrl Pts',(-8.59752137310757,16.6637795661655,3.08170141918379));
#87556=CARTESIAN_POINT('Ctrl Pts',(-8.60188912971016,16.6645955717653,3.06739217437182));
#87557=CARTESIAN_POINT('Ctrl Pts',(-8.60355276122148,16.6648996496659,3.06205177596288));
#87558=CARTESIAN_POINT('Ctrl Pts',(-8.60660809910554,16.6654462275488,3.05243832333154));
#87559=CARTESIAN_POINT('Ctrl Pts',(-8.60798894163173,16.6656890768795,3.04816191184848));
#87560=CARTESIAN_POINT('Ctrl Pts',(-8.61128337021697,16.6662588213993,3.0381176547298));
#87561=CARTESIAN_POINT('Ctrl Pts',(-8.61321323588071,16.6665851808715,3.03235520841634));
#87562=CARTESIAN_POINT('Ctrl Pts',(-8.61893525489873,16.6675318060512,3.01561660642798));
#87563=CARTESIAN_POINT('Ctrl Pts',(-8.6228222725748,16.6681489595967,3.00467321942347));
#87564=CARTESIAN_POINT('Ctrl Pts',(-8.65854569652286,16.6736008560058,2.90777124321152));
#87565=CARTESIAN_POINT('Ctrl Pts',(-8.69826304939138,16.678152806262,2.82493093549761));
#87566=CARTESIAN_POINT('Ctrl Pts',(-8.79777360647408,16.6875817513774,2.65928737288595));
#87567=CARTESIAN_POINT('Ctrl Pts',(-8.85898594760522,16.6924178420713,2.57792151721275));
#87568=CARTESIAN_POINT('Ctrl Pts',(-8.94147503544416,16.6986964128879,2.48918745539993));
#87569=CARTESIAN_POINT('Ctrl Pts',(-8.95511887106203,16.6997288644021,2.47509002708458));
#87570=CARTESIAN_POINT('Ctrl Pts',(-8.97288692182853,16.7010724267843,2.4574548773814));
#87571=CARTESIAN_POINT('Ctrl Pts',(-8.97675370519814,16.7013647636604,2.45365941187148));
#87572=CARTESIAN_POINT('Ctrl Pts',(-8.98290657404069,16.7018300166335,2.44768674881562));
#87573=CARTESIAN_POINT('Ctrl Pts',(-8.98517882041117,16.7020018517127,2.4454952874364));
#87574=CARTESIAN_POINT('Ctrl Pts',(-8.98928045095832,16.7023121018062,2.44156501697216));
#87575=CARTESIAN_POINT('Ctrl Pts',(-8.99110725918038,16.7024503107574,2.4398235725568));
#87576=CARTESIAN_POINT('Ctrl Pts',(-8.99551134324725,16.7027835639416,2.4356469754949));
#87577=CARTESIAN_POINT('Ctrl Pts',(-8.99809296158382,16.7029789573942,2.43321646612632));
#87578=CARTESIAN_POINT('Ctrl Pts',(-9.00598968278818,16.7035766947655,2.42583590974852));
#87579=CARTESIAN_POINT('Ctrl Pts',(-9.01133274247707,16.7039812202781,2.4209161047594));
#87580=CARTESIAN_POINT('Ctrl Pts',(-9.02378380351619,16.7049236230549,2.40962146572087));
#87581=CARTESIAN_POINT('Ctrl Pts',(-9.03091795075709,16.7054633935459,2.40327606803278));
#87582=CARTESIAN_POINT('Ctrl Pts',(-9.06175229133653,16.7077935235339,2.37638652533085));
#87583=CARTESIAN_POINT('Ctrl Pts',(-9.08604630846293,16.709622277208,2.35653840758735));
#87584=CARTESIAN_POINT('Ctrl Pts',(-9.16668436619694,16.7156214222931,2.29486969796859));
#87585=CARTESIAN_POINT('Ctrl Pts',(-9.22540234026355,16.7198782159552,2.25631507270421));
#87586=CARTESIAN_POINT('Ctrl Pts',(-9.37244114266306,16.7299820050387,2.17423456077122));
#87587=CARTESIAN_POINT('Ctrl Pts',(-9.4628400781496,16.735743835191,2.13510103251226));
#87588=CARTESIAN_POINT('Ctrl Pts',(-9.56663521271319,16.7417792056597,2.10209424952478));
#87589=CARTESIAN_POINT('Ctrl Pts',(-9.57681291714972,16.7423653826097,2.0989795763813));
#87590=CARTESIAN_POINT('Ctrl Pts',(-9.59321208410454,16.7433010344993,2.09415596585986));
#87591=CARTESIAN_POINT('Ctrl Pts',(-9.59941231513204,16.7436527723339,2.09237669618511));
#87592=CARTESIAN_POINT('Ctrl Pts',(-9.61046115101857,16.744276045692,2.08928494605108));
#87593=CARTESIAN_POINT('Ctrl Pts',(-9.61530510159173,16.7445480974814,2.08795633413268));
#87594=CARTESIAN_POINT('Ctrl Pts',(-9.62543513290881,16.745114566219,2.08523383755892));
#87595=CARTESIAN_POINT('Ctrl Pts',(-9.63072238379831,16.7454088309738,2.08384457867999));
#87596=CARTESIAN_POINT('Ctrl Pts',(-9.64453428630998,16.7461739642978,2.08029802515142));
#87597=CARTESIAN_POINT('Ctrl Pts',(-9.65307088599521,16.746643321243,2.07818785861079));
#87598=CARTESIAN_POINT('Ctrl Pts',(-9.69105792969666,16.7487167411341,2.06916031618848));
#87599=CARTESIAN_POINT('Ctrl Pts',(-9.72070072987075,16.7502941484425,2.06307985964075));
#87600=CARTESIAN_POINT('Ctrl Pts',(-9.80176894720044,16.7545163770963,2.04905458620525));
#87601=CARTESIAN_POINT('Ctrl Pts',(-9.85346440375555,16.7571084503633,2.04292552629819));
#87602=CARTESIAN_POINT('Ctrl Pts',(-10.0111817393311,16.7648710809417,2.032707118987));
#87603=CARTESIAN_POINT('Ctrl Pts',(-10.1174058516349,16.7698851706157,2.03737030296771));
#87604=CARTESIAN_POINT('Ctrl Pts',(-10.2501813310216,16.7767431854769,2.05776427657442));
#87605=CARTESIAN_POINT('Ctrl Pts',(-10.2780459094226,16.778217607675,2.06287619026194));
#87606=CARTESIAN_POINT('Ctrl Pts',(-10.3111430660749,16.7800295247208,2.06994659648807));
#87607=CARTESIAN_POINT('Ctrl Pts',(-10.3165367368317,16.7803267447539,2.07113078388423));
#87608=CARTESIAN_POINT('Ctrl Pts',(-10.3253432169485,16.7808153949202,2.07311656736173));
#87609=CARTESIAN_POINT('Ctrl Pts',(-10.3287601252649,16.7810058217434,2.07389996190164));
#87610=CARTESIAN_POINT('Ctrl Pts',(-10.3348874431459,16.7813488470887,2.07532796326748));
#87611=CARTESIAN_POINT('Ctrl Pts',(-10.3375988562978,16.7815011869912,2.07596803973086));
#87612=CARTESIAN_POINT('Ctrl Pts',(-10.3435056361329,16.7818342614672,2.07738025665292));
#87613=CARTESIAN_POINT('Ctrl Pts',(-10.3467001928995,16.7820151619234,2.07815541214193));
#87614=CARTESIAN_POINT('Ctrl Pts',(-10.3557322528661,16.7825287369463,2.08037927964959));
#87615=CARTESIAN_POINT('Ctrl Pts',(-10.3615634046876,16.7828628024721,2.08185320674961));
#87616=CARTESIAN_POINT('Ctrl Pts',(-10.3982377228345,16.7849788992025,2.09136418368387));
#87617=CARTESIAN_POINT('Ctrl Pts',(-10.4288184432168,16.7868103938086,2.10037055271427));
#87618=CARTESIAN_POINT('Ctrl Pts',(-10.5378047993339,16.7935220462815,2.1363752297819));
#87619=CARTESIAN_POINT('Ctrl Pts',(-10.6141762955048,16.7985662315793,2.16902539349438));
#87620=CARTESIAN_POINT('Ctrl Pts',(-10.7726139081881,16.8093281580329,2.25331516186067));
#87621=CARTESIAN_POINT('Ctrl Pts',(-10.853171809803,16.8149852562567,2.30699590570295));
#87622=CARTESIAN_POINT('Ctrl Pts',(-10.9361127509703,16.8209286447559,2.37499380210717));
#87623=CARTESIAN_POINT('Ctrl Pts',(-10.9442875758992,16.8215161397155,2.3818466069894));
#87624=CARTESIAN_POINT('Ctrl Pts',(-10.9572897892086,16.8224534801286,2.39299042210945));
#87625=CARTESIAN_POINT('Ctrl Pts',(-10.962164862265,16.8228056014878,2.39722498860482));
#87626=CARTESIAN_POINT('Ctrl Pts',(-10.9707826746308,16.8234293141669,2.40481120940784));
#87627=CARTESIAN_POINT('Ctrl Pts',(-10.974536459162,16.823701424263,2.40815011148967));
#87628=CARTESIAN_POINT('Ctrl Pts',(-10.9784375559301,16.8239846818701,2.41165619030982));
#87629=CARTESIAN_POINT('Ctrl Pts',(-10.9786020687069,16.8239966279747,2.41180411227211));
#87630=CARTESIAN_POINT('Ctrl Pts',(-10.978883013027,16.8240170302606,2.41205683910078));
#87631=CARTESIAN_POINT('Ctrl Pts',(-10.9789994614962,16.8240254872336,2.41216162554785));
#87632=CARTESIAN_POINT('Ctrl Pts',(-10.9791991379893,16.8240399893278,2.41234136297016));
#87633=CARTESIAN_POINT('Ctrl Pts',(-10.979282374201,16.8240460348283,2.4124163047729));
#87634=CARTESIAN_POINT('Ctrl Pts',(-10.9794255190017,16.8240564319165,2.41254521508711));
#87635=CARTESIAN_POINT('Ctrl Pts',(-10.9794854317386,16.8240607836968,2.4125991789991));
#87636=CARTESIAN_POINT('Ctrl Pts',(-10.9796288689124,16.8240712025807,2.41272839555485));
#87637=CARTESIAN_POINT('Ctrl Pts',(-10.9797123891492,16.8240772694894,2.41280365288192));
#87638=CARTESIAN_POINT('Ctrl Pts',(-10.9798739720527,16.8240890073094,2.4129492836395));
#87639=CARTESIAN_POINT('Ctrl Pts',(-10.9799520358144,16.8240946782714,2.41301965585873));
#87640=CARTESIAN_POINT('Ctrl Pts',(-10.9801031638922,16.8241056573949,2.41315592295441));
#87641=CARTESIAN_POINT('Ctrl Pts',(-10.9801762291377,16.8241109655992,2.41322181678415));
#87642=CARTESIAN_POINT('Ctrl Pts',(-10.9803177700751,16.8241212489141,2.41334949124347));
#87643=CARTESIAN_POINT('Ctrl Pts',(-10.9803862465808,16.8241262240627,2.41341127098571));
#87644=CARTESIAN_POINT('Ctrl Pts',(-10.9805189777553,16.8241358679206,2.41353104427522));
#87645=CARTESIAN_POINT('Ctrl Pts',(-10.9805832331218,16.8241405366624,2.41358903705255));
#87646=CARTESIAN_POINT('Ctrl Pts',(-10.9807078527477,16.824149591684,2.41370153080602));
#87647=CARTESIAN_POINT('Ctrl Pts',(-10.980768217595,16.8241539779905,2.41375603110089));
#87648=CARTESIAN_POINT('Ctrl Pts',(-10.9808853543462,16.8241624897608,2.41386180553246));
#87649=CARTESIAN_POINT('Ctrl Pts',(-10.9809421267811,16.8241666152493,2.4139130790962));
#87650=CARTESIAN_POINT('Ctrl Pts',(-10.9810523481726,16.8241746249244,2.4140126403436));
#87651=CARTESIAN_POINT('Ctrl Pts',(-10.9811057975903,16.8241785091325,2.41406092752715));
#87652=CARTESIAN_POINT('Ctrl Pts',(-10.9812096170324,16.8241860539494,2.41415473383529));
#87653=CARTESIAN_POINT('Ctrl Pts',(-10.9812599874718,16.8241897145779,2.41420025253456));
#87654=CARTESIAN_POINT('Ctrl Pts',(-10.9813578705746,16.8241968283109,2.41428871979553));
#87655=CARTESIAN_POINT('Ctrl Pts',(-10.9814053835613,16.8242002814296,2.41433166794877));
#87656=CARTESIAN_POINT('Ctrl Pts',(-10.9814977533478,16.8242069947669,2.41441517428151));
#87657=CARTESIAN_POINT('Ctrl Pts',(-10.9815426104624,16.8242102550004,2.41445573213073));
#87658=CARTESIAN_POINT('Ctrl Pts',(-10.9816298522714,16.8242165958999,2.41453462220327));
#87659=CARTESIAN_POINT('Ctrl Pts',(-10.9816722372521,16.8242196765796,2.41457295414467));
#87660=CARTESIAN_POINT('Ctrl Pts',(-10.9817547027085,16.8242256705554,2.41464754267074));
#87661=CARTESIAN_POINT('Ctrl Pts',(-10.9817947833755,16.8242285838591,2.41468379895186));
#87662=CARTESIAN_POINT('Ctrl Pts',(-10.9818727938503,16.8242342542325,2.4147543737416));
#87663=CARTESIAN_POINT('Ctrl Pts',(-10.9819107238404,16.8242370113098,2.41478869199417));
#87664=CARTESIAN_POINT('Ctrl Pts',(-10.981984573807,16.824242379452,2.41485551692321));
#87665=CARTESIAN_POINT('Ctrl Pts',(-10.9820204939596,16.8242449905248,2.41488802338639));
#87666=CARTESIAN_POINT('Ctrl Pts',(-10.9864840609031,16.8245694570916,2.41892779620237));
#87667=CARTESIAN_POINT('Ctrl Pts',(-10.9908871843587,16.8248901779442,2.4229621633576));
#87668=CARTESIAN_POINT('Ctrl Pts',(-11.0034563171722,16.8258076715597,2.43462096823811));
#87669=CARTESIAN_POINT('Ctrl Pts',(-11.0115599786645,16.8264016112962,2.44231220080105));
#87670=CARTESIAN_POINT('Ctrl Pts',(-11.0297128920729,16.8277381782892,2.45994071603958));
#87671=CARTESIAN_POINT('Ctrl Pts',(-11.0397079374658,16.8284784413074,2.46993234363439));
#87672=CARTESIAN_POINT('Ctrl Pts',(-11.0713776113711,16.8308402135887,2.50252187509461));
#87673=CARTESIAN_POINT('Ctrl Pts',(-11.0924728774062,16.8324383234404,2.52567163089498));
#87674=CARTESIAN_POINT('Ctrl Pts',(-11.148578632239,16.8367851899325,2.59135688103372));
#87675=CARTESIAN_POINT('Ctrl Pts',(-11.1819560770153,16.8394819065812,2.63521941757095));
#87676=CARTESIAN_POINT('Ctrl Pts',(-11.271384801929,16.8472598936627,2.76762371280278));
#87677=CARTESIAN_POINT('Ctrl Pts',(-11.3204992235894,16.8522661009677,2.86041389248033));
#87678=CARTESIAN_POINT('Ctrl Pts',(-11.3631790047849,16.8583530634548,2.9673787933051));
#87679=CARTESIAN_POINT('Ctrl Pts',(-11.3669625602156,16.8589129074277,2.9771657094962));
#87680=CARTESIAN_POINT('Ctrl Pts',(-11.3721255049102,16.8597071562594,2.99095992575757));
#87681=CARTESIAN_POINT('Ctrl Pts',(-11.3735933111791,16.8599365785517,2.99493405085427));
#87682=CARTESIAN_POINT('Ctrl Pts',(-11.3759371798355,16.8603089344008,3.00136593073956));
#87683=CARTESIAN_POINT('Ctrl Pts',(-11.3768239722316,16.860451239458,3.00381978359858));
#87684=CARTESIAN_POINT('Ctrl Pts',(-11.3786806437567,16.8607522380591,3.00900070251351));
#87685=CARTESIAN_POINT('Ctrl Pts',(-11.37964899918,16.8609110225285,3.01172828645264));
#87686=CARTESIAN_POINT('Ctrl Pts',(-11.3820095406738,16.8613025117397,3.01844035267416));
#87687=CARTESIAN_POINT('Ctrl Pts',(-11.383392587008,16.8615357446942,3.02242800150299));
#87688=CARTESIAN_POINT('Ctrl Pts',(-11.3883800039903,16.8623909267684,3.0370113655561));
#87689=CARTESIAN_POINT('Ctrl Pts',(-11.3918799531538,16.8630185848786,3.04764207589597));
#87690=CARTESIAN_POINT('Ctrl Pts',(-11.4139463028609,16.8671570758978,3.11734786036031));
#87691=CARTESIAN_POINT('Ctrl Pts',(-11.428867689185,16.8708333387061,3.1775057498141));
#87692=CARTESIAN_POINT('Ctrl Pts',(-11.4555460369151,16.8797916031711,3.32436425349679));
#87693=CARTESIAN_POINT('Ctrl Pts',(-11.4634335076646,16.885086436231,3.41153702785937));
#87694=CARTESIAN_POINT('Ctrl Pts',(-11.4634995813664,16.8901969352951,3.49889304900151));
#87695=CARTESIAN_POINT('Ctrl Pts',(-11.4634995826939,16.890197038059,3.49889480559032));
#87696=CARTESIAN_POINT('Ctrl Pts',(-11.4634998608992,16.890218590156,3.49926320529145));
#87697=CARTESIAN_POINT('Ctrl Pts',(-11.4635,16.8902401389654,3.49963160344776));
#87698=CARTESIAN_POINT('Ctrl Pts',(-11.4635,16.8902616844768,3.4999999999813));
#87699=CARTESIAN_POINT('Origin',(-10.,13.2,3.5));
#87700=CARTESIAN_POINT('',(-11.4635,17.4596976889334,3.50000000000126));
#87701=CARTESIAN_POINT('',(-11.4635,17.3900944100234,3.49999999998336));
#87702=CARTESIAN_POINT('',(-11.4635,13.2,3.5));
#87703=CARTESIAN_POINT('Ctrl Pts',(-11.4635,17.4596976889334,3.50000000000147));
#87704=CARTESIAN_POINT('Ctrl Pts',(-11.4635,17.4588719371887,3.48584184115301));
#87705=CARTESIAN_POINT('Ctrl Pts',(-11.4632945474571,17.4580511124813,3.47168412291088));
#87706=CARTESIAN_POINT('Ctrl Pts',(-11.4617357048981,17.4549574656788,3.4179879946723));
#87707=CARTESIAN_POINT('Ctrl Pts',(-11.4589848080041,17.4527234553376,3.37850518135659));
#87708=CARTESIAN_POINT('Ctrl Pts',(-11.4535468662214,17.449990889183,3.32931846457098));
#87709=CARTESIAN_POINT('Ctrl Pts',(-11.4523563944236,17.449446188232,3.31946859212755));
#87710=CARTESIAN_POINT('Ctrl Pts',(-11.4503149758051,17.4485895184532,3.30390807950675));
#87711=CARTESIAN_POINT('Ctrl Pts',(-11.4495302569239,17.4482754901577,3.29818918284064));
#87712=CARTESIAN_POINT('Ctrl Pts',(-11.4480068193935,17.4476930029131,3.28755421347788));
#87713=CARTESIAN_POINT('Ctrl Pts',(-11.4472768509405,17.4474242743337,3.28263698843374));
#87714=CARTESIAN_POINT('Ctrl Pts',(-11.4456015620945,17.4468297329295,3.27173461105017));
#87715=CARTESIAN_POINT('Ctrl Pts',(-11.4446440941169,17.4465043060991,3.26575139922252));
#87716=CARTESIAN_POINT('Ctrl Pts',(-11.4417563026737,17.4455627940984,3.24839706262894));
#87717=CARTESIAN_POINT('Ctrl Pts',(-11.439728659212,17.444949769973,3.237042451386));
#87718=CARTESIAN_POINT('Ctrl Pts',(-11.4212560322287,17.439745904489,3.14022555393402));
#87719=CARTESIAN_POINT('Ctrl Pts',(-11.3973518866666,17.4354076449411,3.05635982505373));
#87720=CARTESIAN_POINT('Ctrl Pts',(-11.3368870788253,17.4271664335753,2.89898877971933));
#87721=CARTESIAN_POINT('Ctrl Pts',(-11.3013321761466,17.4232639563814,2.82545208426932));
#87722=CARTESIAN_POINT('Ctrl Pts',(-11.2528409195864,17.4184884305442,2.74342145455409));
#87723=CARTESIAN_POINT('Ctrl Pts',(-11.2456746272575,17.4177938767176,2.73167964255244));
#87724=CARTESIAN_POINT('Ctrl Pts',(-11.2227759201119,17.4156033675284,2.69532327946387));
#87725=CARTESIAN_POINT('Ctrl Pts',(-11.2064722390614,17.4140844559099,2.67107896315827));
#87726=CARTESIAN_POINT('Ctrl Pts',(-11.1862038979949,17.4122223715673,2.64280474480666));
#87727=CARTESIAN_POINT('Ctrl Pts',(-11.1829266803051,17.4119220561996,2.63828783217934));
#87728=CARTESIAN_POINT('Ctrl Pts',(-11.1775387254835,17.4114293667268,2.63095039852335));
#87729=CARTESIAN_POINT('Ctrl Pts',(-11.1754434660505,17.4112380244696,2.62811851870324));
#87730=CARTESIAN_POINT('Ctrl Pts',(-11.1716727526436,17.4108940762779,2.62306045033981));
#87731=CARTESIAN_POINT('Ctrl Pts',(-11.170001146857,17.4107417357631,2.62083145573305));
#87732=CARTESIAN_POINT('Ctrl Pts',(-11.1663526868104,17.4104095193109,2.61599526867111));
#87733=CARTESIAN_POINT('Ctrl Pts',(-11.1643734780443,17.4102294834094,2.61338996270255));
#87734=CARTESIAN_POINT('Ctrl Pts',(-11.1587726500321,17.4097205816032,2.6060684846663));
#87735=CARTESIAN_POINT('Ctrl Pts',(-11.1551310428714,17.4093903631586,2.60136777273101));
#87736=CARTESIAN_POINT('Ctrl Pts',(-11.1325838526483,17.4073505385665,2.57262659433001));
#87737=CARTESIAN_POINT('Ctrl Pts',(-11.1129583976579,17.4055953987589,2.54916302460806));
#87738=CARTESIAN_POINT('Ctrl Pts',(-10.9923092576155,17.3950075509727,2.41377489206962));
#87739=CARTESIAN_POINT('Ctrl Pts',(-10.8752091535502,17.3856502841544,2.31738195737113));
#87740=CARTESIAN_POINT('Ctrl Pts',(-10.7159445468671,17.3750557738834,2.22311735372003));
#87741=CARTESIAN_POINT('Ctrl Pts',(-10.685857934446,17.3731288013647,2.20670766809175));
#87742=CARTESIAN_POINT('Ctrl Pts',(-10.6466688701293,17.3707111786293,2.18708602686426));
#87743=CARTESIAN_POINT('Ctrl Pts',(-10.6380746363782,17.3701864857458,2.18288782066128));
#87744=CARTESIAN_POINT('Ctrl Pts',(-10.6243518940195,17.3693572509917,2.17635022625761));
#87745=CARTESIAN_POINT('Ctrl Pts',(-10.6192500629466,17.3690508198836,2.17395574286725));
#87746=CARTESIAN_POINT('Ctrl Pts',(-10.6100626227117,17.3685022901652,2.16970831394235));
#87747=CARTESIAN_POINT('Ctrl Pts',(-10.6059821036659,17.3682598248807,2.16784457953252));
#87748=CARTESIAN_POINT('Ctrl Pts',(-10.5964126946358,17.3676938870697,2.16352691901005));
#87749=CARTESIAN_POINT('Ctrl Pts',(-10.5909171009728,17.367370927685,2.16108798654001));
#87750=CARTESIAN_POINT('Ctrl Pts',(-10.5750410937572,17.3664437412566,2.15415903627054));
#87751=CARTESIAN_POINT('Ctrl Pts',(-10.5646233332933,17.3658424310925,2.14975533319732));
#87752=CARTESIAN_POINT('Ctrl Pts',(-10.4831436430933,17.361192415147,2.11642089267606));
#87753=CARTESIAN_POINT('Ctrl Pts',(-10.4099537300422,17.357336072496,2.09299650642095));
#87754=CARTESIAN_POINT('Ctrl Pts',(-10.240214844078,17.3487666817711,2.05305067782795));
#87755=CARTESIAN_POINT('Ctrl Pts',(-10.1431799978249,17.3441320348349,2.04025250242193));
#87756=CARTESIAN_POINT('Ctrl Pts',(-10.0087459137742,17.3373492062003,2.03606170318592));
#87757=CARTESIAN_POINT('Ctrl Pts',(-9.97186391986774,17.3354489564038,2.03630612429924));
#87758=CARTESIAN_POINT('Ctrl Pts',(-9.92908098177803,17.3331598033239,2.03820718072639));
#87759=CARTESIAN_POINT('Ctrl Pts',(-9.92313013547809,17.3328394820369,2.03850803110607));
#87760=CARTESIAN_POINT('Ctrl Pts',(-9.91358942151782,17.3323226230293,2.03904880107409));
#87761=CARTESIAN_POINT('Ctrl Pts',(-9.9099982511157,17.3321273237122,2.03926563730749));
#87762=CARTESIAN_POINT('Ctrl Pts',(-9.90361478882863,17.3317787781931,2.03967470237341));
#87763=CARTESIAN_POINT('Ctrl Pts',(-9.90082220755039,17.3316258235908,2.03986170202779));
#87764=CARTESIAN_POINT('Ctrl Pts',(-9.89485727500514,17.3312980782213,2.04027832327276));
#87765=CARTESIAN_POINT('Ctrl Pts',(-9.89168518077645,17.3311231654501,2.0405102721618));
#87766=CARTESIAN_POINT('Ctrl Pts',(-9.883001255395,17.3306426710013,2.04117372165756));
#87767=CARTESIAN_POINT('Ctrl Pts',(-9.87749113210737,17.3303359629823,2.04162611381486));
#87768=CARTESIAN_POINT('Ctrl Pts',(-9.84822082163298,17.3286974769836,2.04419631684733));
#87769=CARTESIAN_POINT('Ctrl Pts',(-9.82451378207117,17.327338122719,2.04686348366081));
#87770=CARTESIAN_POINT('Ctrl Pts',(-9.75184869707101,17.3230934662459,2.05684270121569));
#87771=CARTESIAN_POINT('Ctrl Pts',(-9.70318939514233,17.3201423387567,2.06605964751645));
#87772=CARTESIAN_POINT('Ctrl Pts',(-9.53475145373394,17.3097308080808,2.10690632475298));
#87773=CARTESIAN_POINT('Ctrl Pts',(-9.41857560594761,17.3022497347082,2.15125173290631));
#87774=CARTESIAN_POINT('Ctrl Pts',(-9.28998635481199,17.2940309858853,2.22007968992839));
#87775=CARTESIAN_POINT('Ctrl Pts',(-9.27084304642886,17.2928072528494,2.23088787441236));
#87776=CARTESIAN_POINT('Ctrl Pts',(-9.24499743085002,17.2911540794358,2.2462580813855));
#87777=CARTESIAN_POINT('Ctrl Pts',(-9.23807945970624,17.2907114747922,2.25045017231042));
#87778=CARTESIAN_POINT('Ctrl Pts',(-9.22712872176797,17.290010600403,2.25721076174272));
#87779=CARTESIAN_POINT('Ctrl Pts',(-9.2230732395625,17.289750982392,2.25974199735861));
#87780=CARTESIAN_POINT('Ctrl Pts',(-9.21477948163198,17.2892198994985,2.26497520271294));
#87781=CARTESIAN_POINT('Ctrl Pts',(-9.21054257357367,17.2889485147359,2.26767922799648));
#87782=CARTESIAN_POINT('Ctrl Pts',(-9.20077963473035,17.2883229507987,2.27398102094854));
#87783=CARTESIAN_POINT('Ctrl Pts',(-9.19526379724946,17.2879693552617,2.27759443097687));
#87784=CARTESIAN_POINT('Ctrl Pts',(-9.17791282614335,17.2868563908497,2.28912934509186));
#87785=CARTESIAN_POINT('Ctrl Pts',(-9.16616859921466,17.2861020796294,2.29718651559571));
#87786=CARTESIAN_POINT('Ctrl Pts',(-9.10871167666106,17.2824040253735,2.33785108524658));
#87787=CARTESIAN_POINT('Ctrl Pts',(-9.0647820844768,17.2795546378667,2.37290049232021));
#87788=CARTESIAN_POINT('Ctrl Pts',(-8.95427107604367,17.272181957524,2.47199321365247));
#87789=CARTESIAN_POINT('Ctrl Pts',(-8.89155268798925,17.2677865891433,2.53995264471238));
#87790=CARTESIAN_POINT('Ctrl Pts',(-8.80100736605511,17.2604078516403,2.6588585628784));
#87791=CARTESIAN_POINT('Ctrl Pts',(-8.76906314919216,17.2575252796585,2.70634052589192));
#87792=CARTESIAN_POINT('Ctrl Pts',(-8.73631900626414,17.2540906028738,2.76176261325652));
#87793=CARTESIAN_POINT('Ctrl Pts',(-8.73270235508965,17.2537037971662,2.76798854648252));
#87794=CARTESIAN_POINT('Ctrl Pts',(-8.72738006167122,17.2531229609349,2.77730834974984));
#87795=CARTESIAN_POINT('Ctrl Pts',(-8.72563938765842,17.2529310973758,2.78038221398421));
#87796=CARTESIAN_POINT('Ctrl Pts',(-8.72254539080068,17.2525865925548,2.78589234823257));
#87797=CARTESIAN_POINT('Ctrl Pts',(-8.72118788173025,17.2524342204151,2.78832621034666));
#87798=CARTESIAN_POINT('Ctrl Pts',(-8.71825528267471,17.2521023820623,2.79361951713532));
#87799=CARTESIAN_POINT('Ctrl Pts',(-8.71668282709452,17.2519227588881,2.79648031991992));
#87800=CARTESIAN_POINT('Ctrl Pts',(-8.71228943145303,17.2514161645559,2.80453706259117));
#87801=CARTESIAN_POINT('Ctrl Pts',(-8.7094904204342,17.2510878599189,2.80974480931377));
#87802=CARTESIAN_POINT('Ctrl Pts',(-8.69270201478475,17.2490852816903,2.84143982206972));
#87803=CARTESIAN_POINT('Ctrl Pts',(-8.67949788894564,17.2473673360417,2.86833280008957));
#87804=CARTESIAN_POINT('Ctrl Pts',(-8.60895715249976,17.2374021561013,3.02389738295745));
#87805=CARTESIAN_POINT('Ctrl Pts',(-8.56960624630163,17.2286736701308,3.15991650228304));
#87806=CARTESIAN_POINT('Ctrl Pts',(-8.54435426268167,17.2180163853223,3.34248124600827));
#87807=CARTESIAN_POINT('Ctrl Pts',(-8.54032226325154,17.2155582110068,3.38572783271756));
#87808=CARTESIAN_POINT('Ctrl Pts',(-8.53772415869821,17.2125953871458,3.4392890782443));
#87809=CARTESIAN_POINT('Ctrl Pts',(-8.53733626225622,17.2120346931571,3.44949010209176));
#87810=CARTESIAN_POINT('Ctrl Pts',(-8.53689434022903,17.2111585446041,3.46553029840875));
#87811=CARTESIAN_POINT('Ctrl Pts',(-8.53676847821691,17.210840872091,3.47136702911846));
#87812=CARTESIAN_POINT('Ctrl Pts',(-8.53660789717808,17.2102818071517,3.48167524696837));
#87813=CARTESIAN_POINT('Ctrl Pts',(-8.53655873990505,17.2100399701515,3.48614640689652));
#87814=CARTESIAN_POINT('Ctrl Pts',(-8.53649301699805,17.2094869526471,3.49639805930451));
#87815=CARTESIAN_POINT('Ctrl Pts',(-8.53649020558537,17.2091762024518,3.5021785864081));
#87816=CARTESIAN_POINT('Ctrl Pts',(-8.53657725138206,17.2083186661712,3.51818424825574));
#87817=CARTESIAN_POINT('Ctrl Pts',(-8.53674002402275,17.2077741435633,3.52840876386831));
#87818=CARTESIAN_POINT('Ctrl Pts',(-8.53830768351442,17.2046302898279,3.58777754786572));
#87819=CARTESIAN_POINT('Ctrl Pts',(-8.54208111514923,17.2021055854962,3.63683019445787));
#87820=CARTESIAN_POINT('Ctrl Pts',(-8.56430267392771,17.1933033964237,3.81063429632922));
#87821=CARTESIAN_POINT('Ctrl Pts',(-8.59637155545103,17.1874121537591,3.93306316566266));
#87822=CARTESIAN_POINT('Ctrl Pts',(-8.65796316384873,17.1791560648551,4.08498345037961));
#87823=CARTESIAN_POINT('Ctrl Pts',(-8.67355983529974,17.1772052307554,4.11953574262304));
#87824=CARTESIAN_POINT('Ctrl Pts',(-8.69315747562584,17.1748593711467,4.15881019524725));
#87825=CARTESIAN_POINT('Ctrl Pts',(-8.69586963399928,17.174536823591,4.16416281353827));
#87826=CARTESIAN_POINT('Ctrl Pts',(-8.70026607206328,17.1740170569888,4.17270870316964));
#87827=CARTESIAN_POINT('Ctrl Pts',(-8.70192941258629,17.1738210986347,4.1759127401315));
#87828=CARTESIAN_POINT('Ctrl Pts',(-8.70490404535399,17.1734718145413,4.18159119747568));
#87829=CARTESIAN_POINT('Ctrl Pts',(-8.70621060448901,17.1733187849594,4.18406804645771));
#87830=CARTESIAN_POINT('Ctrl Pts',(-8.7090128036779,17.1729913834971,4.18934343929973));
#87831=CARTESIAN_POINT('Ctrl Pts',(-8.71051041474702,17.1728168928174,4.19214082924066));
#87832=CARTESIAN_POINT('Ctrl Pts',(-8.71462619802512,17.1723387187295,4.19976898363119));
#87833=CARTESIAN_POINT('Ctrl Pts',(-8.71726246976421,17.1720339266524,4.20458985787021));
#87834=CARTESIAN_POINT('Ctrl Pts',(-8.73126238782974,17.1704235518174,4.22985211183068));
#87835=CARTESIAN_POINT('Ctrl Pts',(-8.74308708315786,17.1690914772971,4.25003268284968));
#87836=CARTESIAN_POINT('Ctrl Pts',(-8.78061491428403,17.1649660644128,4.31069811705124));
#87837=CARTESIAN_POINT('Ctrl Pts',(-8.80782773898504,17.162110727891,4.35020948480728));
#87838=CARTESIAN_POINT('Ctrl Pts',(-8.89694144030263,17.1532969468388,4.46688658068318));
#87839=CARTESIAN_POINT('Ctrl Pts',(-8.96476965324224,17.147305422279,4.53918703624663));
#87840=CARTESIAN_POINT('Ctrl Pts',(-9.07293359322012,17.1390057685644,4.63329556498269));
#87841=CARTESIAN_POINT('Ctrl Pts',(-9.10780825204643,17.1364849441852,4.66095023107085));
#87842=CARTESIAN_POINT('Ctrl Pts',(-9.15148991167338,17.1335087445268,4.69245572290251));
#87843=CARTESIAN_POINT('Ctrl Pts',(-9.15914092484352,17.1329938202377,4.69786311511011));
#87844=CARTESIAN_POINT('Ctrl Pts',(-9.17188525710374,17.1321464540739,4.70668795916275));
#87845=CARTESIAN_POINT('Ctrl Pts',(-9.1769489982348,17.1318124283438,4.71014747377519));
#87846=CARTESIAN_POINT('Ctrl Pts',(-9.18616003279409,17.1312095803267,4.71635583248166));
#87847=CARTESIAN_POINT('Ctrl Pts',(-9.19029986374403,17.1309403535939,4.71911553744044));
#87848=CARTESIAN_POINT('Ctrl Pts',(-9.19922522766028,17.1303635534775,4.72499986819879));
#87849=CARTESIAN_POINT('Ctrl Pts',(-9.20401516365908,17.1300562358402,4.72811768763778));
#87850=CARTESIAN_POINT('Ctrl Pts',(-9.21717399626281,17.1292179836665,4.7365735837972));
#87851=CARTESIAN_POINT('Ctrl Pts',(-9.22557921600713,17.1286891452882,4.74185475644286));
#87852=CARTESIAN_POINT('Ctrl Pts',(-9.27173319756821,17.1258200506561,4.77020342660559));
#87853=CARTESIAN_POINT('Ctrl Pts',(-9.31046106934512,17.1235394953266,4.79163688108015));
#87854=CARTESIAN_POINT('Ctrl Pts',(-9.43809348435907,17.1163472351902,4.85489387143371));
#87855=CARTESIAN_POINT('Ctrl Pts',(-9.53024751009269,17.1116542407632,4.88953564061091));
#87856=CARTESIAN_POINT('Ctrl Pts',(-9.69300105913799,17.103411975441,4.93265723552733));
#87857=CARTESIAN_POINT('Ctrl Pts',(-9.76202090600701,17.0999224390044,4.94572430051905));
#87858=CARTESIAN_POINT('Ctrl Pts',(-9.83891811822245,17.0957928662048,4.95462629041437));
#87859=CARTESIAN_POINT('Ctrl Pts',(-9.84614001542342,17.0954026816337,4.95540788722569));
#87860=CARTESIAN_POINT('Ctrl Pts',(-9.85689465785521,17.0948177446156,4.95649087865386));
#87861=CARTESIAN_POINT('Ctrl Pts',(-9.86042327484176,17.0946252042526,4.95683326287034));
#87862=CARTESIAN_POINT('Ctrl Pts',(-9.86672885274059,17.094279973561,4.95742197852261));
#87863=CARTESIAN_POINT('Ctrl Pts',(-9.86950530737975,17.0941275571565,4.95767319973102));
#87864=CARTESIAN_POINT('Ctrl Pts',(-9.87552523888234,17.093796195244,4.95820056229092));
#87865=CARTESIAN_POINT('Ctrl Pts',(-9.87876887914131,17.0936170966035,4.95847381221962));
#87866=CARTESIAN_POINT('Ctrl Pts',(-9.8878635091424,17.0931134296229,4.95920941109442));
#87867=CARTESIAN_POINT('Ctrl Pts',(-9.89371633997681,17.0927875518086,4.95964738181367));
#87868=CARTESIAN_POINT('Ctrl Pts',(-9.92868329617756,17.0908308720101,4.96205255773235));
#87869=CARTESIAN_POINT('Ctrl Pts',(-9.95784648607544,17.0891586370505,4.96318372025525));
#87870=CARTESIAN_POINT('Ctrl Pts',(-10.1177500595326,17.0798383367533,4.9646017841344));
#87871=CARTESIAN_POINT('Ctrl Pts',(-10.2480475836458,17.0717550698591,4.94824077043991));
#87872=CARTESIAN_POINT('Ctrl Pts',(-10.38789059818,17.0633100862285,4.91122870207017));
#87873=CARTESIAN_POINT('Ctrl Pts',(-10.4012804875305,17.0625030973958,4.90747985847637));
#87874=CARTESIAN_POINT('Ctrl Pts',(-10.4537320255814,17.0593492265492,4.89198532720959));
#87875=CARTESIAN_POINT('Ctrl Pts',(-10.4923510385893,17.0570438384852,4.8787990490063));
#87876=CARTESIAN_POINT('Ctrl Pts',(-10.5397055721509,17.0542377249167,4.86038613694877));
#87877=CARTESIAN_POINT('Ctrl Pts',(-10.5490022521349,17.0536878017002,4.85666100422027));
#87878=CARTESIAN_POINT('Ctrl Pts',(-10.563615887336,17.0528247679377,4.85063057503489));
#87879=CARTESIAN_POINT('Ctrl Pts',(-10.5689585275346,17.0525095467221,4.84838867318386));
#87880=CARTESIAN_POINT('Ctrl Pts',(-10.578859026172,17.0519259191515,4.84416486249757));
#87881=CARTESIAN_POINT('Ctrl Pts',(-10.5834203591988,17.0516572349134,4.84219135560843));
#87882=CARTESIAN_POINT('Ctrl Pts',(-10.5933865100063,17.0510705905544,4.83781899551509));
#87883=CARTESIAN_POINT('Ctrl Pts',(-10.5987870354664,17.0507529610569,4.8354105370934));
#87884=CARTESIAN_POINT('Ctrl Pts',(-10.614171316581,17.0498488102283,4.82843755980087));
#87885=CARTESIAN_POINT('Ctrl Pts',(-10.6241186312251,17.049265007791,4.82379329931589));
#87886=CARTESIAN_POINT('Ctrl Pts',(-10.6464347007082,17.0479565860162,4.8130667831795));
#87887=CARTESIAN_POINT('Ctrl Pts',(-10.6587717597692,17.0472341614664,4.80692080262556));
#87888=CARTESIAN_POINT('Ctrl Pts',(-10.7583526944973,17.0414056960573,4.755543919716));
#87889=CARTESIAN_POINT('Ctrl Pts',(-10.8409262174507,17.0366127041982,4.70180478580885));
#87890=CARTESIAN_POINT('Ctrl Pts',(-10.9897659684842,17.0273246723573,4.58203531155994));
#87891=CARTESIAN_POINT('Ctrl Pts',(-11.0563342554216,17.0228408600507,4.51714838519754));
#87892=CARTESIAN_POINT('Ctrl Pts',(-11.1234752021129,17.0173613556811,4.43795447626451));
#87893=CARTESIAN_POINT('Ctrl Pts',(-11.1305471517439,17.0167705152673,4.4294182332478));
#87894=CARTESIAN_POINT('Ctrl Pts',(-11.1402483058166,17.0159394243218,4.41743383277184));
#87895=CARTESIAN_POINT('Ctrl Pts',(-11.1429603594425,17.0157047897291,4.41405287166858));
#87896=CARTESIAN_POINT('Ctrl Pts',(-11.1472919002623,17.0153262488602,4.40860356931809));
#87897=CARTESIAN_POINT('Ctrl Pts',(-11.1489209284143,17.0151830122948,4.40654280131246));
#87898=CARTESIAN_POINT('Ctrl Pts',(-11.1523209227531,17.0148821984651,4.40221782513491));
#87899=CARTESIAN_POINT('Ctrl Pts',(-11.1540907710381,17.0147245419303,4.39995277917936));
#87900=CARTESIAN_POINT('Ctrl Pts',(-11.1583838339886,17.0143395352862,4.3944250416352));
#87901=CARTESIAN_POINT('Ctrl Pts',(-11.1608999422113,17.0141116947388,4.39115688028216));
#87902=CARTESIAN_POINT('Ctrl Pts',(-11.1698111860631,17.0132970377654,4.37948032283051));
#87903=CARTESIAN_POINT('Ctrl Pts',(-11.1761288990633,17.0127051812362,4.37101357559034));
#87904=CARTESIAN_POINT('Ctrl Pts',(-11.2148507413235,17.0089912990027,4.31793064812813));
#87905=CARTESIAN_POINT('Ctrl Pts',(-11.2448007594101,17.0057363308705,4.27158463023519));
#87906=CARTESIAN_POINT('Ctrl Pts',(-11.3106678187458,16.9977663443143,4.15580308637658));
#87907=CARTESIAN_POINT('Ctrl Pts',(-11.3437832115782,16.9930251080985,4.08495758407182));
#87908=CARTESIAN_POINT('Ctrl Pts',(-11.3825432396478,16.9864614586067,3.98112288061025));
#87909=CARTESIAN_POINT('Ctrl Pts',(-11.3929647398744,16.9845428485684,3.9500605103055));
#87910=CARTESIAN_POINT('Ctrl Pts',(-11.4141575606403,16.9802684479199,3.87907566903711));
#87911=CARTESIAN_POINT('Ctrl Pts',(-11.4242978289732,16.9779318108585,3.83899283489547));
#87912=CARTESIAN_POINT('Ctrl Pts',(-11.4347804835949,16.9750933406917,3.78868390867136));
#87913=CARTESIAN_POINT('Ctrl Pts',(-11.4367308346483,16.9745409480612,3.77881526339706));
#87914=CARTESIAN_POINT('Ctrl Pts',(-11.4396458364024,16.9736749061692,3.76322196330849));
#87915=CARTESIAN_POINT('Ctrl Pts',(-11.440678416869,16.9733591218415,3.75751045951987));
#87916=CARTESIAN_POINT('Ctrl Pts',(-11.4425237947289,16.9727775328631,3.74694447946007));
#87917=CARTESIAN_POINT('Ctrl Pts',(-11.4433461293506,16.9725114314014,3.74209177186111));
#87918=CARTESIAN_POINT('Ctrl Pts',(-11.4449133311798,16.9719902371055,3.73255158851063));
#87919=CARTESIAN_POINT('Ctrl Pts',(-11.4456599065061,16.9717350936399,3.72786445836986));
#87920=CARTESIAN_POINT('Ctrl Pts',(-11.4472790070098,16.9711659122954,3.71737110676397));
#87921=CARTESIAN_POINT('Ctrl Pts',(-11.4481394222268,16.9708522559021,3.71156308122382));
#87922=CARTESIAN_POINT('Ctrl Pts',(-11.4502077361232,16.9700690209958,3.69699727558352));
#87923=CARTESIAN_POINT('Ctrl Pts',(-11.4513712851896,16.9696008198982,3.68823336989376));
#87924=CARTESIAN_POINT('Ctrl Pts',(-11.4598112228208,16.9659742048019,3.61992467438711));
#87925=CARTESIAN_POINT('Ctrl Pts',(-11.4634999999992,16.9629297445978,3.55999266409901));
#87926=CARTESIAN_POINT('Ctrl Pts',(-11.4635,16.9599527886714,3.50000000001837));
#87927=CARTESIAN_POINT('Ctrl Pts',(-11.4635,16.8902616844768,3.4999999999813));
#87928=CARTESIAN_POINT('Ctrl Pts',(-11.4635000000007,16.89335037922,3.55281213409296));
#87929=CARTESIAN_POINT('Ctrl Pts',(-11.4606413650418,16.8963691047965,3.60559104637156));
#87930=CARTESIAN_POINT('Ctrl Pts',(-11.4539818303754,16.8997896038938,3.66687379711066));
#87931=CARTESIAN_POINT('Ctrl Pts',(-11.4529498272705,16.9002765088671,3.67563266053759));
#87932=CARTESIAN_POINT('Ctrl Pts',(-11.4511000140096,16.9010830101854,3.6901982549013));
#87933=CARTESIAN_POINT('Ctrl Pts',(-11.4503263766903,16.9014039737232,3.69601027857511));
#87934=CARTESIAN_POINT('Ctrl Pts',(-11.4488634630115,16.9019827164314,3.70651738951463));
#87935=CARTESIAN_POINT('Ctrl Pts',(-11.4481862422548,16.9022408691368,3.7112140504469));
#87936=CARTESIAN_POINT('Ctrl Pts',(-11.4468244644374,16.9027416456609,3.72034368110697));
#87937=CARTESIAN_POINT('Ctrl Pts',(-11.446142347434,16.9029843429946,3.72477695673199));
#87938=CARTESIAN_POINT('Ctrl Pts',(-11.444554207869,16.9035315721379,3.73479218144835));
#87939=CARTESIAN_POINT('Ctrl Pts',(-11.4436361892395,16.9038357232631,3.74037217453491));
#87940=CARTESIAN_POINT('Ctrl Pts',(-11.4410647658515,16.9046559646691,3.75545574832366));
#87941=CARTESIAN_POINT('Ctrl Pts',(-11.4393496905578,16.9051701108722,3.76494862332372));
#87942=CARTESIAN_POINT('Ctrl Pts',(-11.4309564475946,16.9075425178259,3.80891573088206));
#87943=CARTESIAN_POINT('Ctrl Pts',(-11.4231325205218,16.9093644722255,3.84316084965163));
#87944=CARTESIAN_POINT('Ctrl Pts',(-11.4057440918486,16.9128043699665,3.90836671804323));
#87945=CARTESIAN_POINT('Ctrl Pts',(-11.3963689959624,16.9144261951841,3.93935589572659));
#87946=CARTESIAN_POINT('Ctrl Pts',(-11.3649004917138,16.919279613917,4.03215080401589));
#87947=CARTESIAN_POINT('Ctrl Pts',(-11.3396715959119,16.9224448694413,4.09280521524113));
#87948=CARTESIAN_POINT('Ctrl Pts',(-11.2852129221592,16.9284083102357,4.20233560235017));
#87949=CARTESIAN_POINT('Ctrl Pts',(-11.2570400848649,16.9311941940619,4.25159624418857));
#87950=CARTESIAN_POINT('Ctrl Pts',(-11.2119382436526,16.9354307788527,4.32079781009414));
#87951=CARTESIAN_POINT('Ctrl Pts',(-11.1972204389118,16.9367844011855,4.34212018644379));
#87952=CARTESIAN_POINT('Ctrl Pts',(-11.1786012370859,16.9384774087478,4.36761946434593));
#87953=CARTESIAN_POINT('Ctrl Pts',(-11.1752304199506,16.9387831751503,4.37217995211778));
#87954=CARTESIAN_POINT('Ctrl Pts',(-11.1699087221228,16.9392649587196,4.37929298446356));
#87955=CARTESIAN_POINT('Ctrl Pts',(-11.1679757604145,16.9394397609743,4.38185894183996));
#87956=CARTESIAN_POINT('Ctrl Pts',(-11.1643456071108,16.9397677284019,4.38664500593607));
#87957=CARTESIAN_POINT('Ctrl Pts',(-11.1626504970261,16.9399207503906,4.38886662705221));
#87958=CARTESIAN_POINT('Ctrl Pts',(-11.1587509086081,16.9402724849199,4.3939472104895));
#87959=CARTESIAN_POINT('Ctrl Pts',(-11.1565422128257,16.9404714895862,4.39680287283134));
#87960=CARTESIAN_POINT('Ctrl Pts',(-11.1507156676456,16.9409958365497,4.40427879440517));
#87961=CARTESIAN_POINT('Ctrl Pts',(-11.1470805926991,16.9413223380852,4.40888546983398));
#87962=CARTESIAN_POINT('Ctrl Pts',(-11.1216363415272,16.9436026535979,4.44073480434506));
#87963=CARTESIAN_POINT('Ctrl Pts',(-11.0988881056078,16.9456154872101,4.46720970148674));
#87964=CARTESIAN_POINT('Ctrl Pts',(-11.0647434647968,16.9485702712058,4.50418722040169));
#87965=CARTESIAN_POINT('Ctrl Pts',(-11.054090824053,16.9494834867763,4.5153635472015));
#87966=CARTESIAN_POINT('Ctrl Pts',(-11.0159207566497,16.9527198717537,4.55416191571789));
#87967=CARTESIAN_POINT('Ctrl Pts',(-10.9874787585536,16.9550672571449,4.58085054767258));
#87968=CARTESIAN_POINT('Ctrl Pts',(-10.9019234678886,16.9618829091466,4.65493280004682));
#87969=CARTESIAN_POINT('Ctrl Pts',(-10.8422256118354,16.9663371410483,4.69916361321554));
#87970=CARTESIAN_POINT('Ctrl Pts',(-10.7517143338406,16.9725545796161,4.75611699236872));
#87971=CARTESIAN_POINT('Ctrl Pts',(-10.7234227541251,16.9744304313362,4.7726209509193));
#87972=CARTESIAN_POINT('Ctrl Pts',(-10.6817630579084,16.9770949285099,4.7950845818074));
#87973=CARTESIAN_POINT('Ctrl Pts',(-10.6688233222588,16.9779094254456,4.80181424414476));
#87974=CARTESIAN_POINT('Ctrl Pts',(-10.6455079960456,16.9793539818661,4.81350059898834));
#87975=CARTESIAN_POINT('Ctrl Pts',(-10.6351706410618,16.9799865177513,4.81853049408695));
#87976=CARTESIAN_POINT('Ctrl Pts',(-10.6193292975166,16.9809440067562,4.82600894964108));
#87977=CARTESIAN_POINT('Ctrl Pts',(-10.6138678417599,16.9812719926295,4.8285461180024));
#87978=CARTESIAN_POINT('Ctrl Pts',(-10.6038636537693,16.9818689793916,4.83311879244297));
#87979=CARTESIAN_POINT('Ctrl Pts',(-10.5993259182395,16.9821383412929,4.83516496047631));
#87980=CARTESIAN_POINT('Ctrl Pts',(-10.5895606365362,16.9827150026944,4.83950853287391));
#87981=CARTESIAN_POINT('Ctrl Pts',(-10.5843298948976,16.983022049085,4.84179857988866));
#87982=CARTESIAN_POINT('Ctrl Pts',(-10.5702282550169,16.9838449596233,4.84787425520504));
#87983=CARTESIAN_POINT('Ctrl Pts',(-10.5613330313325,16.9843589008717,4.85160293894766));
#87984=CARTESIAN_POINT('Ctrl Pts',(-10.5187725085019,16.9867942688017,4.86895074027179));
#87985=CARTESIAN_POINT('Ctrl Pts',(-10.4846434944711,16.9886766311215,4.88140218961791));
#87986=CARTESIAN_POINT('Ctrl Pts',(-10.4288846717029,16.9916593118974,4.89942365779989));
#87987=CARTESIAN_POINT('Ctrl Pts',(-10.4075305316961,16.9927803697149,4.9057907214393));
#87988=CARTESIAN_POINT('Ctrl Pts',(-10.2948851271674,16.9986036591346,4.9365950587712));
#87989=CARTESIAN_POINT('Ctrl Pts',(-10.2015346873645,17.0031048980956,4.95263414952543));
#87990=CARTESIAN_POINT('Ctrl Pts',(-10.0524265594114,17.0104712656073,4.96359489872749));
#87991=CARTESIAN_POINT('Ctrl Pts',(-9.9973837213499,17.013232520144,4.96453084290432));
#87992=CARTESIAN_POINT('Ctrl Pts',(-9.93187984411485,17.0166986107852,4.96195186618962));
#87993=CARTESIAN_POINT('Ctrl Pts',(-9.92134016759578,17.0172619092052,4.96142267419591));
#87994=CARTESIAN_POINT('Ctrl Pts',(-9.90669143169571,17.0180537263068,4.96052824888311));
#87995=CARTESIAN_POINT('Ctrl Pts',(-9.90257655223886,17.0182771291985,4.96025954052425));
#87996=CARTESIAN_POINT('Ctrl Pts',(-9.89559478404722,17.0186579228885,4.95977397799846));
#87997=CARTESIAN_POINT('Ctrl Pts',(-9.8927272625583,17.0188148204667,4.95956605730135));
#87998=CARTESIAN_POINT('Ctrl Pts',(-9.88723951302259,17.0191160713747,4.95915188745093));
#87999=CARTESIAN_POINT('Ctrl Pts',(-9.88461920395984,17.0192603426548,4.95894702774076));
#88000=CARTESIAN_POINT('Ctrl Pts',(-9.87767504600098,17.0196437916327,4.95838529845521));
#88001=CARTESIAN_POINT('Ctrl Pts',(-9.8733522426987,17.0198836349663,4.95801626112554));
#88002=CARTESIAN_POINT('Ctrl Pts',(-9.85796992065983,17.0207410106391,4.95663414976264));
#88003=CARTESIAN_POINT('Ctrl Pts',(-9.84692064786682,17.0213640781786,4.95551444047278));
#88004=CARTESIAN_POINT('Ctrl Pts',(-9.74400316615693,17.0272281388411,4.94390018908303));
#88005=CARTESIAN_POINT('Ctrl Pts',(-9.6533173247774,17.0328324558723,4.92484761846273));
#88006=CARTESIAN_POINT('Ctrl Pts',(-9.45910243890625,17.0450734821342,4.86439468900163));
#88007=CARTESIAN_POINT('Ctrl Pts',(-9.35723804009431,17.0516348228704,4.81947276901191));
#88008=CARTESIAN_POINT('Ctrl Pts',(-9.25113506556167,17.0584462851287,4.75744798118398));
#88009=CARTESIAN_POINT('Ctrl Pts',(-9.240925936346,17.0591019052583,4.75131158913208));
#88010=CARTESIAN_POINT('Ctrl Pts',(-9.22557039878675,17.060088584932,4.74182475574203));
#88011=CARTESIAN_POINT('Ctrl Pts',(-9.22036845455,17.0604229395197,4.73856553567167));
#88012=CARTESIAN_POINT('Ctrl Pts',(-9.21098603712189,17.0610262242354,4.73260455519468));
#88013=CARTESIAN_POINT('Ctrl Pts',(-9.20679856807581,17.0612955604987,4.72991402640408));
#88014=CARTESIAN_POINT('Ctrl Pts',(-9.19783320450969,17.0618724255376,4.72408877760042));
#88015=CARTESIAN_POINT('Ctrl Pts',(-9.19305976907069,17.0621796995026,4.72094732409402));
#88016=CARTESIAN_POINT('Ctrl Pts',(-9.18026382357236,17.0630038317806,4.71241834118109));
#88017=CARTESIAN_POINT('Ctrl Pts',(-9.17227599569888,17.0635187572762,4.70697912645057));
#88018=CARTESIAN_POINT('Ctrl Pts',(-9.13436238111056,17.0659658059864,4.68060890404718));
#88019=CARTESIAN_POINT('Ctrl Pts',(-9.10517188190542,17.0678583988897,4.65864092643342));
#88020=CARTESIAN_POINT('Ctrl Pts',(-9.05982403226755,17.0708323663943,4.62177620032891));
#88021=CARTESIAN_POINT('Ctrl Pts',(-9.04312832804937,17.0719352408389,4.60756911568014));
#88022=CARTESIAN_POINT('Ctrl Pts',(-8.93123262666583,17.0794070765859,4.50793285170755));
#88023=CARTESIAN_POINT('Ctrl Pts',(-8.84728187068836,17.0853689010154,4.41072904220659));
#88024=CARTESIAN_POINT('Ctrl Pts',(-8.76114283325084,17.0933735187918,4.2796811296197));
#88025=CARTESIAN_POINT('Ctrl Pts',(-8.74596892839718,17.0948801619964,4.25503350423086));
#88026=CARTESIAN_POINT('Ctrl Pts',(-8.72861535363916,17.0967445744688,4.22487766853542));
#88027=CARTESIAN_POINT('Ctrl Pts',(-8.72572463740558,17.0970602087341,4.21978389208233));
#88028=CARTESIAN_POINT('Ctrl Pts',(-8.72127600741376,17.0975541249693,4.21183409849562));
#88029=CARTESIAN_POINT('Ctrl Pts',(-8.71969687718765,17.0977310893847,4.20898994794834));
#88030=CARTESIAN_POINT('Ctrl Pts',(-8.7167814726013,17.0980609088623,4.20369754902429));
#88031=CARTESIAN_POINT('Ctrl Pts',(-8.71544270709535,17.0982136039617,4.2012507329159));
#88032=CARTESIAN_POINT('Ctrl Pts',(-8.71241546813742,17.0985617088266,4.19568019361937));
#88033=CARTESIAN_POINT('Ctrl Pts',(-8.71073137050195,17.0987573879611,4.19255415595445));
#88034=CARTESIAN_POINT('Ctrl Pts',(-8.70638715100488,17.0992673802706,4.1844196142826));
#88035=CARTESIAN_POINT('Ctrl Pts',(-8.70374476120458,17.099582754664,4.17940177013524));
#88036=CARTESIAN_POINT('Ctrl Pts',(-8.68686353710805,17.1016306962625,4.14688767928945));
#88037=CARTESIAN_POINT('Ctrl Pts',(-8.67347216346431,17.1034097810314,4.11896257040469));
#88038=CARTESIAN_POINT('Ctrl Pts',(-8.65608963689965,17.1059271632573,4.07955488685148));
#88039=CARTESIAN_POINT('Ctrl Pts',(-8.65133966569054,17.1066396110208,4.06841377708649));
#88040=CARTESIAN_POINT('Ctrl Pts',(-8.60080211628567,17.1144874411172,3.94567660801309));
#88041=CARTESIAN_POINT('Ctrl Pts',(-8.56883517412668,17.1218969886633,3.82886916603102));
#88042=CARTESIAN_POINT('Ctrl Pts',(-8.54442653661582,17.1318145132362,3.6600858367712));
#88043=CARTESIAN_POINT('Ctrl Pts',(-8.53981477302907,17.1346499176092,3.61036991531203));
#88044=CARTESIAN_POINT('Ctrl Pts',(-8.53732692991212,17.1379739913432,3.55025121128117));
#88045=CARTESIAN_POINT('Ctrl Pts',(-8.53701034204621,17.1385379245376,3.53998702876895));
#88046=CARTESIAN_POINT('Ctrl Pts',(-8.53668420183079,17.1394146461739,3.52393033477724));
#88047=CARTESIAN_POINT('Ctrl Pts',(-8.53660096505459,17.1397297094864,3.51813978944827));
#88048=CARTESIAN_POINT('Ctrl Pts',(-8.53651435601033,17.1402862436664,3.50787584676922));
#88049=CARTESIAN_POINT('Ctrl Pts',(-8.5364971193733,17.1405281412553,3.5034026664653));
#88050=CARTESIAN_POINT('Ctrl Pts',(-8.5365046570984,17.1410839102337,3.49309826001539));
#88051=CARTESIAN_POINT('Ctrl Pts',(-8.53654377336601,17.1413973330742,3.48726709836156));
#88052=CARTESIAN_POINT('Ctrl Pts',(-8.53674677810797,17.1422545982633,3.47126419914061));
#88053=CARTESIAN_POINT('Ctrl Pts',(-8.53698187445544,17.1427962302983,3.46109358731615));
#88054=CARTESIAN_POINT('Ctrl Pts',(-8.53876093803724,17.1456043971672,3.40806755523621));
#88055=CARTESIAN_POINT('Ctrl Pts',(-8.54208194713816,17.14781536184,3.36529080194802));
#88056=CARTESIAN_POINT('Ctrl Pts',(-8.56441014325499,17.1571281113155,3.18232341650703));
#88057=CARTESIAN_POINT('Ctrl Pts',(-8.6018005334906,17.1636681683375,3.04517314002671));
#88058=CARTESIAN_POINT('Ctrl Pts',(-8.67025364937187,17.1724029956135,2.88803060341119));
#88059=CARTESIAN_POINT('Ctrl Pts',(-8.68307400391874,17.1739626017201,2.86090878996597));
#88060=CARTESIAN_POINT('Ctrl Pts',(-8.69940889791892,17.1758862903973,2.82893365977738));
#88061=CARTESIAN_POINT('Ctrl Pts',(-8.70213212062496,17.1762050556995,2.82368186991408));
#88062=CARTESIAN_POINT('Ctrl Pts',(-8.70640801965747,17.1767028185314,2.81555664599556));
#88063=CARTESIAN_POINT('Ctrl Pts',(-8.70793863171435,17.1768804651792,2.81267159479299));
#88064=CARTESIAN_POINT('Ctrl Pts',(-8.71079367157516,17.1772108892496,2.80733336665678));
#88065=CARTESIAN_POINT('Ctrl Pts',(-8.71211545892147,17.1773635014945,2.80487883741931));
#88066=CARTESIAN_POINT('Ctrl Pts',(-8.71512843807533,17.1777105528542,2.79932189678595));
#88067=CARTESIAN_POINT('Ctrl Pts',(-8.7168238491555,17.1779052546297,2.79622183869518));
#88068=CARTESIAN_POINT('Ctrl Pts',(-8.72124182175142,17.1784110513087,2.78821261322978));
#88069=CARTESIAN_POINT('Ctrl Pts',(-8.72398140633879,17.1787231795314,2.7833129630281));
#88070=CARTESIAN_POINT('Ctrl Pts',(-8.74149798929534,17.1807087991807,2.75240399611916));
#88071=CARTESIAN_POINT('Ctrl Pts',(-8.757040392671,17.1824257109178,2.72683878781948));
#88072=CARTESIAN_POINT('Ctrl Pts',(-8.83039316897241,17.1902761721673,2.61411707835031));
#88073=CARTESIAN_POINT('Ctrl Pts',(-8.89666210949767,17.1966890873366,2.53283155719234));
#88074=CARTESIAN_POINT('Ctrl Pts',(-9.00786071697484,17.2059794949853,2.4228859923147));
#88075=CARTESIAN_POINT('Ctrl Pts',(-9.04660170425233,17.2090063177096,2.38844818476036));
#88076=CARTESIAN_POINT('Ctrl Pts',(-9.11066594023569,17.2136721137163,2.33731904039774));
#88077=CARTESIAN_POINT('Ctrl Pts',(-9.13481872247482,17.2153619961065,2.31923599736667));
#88078=CARTESIAN_POINT('Ctrl Pts',(-9.16670577816148,17.2175069302329,2.29686652646461));
#88079=CARTESIAN_POINT('Ctrl Pts',(-9.17394245689282,17.2179882061084,2.29188644760052));
#88080=CARTESIAN_POINT('Ctrl Pts',(-9.18575307003271,17.2187648952296,2.28391445624249));
#88081=CARTESIAN_POINT('Ctrl Pts',(-9.190299621419,17.2190618047691,2.28088252791108));
#88082=CARTESIAN_POINT('Ctrl Pts',(-9.19905795357079,17.2196298216614,2.27511252659459));
#88083=CARTESIAN_POINT('Ctrl Pts',(-9.2032670517212,17.2199010721537,2.27237053870466));
#88084=CARTESIAN_POINT('Ctrl Pts',(-9.21291637723249,17.220519016497,2.26615508261436));
#88085=CARTESIAN_POINT('Ctrl Pts',(-9.21836565383983,17.220865183764,2.26269580938639));
#88086=CARTESIAN_POINT('Ctrl Pts',(-9.23287249434296,17.2217794432786,2.25362075931515));
#88087=CARTESIAN_POINT('Ctrl Pts',(-9.24196890831453,17.2223452532561,2.24806761622092));
#88088=CARTESIAN_POINT('Ctrl Pts',(-9.31856015257893,17.2270491664284,2.20245135112076));
#88089=CARTESIAN_POINT('Ctrl Pts',(-9.38911985454486,17.2309852611936,2.16777620024398));
#88090=CARTESIAN_POINT('Ctrl Pts',(-9.47696599294441,17.2356204052849,2.13306099793535));
#88091=CARTESIAN_POINT('Ctrl Pts',(-9.49189925243254,17.2363999368057,2.1274401848359));
#88092=CARTESIAN_POINT('Ctrl Pts',(-9.58492216299372,17.2412159237708,2.09415299738017));
#88093=CARTESIAN_POINT('Ctrl Pts',(-9.66514665899465,17.2451885944046,2.07291664305876));
#88094=CARTESIAN_POINT('Ctrl Pts',(-9.78009805732002,17.2511028118691,2.05271870301203));
#88095=CARTESIAN_POINT('Ctrl Pts',(-9.81365669131164,17.2528564663376,2.04801658213785));
#88096=CARTESIAN_POINT('Ctrl Pts',(-9.85342394220545,17.2549972999964,2.04384579719927));
#88097=CARTESIAN_POINT('Ctrl Pts',(-9.85950614430575,17.2553264555888,2.04324639113841));
#88098=CARTESIAN_POINT('Ctrl Pts',(-9.86888598383427,17.255836971341,2.0423812883255));
#88099=CARTESIAN_POINT('Ctrl Pts',(-9.87218114048978,17.2560168673899,2.0420886403593));
#88100=CARTESIAN_POINT('Ctrl Pts',(-9.87825172965127,17.2563493454796,2.04157024075065));
#88101=CARTESIAN_POINT('Ctrl Pts',(-9.88102683081592,17.2565017453747,2.04134123638593));
#88102=CARTESIAN_POINT('Ctrl Pts',(-9.88727135032299,17.2568455975948,2.04084387050219));
#88103=CARTESIAN_POINT('Ctrl Pts',(-9.89074105948706,17.2570372918597,2.04057996378357));
#88104=CARTESIAN_POINT('Ctrl Pts',(-9.90091087071076,17.2576009496986,2.03984291602412));
#88105=CARTESIAN_POINT('Ctrl Pts',(-9.90761323485814,17.2579747096085,2.03940353022375));
#88106=CARTESIAN_POINT('Ctrl Pts',(-9.95554117129185,17.2606625959298,2.03659273057803));
#88107=CARTESIAN_POINT('Ctrl Pts',(-9.99684455670688,17.2630587374229,2.03592115081653));
#88108=CARTESIAN_POINT('Ctrl Pts',(-10.120386982239,17.2703597784982,2.03913993008715));
#88109=CARTESIAN_POINT('Ctrl Pts',(-10.202328520742,17.2753715873642,2.0482188816));
#88110=CARTESIAN_POINT('Ctrl Pts',(-10.3405837684763,17.2837873104213,2.0754751554899));
#88111=CARTESIAN_POINT('Ctrl Pts',(-10.397365972315,17.2872338856815,2.09025898361895));
#88112=CARTESIAN_POINT('Ctrl Pts',(-10.4842638695639,17.2924524093954,2.11855364923184));
#88113=CARTESIAN_POINT('Ctrl Pts',(-10.5150670675056,17.2942915208246,2.12974028992148));
#88114=CARTESIAN_POINT('Ctrl Pts',(-10.5538550286932,17.296594648696,2.14531978090492));
#88115=CARTESIAN_POINT('Ctrl Pts',(-10.5622081647165,17.2970898911657,2.14876505614868));
#88116=CARTESIAN_POINT('Ctrl Pts',(-10.5756123665536,17.2978835121415,2.15443947551393));
#88117=CARTESIAN_POINT('Ctrl Pts',(-10.5806835719353,17.2981835092858,2.15662019070045));
#88118=CARTESIAN_POINT('Ctrl Pts',(-10.5903320360833,17.2987538380874,2.16083405799658));
#88119=CARTESIAN_POINT('Ctrl Pts',(-10.5949114244475,17.2990243370432,2.16286211220678));
#88120=CARTESIAN_POINT('Ctrl Pts',(-10.6053653725786,17.2996414375386,2.16755614305354));
#88121=CARTESIAN_POINT('Ctrl Pts',(-10.6112329197835,17.2999875089762,2.17023754534025));
#88122=CARTESIAN_POINT('Ctrl Pts',(-10.6265229437274,17.3008886688687,2.17734749789746));
#88123=CARTESIAN_POINT('Ctrl Pts',(-10.635916321421,17.3014416370989,2.18183799177558));
#88124=CARTESIAN_POINT('Ctrl Pts',(-10.706154980103,17.3055730585518,2.2163410809698));
#88125=CARTESIAN_POINT('Ctrl Pts',(-10.7648984811528,17.3090036579923,2.25045333873286));
#88126=CARTESIAN_POINT('Ctrl Pts',(-10.8429548295491,17.313662117074,2.30335533918458));
#88127=CARTESIAN_POINT('Ctrl Pts',(-10.8644355218974,17.3149562520115,2.31877920765174));
#88128=CARTESIAN_POINT('Ctrl Pts',(-10.9366821680572,17.3193802119256,2.37368152666745));
#88129=CARTESIAN_POINT('Ctrl Pts',(-10.9852561675272,17.3224774912393,2.41591670478913));
#88130=CARTESIAN_POINT('Ctrl Pts',(-11.0645338892668,17.3280195049125,2.49459162579542));
#88131=CARTESIAN_POINT('Ctrl Pts',(-11.0965295312416,17.3304194677486,2.52958740422337));
#88132=CARTESIAN_POINT('Ctrl Pts',(-11.1330129578751,17.3334481403963,2.57360394959969));
#88133=CARTESIAN_POINT('Ctrl Pts',(-11.1391816357424,17.3339711740101,2.58120013310973));
#88134=CARTESIAN_POINT('Ctrl Pts',(-11.1477645250759,17.3347154103938,2.59198851656597));
#88135=CARTESIAN_POINT('Ctrl Pts',(-11.1502426612193,17.3349322771497,2.5951298001296));
#88136=CARTESIAN_POINT('Ctrl Pts',(-11.154465064848,17.335305278341,2.60052748914215));
#88137=CARTESIAN_POINT('Ctrl Pts',(-11.1562156958889,17.3354609678447,2.60277893011944));
#88138=CARTESIAN_POINT('Ctrl Pts',(-11.1595844787085,17.3357626114881,2.60713766696617));
#88139=CARTESIAN_POINT('Ctrl Pts',(-11.1612034821628,17.335908498797,2.60924426367743));
#88140=CARTESIAN_POINT('Ctrl Pts',(-11.1650865367989,17.3362605970419,2.61432535016366));
#88141=CARTESIAN_POINT('Ctrl Pts',(-11.1673449333696,17.3364671933104,2.61730411267632));
#88142=CARTESIAN_POINT('Ctrl Pts',(-11.175585578828,17.3372276275163,2.628260232211));
#88143=CARTESIAN_POINT('Ctrl Pts',(-11.1814975275428,17.3377860168106,2.63628983034558));
#88144=CARTESIAN_POINT('Ctrl Pts',(-11.2515593078446,17.3445536178853,2.73351304884013));
#88145=CARTESIAN_POINT('Ctrl Pts',(-11.3055466259008,17.3512792384178,2.82959076645209));
#88146=CARTESIAN_POINT('Ctrl Pts',(-11.3734912880735,17.3617503272508,2.99053156222294));
#88147=CARTESIAN_POINT('Ctrl Pts',(-11.3947138580813,17.3655826748097,3.051880485676));
#88148=CARTESIAN_POINT('Ctrl Pts',(-11.4210080933477,17.3712966023831,3.14816167448934));
#88149=CARTESIAN_POINT('Ctrl Pts',(-11.4290067638186,17.3732622520977,3.18220420014149));
#88150=CARTESIAN_POINT('Ctrl Pts',(-11.4375673537468,17.3756982717713,3.22555951952907));
#88151=CARTESIAN_POINT('Ctrl Pts',(-11.439269932196,17.3762044368888,3.23463319415922));
#88152=CARTESIAN_POINT('Ctrl Pts',(-11.441860804296,17.3770112965359,3.24920003326018));
#88153=CARTESIAN_POINT('Ctrl Pts',(-11.4428038072576,17.3773137079633,3.2546831085364));
#88154=CARTESIAN_POINT('Ctrl Pts',(-11.4445346874309,17.3778859616642,3.26510263078824));
#88155=CARTESIAN_POINT('Ctrl Pts',(-11.4453285821394,17.3781559895576,3.27003798626276));
#88156=CARTESIAN_POINT('Ctrl Pts',(-11.4470767804593,17.3787683762951,3.28127269851218));
#88157=CARTESIAN_POINT('Ctrl Pts',(-11.4480152703731,17.3791102345977,3.28757443779273));
#88158=CARTESIAN_POINT('Ctrl Pts',(-11.4503414674635,17.3799931653142,3.30392652295263));
#88159=CARTESIAN_POINT('Ctrl Pts',(-11.4516658838143,17.3805322576375,3.31398562068876));
#88160=CARTESIAN_POINT('Ctrl Pts',(-11.4599550046097,17.3841744734214,3.38243507604782));
#88161=CARTESIAN_POINT('Ctrl Pts',(-11.4634999999993,17.387168492118,3.4411881824418));
#88162=CARTESIAN_POINT('Ctrl Pts',(-11.4635,17.3900944100234,3.49999999998336));
#88163=CARTESIAN_POINT('Origin',(-10.,13.2,3.5));
#88164=CARTESIAN_POINT('',(-11.4635,17.9619558011997,3.500000000001));
#88165=CARTESIAN_POINT('',(-11.4635,17.8879846534521,3.50000000000001));
#88166=CARTESIAN_POINT('',(-11.4635,13.2,3.5));
#88167=CARTESIAN_POINT('Ctrl Pts',(-11.4635,17.9619558011997,3.500000000001));
#88168=CARTESIAN_POINT('Ctrl Pts',(-11.4635000000001,17.9578239784063,3.4269116130009));
#88169=CARTESIAN_POINT('Ctrl Pts',(-11.4580248356914,17.9534532242815,3.35392967682306));
#88170=CARTESIAN_POINT('Ctrl Pts',(-11.4386952867223,17.9456567463325,3.22581223811122));
#88171=CARTESIAN_POINT('Ctrl Pts',(-11.427041201044,17.9422473245681,3.17048996468713));
#88172=CARTESIAN_POINT('Ctrl Pts',(-11.3989284884513,17.9358886003781,3.06710694649229));
#88173=CARTESIAN_POINT('Ctrl Pts',(-11.3831101110572,17.9329320672596,3.01895479262035));
#88174=CARTESIAN_POINT('Ctrl Pts',(-11.3541030665059,17.9283604139683,2.94401487060868));
#88175=CARTESIAN_POINT('Ctrl Pts',(-11.3425393561018,17.9266968833111,2.91664518778092));
#88176=CARTESIAN_POINT('Ctrl Pts',(-11.3265067049631,17.9245801650968,2.88170514673387));
#88177=CARTESIAN_POINT('Ctrl Pts',(-11.3227923620327,17.9241015917339,2.87379800744325));
#88178=CARTESIAN_POINT('Ctrl Pts',(-11.31664492699,17.923328244677,2.8610100793101));
#88179=CARTESIAN_POINT('Ctrl Pts',(-11.3142550004792,17.9230319975196,2.85610887772145));
#88180=CARTESIAN_POINT('Ctrl Pts',(-11.3096102118658,17.9224645756437,2.84671706660158));
#88181=CARTESIAN_POINT('Ctrl Pts',(-11.3073595088221,17.92219326236,2.84222449600517));
#88182=CARTESIAN_POINT('Ctrl Pts',(-11.3021563952054,17.9215742502647,2.83197090117125));
#88183=CARTESIAN_POINT('Ctrl Pts',(-11.2991887975369,17.921227085385,2.82621767265183));
#88184=CARTESIAN_POINT('Ctrl Pts',(-11.2912031422431,17.920308212583,2.81098495506568));
#88185=CARTESIAN_POINT('Ctrl Pts',(-11.2861188326014,17.9197388254639,2.80154052140793));
#88186=CARTESIAN_POINT('Ctrl Pts',(-11.2389266539427,17.9145910892826,2.71614085320336));
#88187=CARTESIAN_POINT('Ctrl Pts',(-11.1902382435879,17.9102642492208,2.64401527820695));
#88188=CARTESIAN_POINT('Ctrl Pts',(-11.0654196758604,17.9005952699772,2.49053097405107));
#88189=CARTESIAN_POINT('Ctrl Pts',(-10.9858480790831,17.8953398435327,2.41268933228949));
#88190=CARTESIAN_POINT('Ctrl Pts',(-10.8899467279994,17.8889918056793,2.33813170259552));
#88191=CARTESIAN_POINT('Ctrl Pts',(-10.8815646440005,17.8884366667639,2.33175906337484));
#88192=CARTESIAN_POINT('Ctrl Pts',(-10.8687195194081,17.8875842818664,2.32221027341934));
#88193=CARTESIAN_POINT('Ctrl Pts',(-10.8643060493826,17.8872911164504,2.31896769958697));
#88194=CARTESIAN_POINT('Ctrl Pts',(-10.8570466201691,17.8868082445939,2.31369668539351));
#88195=CARTESIAN_POINT('Ctrl Pts',(-10.8542113726267,17.8866194896457,2.31165350433316));
#88196=CARTESIAN_POINT('Ctrl Pts',(-10.8487351897889,17.8862545441104,2.30773689485491));
#88197=CARTESIAN_POINT('Ctrl Pts',(-10.8460952984626,17.8860784503454,2.30586203486353));
#88198=CARTESIAN_POINT('Ctrl Pts',(-10.8434384098184,17.8859010338455,2.30398833658764));
#88199=CARTESIAN_POINT('Ctrl Pts',(-10.8434275861427,17.8859003110802,2.30398070370547));
#88200=CARTESIAN_POINT('Ctrl Pts',(-10.8434058271742,17.8858988580898,2.3039653596707));
#88201=CARTESIAN_POINT('Ctrl Pts',(-10.8433948918587,17.8858981278632,2.30395764850664));
#88202=CARTESIAN_POINT('Ctrl Pts',(-10.843372907423,17.885896659804,2.30394214637937));
#88203=CARTESIAN_POINT('Ctrl Pts',(-10.8433618582589,17.8858959219684,2.30393435538978));
#88204=CARTESIAN_POINT('Ctrl Pts',(-10.8433396437819,17.8858944385345,2.30391869197265));
#88205=CARTESIAN_POINT('Ctrl Pts',(-10.8433284786114,17.8858936929456,2.30391081965029));
#88206=CARTESIAN_POINT('Ctrl Pts',(-10.8433060299012,17.8858921938567,2.30389499201663));
#88207=CARTESIAN_POINT('Ctrl Pts',(-10.8432947463136,17.8858914403534,2.30388703667655));
#88208=CARTESIAN_POINT('Ctrl Pts',(-10.8432720585338,17.885889925286,2.30387104144625));
#88209=CARTESIAN_POINT('Ctrl Pts',(-10.8432606542248,17.8858891637141,2.30386300147888));
#88210=CARTESIAN_POINT('Ctrl Pts',(-10.8432377224495,17.8858876323389,2.30384683521));
#88211=CARTESIAN_POINT('Ctrl Pts',(-10.8432261951198,17.8858868625446,2.30383870901004));
#88212=CARTESIAN_POINT('Ctrl Pts',(-10.8432030147971,17.8858853145572,2.30382236852533));
#88213=CARTESIAN_POINT('Ctrl Pts',(-10.8431913618671,17.8858845363681,2.30381415429038));
#88214=CARTESIAN_POINT('Ctrl Pts',(-10.8431679279395,17.8858829714301,2.30379763605739));
#88215=CARTESIAN_POINT('Ctrl Pts',(-10.843156146843,17.8858821846745,2.30378933199517));
#88216=CARTESIAN_POINT('Ctrl Pts',(-10.8431324539833,17.8858806024298,2.30377263229248));
#88217=CARTESIAN_POINT('Ctrl Pts',(-10.8431205421937,17.8858798069388,2.30376423663924));
#88218=CARTESIAN_POINT('Ctrl Pts',(-10.8430965851956,17.8858782070392,2.30374735183211));
#88219=CARTESIAN_POINT('Ctrl Pts',(-10.8430845400392,17.885877402634,2.30373886272102));
#88220=CARTESIAN_POINT('Ctrl Pts',(-10.8430603135512,17.8858757847215,2.30372178907369));
#88221=CARTESIAN_POINT('Ctrl Pts',(-10.8430481322439,17.8858749712158,2.30371320456085));
#88222=CARTESIAN_POINT('Ctrl Pts',(-10.8430236306788,17.8858733349168,2.30369593817276));
#88223=CARTESIAN_POINT('Ctrl Pts',(-10.8430113103858,17.8858725121211,2.3036872562792));
#88224=CARTESIAN_POINT('Ctrl Pts',(-10.8429865280067,17.8858708570519,2.3036697931459));
#88225=CARTESIAN_POINT('Ctrl Pts',(-10.8429740658253,17.885870024772,2.30366101184557));
#88226=CARTESIAN_POINT('Ctrl Pts',(-10.8429489966553,17.8858683505329,2.30364334779481));
#88227=CARTESIAN_POINT('Ctrl Pts',(-10.8429363896473,17.8858675085723,2.30363446503748));
#88228=CARTESIAN_POINT('Ctrl Pts',(-10.8429110276435,17.8858658147591,2.30361659585214));
#88229=CARTESIAN_POINT('Ctrl Pts',(-10.8428982727602,17.8858649629139,2.30360760951048));
#88230=CARTESIAN_POINT('Ctrl Pts',(-10.8428726119136,17.8858632491246,2.30358953099901));
#88231=CARTESIAN_POINT('Ctrl Pts',(-10.8428597059039,17.8858623871774,2.30358043880382));
#88232=CARTESIAN_POINT('Ctrl Pts',(-10.8428337396388,17.8858606529723,2.30356214637712));
#88233=CARTESIAN_POINT('Ctrl Pts',(-10.8428206792984,17.8858597807086,2.30355294609324));
#88234=CARTESIAN_POINT('Ctrl Pts',(-10.8427944009659,17.885858025643,2.30353443511238));
#88235=CARTESIAN_POINT('Ctrl Pts',(-10.8427811830113,17.8858571428433,2.30352512444957));
#88236=CARTESIAN_POINT('Ctrl Pts',(-10.8427545859658,17.8858553664726,2.30350639027972));
#88237=CARTESIAN_POINT('Ctrl Pts',(-10.8427412069267,17.8858544729048,2.30349696681726));
#88238=CARTESIAN_POINT('Ctrl Pts',(-10.842714284224,17.8858526747645,2.30347800461539));
#88239=CARTESIAN_POINT('Ctrl Pts',(-10.8427007405361,17.8858517701902,2.30346846586716));
#88240=CARTESIAN_POINT('Ctrl Pts',(-10.8404691647733,17.8857027238442,2.30189683546785));
#88241=CARTESIAN_POINT('Ctrl Pts',(-10.8382468456193,17.8855541588349,2.30034095043559));
#88242=CARTESIAN_POINT('Ctrl Pts',(-10.8330583046954,17.8852069902392,2.29672981692358));
#88243=CARTESIAN_POINT('Ctrl Pts',(-10.8300888051139,17.8850080690524,2.29467935902838));
#88244=CARTESIAN_POINT('Ctrl Pts',(-10.8222730246246,17.8844839683172,2.28932509537366));
#88245=CARTESIAN_POINT('Ctrl Pts',(-10.8174144624592,17.8841576307521,2.28603943806788));
#88246=CARTESIAN_POINT('Ctrl Pts',(-10.7836405927923,17.8818861545121,2.26349415627565));
#88247=CARTESIAN_POINT('Ctrl Pts',(-10.7540692663234,17.8798825235075,2.24524167790199));
#88248=CARTESIAN_POINT('Ctrl Pts',(-10.6032233788279,17.8696946768747,2.15939314137159));
#88249=CARTESIAN_POINT('Ctrl Pts',(-10.4734052830455,17.8611155959333,2.10823768925242));
#88250=CARTESIAN_POINT('Ctrl Pts',(-10.2986176619481,17.8507636209629,2.06670879154108));
#88251=CARTESIAN_POINT('Ctrl Pts',(-10.258551709108,17.8484600692726,2.05894216926438));
#88252=CARTESIAN_POINT('Ctrl Pts',(-10.2086289047256,17.8456742942333,2.05141443943374));
#88253=CARTESIAN_POINT('Ctrl Pts',(-10.1990329485125,17.845142607357,2.05006481595887));
#88254=CARTESIAN_POINT('Ctrl Pts',(-10.1838084353106,17.8443049085491,2.04807755632345));
#88255=CARTESIAN_POINT('Ctrl Pts',(-10.1781884790737,17.8439969407621,2.04737713410297));
#88256=CARTESIAN_POINT('Ctrl Pts',(-10.1676185234017,17.8434200424035,2.04612205167216));
#88257=CARTESIAN_POINT('Ctrl Pts',(-10.1626694965585,17.8431508848909,2.04556000682067));
#88258=CARTESIAN_POINT('Ctrl Pts',(-10.1515485599541,17.8425481694316,2.04435451126075));
#88259=CARTESIAN_POINT('Ctrl Pts',(-10.145375211774,17.8422150513704,2.04372502447737));
#88260=CARTESIAN_POINT('Ctrl Pts',(-10.1296368357753,17.8413694091386,2.04222128193478));
#88261=CARTESIAN_POINT('Ctrl Pts',(-10.1200667829685,17.8408585933469,2.04140188073448));
#88262=CARTESIAN_POINT('Ctrl Pts',(-10.062435512613,17.8378018763012,2.03703846571261));
#88263=CARTESIAN_POINT('Ctrl Pts',(-10.0142289255224,17.8353276865979,2.03577570216286));
#88264=CARTESIAN_POINT('Ctrl Pts',(-9.83019161944957,17.8260784313615,2.04004682925809));
#88265=CARTESIAN_POINT('Ctrl Pts',(-9.69545837745759,17.8197750539726,2.06210368799201));
#88266=CARTESIAN_POINT('Ctrl Pts',(-9.5374567626927,17.811338270566,2.11120139820152));
#88267=CARTESIAN_POINT('Ctrl Pts',(-9.50947450521493,17.8097989529983,2.12083637474761));
#88268=CARTESIAN_POINT('Ctrl Pts',(-9.47629497950738,17.8078980422194,2.13339836837976));
#88269=CARTESIAN_POINT('Ctrl Pts',(-9.4707972449517,17.8075805344892,2.13551789688634));
#88270=CARTESIAN_POINT('Ctrl Pts',(-9.46227778772306,17.8070843533241,2.13886161581068));
#88271=CARTESIAN_POINT('Ctrl Pts',(-9.45924704052482,17.8069070175854,2.14006282686155));
#88272=CARTESIAN_POINT('Ctrl Pts',(-9.45363255578693,17.8065769304739,2.14230981617012));
#88273=CARTESIAN_POINT('Ctrl Pts',(-9.45104777842761,17.8064243422645,2.14335285449391));
#88274=CARTESIAN_POINT('Ctrl Pts',(-9.44518846632145,17.8060770357351,2.14573675658051));
#88275=CARTESIAN_POINT('Ctrl Pts',(-9.44191581964567,17.8058820525349,2.14708210985472));
#88276=CARTESIAN_POINT('Ctrl Pts',(-9.43344675395032,17.805374936047,2.15059961814272));
#88277=CARTESIAN_POINT('Ctrl Pts',(-9.42825798729957,17.8050617602296,2.15278990502998));
#88278=CARTESIAN_POINT('Ctrl Pts',(-9.39526196264111,17.8030549984217,2.16694316912226));
#88279=CARTESIAN_POINT('Ctrl Pts',(-9.36782067236811,17.8013169475566,2.17973576615908));
#88280=CARTESIAN_POINT('Ctrl Pts',(-9.24949964985647,17.7935776189337,2.23942934116641));
#88281=CARTESIAN_POINT('Ctrl Pts',(-9.16328154215047,17.7873119295541,2.29493079105269));
#88282=CARTESIAN_POINT('Ctrl Pts',(-9.02758784870345,17.7769605572523,2.40391635103249));
#88283=CARTESIAN_POINT('Ctrl Pts',(-8.97500043135013,17.7727900003606,2.45292648651613));
#88284=CARTESIAN_POINT('Ctrl Pts',(-8.9152158207681,17.7678775462634,2.51748400504331));
#88285=CARTESIAN_POINT('Ctrl Pts',(-8.90441227605018,17.7669818123857,2.52954548556323));
#88286=CARTESIAN_POINT('Ctrl Pts',(-8.88926512874283,17.7657138636953,2.54703174425177));
#88287=CARTESIAN_POINT('Ctrl Pts',(-8.88475681066598,17.7653348908372,2.55231171703899));
#88288=CARTESIAN_POINT('Ctrl Pts',(-8.87701362477559,17.7646811575558,2.56151202445327));
#88289=CARTESIAN_POINT('Ctrl Pts',(-8.87376131796731,17.7644056907506,2.56541746689523));
#88290=CARTESIAN_POINT('Ctrl Pts',(-8.86755013074508,17.763877866892,2.57295550650969));
#88291=CARTESIAN_POINT('Ctrl Pts',(-8.86458822511482,17.7636253898667,2.57658552023413));
#88292=CARTESIAN_POINT('Ctrl Pts',(-8.8576452398546,17.7630316850439,2.5851785251133));
#88293=CARTESIAN_POINT('Ctrl Pts',(-8.85367897367856,17.7626910489818,2.59015340013253));
#88294=CARTESIAN_POINT('Ctrl Pts',(-8.83996499907785,17.7615079166721,2.60758682558888));
#88295=CARTESIAN_POINT('Ctrl Pts',(-8.83038674689719,17.7606720659456,2.62017766508086));
#88296=CARTESIAN_POINT('Ctrl Pts',(-8.74674393411434,17.7532791232034,2.73390866112099));
#88297=CARTESIAN_POINT('Ctrl Pts',(-8.68575762727706,17.7472738200766,2.84401529859718));
#88298=CARTESIAN_POINT('Ctrl Pts',(-8.61935589402173,17.7384836200859,3.01147680254895));
#88299=CARTESIAN_POINT('Ctrl Pts',(-8.60204043507687,17.7357868222409,3.06348961712328));
#88300=CARTESIAN_POINT('Ctrl Pts',(-8.58102961438722,17.7316724426748,3.14083533779503));
#88301=CARTESIAN_POINT('Ctrl Pts',(-8.57501570909544,17.7303456128719,3.16549166542026));
#88302=CARTESIAN_POINT('Ctrl Pts',(-8.56845372326699,17.7286827195154,3.19579734255523));
#88303=CARTESIAN_POINT('Ctrl Pts',(-8.56729313849824,17.7283788876822,3.20131112148117));
#88304=CARTESIAN_POINT('Ctrl Pts',(-8.56552263529681,17.7278995208726,3.20997033744673));
#88305=CARTESIAN_POINT('Ctrl Pts',(-8.56489114420386,17.7277251813479,3.21311136896306));
#88306=CARTESIAN_POINT('Ctrl Pts',(-8.5637281287112,17.7273976609008,3.21899613462274));
#88307=CARTESIAN_POINT('Ctrl Pts',(-8.56319414661685,17.7272446198982,3.22173933108814));
#88308=CARTESIAN_POINT('Ctrl Pts',(-8.56198641520402,17.7268922843095,3.22803991315835));
#88309=CARTESIAN_POINT('Ctrl Pts',(-8.56131800893608,17.7266926933202,3.23159827329077));
#88310=CARTESIAN_POINT('Ctrl Pts',(-8.55959418159968,17.7261656863293,3.24096679676589));
#88311=CARTESIAN_POINT('Ctrl Pts',(-8.55856072181247,17.7258370919892,3.2467808716604));
#88312=CARTESIAN_POINT('Ctrl Pts',(-8.55154323838913,17.7235146954363,3.28769566456115));
#88313=CARTESIAN_POINT('Ctrl Pts',(-8.54680723604831,17.7214594734258,3.32299572999621));
#88314=CARTESIAN_POINT('Ctrl Pts',(-8.54319327805999,17.7192645070637,3.36018041392662));
#88315=CARTESIAN_POINT('Ctrl Pts',(-8.54302634261115,17.7191611137012,3.36193080220547));
#88316=CARTESIAN_POINT('Ctrl Pts',(-8.53018468905039,17.7110476105424,3.49919795017696));
#88317=CARTESIAN_POINT('Ctrl Pts',(-8.53647081074344,17.7026501029379,3.635827922689));
#88318=CARTESIAN_POINT('Ctrl Pts',(-8.56907111877884,17.6924542680991,3.80974090697808));
#88319=CARTESIAN_POINT('Ctrl Pts',(-8.57826232761715,17.690150220451,3.84951301165193));
#88320=CARTESIAN_POINT('Ctrl Pts',(-8.5916791977902,17.6873639368033,3.89819426936433));
#88321=CARTESIAN_POINT('Ctrl Pts',(-8.59434676426212,17.686832215656,3.90751091433013));
#88322=CARTESIAN_POINT('Ctrl Pts',(-8.59871965684432,17.6859944753849,3.92222946931813));
#88323=CARTESIAN_POINT('Ctrl Pts',(-8.60036411147688,17.685686500077,3.92764904500284));
#88324=CARTESIAN_POINT('Ctrl Pts',(-8.60351383613661,17.6851095950187,3.93781668766136));
#88325=CARTESIAN_POINT('Ctrl Pts',(-8.60501196209861,17.6848404382733,3.94256686818767));
#88326=CARTESIAN_POINT('Ctrl Pts',(-8.60843085066892,17.6842377340939,3.95321744790083));
#88327=CARTESIAN_POINT('Ctrl Pts',(-8.61036495403166,17.6839046264723,3.9591134860673));
#88328=CARTESIAN_POINT('Ctrl Pts',(-8.6153880054529,17.683059028771,3.97410348257388));
#88329=CARTESIAN_POINT('Ctrl Pts',(-8.6185291049438,17.6825482467557,3.98317973840741));
#88330=CARTESIAN_POINT('Ctrl Pts',(-8.6379644586361,17.6794920708317,4.03759919658659));
#88331=CARTESIAN_POINT('Ctrl Pts',(-8.6564012139647,17.6770183582863,4.08214828575086));
#88332=CARTESIAN_POINT('Ctrl Pts',(-8.73510654454,17.6677689893309,4.24856225075011));
#88333=CARTESIAN_POINT('Ctrl Pts',(-8.81002895951557,17.6614651798074,4.36270683062671));
#88334=CARTESIAN_POINT('Ctrl Pts',(-8.91911828506474,17.6530278511486,4.48711831444707));
#88335=CARTESIAN_POINT('Ctrl Pts',(-8.9392959813472,17.6514884948445,4.50876885197372));
#88336=CARTESIAN_POINT('Ctrl Pts',(-8.96426060298913,17.6495875407139,4.53397817676267));
#88337=CARTESIAN_POINT('Ctrl Pts',(-8.96843185532628,17.6492700307065,4.5381397444796));
#88338=CARTESIAN_POINT('Ctrl Pts',(-8.97494986446247,17.6487738467438,4.54456454955388));
#88339=CARTESIAN_POINT('Ctrl Pts',(-8.97727929380474,17.6485965105091,4.54684537313068));
#88340=CARTESIAN_POINT('Ctrl Pts',(-8.98161443411119,17.6482664229571,4.55106177675149));
#88341=CARTESIAN_POINT('Ctrl Pts',(-8.98361806431465,17.6481138348071,4.55299942060114));
#88342=CARTESIAN_POINT('Ctrl Pts',(-8.98817779696077,17.6477665290395,4.55738384692001));
#88343=CARTESIAN_POINT('Ctrl Pts',(-8.99073723378629,17.6475715465466,4.55982707951923));
#88344=CARTESIAN_POINT('Ctrl Pts',(-8.9985530973578,17.6469760853124,4.56723409831569));
#88345=CARTESIAN_POINT('Ctrl Pts',(-9.00383738690238,17.6465734479188,4.57216815999237));
#88346=CARTESIAN_POINT('Ctrl Pts',(-9.05416188240701,17.6427404158983,4.61846409589018));
#88347=CARTESIAN_POINT('Ctrl Pts',(-9.10171217327623,17.6391317510532,4.65700005529325));
#88348=CARTESIAN_POINT('Ctrl Pts',(-9.22323811343783,17.6302030209578,4.74347065517678));
#88349=CARTESIAN_POINT('Ctrl Pts',(-9.29941152893627,17.624854729779,4.78792696285389));
#88350=CARTESIAN_POINT('Ctrl Pts',(-9.43014256999832,17.6163708146461,4.84917364584562));
#88351=CARTESIAN_POINT('Ctrl Pts',(-9.48250758203226,17.6131349431901,4.87011305201036));
#88352=CARTESIAN_POINT('Ctrl Pts',(-9.54948642130707,17.6092044557011,4.89250613356463));
#88353=CARTESIAN_POINT('Ctrl Pts',(-9.5630836262307,17.6084168115938,4.89683210129315));
#88354=CARTESIAN_POINT('Ctrl Pts',(-9.58305907327476,17.6072743308619,4.90286708486127));
#88355=CARTESIAN_POINT('Ctrl Pts',(-9.5893887856905,17.6069144364822,4.90473279553286));
#88356=CARTESIAN_POINT('Ctrl Pts',(-9.60056225899826,17.6062828228035,4.9079442498121));
#88357=CARTESIAN_POINT('Ctrl Pts',(-9.60540070734563,17.6060105270658,4.90930795734217));
#88358=CARTESIAN_POINT('Ctrl Pts',(-9.61485246839317,17.6054809339384,4.91191942654198));
#88359=CARTESIAN_POINT('Ctrl Pts',(-9.61946505154907,17.6052235626942,4.91316957294662));
#88360=CARTESIAN_POINT('Ctrl Pts',(-9.63189308756626,17.6045329590859,4.91647267721811));
#88361=CARTESIAN_POINT('Ctrl Pts',(-9.639719620246,17.6041010790802,4.9184835549955));
#88362=CARTESIAN_POINT('Ctrl Pts',(-9.66884158486058,17.6025049679884,4.92570930729709));
#88363=CARTESIAN_POINT('Ctrl Pts',(-9.69023728368727,17.6013539024372,4.93051041619764));
#88364=CARTESIAN_POINT('Ctrl Pts',(-9.83321543457981,17.5937893420194,4.95923565003717));
#88365=CARTESIAN_POINT('Ctrl Pts',(-9.957299462264,17.5878883868208,4.96811566504678));
#88366=CARTESIAN_POINT('Ctrl Pts',(-10.1304558421928,17.5794000935249,4.95851451678677));
#88367=CARTESIAN_POINT('Ctrl Pts',(-10.1797142162176,17.5769486768567,4.95326717481122));
#88368=CARTESIAN_POINT('Ctrl Pts',(-10.2521736082169,17.5731731433739,4.94180786873347));
#88369=CARTESIAN_POINT('Ctrl Pts',(-10.2756428542167,17.5719233564681,4.9375055985162));
#88370=CARTESIAN_POINT('Ctrl Pts',(-10.3044074310637,17.5703469432101,4.93150233513576));
#88371=CARTESIAN_POINT('Ctrl Pts',(-10.309813259346,17.5700487251547,4.93034211360473));
#88372=CARTESIAN_POINT('Ctrl Pts',(-10.3183182907482,17.569576267359,4.92846625171156));
#88373=CARTESIAN_POINT('Ctrl Pts',(-10.3214220135591,17.5694031666901,4.92777107944794));
#88374=CARTESIAN_POINT('Ctrl Pts',(-10.3272526413961,17.5690766460578,4.92644515932871));
#88375=CARTESIAN_POINT('Ctrl Pts',(-10.3299800164562,17.5689233561522,4.92581670356375));
#88376=CARTESIAN_POINT('Ctrl Pts',(-10.3362090010159,17.5685720058649,4.9243625594138));
#88377=CARTESIAN_POINT('Ctrl Pts',(-10.3397093774856,17.5683736595702,4.92353178092481));
#88378=CARTESIAN_POINT('Ctrl Pts',(-10.3489986291461,17.5678449511419,4.92129085924924));
#88379=CARTESIAN_POINT('Ctrl Pts',(-10.3547819553959,17.5675133682873,4.91985827158666));
#88380=CARTESIAN_POINT('Ctrl Pts',(-10.3962846576127,17.5651172426492,4.90930824305567));
#88381=CARTESIAN_POINT('Ctrl Pts',(-10.4316543743009,17.5629868948466,4.89888002205068));
#88382=CARTESIAN_POINT('Ctrl Pts',(-10.4740090227203,17.5603580698054,4.88463315418522));
#88383=CARTESIAN_POINT('Ctrl Pts',(-10.4814081602794,17.5598958869296,4.88207803891197));
#88384=CARTESIAN_POINT('Ctrl Pts',(-10.5738298382263,17.5540886316416,4.84933020041805));
#88385=CARTESIAN_POINT('Ctrl Pts',(-10.6559048637199,17.5485832701968,4.81139706520054));
#88386=CARTESIAN_POINT('Ctrl Pts',(-10.799984597677,17.5386954894317,4.72787618470692));
#88387=CARTESIAN_POINT('Ctrl Pts',(-10.8629157447394,17.5342835172413,4.68449759238966));
#88388=CARTESIAN_POINT('Ctrl Pts',(-10.930957353166,17.5294327267869,4.6292822165174));
#88389=CARTESIAN_POINT('Ctrl Pts',(-10.9396484202009,17.5288112897752,4.62206094951987));
#88390=CARTESIAN_POINT('Ctrl Pts',(-10.952833039658,17.5278655176554,4.61084543035098));
#88391=CARTESIAN_POINT('Ctrl Pts',(-10.9573869321956,17.5275382868186,4.60692304843774));
#88392=CARTESIAN_POINT('Ctrl Pts',(-10.9656262254777,17.5269451510172,4.59973745541037));
#88393=CARTESIAN_POINT('Ctrl Pts',(-10.9693195553986,17.5266788720254,4.59648350580626));
#88394=CARTESIAN_POINT('Ctrl Pts',(-10.9773256792928,17.5261007403383,4.58935777227946));
#88395=CARTESIAN_POINT('Ctrl Pts',(-10.981632043298,17.5257891895024,4.58547886774723));
#88396=CARTESIAN_POINT('Ctrl Pts',(-10.9933223423192,17.5249417548551,4.57482250964639));
#88397=CARTESIAN_POINT('Ctrl Pts',(-11.0006599533003,17.5244079982775,4.5679945540802));
#88398=CARTESIAN_POINT('Ctrl Pts',(-11.0375756975071,17.521712250289,4.53292842725173));
#88399=CARTESIAN_POINT('Ctrl Pts',(-11.0660324666245,17.5196005097642,4.50353357470093));
#88400=CARTESIAN_POINT('Ctrl Pts',(-11.1022345768859,17.5168433420942,4.462857692943));
#88401=CARTESIAN_POINT('Ctrl Pts',(-11.1111056863723,17.5161615391143,4.45260703573738));
#88402=CARTESIAN_POINT('Ctrl Pts',(-11.1845009977094,17.5104605487613,4.36537767396796));
#88403=CARTESIAN_POINT('Ctrl Pts',(-11.241082235174,17.5056887480822,4.282071235387));
#88404=CARTESIAN_POINT('Ctrl Pts',(-11.3137233050653,17.4981232185244,4.14711201045561));
#88405=CARTESIAN_POINT('Ctrl Pts',(-11.3362213109601,17.4954650164465,4.09927827994936));
#88406=CARTESIAN_POINT('Ctrl Pts',(-11.3599703610437,17.4921239996376,4.04075849799416));
#88407=CARTESIAN_POINT('Ctrl Pts',(-11.3637563742515,17.4915719389034,4.03113809474442));
#88408=CARTESIAN_POINT('Ctrl Pts',(-11.3688971448324,17.4907934175572,4.01765778190089));
#88409=CARTESIAN_POINT('Ctrl Pts',(-11.3703382141775,17.4905718491006,4.01383085761642));
#88410=CARTESIAN_POINT('Ctrl Pts',(-11.3727625386571,17.4901932911696,4.00731004933062));
#88411=CARTESIAN_POINT('Ctrl Pts',(-11.3737539616162,17.4900367814853,4.00461918960409));
#88412=CARTESIAN_POINT('Ctrl Pts',(-11.37564102332,17.4897355675442,3.99945066411598));
#88413=CARTESIAN_POINT('Ctrl Pts',(-11.3765378879962,17.4895909413184,3.99697347374855));
#88414=CARTESIAN_POINT('Ctrl Pts',(-11.3789060998942,17.4892051405479,3.99037674620755));
#88415=CARTESIAN_POINT('Ctrl Pts',(-11.3803656621054,17.4889632850971,3.98625304463578));
#88416=CARTESIAN_POINT('Ctrl Pts',(-11.3855398127446,17.4880912300412,3.97142347368022));
#88417=CARTESIAN_POINT('Ctrl Pts',(-11.3891484184817,17.4874552490466,3.96068136443337));
#88418=CARTESIAN_POINT('Ctrl Pts',(-11.416662355422,17.4823852448033,3.87551379928805));
#88419=CARTESIAN_POINT('Ctrl Pts',(-11.4346925467503,17.4776902797076,3.79932930308715));
#88420=CARTESIAN_POINT('Ctrl Pts',(-11.4577793617561,17.4685288148826,3.64894812463189));
#88421=CARTESIAN_POINT('Ctrl Pts',(-11.4634454599711,17.4640771657698,3.57506731411596));
#88422=CARTESIAN_POINT('Ctrl Pts',(-11.4634998694394,17.4597393327923,3.50071396372807));
#88423=CARTESIAN_POINT('Ctrl Pts',(-11.4635,17.4597185093157,3.5003569817236));
#88424=CARTESIAN_POINT('Ctrl Pts',(-11.4635,17.4596976889334,3.50000000000147));
#88425=CARTESIAN_POINT('Ctrl Pts',(-11.4635,17.3900944100234,3.49999999998336));
#88426=CARTESIAN_POINT('Ctrl Pts',(-11.4635,17.3901118316435,3.50035017971462));
#88427=CARTESIAN_POINT('Ctrl Pts',(-11.4634998743219,17.3901292509645,3.50070036152164));
#88428=CARTESIAN_POINT('Ctrl Pts',(-11.4634232107731,17.3954410713135,3.60749892398405));
#88429=CARTESIAN_POINT('Ctrl Pts',(-11.4517336778086,17.4004712680935,3.71361410049286));
#88430=CARTESIAN_POINT('Ctrl Pts',(-11.4265572899447,17.4062653768113,3.82689258636057));
#88431=CARTESIAN_POINT('Ctrl Pts',(-11.4243816898007,17.4067472219701,3.83624583449666));
#88432=CARTESIAN_POINT('Ctrl Pts',(-11.4135765864115,17.4090570377892,3.88071088108472));
#88433=CARTESIAN_POINT('Ctrl Pts',(-11.4037405105374,17.4109219057271,3.91551379594425));
#88434=CARTESIAN_POINT('Ctrl Pts',(-11.3908044029715,17.4131714204938,3.95555516354608));
#88435=CARTESIAN_POINT('Ctrl Pts',(-11.3889476865259,17.4134901425403,3.96118512126444));
#88436=CARTESIAN_POINT('Ctrl Pts',(-11.3859119343481,17.414004946086,3.97020553439422));
#88437=CARTESIAN_POINT('Ctrl Pts',(-11.3847545215386,17.4141998053295,3.97360326103394));
#88438=CARTESIAN_POINT('Ctrl Pts',(-11.3826724427108,17.414547904469,3.97964257435268));
#88439=CARTESIAN_POINT('Ctrl Pts',(-11.3817526860329,17.4147008560748,3.98228580478788));
#88440=CARTESIAN_POINT('Ctrl Pts',(-11.3797691210174,17.4150289910918,3.9879339952793));
#88441=CARTESIAN_POINT('Ctrl Pts',(-11.378703092195,17.4152042991161,3.99093807576274));
#88442=CARTESIAN_POINT('Ctrl Pts',(-11.3757515294863,17.4156868029366,3.99917017810984));
#88443=CARTESIAN_POINT('Ctrl Pts',(-11.373846036362,17.4159951399575,4.0043909237259));
#88444=CARTESIAN_POINT('Ctrl Pts',(-11.3634697797325,17.4176569957082,4.03232515171355));
#88445=CARTESIAN_POINT('Ctrl Pts',(-11.3544658479301,17.4190390050037,4.05483514030286));
#88446=CARTESIAN_POINT('Ctrl Pts',(-11.3248763417866,17.423383834201,4.12379109733525));
#88447=CARTESIAN_POINT('Ctrl Pts',(-11.3024292909585,17.4264157589203,4.16939523533212));
#88448=CARTESIAN_POINT('Ctrl Pts',(-11.2134287976125,17.4373835713428,4.32871474393081));
#88449=CARTESIAN_POINT('Ctrl Pts',(-11.1339572335214,17.4453196294646,4.43452212936244));
#88450=CARTESIAN_POINT('Ctrl Pts',(-11.0305686817836,17.4535245710539,4.53922929663182));
#88451=CARTESIAN_POINT('Ctrl Pts',(-11.0195775655764,17.4543756868927,4.55001473898854));
#88452=CARTESIAN_POINT('Ctrl Pts',(-11.0039785927214,17.4555548920237,4.5648458852139));
#88453=CARTESIAN_POINT('Ctrl Pts',(-10.9995127015503,17.4558892900867,4.56903888373531));
#88454=CARTESIAN_POINT('Ctrl Pts',(-10.9912871632337,17.4564994221153,4.57666518926656));
#88455=CARTESIAN_POINT('Ctrl Pts',(-10.9875356899264,17.4567755207186,4.58010713903906));
#88456=CARTESIAN_POINT('Ctrl Pts',(-10.9799015531358,17.4573330368785,4.58703838242448));
#88457=CARTESIAN_POINT('Ctrl Pts',(-10.9760180279437,17.4576144081816,4.59052661994265));
#88458=CARTESIAN_POINT('Ctrl Pts',(-10.9663976867104,17.4583059808391,4.5990751917334));
#88459=CARTESIAN_POINT('Ctrl Pts',(-10.9606396642389,17.4587151838444,4.6041115000149));
#88460=CARTESIAN_POINT('Ctrl Pts',(-10.9391536579251,17.4602250190152,4.62260911289105));
#88461=CARTESIAN_POINT('Ctrl Pts',(-10.9231796797913,17.461313912191,4.63578173463947));
#88462=CARTESIAN_POINT('Ctrl Pts',(-10.8262236512845,17.4677373760064,4.71233715438699));
#88463=CARTESIAN_POINT('Ctrl Pts',(-10.7390244388223,17.4727330272248,4.76738001320493));
#88464=CARTESIAN_POINT('Ctrl Pts',(-10.5681313606736,17.4819959013363,4.85157077544888));
#88465=CARTESIAN_POINT('Ctrl Pts',(-10.4861818901234,17.4862531774624,4.88316316703846));
#88466=CARTESIAN_POINT('Ctrl Pts',(-10.3910954852738,17.4914700777515,4.91032020450472));
#88467=CARTESIAN_POINT('Ctrl Pts',(-10.380245438761,17.4920694113205,4.91328417128766));
#88468=CARTESIAN_POINT('Ctrl Pts',(-10.3651422310072,17.4929106292886,4.91722349145991));
#88469=CARTESIAN_POINT('Ctrl Pts',(-10.3609169759793,17.4931467182116,4.91830540049501));
#88470=CARTESIAN_POINT('Ctrl Pts',(-10.3541336692455,17.4935270337457,4.92001004416762));
#88471=CARTESIAN_POINT('Ctrl Pts',(-10.3515786297263,17.4936705792308,4.9206448001254));
#88472=CARTESIAN_POINT('Ctrl Pts',(-10.3462336226318,17.4939715083602,4.9219573734681));
#88473=CARTESIAN_POINT('Ctrl Pts',(-10.3434433669256,17.4941289684383,4.92263387652933));
#88474=CARTESIAN_POINT('Ctrl Pts',(-10.3366606061746,17.4945125933328,4.92425725313198));
#88475=CARTESIAN_POINT('Ctrl Pts',(-10.3326660877724,17.4947392400125,4.925195551515));
#88476=CARTESIAN_POINT('Ctrl Pts',(-10.3185117594551,17.4955447689318,4.92845760562177));
#88477=CARTESIAN_POINT('Ctrl Pts',(-10.3083313731042,17.496128545168,4.93068956228364));
#88478=CARTESIAN_POINT('Ctrl Pts',(-10.2455902909537,17.4997496787971,4.94374423138855));
#88479=CARTESIAN_POINT('Ctrl Pts',(-10.1924952005466,17.5029132940792,4.95177703559117));
#88480=CARTESIAN_POINT('Ctrl Pts',(-10.0456223210248,17.5117337608868,4.9657986311013));
#88481=CARTESIAN_POINT('Ctrl Pts',(-9.95150994499491,17.517447464102,4.96570733375202));
#88482=CARTESIAN_POINT('Ctrl Pts',(-9.80019365985088,17.5263611925037,4.9509614905418));
#88483=CARTESIAN_POINT('Ctrl Pts',(-9.74271634377965,17.5296864863694,4.94188010459113));
#88484=CARTESIAN_POINT('Ctrl Pts',(-9.67604753182678,17.5334646805047,4.92723135503667));
#88485=CARTESIAN_POINT('Ctrl Pts',(-9.66619180273169,17.5340212531672,4.92495846855044));
#88486=CARTESIAN_POINT('Ctrl Pts',(-9.65017652801991,17.5349226063282,4.92108981353197));
#88487=CARTESIAN_POINT('Ctrl Pts',(-9.6440025453729,17.5352693387079,4.91955575225472));
#88488=CARTESIAN_POINT('Ctrl Pts',(-9.63299648130918,17.5358861620822,4.91674473486965));
#88489=CARTESIAN_POINT('Ctrl Pts',(-9.62816059589988,17.5361567412584,4.91548319839224));
#88490=CARTESIAN_POINT('Ctrl Pts',(-9.61794993275202,17.5367271488579,4.91276360682446));
#88491=CARTESIAN_POINT('Ctrl Pts',(-9.61257681493703,17.5370267811562,4.91129959239862));
#88492=CARTESIAN_POINT('Ctrl Pts',(-9.5982955130578,17.537821831745,4.90732065745172));
#88493=CARTESIAN_POINT('Ctrl Pts',(-9.58940252946597,17.5383155091124,4.90475181089187));
#88494=CARTESIAN_POINT('Ctrl Pts',(-9.54677043447824,17.5406760592543,4.89199757467937));
#88495=CARTESIAN_POINT('Ctrl Pts',(-9.51338085990163,17.5425060392056,4.88067967296219));
#88496=CARTESIAN_POINT('Ctrl Pts',(-9.37419781118695,17.5500997038759,4.82782408244247));
#88497=CARTESIAN_POINT('Ctrl Pts',(-9.27302938255267,17.5554988953047,4.77524864099147));
#88498=CARTESIAN_POINT('Ctrl Pts',(-9.12513788524783,17.5642702890941,4.67502166454493));
#88499=CARTESIAN_POINT('Ctrl Pts',(-9.07381148279971,17.5675211284077,4.63500333362759));
#88500=CARTESIAN_POINT('Ctrl Pts',(-9.0199042704289,17.5713762511422,4.58687503687647));
#88501=CARTESIAN_POINT('Ctrl Pts',(-9.01452338673882,17.5717663172343,4.58199853293749));
#88502=CARTESIAN_POINT('Ctrl Pts',(-9.00656977660599,17.5723511494341,4.5746819119016));
#88503=CARTESIAN_POINT('Ctrl Pts',(-9.00396918328724,17.5725437053308,4.57227208866901));
#88504=CARTESIAN_POINT('Ctrl Pts',(-8.9993387550151,17.5728890007823,4.56794995198253));
#88505=CARTESIAN_POINT('Ctrl Pts',(-8.99730560421565,17.5730414665856,4.56604126358206));
#88506=CARTESIAN_POINT('Ctrl Pts',(-8.9929096653069,17.5733729821718,4.56189072697876));
#88507=CARTESIAN_POINT('Ctrl Pts',(-8.99054893467253,17.5735521854983,4.55964683010825));
#88508=CARTESIAN_POINT('Ctrl Pts',(-8.98395114377067,17.5740562661145,4.55333351071517));
#88509=CARTESIAN_POINT('Ctrl Pts',(-8.97973111711057,17.574382455711,4.54924647593237));
#88510=CARTESIAN_POINT('Ctrl Pts',(-8.95464460600604,17.5763435820412,4.52465611233313));
#88511=CARTESIAN_POINT('Ctrl Pts',(-8.93437342704047,17.5780201598257,4.50355758071698));
#88512=CARTESIAN_POINT('Ctrl Pts',(-8.82645584321613,17.5873963767549,4.38427710832873));
#88513=CARTESIAN_POINT('Ctrl Pts',(-8.75172550222423,17.5955351852506,4.27522152949078));
#88514=CARTESIAN_POINT('Ctrl Pts',(-8.6858230676814,17.6040902584944,4.14420280271838));
#88515=CARTESIAN_POINT('Ctrl Pts',(-8.67927480077941,17.6049616629923,4.13066887432615));
#88516=CARTESIAN_POINT('Ctrl Pts',(-8.65651336366731,17.6080686923473,4.08171569292694));
#88517=CARTESIAN_POINT('Ctrl Pts',(-8.64150633373492,17.6102674235222,4.04575163792697));
#88518=CARTESIAN_POINT('Ctrl Pts',(-8.62451288263724,17.6129639794557,3.99996508175568));
#88519=CARTESIAN_POINT('Ctrl Pts',(-8.62116845990515,17.6135064680905,3.99066636707362));
#88520=CARTESIAN_POINT('Ctrl Pts',(-8.61602252330961,17.6143605062135,3.97589055785633));
#88521=CARTESIAN_POINT('Ctrl Pts',(-8.61415879484026,17.6146740931979,3.97043557949224));
#88522=CARTESIAN_POINT('Ctrl Pts',(-8.61074723463179,17.6152562600888,3.96025399322193));
#88523=CARTESIAN_POINT('Ctrl Pts',(-8.60919117785093,17.615525105987,3.9555302464576));
#88524=CARTESIAN_POINT('Ctrl Pts',(-8.60578839601599,17.6161205256032,3.94502038301076));
#88525=CARTESIAN_POINT('Ctrl Pts',(-8.60395354374617,17.6164467085272,3.93923049926078));
#88526=CARTESIAN_POINT('Ctrl Pts',(-8.59872036833839,17.6173923032128,3.92235307708058));
#88527=CARTESIAN_POINT('Ctrl Pts',(-8.59541767493327,17.6180086133816,3.91123622194467));
#88528=CARTESIAN_POINT('Ctrl Pts',(-8.56747824567873,17.6234039610684,3.81292663561796));
#88529=CARTESIAN_POINT('Ctrl Pts',(-8.55085475199813,17.6279072818749,3.72365695569299));
#88530=CARTESIAN_POINT('Ctrl Pts',(-8.533580578868,17.6371570833504,3.53495418990895));
#88531=CARTESIAN_POINT('Ctrl Pts',(-8.53456894239786,17.6418671210789,3.43584470829085));
#88532=CARTESIAN_POINT('Ctrl Pts',(-8.54807202494477,17.6481363896877,3.31490854797101));
#88533=CARTESIAN_POINT('Ctrl Pts',(-8.55113658133171,17.6493331163671,3.29227814268081));
#88534=CARTESIAN_POINT('Ctrl Pts',(-8.55561816506595,17.6508601616528,3.26414985019038));
#88535=CARTESIAN_POINT('Ctrl Pts',(-8.55653952240296,17.6511647629068,3.25857501004589));
#88536=CARTESIAN_POINT('Ctrl Pts',(-8.55804020900779,17.6516469034471,3.24981063341906));
#88537=CARTESIAN_POINT('Ctrl Pts',(-8.55859790152844,17.6518232524112,3.24661738794344));
#88538=CARTESIAN_POINT('Ctrl Pts',(-8.55965541389894,17.6521525344702,3.2406787507769));
#88539=CARTESIAN_POINT('Ctrl Pts',(-8.56015247923612,17.6523053123376,3.23793292164641));
#88540=CARTESIAN_POINT('Ctrl Pts',(-8.56130283555837,17.6526544038414,3.23168033414738));
#88541=CARTESIAN_POINT('Ctrl Pts',(-8.56196109393796,17.6528509930842,3.22817454469519));
#88542=CARTESIAN_POINT('Ctrl Pts',(-8.56401891739766,17.6534559626331,3.21743157247173));
#88543=CARTESIAN_POINT('Ctrl Pts',(-8.56546032705713,17.6538666005006,3.21020264331594));
#88544=CARTESIAN_POINT('Ctrl Pts',(-8.5689306762007,17.6548254945706,3.19345883145994));
#88545=CARTESIAN_POINT('Ctrl Pts',(-8.57099998959353,17.6553757334034,3.18395275969089));
#88546=CARTESIAN_POINT('Ctrl Pts',(-8.57849725574626,17.6572964512541,3.15109153798487));
#88547=CARTESIAN_POINT('Ctrl Pts',(-8.58440407701065,17.6586875463456,3.12785051971576));
#88548=CARTESIAN_POINT('Ctrl Pts',(-8.61956688884625,17.6663328876613,3.00248503434452));
#88549=CARTESIAN_POINT('Ctrl Pts',(-8.65930538374638,17.6728484501436,2.9036308438086));
#88550=CARTESIAN_POINT('Ctrl Pts',(-8.74220046611629,17.6832461170692,2.74859271691442));
#88551=CARTESIAN_POINT('Ctrl Pts',(-8.7793407174693,17.6872548381788,2.68965089974101));
#88552=CARTESIAN_POINT('Ctrl Pts',(-8.82672939338587,17.6916886023975,2.62514133882135));
#88553=CARTESIAN_POINT('Ctrl Pts',(-8.83301031450446,17.6922643482836,2.61678050558614));
#88554=CARTESIAN_POINT('Ctrl Pts',(-8.8432762975806,17.6931866248221,2.60341568834927));
#88555=CARTESIAN_POINT('Ctrl Pts',(-8.84720541888654,17.6935353165691,2.59836936209461));
#88556=CARTESIAN_POINT('Ctrl Pts',(-8.85427438624654,17.6941551124248,2.58941215777186));
#88557=CARTESIAN_POINT('Ctrl Pts',(-8.8574014761455,17.6944267128967,2.58549138080646));
#88558=CARTESIAN_POINT('Ctrl Pts',(-8.86399630381798,17.6949941681164,2.57730935074074));
#88559=CARTESIAN_POINT('Ctrl Pts',(-8.86746801186787,17.6952898587108,2.57305138817842));
#88560=CARTESIAN_POINT('Ctrl Pts',(-8.8766369162829,17.6960629488439,2.56193436571817));
#88561=CARTESIAN_POINT('Ctrl Pts',(-8.88237301143417,17.6965387770117,2.55510758747513));
#88562=CARTESIAN_POINT('Ctrl Pts',(-8.90865565954354,17.6986845061437,2.52440165625672));
#88563=CARTESIAN_POINT('Ctrl Pts',(-8.92990829573542,17.7003253466624,2.50113638001455));
#88564=CARTESIAN_POINT('Ctrl Pts',(-8.9904530631839,17.7047702522717,2.43901030343049));
#88565=CARTESIAN_POINT('Ctrl Pts',(-9.03122073871089,17.7075139161828,2.40165964840001));
#88566=CARTESIAN_POINT('Ctrl Pts',(-9.13563208172349,17.7141199661283,2.31634724544742));
#88567=CARTESIAN_POINT('Ctrl Pts',(-9.20126134074058,17.7179283050911,2.27110560290923));
#88568=CARTESIAN_POINT('Ctrl Pts',(-9.31230364533523,17.7243025098907,2.20722746515281));
#88569=CARTESIAN_POINT('Ctrl Pts',(-9.35554082193359,17.7267714388952,2.18513932948893));
#88570=CARTESIAN_POINT('Ctrl Pts',(-9.40611147556573,17.7297316157522,2.16239889929933));
#88571=CARTESIAN_POINT('Ctrl Pts',(-9.4124524456134,17.7301040600874,2.15960149522739));
#88572=CARTESIAN_POINT('Ctrl Pts',(-9.42204864971335,17.7306699624267,2.15544917650193));
#88573=CARTESIAN_POINT('Ctrl Pts',(-9.42528939379872,17.7308614600435,2.15406077445715));
#88574=CARTESIAN_POINT('Ctrl Pts',(-9.43110111608624,17.7312056225211,2.15159572866431));
#88575=CARTESIAN_POINT('Ctrl Pts',(-9.43367018266171,17.7313580211446,2.15051470667567));
#88576=CARTESIAN_POINT('Ctrl Pts',(-9.43926164896605,17.7316902908853,2.14818068654894));
#88577=CARTESIAN_POINT('Ctrl Pts',(-9.44228512644287,17.731870321579,2.14693049922756));
#88578=CARTESIAN_POINT('Ctrl Pts',(-9.45081215716482,17.7323790230291,2.1434380662092));
#88579=CARTESIAN_POINT('Ctrl Pts',(-9.45632514717821,17.7327090441116,2.14121921603814));
#88580=CARTESIAN_POINT('Ctrl Pts',(-9.4902068885551,17.7347435125991,2.12782181136136));
#88581=CARTESIAN_POINT('Ctrl Pts',(-9.51890391212215,17.7364932168763,2.11749926359997));
#88582=CARTESIAN_POINT('Ctrl Pts',(-9.68976715258485,17.7469809485578,2.06200231590536));
#88583=CARTESIAN_POINT('Ctrl Pts',(-9.83785353769738,17.7562366134552,2.03787712513248));
#88584=CARTESIAN_POINT('Ctrl Pts',(-10.022750255126,17.7668392697681,2.03624148279399));
#88585=CARTESIAN_POINT('Ctrl Pts',(-10.0584480154951,17.7688493976806,2.037231832681));
#88586=CARTESIAN_POINT('Ctrl Pts',(-10.1036437061987,17.7713484283084,2.04014310637531));
#88587=CARTESIAN_POINT('Ctrl Pts',(-10.1132051167827,17.7718745279285,2.04085340853659));
#88588=CARTESIAN_POINT('Ctrl Pts',(-10.1284356838471,17.772708569787,2.04213547338658));
#88589=CARTESIAN_POINT('Ctrl Pts',(-10.1341095636404,17.7730183929772,2.04264646394079));
#88590=CARTESIAN_POINT('Ctrl Pts',(-10.1447365703374,17.7735970653998,2.04366612164185));
#88591=CARTESIAN_POINT('Ctrl Pts',(-10.1496903513523,17.7738661541973,2.04416696025721));
#88592=CARTESIAN_POINT('Ctrl Pts',(-10.1607695559939,17.7744665366552,2.04534424117778));
#88593=CARTESIAN_POINT('Ctrl Pts',(-10.1668934776774,17.7747974066536,2.04603411473797));
#88594=CARTESIAN_POINT('Ctrl Pts',(-10.1849565524343,17.7757705348163,2.04818458616306));
#88595=CARTESIAN_POINT('Ctrl Pts',(-10.1968824234658,17.7764094028898,2.04975372955319));
#88596=CARTESIAN_POINT('Ctrl Pts',(-10.3145222023831,17.7826786809046,2.06671005826602));
#88597=CARTESIAN_POINT('Ctrl Pts',(-10.4182719623035,17.7879136466969,2.09348082910684));
#88598=CARTESIAN_POINT('Ctrl Pts',(-10.6086148518675,17.797810547104,2.16554568724975));
#88599=CARTESIAN_POINT('Ctrl Pts',(-10.6954106355574,17.802467316993,2.20865197085244));
#88600=CARTESIAN_POINT('Ctrl Pts',(-10.7865368028056,17.8081459059013,2.26577527437407));
#88601=CARTESIAN_POINT('Ctrl Pts',(-10.7956976482237,17.8087264481061,2.27166126244881));
#88602=CARTESIAN_POINT('Ctrl Pts',(-10.8083954067449,17.8095459718198,2.28002142120657));
#88603=CARTESIAN_POINT('Ctrl Pts',(-10.8119885673194,17.8097795586055,2.28240999020734));
#88604=CARTESIAN_POINT('Ctrl Pts',(-10.8179436068104,17.8101695823702,2.28640671123506));
#88605=CARTESIAN_POINT('Ctrl Pts',(-10.8203114573716,17.8103254300458,2.28800597069467));
#88606=CARTESIAN_POINT('Ctrl Pts',(-10.8250403624105,17.8106382457493,2.29122010571193));
#88607=CARTESIAN_POINT('Ctrl Pts',(-10.8274013960218,17.8107952141674,2.29283498973477));
#88608=CARTESIAN_POINT('Ctrl Pts',(-10.8332399417959,17.8111852997872,2.29685357484579));
#88609=CARTESIAN_POINT('Ctrl Pts',(-10.8367117792895,17.8114189582012,2.2992654254785));
#88610=CARTESIAN_POINT('Ctrl Pts',(-10.8441874103144,17.8119256661923,2.30450683688911));
#88611=CARTESIAN_POINT('Ctrl Pts',(-10.8481875217635,17.8121990415199,2.30734153533154));
#88612=CARTESIAN_POINT('Ctrl Pts',(-10.9042380773631,17.8160604130468,2.34748662992855));
#88613=CARTESIAN_POINT('Ctrl Pts',(-10.9537939315528,17.8198464211563,2.38815064265674));
#88614=CARTESIAN_POINT('Ctrl Pts',(-11.0526219357131,17.8279614156668,2.48072793096994));
#88615=CARTESIAN_POINT('Ctrl Pts',(-11.1010830048244,17.8322899445141,2.53328114616172));
#88616=CARTESIAN_POINT('Ctrl Pts',(-11.1918909404484,17.8409473916704,2.64748570978296));
#88617=CARTESIAN_POINT('Ctrl Pts',(-11.2337491099602,17.8452543222788,2.70927222607752));
#88618=CARTESIAN_POINT('Ctrl Pts',(-11.2759690350652,17.8499696596895,2.78316870735907));
#88619=CARTESIAN_POINT('Ctrl Pts',(-11.2811154986643,17.8505520234833,2.79240748457018));
#88620=CARTESIAN_POINT('Ctrl Pts',(-11.2892296449729,17.8514827883663,2.80735252733558));
#88621=CARTESIAN_POINT('Ctrl Pts',(-11.2922605761713,17.8518334148956,2.81302386942059));
#88622=CARTESIAN_POINT('Ctrl Pts',(-11.2975909164472,17.8524554171044,2.82315787441935));
#88623=CARTESIAN_POINT('Ctrl Pts',(-11.2999049141898,17.852727301782,2.82761271253535));
#88624=CARTESIAN_POINT('Ctrl Pts',(-11.3046952994113,17.8532941181707,2.83695217650359));
#88625=CARTESIAN_POINT('Ctrl Pts',(-11.3071672861186,17.8535888933793,2.84183898036212));
#88626=CARTESIAN_POINT('Ctrl Pts',(-11.3135565241108,17.8543568766343,2.85464768788544));
#88627=CARTESIAN_POINT('Ctrl Pts',(-11.3174295860666,17.8548285517584,2.8625914660458));
#88628=CARTESIAN_POINT('Ctrl Pts',(-11.3344312558645,17.8569275597156,2.89827950674739));
#88629=CARTESIAN_POINT('Ctrl Pts',(-11.3467575681557,17.8585273990875,2.92639860804597));
#88630=CARTESIAN_POINT('Ctrl Pts',(-11.3779860108728,17.862827697885,3.00420653259897));
#88631=CARTESIAN_POINT('Ctrl Pts',(-11.3950807055843,17.8654727992214,3.05457097368899));
#88632=CARTESIAN_POINT('Ctrl Pts',(-11.4422329324372,17.8740621023824,3.22313749027782));
#88633=CARTESIAN_POINT('Ctrl Pts',(-11.460270395434,17.8797855169432,3.34414361695665));
#88634=CARTESIAN_POINT('Ctrl Pts',(-11.4633680666843,17.8867754093377,3.47730877028001));
#88635=CARTESIAN_POINT('Ctrl Pts',(-11.4635,17.8873766710606,3.48865438790481));
#88636=CARTESIAN_POINT('Ctrl Pts',(-11.4635,17.8879846534521,3.50000000000001));
#88637=CARTESIAN_POINT('Origin',(-10.,13.2,3.5));
#88638=CARTESIAN_POINT('',(-11.4635,18.4603263886907,3.50000000004768));
#88639=CARTESIAN_POINT('',(-11.4635,18.3899253605917,3.49999999994518));
#88640=CARTESIAN_POINT('',(-11.4635,13.2,3.5));
#88641=CARTESIAN_POINT('',(-11.463499980138,17.9619694309472,3.50024111453588));
#88642=CARTESIAN_POINT('Ctrl Pts',(-11.4635,18.4603263886907,3.50000000004768));
#88643=CARTESIAN_POINT('Ctrl Pts',(-11.4635,18.460305879277,3.49958063693336));
#88644=CARTESIAN_POINT('Ctrl Pts',(-11.4634998197481,18.4602853715295,3.49916126965186));
#88645=CARTESIAN_POINT('Ctrl Pts',(-11.4634249137899,18.4560247057668,3.41202621381093));
#88646=CARTESIAN_POINT('Ctrl Pts',(-11.4556434752369,18.4518825987025,3.32549418675632));
#88647=CARTESIAN_POINT('Ctrl Pts',(-11.4378193502063,18.4468251008909,3.22669595506432));
#88648=CARTESIAN_POINT('Ctrl Pts',(-11.4352005304622,18.4461299873744,3.21326143532275));
#88649=CARTESIAN_POINT('Ctrl Pts',(-11.4272159367172,18.4441323921311,3.17515485567764));
#88650=CARTESIAN_POINT('Ctrl Pts',(-11.4213998510644,18.4428132252866,3.15058332916228));
#88651=CARTESIAN_POINT('Ctrl Pts',(-11.4134598854698,18.4411478132214,3.12052996780278));
#88652=CARTESIAN_POINT('Ctrl Pts',(-11.4119344631874,18.4408331646694,3.11489297263277));
#88653=CARTESIAN_POINT('Ctrl Pts',(-11.4094985223399,18.4403386017206,3.10610032778138));
#88654=CARTESIAN_POINT('Ctrl Pts',(-11.4086110313423,18.44015998106,3.10293829421691));
#88655=CARTESIAN_POINT('Ctrl Pts',(-11.4069512519329,18.439828737345,3.09710028297323));
#88656=CARTESIAN_POINT('Ctrl Pts',(-11.4061819639129,18.4396762872046,3.09442350746303));
#88657=CARTESIAN_POINT('Ctrl Pts',(-11.4044268224553,18.4393308837154,3.08838142973162));
#88658=CARTESIAN_POINT('Ctrl Pts',(-11.4034365171435,18.4391376777022,3.08501748369245));
#88659=CARTESIAN_POINT('Ctrl Pts',(-11.4004128728132,18.4385528517805,3.0748811512526));
#88660=CARTESIAN_POINT('Ctrl Pts',(-11.3983425626439,18.4381591820158,3.06812001286215));
#88661=CARTESIAN_POINT('Ctrl Pts',(-11.3728629401674,18.4333958802512,2.98701385942724));
#88662=CARTESIAN_POINT('Ctrl Pts',(-11.3436016507737,18.4287379334421,2.91464580565684));
#88663=CARTESIAN_POINT('Ctrl Pts',(-11.2527196815604,18.4165204839546,2.73307023446575));
#88664=CARTESIAN_POINT('Ctrl Pts',(-11.1825871214322,18.409007181454,2.62880155910358));
#88665=CARTESIAN_POINT('Ctrl Pts',(-11.0895831235252,18.4011348357045,2.52281435772815));
#88666=CARTESIAN_POINT('Ctrl Pts',(-11.0789425202442,18.4002583535346,2.51107824967673));
#88667=CARTESIAN_POINT('Ctrl Pts',(-11.0637612340603,18.3990407746432,2.49487074824493));
#88668=CARTESIAN_POINT('Ctrl Pts',(-11.0593789778347,18.3986930308012,2.49025302231686));
#88669=CARTESIAN_POINT('Ctrl Pts',(-11.0517189109866,18.3980915581022,2.4822861206325));
#88670=CARTESIAN_POINT('Ctrl Pts',(-11.04845491002,18.3978372425868,2.47892384693884));
#88671=CARTESIAN_POINT('Ctrl Pts',(-11.04161781106,18.3973085991602,2.47194824660048));
#88672=CARTESIAN_POINT('Ctrl Pts',(-11.0380419249297,18.3970343976213,2.46833773211748));
#88673=CARTESIAN_POINT('Ctrl Pts',(-11.0295390167171,18.3963877222697,2.45984145077911));
#88674=CARTESIAN_POINT('Ctrl Pts',(-11.0245958858855,18.3960159626125,2.45497192987823));
#88675=CARTESIAN_POINT('Ctrl Pts',(-11.0080203867486,18.3947830139337,2.43887393179582));
#88676=CARTESIAN_POINT('Ctrl Pts',(-10.9962363865108,18.393928590349,2.4278028528805));
#88677=CARTESIAN_POINT('Ctrl Pts',(-10.9312974310554,18.3893336115024,2.36878776201491));
#88678=CARTESIAN_POINT('Ctrl Pts',(-10.8748609018125,18.3857506221195,2.32459540473324));
#88679=CARTESIAN_POINT('Ctrl Pts',(-10.7602217348753,18.3789751071697,2.2476772451079));
#88680=CARTESIAN_POINT('Ctrl Pts',(-10.7025747185099,18.3757794943974,2.21445032764282));
#88681=CARTESIAN_POINT('Ctrl Pts',(-10.5848150770486,18.3693420686225,2.1568694164821));
#88682=CARTESIAN_POINT('Ctrl Pts',(-10.5249499028337,18.3661096351238,2.13236182701676));
#88683=CARTESIAN_POINT('Ctrl Pts',(-10.4567851587557,18.3622757321086,2.10959277657474));
#88684=CARTESIAN_POINT('Ctrl Pts',(-10.449884208799,18.3618858722579,2.10734457867439));
#88685=CARTESIAN_POINT('Ctrl Pts',(-10.4395892032237,18.3613013292265,2.10407516594304));
#88686=CARTESIAN_POINT('Ctrl Pts',(-10.4362075924814,18.3611088537747,2.10301476541483));
#88687=CARTESIAN_POINT('Ctrl Pts',(-10.4301591372461,18.3607636928539,2.10114220226178));
#88688=CARTESIAN_POINT('Ctrl Pts',(-10.4274937914302,18.3606112808486,2.10032536645806));
#88689=CARTESIAN_POINT('Ctrl Pts',(-10.4217102482266,18.3602798739353,2.0985709727797));
#88690=CARTESIAN_POINT('Ctrl Pts',(-10.418591294329,18.3601007255307,2.09763621706746));
#88691=CARTESIAN_POINT('Ctrl Pts',(-10.4098375950896,18.3595967810701,2.09504452326377));
#88692=CARTESIAN_POINT('Ctrl Pts',(-10.404196022321,18.359270673273,2.0934111051519));
#88693=CARTESIAN_POINT('Ctrl Pts',(-10.3703976567771,18.3573097057194,2.08384550561585));
#88694=CARTESIAN_POINT('Ctrl Pts',(-10.3420198034,18.3556332063853,2.07672553850967));
#88695=CARTESIAN_POINT('Ctrl Pts',(-10.1848960761534,18.3462568893866,2.04227359048706));
#88696=CARTESIAN_POINT('Ctrl Pts',(-10.0531243701796,18.3381178417071,2.0315530670365));
#88697=CARTESIAN_POINT('Ctrl Pts',(-9.90666535343219,18.3295622095059,2.03940180630877));
#88698=CARTESIAN_POINT('Ctrl Pts',(-9.89166027498138,18.3286904618118,2.04043809171958));
#88699=CARTESIAN_POINT('Ctrl Pts',(-9.83785841115321,18.32558299914,2.04498806172054));
#88700=CARTESIAN_POINT('Ctrl Pts',(-9.79918761131266,18.3233841785883,2.049819176046));
#88701=CARTESIAN_POINT('Ctrl Pts',(-9.75100867613171,18.3206877824563,2.05780267367915));
#88702=CARTESIAN_POINT('Ctrl Pts',(-9.74128086831317,18.3201455351903,2.05951597543374));
#88703=CARTESIAN_POINT('Ctrl Pts',(-9.72590646228866,18.3192918566514,2.06238454851116));
#88704=CARTESIAN_POINT('Ctrl Pts',(-9.72024818115562,18.3189783897852,2.0634748958149));
#88705=CARTESIAN_POINT('Ctrl Pts',(-9.70972022318426,18.3183964350008,2.06556818963613));
#88706=CARTESIAN_POINT('Ctrl Pts',(-9.7048489475392,18.3181276813513,2.06656258438403));
#88707=CARTESIAN_POINT('Ctrl Pts',(-9.69404005504112,18.3175324535535,2.06882648589941));
#88708=CARTESIAN_POINT('Ctrl Pts',(-9.68810506205997,18.317206370015,2.07010816332517));
#88709=CARTESIAN_POINT('Ctrl Pts',(-9.67086131093827,18.3162610291871,2.07394446699512));
#88710=CARTESIAN_POINT('Ctrl Pts',(-9.65957457624271,18.3156448720494,2.07659661339339));
#88711=CARTESIAN_POINT('Ctrl Pts',(-9.56037669508277,18.3102500411353,2.10115345727933));
#88712=CARTESIAN_POINT('Ctrl Pts',(-9.47464097754121,18.3057470404164,2.13104385555205));
#88713=CARTESIAN_POINT('Ctrl Pts',(-9.30227910286357,18.2964980561357,2.20973209765766));
#88714=CARTESIAN_POINT('Ctrl Pts',(-9.21674722820046,18.29178851166,2.25979147703072));
#88715=CARTESIAN_POINT('Ctrl Pts',(-9.11846348162114,18.2855188745269,2.33156170886885));
#88716=CARTESIAN_POINT('Ctrl Pts',(-9.10032389052748,18.2843210490912,2.3454708939321));
#88717=CARTESIAN_POINT('Ctrl Pts',(-9.07811571368894,18.2827928218647,2.36334105916751));
#88718=CARTESIAN_POINT('Ctrl Pts',(-9.07373360048407,18.2824881884611,2.3669092092179));
#88719=CARTESIAN_POINT('Ctrl Pts',(-9.06687094261138,18.2820060441997,2.37256356417207));
#88720=CARTESIAN_POINT('Ctrl Pts',(-9.06437642869678,18.2818297242262,2.37463282126245));
#88721=CARTESIAN_POINT('Ctrl Pts',(-9.0597478100679,18.2815005288813,2.37849839478609));
#88722=CARTESIAN_POINT('Ctrl Pts',(-9.05761195636958,18.2813478088793,2.38029253552979));
#88723=CARTESIAN_POINT('Ctrl Pts',(-9.0527581605981,18.2809988956974,2.38439350295164));
#88724=CARTESIAN_POINT('Ctrl Pts',(-9.05004351961214,18.2808024274578,2.38670415280383));
#88725=CARTESIAN_POINT('Ctrl Pts',(-9.04174726067114,18.2801979904188,2.3938182043957));
#88726=CARTESIAN_POINT('Ctrl Pts',(-9.03619352091398,18.2797877689786,2.39865375852849));
#88727=CARTESIAN_POINT('Ctrl Pts',(-9.02339644429872,18.2788299553239,2.40996689593485));
#88728=CARTESIAN_POINT('Ctrl Pts',(-9.01618072135711,18.2782803858726,2.41647506245189));
#88729=CARTESIAN_POINT('Ctrl Pts',(-8.99161186198607,18.2763778638458,2.43908250913721));
#88730=CARTESIAN_POINT('Ctrl Pts',(-8.97458544319715,18.2750049034491,2.45553006933888));
#88731=CARTESIAN_POINT('Ctrl Pts',(-8.88492225065472,18.2675092661216,2.54645112277648));
#88732=CARTESIAN_POINT('Ctrl Pts',(-8.81998344828882,18.2611325988924,2.62809635084505));
#88733=CARTESIAN_POINT('Ctrl Pts',(-8.72567769569843,18.2507048969611,2.77673087629157));
#88734=CARTESIAN_POINT('Ctrl Pts',(-8.69164126348345,18.2465502234151,2.84029144468313));
#88735=CARTESIAN_POINT('Ctrl Pts',(-8.65815195033402,18.2419784701932,2.91571701249542));
#88736=CARTESIAN_POINT('Ctrl Pts',(-8.65398887242578,18.241399510519,2.92537242457397));
#88737=CARTESIAN_POINT('Ctrl Pts',(-8.64745530838666,18.2404731726366,2.9409863941933));
#88738=CARTESIAN_POINT('Ctrl Pts',(-8.64501935067858,18.240123601725,2.94691700796016));
#88739=CARTESIAN_POINT('Ctrl Pts',(-8.64074723753743,18.2395028808195,2.95751558923527));
#88740=CARTESIAN_POINT('Ctrl Pts',(-8.63889597138808,18.2392312282752,2.96217732257645));
#88741=CARTESIAN_POINT('Ctrl Pts',(-8.63507131302106,18.23866430484,2.97195455633938));
#88742=CARTESIAN_POINT('Ctrl Pts',(-8.633102625493,18.2383691940049,2.97707182156747));
#88743=CARTESIAN_POINT('Ctrl Pts',(-8.62802372429944,18.2375990373238,2.99049822234671));
#88744=CARTESIAN_POINT('Ctrl Pts',(-8.62496020263657,18.2371255416287,2.99882485810536));
#88745=CARTESIAN_POINT('Ctrl Pts',(-8.61151180889401,18.2350051508829,3.03642929147105));
#88746=CARTESIAN_POINT('Ctrl Pts',(-8.60198460000047,18.2333864648875,3.06600647269196));
#88747=CARTESIAN_POINT('Ctrl Pts',(-8.57846400182034,18.229019738145,3.14787026383066));
#88748=CARTESIAN_POINT('Ctrl Pts',(-8.56641727500736,18.2263293464914,3.20066553553344));
#88749=CARTESIAN_POINT('Ctrl Pts',(-8.54183678321948,18.219158459604,3.34482448731));
#88750=CARTESIAN_POINT('Ctrl Pts',(-8.53496245012168,18.2147723729107,3.43689280186033));
#88751=CARTESIAN_POINT('Ctrl Pts',(-8.53754423832916,18.2082109869565,3.56720180067189));
#88752=CARTESIAN_POINT('Ctrl Pts',(-8.53979779232265,18.2062443440248,3.60536592954274));
#88753=CARTESIAN_POINT('Ctrl Pts',(-8.54413110599138,18.2038807562438,3.64937929689087));
#88754=CARTESIAN_POINT('Ctrl Pts',(-8.54475717141538,18.2035575305676,3.65535996349483));
#88755=CARTESIAN_POINT('Ctrl Pts',(-8.54581845721097,18.2030368785766,3.66492831928239));
#88756=CARTESIAN_POINT('Ctrl Pts',(-8.54623014663386,18.2028407197793,3.66851861250998));
#88757=CARTESIAN_POINT('Ctrl Pts',(-8.54698450569791,18.202491210542,3.67488873074131));
#88758=CARTESIAN_POINT('Ctrl Pts',(-8.54732186238593,18.2023381576455,3.67766913976863));
#88759=CARTESIAN_POINT('Ctrl Pts',(-8.54805816432342,18.2020108584658,3.68359523384247));
#88760=CARTESIAN_POINT('Ctrl Pts',(-8.5484593453137,18.2018364943468,3.68674054588089));
#88761=CARTESIAN_POINT('Ctrl Pts',(-8.54958233143627,18.2013590155019,3.69532259462514));
#88762=CARTESIAN_POINT('Ctrl Pts',(-8.55032447393351,18.201054797379,3.70075656009415));
#88763=CARTESIAN_POINT('Ctrl Pts',(-8.55437270390683,18.1994527304693,3.72920411785553));
#88764=CARTESIAN_POINT('Ctrl Pts',(-8.55819614186551,18.1981287061099,3.75213947688313));
#88765=CARTESIAN_POINT('Ctrl Pts',(-8.57148853977891,18.1940381126278,3.82162628792636));
#88766=CARTESIAN_POINT('Ctrl Pts',(-8.58267859708684,18.1912106438536,3.86781510999968));
#88767=CARTESIAN_POINT('Ctrl Pts',(-8.6003107719879,18.1874638655781,3.92769759981641));
#88768=CARTESIAN_POINT('Ctrl Pts',(-8.60474691571355,18.1865655478461,3.94195474631465));
#88769=CARTESIAN_POINT('Ctrl Pts',(-8.64656934134801,18.1784864386296,4.06945521901297));
#88770=CARTESIAN_POINT('Ctrl Pts',(-8.69745621073154,18.1713485237048,4.1778223515542));
#88771=CARTESIAN_POINT('Ctrl Pts',(-8.76965133232844,18.1637680148181,4.29268047655825));
#88772=CARTESIAN_POINT('Ctrl Pts',(-8.77859424787018,18.1628617674995,4.30639208900063));
#88773=CARTESIAN_POINT('Ctrl Pts',(-8.79138228111036,18.1616099622326,4.32529820714146));
#88774=CARTESIAN_POINT('Ctrl Pts',(-8.79503436204307,18.1612572570753,4.33062129417682));
#88775=CARTESIAN_POINT('Ctrl Pts',(-8.80141107217604,18.160649576428,4.33978509369104));
#88776=CARTESIAN_POINT('Ctrl Pts',(-8.80411921791235,18.160393984744,4.34363711229598));
#88777=CARTESIAN_POINT('Ctrl Pts',(-8.80977914911257,18.1598649053192,4.35160567984025));
#88778=CARTESIAN_POINT('Ctrl Pts',(-8.81273381393622,18.1595915319445,4.35572011320508));
#88779=CARTESIAN_POINT('Ctrl Pts',(-8.81973081911321,18.1589506969351,4.36535758699385));
#88780=CARTESIAN_POINT('Ctrl Pts',(-8.82379067892185,18.1585839132971,4.37086780161749));
#88781=CARTESIAN_POINT('Ctrl Pts',(-8.83724460269244,18.1573846738881,4.38886232623131));
#88782=CARTESIAN_POINT('Ctrl Pts',(-8.84680011058927,18.1565584771449,4.401224937952));
#88783=CARTESIAN_POINT('Ctrl Pts',(-8.89836939328373,18.1522279516469,4.46578011162198));
#88784=CARTESIAN_POINT('Ctrl Pts',(-8.94373413819298,18.1488605888867,4.51519701152448));
#88785=CARTESIAN_POINT('Ctrl Pts',(-9.06481012093965,18.1406413167421,4.63015092244525));
#88786=CARTESIAN_POINT('Ctrl Pts',(-9.14414358080489,18.1359038938782,4.69135582410406));
#88787=CARTESIAN_POINT('Ctrl Pts',(-9.23652317510664,18.1304278437169,4.74860397759186));
#88788=CARTESIAN_POINT('Ctrl Pts',(-9.24399906008339,18.1299848224608,4.75314457642625));
#88789=CARTESIAN_POINT('Ctrl Pts',(-9.27687815983106,18.1280350488744,4.77271292993974));
#88790=CARTESIAN_POINT('Ctrl Pts',(-9.30269041516959,18.1265008754473,4.78703632725073));
#88791=CARTESIAN_POINT('Ctrl Pts',(-9.33388411192781,18.124622099306,4.80313204432515));
#88792=CARTESIAN_POINT('Ctrl Pts',(-9.33886659823773,18.1243212710927,4.80566692703695));
#88793=CARTESIAN_POINT('Ctrl Pts',(-9.34701491198261,18.1238279070188,4.80975385298613));
#88794=CARTESIAN_POINT('Ctrl Pts',(-9.35017208711968,18.1236364077278,4.81132313473618));
#88795=CARTESIAN_POINT('Ctrl Pts',(-9.35583452461162,18.1232922920906,4.81411219250663));
#88796=CARTESIAN_POINT('Ctrl Pts',(-9.35833762876833,18.1231399422797,4.81533623661545));
#88797=CARTESIAN_POINT('Ctrl Pts',(-9.36378557944347,18.1228078407614,4.81798108921505));
#88798=CARTESIAN_POINT('Ctrl Pts',(-9.36673165664286,18.1226279299996,4.81939916072543));
#88799=CARTESIAN_POINT('Ctrl Pts',(-9.37503966427136,18.1221197282104,4.82336392003349));
#88800=CARTESIAN_POINT('Ctrl Pts',(-9.38041230908795,18.1217900904387,4.82588784476125));
#88801=CARTESIAN_POINT('Ctrl Pts',(-9.4133852256455,18.1197616676322,4.84113346643551));
#88802=CARTESIAN_POINT('Ctrl Pts',(-9.44135909527531,18.118017923052,4.85302473898123));
#88803=CARTESIAN_POINT('Ctrl Pts',(-9.60717476930379,18.1076332521575,4.91749171127662));
#88804=CARTESIAN_POINT('Ctrl Pts',(-9.75196863201047,18.098481726129,4.94985759566105));
#88805=CARTESIAN_POINT('Ctrl Pts',(-9.93627684388861,18.087870032089,4.96258483165601));
#88806=CARTESIAN_POINT('Ctrl Pts',(-9.97346048288491,18.0857737466383,4.96373188640445));
#88807=CARTESIAN_POINT('Ctrl Pts',(-10.0203754660057,18.0831841761497,4.96339047443034));
#88808=CARTESIAN_POINT('Ctrl Pts',(-10.0301001733236,18.0826503653312,4.96322275346304));
#88809=CARTESIAN_POINT('Ctrl Pts',(-10.0455479906651,18.0818069766843,4.96280225399948));
#88810=CARTESIAN_POINT('Ctrl Pts',(-10.0512724179839,18.0814954444591,4.96261279709148));
#88811=CARTESIAN_POINT('Ctrl Pts',(-10.061966088498,18.0809153026888,4.96219601857289));
#88812=CARTESIAN_POINT('Ctrl Pts',(-10.0669355555847,18.0806464409274,4.96197695778642));
#88813=CARTESIAN_POINT('Ctrl Pts',(-10.0780126845546,18.0800487430345,4.96143206451101));
#88814=CARTESIAN_POINT('Ctrl Pts',(-10.0841196351042,18.0797203139707,4.96109327103889));
#88815=CARTESIAN_POINT('Ctrl Pts',(-10.1020104719013,18.0787612406288,4.95998820418168));
#88816=CARTESIAN_POINT('Ctrl Pts',(-10.1137875738955,18.0781338387717,4.95911757292547));
#88817=CARTESIAN_POINT('Ctrl Pts',(-10.2383763393507,18.0715350691834,4.94838960110358));
#88818=CARTESIAN_POINT('Ctrl Pts',(-10.3496915224269,18.0660147711867,4.92561390740946));
#88819=CARTESIAN_POINT('Ctrl Pts',(-10.5430357221998,18.0561195033918,4.86201860559945));
#88820=CARTESIAN_POINT('Ctrl Pts',(-10.6259903220343,18.0517457478222,4.82593917085188));
#88821=CARTESIAN_POINT('Ctrl Pts',(-10.7148714271918,18.0463938439508,4.77707317547384));
#88822=CARTESIAN_POINT('Ctrl Pts',(-10.7245987176453,18.0457984844762,4.77157922926082));
#88823=CARTESIAN_POINT('Ctrl Pts',(-10.7380233564547,18.0449620298901,4.76379297504879));
#88824=CARTESIAN_POINT('Ctrl Pts',(-10.7417750592143,18.0447266461463,4.76159459375992));
#88825=CARTESIAN_POINT('Ctrl Pts',(-10.7477796778929,18.0443472088053,4.75804003036361));
#88826=CARTESIAN_POINT('Ctrl Pts',(-10.7500388626585,18.0442038308838,4.75669442146568));
#88827=CARTESIAN_POINT('Ctrl Pts',(-10.7547082675129,18.0439061825315,4.75389616808107));
#88828=CARTESIAN_POINT('Ctrl Pts',(-10.757117931372,18.0437518534961,4.75244265614762));
#88829=CARTESIAN_POINT('Ctrl Pts',(-10.7629272918916,18.0433780576804,4.74891555166151));
#88830=CARTESIAN_POINT('Ctrl Pts',(-10.766322736036,18.0431581454986,4.74683502171039));
#88831=CARTESIAN_POINT('Ctrl Pts',(-10.7735832420335,18.0426848905361,4.74234534665398));
#88832=CARTESIAN_POINT('Ctrl Pts',(-10.7774456252167,18.0424312879585,4.73993197048965));
#88833=CARTESIAN_POINT('Ctrl Pts',(-10.7881472967579,18.04172361975,4.73317546495951));
#88834=CARTESIAN_POINT('Ctrl Pts',(-10.7949617823173,18.0412672879427,4.72879357406561));
#88835=CARTESIAN_POINT('Ctrl Pts',(-10.8612425498917,18.036775376924,4.6853912249787));
#88836=CARTESIAN_POINT('Ctrl Pts',(-10.9178210664261,18.032522085959,4.64214438463844));
#88837=CARTESIAN_POINT('Ctrl Pts',(-11.0644954775595,18.0207259893287,4.51207153969219));
#88838=CARTESIAN_POINT('Ctrl Pts',(-11.1469853518544,18.01322510673,4.4175375367201));
#88839=CARTESIAN_POINT('Ctrl Pts',(-11.2252839631058,18.0053622405181,4.30047672833203));
#88840=CARTESIAN_POINT('Ctrl Pts',(-11.2338868586401,18.0044846565566,4.28715121212105));
#88841=CARTESIAN_POINT('Ctrl Pts',(-11.2456388705706,18.003265809474,4.26828160350215));
#88842=CARTESIAN_POINT('Ctrl Pts',(-11.2489707526794,18.0029178810214,4.26285311751713));
#88843=CARTESIAN_POINT('Ctrl Pts',(-11.2546926658241,18.0023161777078,4.25339267992669));
#88844=CARTESIAN_POINT('Ctrl Pts',(-11.257098945586,18.0020618150956,4.2493707076995));
#88845=CARTESIAN_POINT('Ctrl Pts',(-11.2620735029621,18.0015331576576,4.2409646001257));
#88846=CARTESIAN_POINT('Ctrl Pts',(-11.2646383566638,18.0012589887489,4.23657850448676));
#88847=CARTESIAN_POINT('Ctrl Pts',(-11.2706498608229,18.0006125394463,4.22617441092761));
#88848=CARTESIAN_POINT('Ctrl Pts',(-11.2740766970947,18.0002409718061,4.22014506598883));
#88849=CARTESIAN_POINT('Ctrl Pts',(-11.2853388293614,17.999009336301,4.19999788635851));
#88850=CARTESIAN_POINT('Ctrl Pts',(-11.2929834927825,17.9981560137514,4.18577449780025));
#88851=CARTESIAN_POINT('Ctrl Pts',(-11.3331476541466,17.9935715335456,4.1079862632371));
#88852=CARTESIAN_POINT('Ctrl Pts',(-11.3612191673311,17.9899970914573,4.04223045109406));
#88853=CARTESIAN_POINT('Ctrl Pts',(-11.4226428766687,17.9807015803029,3.86309204643886));
#88854=CARTESIAN_POINT('Ctrl Pts',(-11.4472680267064,17.9751526385864,3.74729994583407));
#88855=CARTESIAN_POINT('Ctrl Pts',(-11.4592437504637,17.9681213374443,3.61283172611907));
#88856=CARTESIAN_POINT('Ctrl Pts',(-11.4604598594377,17.9672202794926,3.59581372707619));
#88857=CARTESIAN_POINT('Ctrl Pts',(-11.4616550083964,17.9660274655777,3.57364332553573));
#88858=CARTESIAN_POINT('Ctrl Pts',(-11.461904785929,17.9657497546037,3.56850619131987));
#88859=CARTESIAN_POINT('Ctrl Pts',(-11.4622614894896,17.9653025539731,3.56027574860804));
#88860=CARTESIAN_POINT('Ctrl Pts',(-11.46238569214,17.9651340072504,3.55718318435738));
#88861=CARTESIAN_POINT('Ctrl Pts',(-11.4625994671436,17.9648179939412,3.55140310766918));
#88862=CARTESIAN_POINT('Ctrl Pts',(-11.4626914434299,17.9646706616208,3.54871572285166));
#88863=CARTESIAN_POINT('Ctrl Pts',(-11.4628630676688,17.9643708328295,3.54326149629697));
#88864=CARTESIAN_POINT('Ctrl Pts',(-11.4629422732561,17.9642183134261,3.5404946499136));
#88865=CARTESIAN_POINT('Ctrl Pts',(-11.4631079706877,17.9638631658427,3.53406918213765));
#88866=CARTESIAN_POINT('Ctrl Pts',(-11.4631885891396,17.9636602249721,3.53041044377951));
#88867=CARTESIAN_POINT('Ctrl Pts',(-11.4634170261843,17.9629648009995,3.51791536916427));
#88868=CARTESIAN_POINT('Ctrl Pts',(-11.4634985242079,17.9624689422961,3.50907821602269));
#88869=CARTESIAN_POINT('Ctrl Pts',(-11.463499980138,17.9619694309472,3.50024111453588));
#88870=CARTESIAN_POINT('Ctrl Pts',(-11.4634999799479,17.9619694960085,3.50024226556802));
#88871=CARTESIAN_POINT('Ctrl Pts',(-11.463499993316,17.9619649313701,3.50016151024927));
#88872=CARTESIAN_POINT('Ctrl Pts',(-11.4635,17.9619603664338,3.50008075505999));
#88873=CARTESIAN_POINT('Ctrl Pts',(-11.4635,17.9619558011997,3.500000000001));
#88874=CARTESIAN_POINT('',(-11.4634999772434,17.8879984848035,3.50025808640535));
#88875=CARTESIAN_POINT('Ctrl Pts',(-11.4635,17.8879846534521,3.50000000000001));
#88876=CARTESIAN_POINT('Ctrl Pts',(-11.4635,17.887989263516,3.50008602880244));
#88877=CARTESIAN_POINT('Ctrl Pts',(-11.4634999924145,17.8879938739664,3.50017205760456));
#88878=CARTESIAN_POINT('Ctrl Pts',(-11.4634999772434,17.8879984848035,3.50025808640535));
#88879=CARTESIAN_POINT('Ctrl Pts',(-11.4634999771172,17.887998523106,3.50025880105015));
#88880=CARTESIAN_POINT('Ctrl Pts',(-11.4634996087456,17.8881101705811,3.50234191384813));
#88881=CARTESIAN_POINT('Ctrl Pts',(-11.4634947927927,17.8882220441916,3.50442501346896));
#88882=CARTESIAN_POINT('Ctrl Pts',(-11.4634714769766,17.8885042117665,3.50966808511906));
#88883=CARTESIAN_POINT('Ctrl Pts',(-11.4634471899595,17.8886748059766,3.51282800156928));
#88884=CARTESIAN_POINT('Ctrl Pts',(-11.4633823754428,17.8889961405689,3.51876067975669));
#88885=CARTESIAN_POINT('Ctrl Pts',(-11.4633442007053,17.8891467536511,3.5215334591941));
#88886=CARTESIAN_POINT('Ctrl Pts',(-11.4632535428089,17.8894440913529,3.52699133134601));
#88887=CARTESIAN_POINT('Ctrl Pts',(-11.4632015487399,17.8895907894249,3.52967642531825));
#88888=CARTESIAN_POINT('Ctrl Pts',(-11.4630824093265,17.8898859408203,3.53506302975147));
#88889=CARTESIAN_POINT('Ctrl Pts',(-11.4630151725527,17.8900343938093,3.53776449617177));
#88890=CARTESIAN_POINT('Ctrl Pts',(-11.4628100360454,17.8904430863153,3.54518070824536));
#88891=CARTESIAN_POINT('Ctrl Pts',(-11.462656825867,17.8907041566108,3.54989495404495));
#88892=CARTESIAN_POINT('Ctrl Pts',(-11.4619714825889,17.8917253615931,3.56824932931909));
#88893=CARTESIAN_POINT('Ctrl Pts',(-11.4612713258228,17.8924940946772,3.5818820591066));
#88894=CARTESIAN_POINT('Ctrl Pts',(-11.4517366343295,17.9008109229354,3.72768223507119));
#88895=CARTESIAN_POINT('Ctrl Pts',(-11.4251887040487,17.9090236194612,3.85807459512349));
#88896=CARTESIAN_POINT('Ctrl Pts',(-11.360756277425,17.9205562276393,4.0423170640801));
#88897=CARTESIAN_POINT('Ctrl Pts',(-11.3362677186452,17.9241755032336,4.10012965474018));
#88898=CARTESIAN_POINT('Ctrl Pts',(-11.3013731368282,17.9285127985954,4.16969255369424));
#88899=CARTESIAN_POINT('Ctrl Pts',(-11.2943956174074,17.9293469927661,4.18308137683167));
#88900=CARTESIAN_POINT('Ctrl Pts',(-11.2839993316971,17.9305438111077,4.20229876397182));
#88901=CARTESIAN_POINT('Ctrl Pts',(-11.2807455757794,17.9309121963055,4.20821508734007));
#88902=CARTESIAN_POINT('Ctrl Pts',(-11.2749860500647,17.9315536606731,4.21851815616438));
#88903=CARTESIAN_POINT('Ctrl Pts',(-11.272498311363,17.931827373199,4.22291480622881));
#88904=CARTESIAN_POINT('Ctrl Pts',(-11.2676345724193,17.9323560900038,4.23140772773798));
#88905=CARTESIAN_POINT('Ctrl Pts',(-11.2652613601635,17.9326111892698,4.23550551635607));
#88906=CARTESIAN_POINT('Ctrl Pts',(-11.2595560068576,17.9332176857829,4.24524752570933));
#88907=CARTESIAN_POINT('Ctrl Pts',(-11.2562057396522,17.9335684276562,4.25088104953298));
#88908=CARTESIAN_POINT('Ctrl Pts',(-11.2440491297574,17.934822115061,4.27101347300195));
#88909=CARTESIAN_POINT('Ctrl Pts',(-11.2350285156226,17.9357173061254,4.28538182424198));
#88910=CARTESIAN_POINT('Ctrl Pts',(-11.1663487169399,17.9422875970031,4.39066689345395));
#88911=CARTESIAN_POINT('Ctrl Pts',(-11.0969726289713,17.9475663700131,4.47483874800094));
#88912=CARTESIAN_POINT('Ctrl Pts',(-10.9776803205141,17.9556474304084,4.59053730667888));
#88913=CARTESIAN_POINT('Ctrl Pts',(-10.9341394120926,17.9584430351183,4.6280573191357));
#88914=CARTESIAN_POINT('Ctrl Pts',(-10.8690077875601,17.9625812994912,4.67782003646447));
#88915=CARTESIAN_POINT('Ctrl Pts',(-10.8491353127244,17.9638388754578,4.69222635359976));
#88916=CARTESIAN_POINT('Ctrl Pts',(-10.8206982501887,17.9656453678623,4.71176975521268));
#88917=CARTESIAN_POINT('Ctrl Pts',(-10.8124282279415,17.9661715317254,4.71732983286636));
#88918=CARTESIAN_POINT('Ctrl Pts',(-10.7997008921494,17.9669835334379,4.72569918099538));
#88919=CARTESIAN_POINT('Ctrl Pts',(-10.7952839741127,17.9672657406665,4.7285696553665));
#88920=CARTESIAN_POINT('Ctrl Pts',(-10.7879834304738,17.9677330250821,4.73325827940501));
#88921=CARTESIAN_POINT('Ctrl Pts',(-10.7851087417519,17.9679172364231,4.7350903341782));
#88922=CARTESIAN_POINT('Ctrl Pts',(-10.779545419841,17.9682741969351,4.73860859857566));
#88923=CARTESIAN_POINT('Ctrl Pts',(-10.7768576476883,17.9684468591731,4.74029614080542));
#88924=CARTESIAN_POINT('Ctrl Pts',(-10.7718826276345,17.9687668745793,4.74339723693117));
#88925=CARTESIAN_POINT('Ctrl Pts',(-10.7695969615272,17.9689140653315,4.7448132374431));
#88926=CARTESIAN_POINT('Ctrl Pts',(-10.7643185742832,17.9692543570505,4.74806317412578));
#88927=CARTESIAN_POINT('Ctrl Pts',(-10.7613231646898,17.9694477427382,4.74989263858129));
#88928=CARTESIAN_POINT('Ctrl Pts',(-10.7535860170618,17.9699479056553,4.75458001608911));
#88929=CARTESIAN_POINT('Ctrl Pts',(-10.7488346345796,17.9702556792723,4.75742180271658));
#88930=CARTESIAN_POINT('Ctrl Pts',(-10.7194682177947,17.9721611784279,4.77476028702277));
#88931=CARTESIAN_POINT('Ctrl Pts',(-10.6944507460462,17.9737985017231,4.78855975656396));
#88932=CARTESIAN_POINT('Ctrl Pts',(-10.5756576750906,17.9815822313934,4.84962085526537));
#88933=CARTESIAN_POINT('Ctrl Pts',(-10.477374481719,17.9880222210261,4.88743370361108));
#88934=CARTESIAN_POINT('Ctrl Pts',(-10.3001367619972,17.9989243097765,4.93453619122959));
#88935=CARTESIAN_POINT('Ctrl Pts',(-10.2228802093233,18.003462250837,4.94855225895876));
#88936=CARTESIAN_POINT('Ctrl Pts',(-10.1335643216425,18.008431491231,4.95743670003048));
#88937=CARTESIAN_POINT('Ctrl Pts',(-10.1222532008044,18.009055997427,4.9584290616));
#88938=CARTESIAN_POINT('Ctrl Pts',(-10.1049258693375,18.010005512237,4.95974624073034));
#88939=CARTESIAN_POINT('Ctrl Pts',(-10.0989174692475,18.0103334510483,4.9601656964797));
#88940=CARTESIAN_POINT('Ctrl Pts',(-10.0884273542918,18.0109037547198,4.96083298077675));
#88941=CARTESIAN_POINT('Ctrl Pts',(-10.0839468002151,18.0111466289908,4.96109730342239));
#88942=CARTESIAN_POINT('Ctrl Pts',(-10.0738419275788,18.0116927929174,4.96164678801592));
#88943=CARTESIAN_POINT('Ctrl Pts',(-10.0682170181941,18.0119957111346,4.96192010822445));
#88944=CARTESIAN_POINT('Ctrl Pts',(-10.0530596984043,18.0128090727179,4.96256894649914));
#88945=CARTESIAN_POINT('Ctrl Pts',(-10.043524872726,18.0133176284255,4.96288374319325));
#88946=CARTESIAN_POINT('Ctrl Pts',(-9.99999183384938,18.0156261071092,4.96389500258682));
#88947=CARTESIAN_POINT('Ctrl Pts',(-9.96597749113655,18.0173921232223,4.96349966908337));
#88948=CARTESIAN_POINT('Ctrl Pts',(-9.78108619632389,18.0268394819998,4.95490035299515));
#88949=CARTESIAN_POINT('Ctrl Pts',(-9.63218764684898,18.0337900855613,4.92455732752997));
#88950=CARTESIAN_POINT('Ctrl Pts',(-9.46189257301755,18.0430388384167,4.86132622355269));
#88951=CARTESIAN_POINT('Ctrl Pts',(-9.43354805247602,18.0446288798754,4.8497779897763));
#88952=CARTESIAN_POINT('Ctrl Pts',(-9.4001524608048,18.046586626404,4.83493466739257));
#88953=CARTESIAN_POINT('Ctrl Pts',(-9.3947314374909,18.0469071304095,4.83248549759034));
#88954=CARTESIAN_POINT('Ctrl Pts',(-9.38635110371162,18.0474070286117,4.8286376462023));
#88955=CARTESIAN_POINT('Ctrl Pts',(-9.38338123727799,18.0475850532611,4.82726194244078));
#88956=CARTESIAN_POINT('Ctrl Pts',(-9.37789093821161,18.0479158161645,4.82469631755533));
#88957=CARTESIAN_POINT('Ctrl Pts',(-9.37536927608101,18.0480683863659,4.82350915254318));
#88958=CARTESIAN_POINT('Ctrl Pts',(-9.36966698942193,18.0484148714559,4.8208046654541));
#88959=CARTESIAN_POINT('Ctrl Pts',(-9.36648846052105,18.0486090453774,4.81928306186363));
#88960=CARTESIAN_POINT('Ctrl Pts',(-9.35708210139169,18.0491866873134,4.81473828244191));
#88961=CARTESIAN_POINT('Ctrl Pts',(-9.35087028261773,18.0495720846605,4.81168242414956));
#88962=CARTESIAN_POINT('Ctrl Pts',(-9.30237405746508,18.0526104411209,4.78739620787788));
#88963=CARTESIAN_POINT('Ctrl Pts',(-9.26112366012086,18.0553707932687,4.76417240627522));
#88964=CARTESIAN_POINT('Ctrl Pts',(-9.196573746687,18.0598976390821,4.72359145243149));
#88965=CARTESIAN_POINT('Ctrl Pts',(-9.17253583938214,18.0616331493684,4.70746543446746));
#88966=CARTESIAN_POINT('Ctrl Pts',(-9.10087630023947,18.0669313104379,4.65624682541889));
#88967=CARTESIAN_POINT('Ctrl Pts',(-9.05488740484713,18.0705033852549,4.61896951611743));
#88968=CARTESIAN_POINT('Ctrl Pts',(-8.96099606454717,18.0780591133946,4.53293489082242));
#88969=CARTESIAN_POINT('Ctrl Pts',(-8.91399017038175,18.0820112074612,4.48339631386365));
#88970=CARTESIAN_POINT('Ctrl Pts',(-8.86057649106344,18.0866971070263,4.4185831671818));
#88971=CARTESIAN_POINT('Ctrl Pts',(-8.85074373803303,18.0875692031448,4.40625109072412));
#88972=CARTESIAN_POINT('Ctrl Pts',(-8.83691561492532,18.0888099478358,4.38832098849814));
#88973=CARTESIAN_POINT('Ctrl Pts',(-8.83275759429778,18.089184962231,4.38285028968508));
#88974=CARTESIAN_POINT('Ctrl Pts',(-8.82559803179066,18.0898341362901,4.37329146624862));
#88975=CARTESIAN_POINT('Ctrl Pts',(-8.82257894870636,18.0901089746129,4.36921668002116));
#88976=CARTESIAN_POINT('Ctrl Pts',(-8.81680031278948,18.0906371756653,4.36133203753208));
#88977=CARTESIAN_POINT('Ctrl Pts',(-8.81403783317806,18.0908906491108,4.35752441263949));
#88978=CARTESIAN_POINT('Ctrl Pts',(-8.80754090980717,18.091489119169,4.34847802421088));
#88979=CARTESIAN_POINT('Ctrl Pts',(-8.80382253929078,18.0918335008506,4.34322780056042));
#88980=CARTESIAN_POINT('Ctrl Pts',(-8.79084497680795,18.0930422045479,4.32464529100944));
#88981=CARTESIAN_POINT('Ctrl Pts',(-8.78177289882597,18.0938994907646,4.31118338475427));
#88982=CARTESIAN_POINT('Ctrl Pts',(-8.70700508299732,18.101078930073,4.1961523900241));
#88983=CARTESIAN_POINT('Ctrl Pts',(-8.65391226871675,18.1068938705064,4.08695338616846));
#88984=CARTESIAN_POINT('Ctrl Pts',(-8.59624173516248,18.1155995993522,3.91787652720263));
#88985=CARTESIAN_POINT('Ctrl Pts',(-8.58086803654647,18.1184301359661,3.86224526518128));
#88986=CARTESIAN_POINT('Ctrl Pts',(-8.56334897873854,18.1227277589649,3.78026900655125));
#88987=CARTESIAN_POINT('Ctrl Pts',(-8.5585682162571,18.1240945177659,3.75454099360245));
#88988=CARTESIAN_POINT('Ctrl Pts',(-8.55359102390566,18.1258022523152,3.72308222037375));
#88989=CARTESIAN_POINT('Ctrl Pts',(-8.55273494057883,18.1261089173885,3.71745907388404));
#88990=CARTESIAN_POINT('Ctrl Pts',(-8.55144613864575,18.126591806441,3.70864876042961));
#88991=CARTESIAN_POINT('Ctrl Pts',(-8.55099110139725,18.1267668063105,3.7054648530403));
#88992=CARTESIAN_POINT('Ctrl Pts',(-8.55016039743586,18.1270949386858,3.69951236309469));
#88993=CARTESIAN_POINT('Ctrl Pts',(-8.5497821615139,18.1272479264566,3.69674419102849));
#88994=CARTESIAN_POINT('Ctrl Pts',(-8.5489341119503,18.1275993095779,3.69040228667864));
#88995=CARTESIAN_POINT('Ctrl Pts',(-8.54846957402789,18.1277979948724,3.6868278997851));
#88996=CARTESIAN_POINT('Ctrl Pts',(-8.54728584671542,18.1283209578516,3.67744872986739));
#88997=CARTESIAN_POINT('Ctrl Pts',(-8.54658825216556,18.1286463851502,3.67164134644519));
#88998=CARTESIAN_POINT('Ctrl Pts',(-8.5420151639162,18.130903836636,3.63154239267359));
#88999=CARTESIAN_POINT('Ctrl Pts',(-8.53931911876848,18.1328935881627,3.59712969771141));
#89000=CARTESIAN_POINT('Ctrl Pts',(-8.5358585157125,18.1376369505387,3.51637307954069));
#89001=CARTESIAN_POINT('Ctrl Pts',(-8.53607397644721,18.1404156644546,3.4700231354266));
#89002=CARTESIAN_POINT('Ctrl Pts',(-8.54492883175439,18.1506467534406,3.30026839031113));
#89003=CARTESIAN_POINT('Ctrl Pts',(-8.56699893240249,18.1580617792506,3.17806274418342));
#89004=CARTESIAN_POINT('Ctrl Pts',(-8.60893570279792,18.1658460437972,3.04500311375358));
#89005=CARTESIAN_POINT('Ctrl Pts',(-8.61393060122558,18.1667200597582,3.0300067077447));
#89006=CARTESIAN_POINT('Ctrl Pts',(-8.62144626553979,18.1679630234602,3.00860489570334));
#89007=CARTESIAN_POINT('Ctrl Pts',(-8.62377068244079,18.1683383684147,3.0021321309092));
#89008=CARTESIAN_POINT('Ctrl Pts',(-8.62788858897168,18.168987928468,2.99091429606747));
#89009=CARTESIAN_POINT('Ctrl Pts',(-8.62966126817891,18.1692628244981,2.98616175775453));
#89010=CARTESIAN_POINT('Ctrl Pts',(-8.63312498941516,18.1697910064823,2.97702096563025));
#89011=CARTESIAN_POINT('Ctrl Pts',(-8.63481254280004,18.170044403917,2.97263146437586));
#89012=CARTESIAN_POINT('Ctrl Pts',(-8.63885669885756,18.1706424949359,2.9622616997818));
#89013=CARTESIAN_POINT('Ctrl Pts',(-8.64123161098919,18.1709865754877,2.95628864957481));
#89014=CARTESIAN_POINT('Ctrl Pts',(-8.64972965805799,18.1721932012086,2.93531899424917));
#89015=CARTESIAN_POINT('Ctrl Pts',(-8.6560624617088,18.1730487427763,2.92040828574774));
#89016=CARTESIAN_POINT('Ctrl Pts',(-8.7119290733633,18.1802473442794,2.79471118872531));
#89017=CARTESIAN_POINT('Ctrl Pts',(-8.7748155740205,18.1860793198079,2.69037997932913));
#89018=CARTESIAN_POINT('Ctrl Pts',(-8.8853635842846,18.1947922348901,2.54988766795997));
#89019=CARTESIAN_POINT('Ctrl Pts',(-8.92348415812956,18.1976106183449,2.50690356087113));
#89020=CARTESIAN_POINT('Ctrl Pts',(-8.97629785877265,18.2014443852056,2.45397516166054));
#89021=CARTESIAN_POINT('Ctrl Pts',(-8.98878590472146,18.2023463288817,2.44189790488529));
#89022=CARTESIAN_POINT('Ctrl Pts',(-9.00991098520214,18.2038705105562,2.42218331420514));
#89023=CARTESIAN_POINT('Ctrl Pts',(-9.0184288233795,18.2044846692273,2.4144203971475));
#89024=CARTESIAN_POINT('Ctrl Pts',(-9.03022653676245,18.2053361998756,2.40392066489235));
#89025=CARTESIAN_POINT('Ctrl Pts',(-9.03342825634286,18.2055673800023,2.4010962088129));
#89026=CARTESIAN_POINT('Ctrl Pts',(-9.03882866374633,18.2059575527906,2.39637399998643));
#89027=CARTESIAN_POINT('Ctrl Pts',(-9.04102075045574,18.2061159932624,2.39446868689435));
#89028=CARTESIAN_POINT('Ctrl Pts',(-9.04518634891259,18.2064172303025,2.39086975300984));
#89029=CARTESIAN_POINT('Ctrl Pts',(-9.04715873032829,18.2065599282459,2.38917484378417));
#89030=CARTESIAN_POINT('Ctrl Pts',(-9.05232038334082,18.2069335066419,2.38476318818663));
#89031=CARTESIAN_POINT('Ctrl Pts',(-9.05551679758988,18.2071649911372,2.38205488429413));
#89032=CARTESIAN_POINT('Ctrl Pts',(-9.06654506946966,18.2079640092833,2.37279174644536));
#89033=CARTESIAN_POINT('Ctrl Pts',(-9.07443370609425,18.2085361572852,2.36630534187619));
#89034=CARTESIAN_POINT('Ctrl Pts',(-9.16618876500408,18.2151913918364,2.29245604532219));
#89035=CARTESIAN_POINT('Ctrl Pts',(-9.25716317435109,18.2217682499649,2.23445878972017));
#89036=CARTESIAN_POINT('Ctrl Pts',(-9.44109545425367,18.2340646247692,2.14391946224767));
#89037=CARTESIAN_POINT('Ctrl Pts',(-9.53261868003092,18.2397757914085,2.10971616412372));
#89038=CARTESIAN_POINT('Ctrl Pts',(-9.63817833650661,18.2458235153786,2.08188366322053));
#89039=CARTESIAN_POINT('Ctrl Pts',(-9.64951566279887,18.2464666887299,2.07903919781908));
#89040=CARTESIAN_POINT('Ctrl Pts',(-9.66681283178383,18.2474385203373,2.07491906186062));
#89041=CARTESIAN_POINT('Ctrl Pts',(-9.67274839694089,18.2477703253788,2.07354433676447));
#89042=CARTESIAN_POINT('Ctrl Pts',(-9.68307821917085,18.2483449020125,2.07121973557085));
#89043=CARTESIAN_POINT('Ctrl Pts',(-9.68746855863009,18.2485882077633,2.07025297413599));
#89044=CARTESIAN_POINT('Ctrl Pts',(-9.6973210561208,18.2491322325151,2.06813098519359));
#89045=CARTESIAN_POINT('Ctrl Pts',(-9.7027855272989,18.2494325994448,2.06698674917736));
#89046=CARTESIAN_POINT('Ctrl Pts',(-9.71738896165846,18.2502317418174,2.0640159802438));
#89047=CARTESIAN_POINT('Ctrl Pts',(-9.72653913288657,18.2507287439758,2.06224540913756));
#89048=CARTESIAN_POINT('Ctrl Pts',(-9.76703927070889,18.2529127676223,2.05480920380854));
#89049=CARTESIAN_POINT('Ctrl Pts',(-9.79855360886277,18.2545702847652,2.05008045577953));
#89050=CARTESIAN_POINT('Ctrl Pts',(-9.98267534778406,18.2640573038775,2.02857265150947));
#89051=CARTESIAN_POINT('Ctrl Pts',(-10.1369792643312,18.2711112119794,2.03486311084391));
#89052=CARTESIAN_POINT('Ctrl Pts',(-10.3176100446488,18.2804886518688,2.07104904688613));
#89053=CARTESIAN_POINT('Ctrl Pts',(-10.3475477689308,18.2820854523383,2.07803401845936));
#89054=CARTESIAN_POINT('Ctrl Pts',(-10.3829957838397,18.2840507620222,2.08749090220312));
#89055=CARTESIAN_POINT('Ctrl Pts',(-10.388740816691,18.2843716463479,2.08906120019572));
#89056=CARTESIAN_POINT('Ctrl Pts',(-10.3976294015769,18.2848720115687,2.09154913753787));
#89057=CARTESIAN_POINT('Ctrl Pts',(-10.4007797951124,18.2850501188187,2.09244235344751));
#89058=CARTESIAN_POINT('Ctrl Pts',(-10.4066059410909,18.285380956119,2.09411535807451));
#89059=CARTESIAN_POINT('Ctrl Pts',(-10.4092824785304,18.2855335174898,2.09489222117054));
#89060=CARTESIAN_POINT('Ctrl Pts',(-10.4153363291556,18.2858798804483,2.09666811200862));
#89061=CARTESIAN_POINT('Ctrl Pts',(-10.4187122479847,18.2860739402845,2.09767168358409));
#89062=CARTESIAN_POINT('Ctrl Pts',(-10.4289245109951,18.2866636686938,2.10074768370778));
#89063=CARTESIAN_POINT('Ctrl Pts',(-10.4357492301552,18.2870614362393,2.10285795819934));
#89064=CARTESIAN_POINT('Ctrl Pts',(-10.493262076955,18.2904428245268,2.12110391151845));
#89065=CARTESIAN_POINT('Ctrl Pts',(-10.5430466602286,18.2935617722061,2.13994076776042));
#89066=CARTESIAN_POINT('Ctrl Pts',(-10.67297216189,18.3020295654065,2.19737249957229));
#89067=CARTESIAN_POINT('Ctrl Pts',(-10.7508180731415,18.307442779777,2.24063369505736));
#89068=CARTESIAN_POINT('Ctrl Pts',(-10.8758212052372,18.316378916286,2.3258350079595));
#89069=CARTESIAN_POINT('Ctrl Pts',(-10.925088345171,18.3199792427879,2.36424504518652));
#89070=CARTESIAN_POINT('Ctrl Pts',(-10.9830163101908,18.3242965685847,2.41568551673987));
#89071=CARTESIAN_POINT('Ctrl Pts',(-10.9941203317286,18.3251285396392,2.4258567346156));
#89072=CARTESIAN_POINT('Ctrl Pts',(-11.0099683928408,18.326322774443,2.44082976484213));
#89073=CARTESIAN_POINT('Ctrl Pts',(-11.0148390511286,18.3266907646281,2.44549564058799));
#89074=CARTESIAN_POINT('Ctrl Pts',(-11.0233001570769,18.3273317716017,2.45371392742774));
#89075=CARTESIAN_POINT('Ctrl Pts',(-11.0269047682177,18.3276054190621,2.45725153798602));
#89076=CARTESIAN_POINT('Ctrl Pts',(-11.0338548678405,18.3281341750756,2.4641434440977));
#89077=CARTESIAN_POINT('Ctrl Pts',(-11.0372025199864,18.3283893776532,2.4674954598534));
#89078=CARTESIAN_POINT('Ctrl Pts',(-11.0451482068862,18.3289963794379,2.47552914429914));
#89079=CARTESIAN_POINT('Ctrl Pts',(-11.0497311690379,18.3293475207092,2.48022562142863));
#89080=CARTESIAN_POINT('Ctrl Pts',(-11.0660811265318,18.3306041327653,2.49720756410111));
#89081=CARTESIAN_POINT('Ctrl Pts',(-11.0776655487432,18.3315018008122,2.50966741212571));
#89082=CARTESIAN_POINT('Ctrl Pts',(-11.1607853913352,18.3380046036386,2.60225462224212));
#89083=CARTESIAN_POINT('Ctrl Pts',(-11.2235240166911,18.3432243978081,2.68983880930622));
#89084=CARTESIAN_POINT('Ctrl Pts',(-11.3090981423567,18.3517232941099,2.84225165472479));
#89085=CARTESIAN_POINT('Ctrl Pts',(-11.3379825296583,18.3549990369876,2.90319823702338));
#89086=CARTESIAN_POINT('Ctrl Pts',(-11.3729990341876,18.3598992749333,2.99253236341333));
#89087=CARTESIAN_POINT('Ctrl Pts',(-11.3826503272776,18.3613884403787,3.01945072323726));
#89088=CARTESIAN_POINT('Ctrl Pts',(-11.3933146265079,18.3632332878534,3.05218232439173));
#89089=CARTESIAN_POINT('Ctrl Pts',(-11.3950895412571,18.3635478584082,3.05774273482604));
#89090=CARTESIAN_POINT('Ctrl Pts',(-11.3978005079577,18.3640404674818,3.06641431686641));
#89091=CARTESIAN_POINT('Ctrl Pts',(-11.3987595621253,18.3642171996847,3.06951830281881));
#89092=CARTESIAN_POINT('Ctrl Pts',(-11.400522910386,18.3645468154811,3.07529350162224));
#89093=CARTESIAN_POINT('Ctrl Pts',(-11.401329906553,18.3646995408946,3.07796383462544));
#89094=CARTESIAN_POINT('Ctrl Pts',(-11.4031484898235,18.3650480138882,3.08404421253774));
#89095=CARTESIAN_POINT('Ctrl Pts',(-11.4041552791101,18.3652440331692,3.08745563485443));
#89096=CARTESIAN_POINT('Ctrl Pts',(-11.4067406090546,18.3657554880852,3.09633491819155));
#89097=CARTESIAN_POINT('Ctrl Pts',(-11.4082996934079,18.3660719947437,3.10180832401046));
#89098=CARTESIAN_POINT('Ctrl Pts',(-11.4182370686533,18.3681423322619,3.13748350147459));
#89099=CARTESIAN_POINT('Ctrl Pts',(-11.4256746729285,18.3699438206818,3.16793669692388));
#89100=CARTESIAN_POINT('Ctrl Pts',(-11.4528988643753,18.3776735780483,3.29729601855312));
#89101=CARTESIAN_POINT('Ctrl Pts',(-11.4634117725477,18.3838503472647,3.39787060296645));
#89102=CARTESIAN_POINT('Ctrl Pts',(-11.4634998156995,18.389874919343,3.49915186239209));
#89103=CARTESIAN_POINT('Ctrl Pts',(-11.4635,18.3899001415702,3.49957593289561));
#89104=CARTESIAN_POINT('Ctrl Pts',(-11.4635,18.3899253605917,3.49999999994518));
#89105=CARTESIAN_POINT('Origin',(-10.,13.2,3.5));
#89106=CARTESIAN_POINT('',(-11.4635,18.9594567372512,3.50000000000276));
#89107=CARTESIAN_POINT('',(-11.4635,18.8903920399481,3.49999999999848));
#89108=CARTESIAN_POINT('',(-11.4635,13.2,3.5));
#89109=CARTESIAN_POINT('Ctrl Pts',(-11.4635,18.9594567372512,3.50000000000276));
#89110=CARTESIAN_POINT('Ctrl Pts',(-11.4635000000001,18.9578291943808,3.47145831790744));
#89111=CARTESIAN_POINT('Ctrl Pts',(-11.462665060547,18.9562256754957,3.44292102721574));
#89112=CARTESIAN_POINT('Ctrl Pts',(-11.4605522721912,18.954228287802,3.4068502485034));
#89113=CARTESIAN_POINT('Ctrl Pts',(-11.4600497231483,18.9538106957395,3.39927947085835));
#89114=CARTESIAN_POINT('Ctrl Pts',(-11.4590919408327,18.9531013841429,3.38637053391844));
#89115=CARTESIAN_POINT('Ctrl Pts',(-11.4586662336761,18.9528087540919,3.38103039393257));
#89116=CARTESIAN_POINT('Ctrl Pts',(-11.4578155799634,18.9522633951236,3.37105163649082));
#89117=CARTESIAN_POINT('Ctrl Pts',(-11.4573977917925,18.9520104467364,3.36641249005495));
#89118=CARTESIAN_POINT('Ctrl Pts',(-11.4564834460767,18.951486156403,3.35677482078956));
#89119=CARTESIAN_POINT('Ctrl Pts',(-11.4559832875043,18.9512149303026,3.35177669537899));
#89120=CARTESIAN_POINT('Ctrl Pts',(-11.4547809158592,18.9505966298355,3.34035511580458));
#89121=CARTESIAN_POINT('Ctrl Pts',(-11.4540618714463,18.9502500851136,3.33393351322411));
#89122=CARTESIAN_POINT('Ctrl Pts',(-11.4516608367582,18.9491616239936,3.31370299390724));
#89123=CARTESIAN_POINT('Ctrl Pts',(-11.4498244554434,18.9484245248361,3.29991295529326));
#89124=CARTESIAN_POINT('Ctrl Pts',(-11.442968009881,18.9459579681926,3.25349375770704));
#89125=CARTESIAN_POINT('Ctrl Pts',(-11.4370405709005,18.944256503438,3.22100787230089));
#89126=CARTESIAN_POINT('Ctrl Pts',(-11.4085163732689,18.93745415692,3.08995576641959));
#89127=CARTESIAN_POINT('Ctrl Pts',(-11.3768348745937,18.9326202645166,2.99365926308));
#89128=CARTESIAN_POINT('Ctrl Pts',(-11.3147856679703,18.9252004746787,2.85522834193555));
#89129=CARTESIAN_POINT('Ctrl Pts',(-11.2917134742703,18.922698433926,2.81016852005433));
#89130=CARTESIAN_POINT('Ctrl Pts',(-11.2542362093617,18.9188526869045,2.74547470155571));
#89131=CARTESIAN_POINT('Ctrl Pts',(-11.2415999240966,18.9175865732557,2.72485718204888));
#89132=CARTESIAN_POINT('Ctrl Pts',(-11.2254419267573,18.9159918217724,2.69990303174952));
#89133=CARTESIAN_POINT('Ctrl Pts',(-11.2223978880725,18.9156923816115,2.69525999496594));
#89134=CARTESIAN_POINT('Ctrl Pts',(-11.2175657435833,18.9152184194566,2.68798025957375));
#89135=CARTESIAN_POINT('Ctrl Pts',(-11.2157952889568,18.9150450487089,2.68533183826622));
#89136=CARTESIAN_POINT('Ctrl Pts',(-11.2124536734647,18.9147183135099,2.68036827284475));
#89137=CARTESIAN_POINT('Ctrl Pts',(-11.2108845131558,18.9145650812808,2.6780518423833));
#89138=CARTESIAN_POINT('Ctrl Pts',(-11.2072871023027,18.9142142442614,2.67277392036233));
#89139=CARTESIAN_POINT('Ctrl Pts',(-11.2052545944049,18.9140163566227,2.66981538419494));
#89140=CARTESIAN_POINT('Ctrl Pts',(-11.1998352403013,18.9134896637938,2.66198877384909));
#89141=CARTESIAN_POINT('Ctrl Pts',(-11.1964296888148,18.9131596522619,2.65713380877139));
#89142=CARTESIAN_POINT('Ctrl Pts',(-11.1720354369948,18.9108033320287,2.62280302316445));
#89143=CARTESIAN_POINT('Ctrl Pts',(-11.1499909314023,18.9087136076269,2.59409600858215));
#89144=CARTESIAN_POINT('Ctrl Pts',(-11.120690503431,18.9060139185949,2.55873490049831));
#89145=CARTESIAN_POINT('Ctrl Pts',(-11.1143989322536,18.9054384570796,2.55129445753025));
#89146=CARTESIAN_POINT('Ctrl Pts',(-11.022462339847,18.8970959369846,2.44474629186931));
#89147=CARTESIAN_POINT('Ctrl Pts',(-10.9239448553004,18.8890514035154,2.35749200973739));
#89148=CARTESIAN_POINT('Ctrl Pts',(-10.7944785686214,18.8800991801085,2.27066919219183));
#89149=CARTESIAN_POINT('Ctrl Pts',(-10.7734785295382,18.8786887966517,2.25734900371317));
#89150=CARTESIAN_POINT('Ctrl Pts',(-10.7418555516207,18.8766259650343,2.23840317068915));
#89151=CARTESIAN_POINT('Ctrl Pts',(-10.7314870722249,18.8759590209082,2.23236326402638));
#89152=CARTESIAN_POINT('Ctrl Pts',(-10.7147980827225,18.8749003001296,2.22291445535111));
#89153=CARTESIAN_POINT('Ctrl Pts',(-10.7085248848645,18.8745056258549,2.2194234589353));
#89154=CARTESIAN_POINT('Ctrl Pts',(-10.6965336402723,18.8737573740352,2.21286549456926));
#89155=CARTESIAN_POINT('Ctrl Pts',(-10.6908204040481,18.8734035051903,2.20979012623903));
#89156=CARTESIAN_POINT('Ctrl Pts',(-10.680720760227,18.8727825230568,2.2044399246955));
#89157=CARTESIAN_POINT('Ctrl Pts',(-10.6763429596706,18.8725148518274,2.20214913650963));
#89158=CARTESIAN_POINT('Ctrl Pts',(-10.6677353349726,18.8719914605706,2.19770037266136));
#89159=CARTESIAN_POINT('Ctrl Pts',(-10.6635064465607,18.8717356845554,2.19554072771858));
#89160=CARTESIAN_POINT('Ctrl Pts',(-10.6521947357998,18.8710551061784,2.18983320573347));
#89161=CARTESIAN_POINT('Ctrl Pts',(-10.6450934360713,18.8706315847703,2.1863221611519));
#89162=CARTESIAN_POINT('Ctrl Pts',(-10.6191738998113,18.8690989621495,2.17376780874764));
#89163=CARTESIAN_POINT('Ctrl Pts',(-10.6001907456747,18.8680016867728,2.16506956369669));
#89164=CARTESIAN_POINT('Ctrl Pts',(-10.4663302910516,18.8604247647738,2.10716647191824));
#89165=CARTESIAN_POINT('Ctrl Pts',(-10.3457566208648,18.8544723974564,2.07244867197357));
#89166=CARTESIAN_POINT('Ctrl Pts',(-10.1730514120716,18.8459214830301,2.04591561735527));
#89167=CARTESIAN_POINT('Ctrl Pts',(-10.1235194088822,18.8434583642121,2.04087338114476));
#89168=CARTESIAN_POINT('Ctrl Pts',(-10.0499282429259,18.8396665857575,2.03715612671095));
#89169=CARTESIAN_POINT('Ctrl Pts',(-10.0260012858663,18.8384130043831,2.0365353339157));
#89170=CARTESIAN_POINT('Ctrl Pts',(-9.99653694512305,18.8368323285651,2.03649363297941));
#89171=CARTESIAN_POINT('Ctrl Pts',(-9.99100268723458,18.8365338248773,2.03651719331993));
#89172=CARTESIAN_POINT('Ctrl Pts',(-9.98228711176768,18.8360610154672,2.03660373526586));
#89173=CARTESIAN_POINT('Ctrl Pts',(-9.97910558038905,18.835887851657,2.03664570356983));
#89174=CARTESIAN_POINT('Ctrl Pts',(-9.97312594475074,18.8355612810369,2.0367440867218));
#89175=CARTESIAN_POINT('Ctrl Pts',(-9.9703278518384,18.8354080047915,2.03679815276146));
#89176=CARTESIAN_POINT('Ctrl Pts',(-9.96393511218208,18.8350567752785,2.03694002069192));
#89177=CARTESIAN_POINT('Ctrl Pts',(-9.96034062508318,18.8348585368182,2.03703304459769));
#89178=CARTESIAN_POINT('Ctrl Pts',(-9.95079753599882,18.8343303025055,2.03731521190371));
#89179=CARTESIAN_POINT('Ctrl Pts',(-9.94484974566822,18.8339990893216,2.0375273955443));
#89180=CARTESIAN_POINT('Ctrl Pts',(-9.90222655173997,18.8316120934399,2.03930833121028));
#89181=CARTESIAN_POINT('Ctrl Pts',(-9.86562304320559,18.8294910562788,2.04222011333611));
#89182=CARTESIAN_POINT('Ctrl Pts',(-9.818036327895,18.8266727987988,2.04781297247808));
#89183=CARTESIAN_POINT('Ctrl Pts',(-9.80691735349685,18.8260099083856,2.04924949616924));
#89184=CARTESIAN_POINT('Ctrl Pts',(-9.70949540439554,18.8201688953874,2.06297580970964));
#89185=CARTESIAN_POINT('Ctrl Pts',(-9.6244334270762,18.8148552283334,2.08282606282197));
#89186=CARTESIAN_POINT('Ctrl Pts',(-9.46932776818362,18.8051593116639,2.13397758086038));
#89187=CARTESIAN_POINT('Ctrl Pts',(-9.39897788043555,18.8007572881146,2.16343518342935));
#89188=CARTESIAN_POINT('Ctrl Pts',(-9.32118529193298,18.7959158614292,2.20340044214389));
#89189=CARTESIAN_POINT('Ctrl Pts',(-9.31119868307332,18.7952946633065,2.20867797309247));
#89190=CARTESIAN_POINT('Ctrl Pts',(-9.29599386014975,18.794349177264,2.21693970685566));
#89191=CARTESIAN_POINT('Ctrl Pts',(-9.29073141822298,18.7940219963281,2.21984124375142));
#89192=CARTESIAN_POINT('Ctrl Pts',(-9.28119126483665,18.7934289127674,2.2251782555804));
#89193=CARTESIAN_POINT('Ctrl Pts',(-9.27690770363486,18.7931626364467,2.22760304560641));
#89194=CARTESIAN_POINT('Ctrl Pts',(-9.26760659221794,18.7925844665923,2.2329302526694));
#89195=CARTESIAN_POINT('Ctrl Pts',(-9.26259387481363,18.792272875214,2.2358409687759));
#89196=CARTESIAN_POINT('Ctrl Pts',(-9.24895831080855,18.791425221753,2.24386738297079));
#89197=CARTESIAN_POINT('Ctrl Pts',(-9.24037044228102,18.7908912887596,2.2490420821605));
#89198=CARTESIAN_POINT('Ctrl Pts',(-9.19699109352886,18.7881929986118,2.27579215671435));
#89199=CARTESIAN_POINT('Ctrl Pts',(-9.16306112427864,18.7860790096998,2.29873322758832));
#89200=CARTESIAN_POINT('Ctrl Pts',(-9.1193267985195,18.7833255144796,2.33105705393178));
#89201=CARTESIAN_POINT('Ctrl Pts',(-9.10862843243184,18.7826494810306,2.33919440098863));
#89202=CARTESIAN_POINT('Ctrl Pts',(-8.99486002225649,18.7754244934497,2.42822885269533));
#89203=CARTESIAN_POINT('Ctrl Pts',(-8.90300049832303,18.7693290904473,2.52245937698914));
#89204=CARTESIAN_POINT('Ctrl Pts',(-8.8075067865231,18.7611551842407,2.65109188041892));
#89205=CARTESIAN_POINT('Ctrl Pts',(-8.79080652531311,18.7596352954806,2.67505395789347));
#89206=CARTESIAN_POINT('Ctrl Pts',(-8.77162427778422,18.7577561293549,2.70441229399017));
#89207=CARTESIAN_POINT('Ctrl Pts',(-8.76844289227744,18.7574397730328,2.7093459663302));
#89208=CARTESIAN_POINT('Ctrl Pts',(-8.76354360579448,18.7569450064434,2.71704506321135));
#89209=CARTESIAN_POINT('Ctrl Pts',(-8.7618050676932,18.7567679216277,2.71979736157814));
#89210=CARTESIAN_POINT('Ctrl Pts',(-8.75859477684193,18.7564380567307,2.72491736311356));
#89211=CARTESIAN_POINT('Ctrl Pts',(-8.75712059851864,18.756285437895,2.72728348337096));
#89212=CARTESIAN_POINT('Ctrl Pts',(-8.75378728448964,18.7559377431985,2.73266781406443));
#89213=CARTESIAN_POINT('Ctrl Pts',(-8.75193235644096,18.7557423999877,2.73568856319722));
#89214=CARTESIAN_POINT('Ctrl Pts',(-8.74631078210339,18.755144766432,2.7449183258558));
#89215=CARTESIAN_POINT('Ctrl Pts',(-8.74257941991845,18.7547402948701,2.75114856610679));
#89216=CARTESIAN_POINT('Ctrl Pts',(-8.70231213597262,18.7502914778474,2.81953223133805));
#89217=CARTESIAN_POINT('Ctrl Pts',(-8.67037403145688,18.7460006796192,2.88427051163823));
#89218=CARTESIAN_POINT('Ctrl Pts',(-8.60708928850038,18.7358603453108,3.04068227358088));
#89219=CARTESIAN_POINT('Ctrl Pts',(-8.57979994851503,18.7300149683673,3.13365528258996));
#89220=CARTESIAN_POINT('Ctrl Pts',(-8.55373819961013,18.7218892903862,3.2717772272273));
#89221=CARTESIAN_POINT('Ctrl Pts',(-8.54754378370078,18.7194051674711,3.31525601120711));
#89222=CARTESIAN_POINT('Ctrl Pts',(-8.54235836658396,18.7164350912081,3.36880853377542));
#89223=CARTESIAN_POINT('Ctrl Pts',(-8.54150394302759,18.7158915010358,3.37867567906812));
#89224=CARTESIAN_POINT('Ctrl Pts',(-8.54031488289668,18.7150394081234,3.39424454859444));
#89225=CARTESIAN_POINT('Ctrl Pts',(-8.53991335812582,18.7147288339642,3.39994073703175));
#89226=CARTESIAN_POINT('Ctrl Pts',(-8.53922436195622,18.7141495768639,3.41060456816035));
#89227=CARTESIAN_POINT('Ctrl Pts',(-8.53892886784122,18.7138806484491,3.41557159509564));
#89228=CARTESIAN_POINT('Ctrl Pts',(-8.53832538304471,18.7132816639919,3.42667023703583));
#89229=CARTESIAN_POINT('Ctrl Pts',(-8.53803063053482,18.7129520235042,3.43280249778797));
#89230=CARTESIAN_POINT('Ctrl Pts',(-8.53738267060471,18.7121211849862,3.4483185343291));
#89231=CARTESIAN_POINT('Ctrl Pts',(-8.53708117020793,18.7116215922586,3.4577042665429));
#89232=CARTESIAN_POINT('Ctrl Pts',(-8.53586225876163,18.708753215202,3.51189922046019));
#89233=CARTESIAN_POINT('Ctrl Pts',(-8.53691318857981,18.7064460014785,3.55673096663508));
#89234=CARTESIAN_POINT('Ctrl Pts',(-8.54968398214165,18.6971569430534,3.74052264773319));
#89235=CARTESIAN_POINT('Ctrl Pts',(-8.57916718813452,18.6907032628381,3.87748462954363));
#89236=CARTESIAN_POINT('Ctrl Pts',(-8.63793376626102,18.6820770777782,4.03618919786933));
#89237=CARTESIAN_POINT('Ctrl Pts',(-8.64915245984553,18.6805246905454,4.06385633100031));
#89238=CARTESIAN_POINT('Ctrl Pts',(-8.66359422740778,18.6786091533332,4.0965624434258));
#89239=CARTESIAN_POINT('Ctrl Pts',(-8.66601275945561,18.6782908813501,4.10195114220656));
#89240=CARTESIAN_POINT('Ctrl Pts',(-8.66981799446867,18.6777937613714,4.1102939709825));
#89241=CARTESIAN_POINT('Ctrl Pts',(-8.67118209836014,18.6776162592269,4.11325841430237));
#89242=CARTESIAN_POINT('Ctrl Pts',(-8.67372959951746,18.6772860240727,4.11874618579013));
#89243=CARTESIAN_POINT('Ctrl Pts',(-8.67491029629567,18.6771334554957,4.12127070941791));
#89244=CARTESIAN_POINT('Ctrl Pts',(-8.67760458946536,18.676786403326,4.12698893032943));
#89245=CARTESIAN_POINT('Ctrl Pts',(-8.67912254085213,18.6765916564754,4.13018051218103));
#89246=CARTESIAN_POINT('Ctrl Pts',(-8.68377172557635,18.675997611975,4.13986509793267));
#89247=CARTESIAN_POINT('Ctrl Pts',(-8.68693933659286,18.6755961703262,4.14634039314462));
#89248=CARTESIAN_POINT('Ctrl Pts',(-8.71653709972075,18.6718768605277,4.2057291433559));
#89249=CARTESIAN_POINT('Ctrl Pts',(-8.74610203361513,18.6683920460409,4.25701328215571));
#89250=CARTESIAN_POINT('Ctrl Pts',(-8.82481791271013,18.6598477659351,4.37623623054966));
#89251=CARTESIAN_POINT('Ctrl Pts',(-8.8768657948442,18.6547586832,4.44202636772783));
#89252=CARTESIAN_POINT('Ctrl Pts',(-8.97649241125211,18.6461771310912,4.54788486957857));
#89253=CARTESIAN_POINT('Ctrl Pts',(-9.02152644143322,18.6426234263662,4.59005572209119));
#89254=CARTESIAN_POINT('Ctrl Pts',(-9.08063182070296,18.638355406718,4.63877922239412));
#89255=CARTESIAN_POINT('Ctrl Pts',(-9.0923185113176,18.6375290491734,4.64811598060108));
#89256=CARTESIAN_POINT('Ctrl Pts',(-9.10946471013047,18.6363414165798,4.66138898644044));
#89257=CARTESIAN_POINT('Ctrl Pts',(-9.11481119916441,18.6359745013952,4.66546911984733));
#89258=CARTESIAN_POINT('Ctrl Pts',(-9.12421805958479,18.6353348120661,4.67254582218144));
#89259=CARTESIAN_POINT('Ctrl Pts',(-9.12826612854073,18.6350614141095,4.67555849301908));
#89260=CARTESIAN_POINT('Ctrl Pts',(-9.13614722561148,18.6345327425181,4.68136070121678));
#89261=CARTESIAN_POINT('Ctrl Pts',(-9.13997838087901,18.6342773772397,4.68415266649632));
#89262=CARTESIAN_POINT('Ctrl Pts',(-9.14915793260964,18.6336693615064,4.69077424233487));
#89263=CARTESIAN_POINT('Ctrl Pts',(-9.15451874174152,18.6333173747335,4.69458652415774));
#89264=CARTESIAN_POINT('Ctrl Pts',(-9.1739254525707,18.6320540589711,4.70819131998691));
#89265=CARTESIAN_POINT('Ctrl Pts',(-9.18811754223349,18.6311506458519,4.71777351370964));
#89266=CARTESIAN_POINT('Ctrl Pts',(-9.28875326198152,18.6248789732538,4.7831791049219));
#89267=CARTESIAN_POINT('Ctrl Pts',(-9.38070554854212,18.6198602707876,4.82999908465359));
#89268=CARTESIAN_POINT('Ctrl Pts',(-9.50545663544112,18.6133661425768,4.87775161444595));
#89269=CARTESIAN_POINT('Ctrl Pts',(-9.53443329508618,18.6118760658344,4.88781131737711));
#89270=CARTESIAN_POINT('Ctrl Pts',(-9.60869360125336,18.608061574664,4.9110042635383));
#89271=CARTESIAN_POINT('Ctrl Pts',(-9.65433276132393,18.6057213963754,4.92287290912014));
#89272=CARTESIAN_POINT('Ctrl Pts',(-9.72310857799154,18.6021007305993,4.93725387481766));
#89273=CARTESIAN_POINT('Ctrl Pts',(-9.74586342164085,18.6008876361038,4.94145136592426));
#89274=CARTESIAN_POINT('Ctrl Pts',(-9.77411408771597,18.5993524618504,4.94597295672184));
#89275=CARTESIAN_POINT('Ctrl Pts',(-9.77952602960481,18.5990570571561,4.94680802576002));
#89276=CARTESIAN_POINT('Ctrl Pts',(-9.7880769981455,18.5985880630172,4.94807835891727));
#89277=CARTESIAN_POINT('Ctrl Pts',(-9.79121302620802,18.5984155848264,4.94853384201511));
#89278=CARTESIAN_POINT('Ctrl Pts',(-9.79712395640153,18.5980895511239,4.94937276366743));
#89279=CARTESIAN_POINT('Ctrl Pts',(-9.79989849359706,18.597936120649,4.94975842256653));
#89280=CARTESIAN_POINT('Ctrl Pts',(-9.80625804520421,18.5975835536242,4.95062379251562));
#89281=CARTESIAN_POINT('Ctrl Pts',(-9.8098437415754,18.5973841239265,4.95109818043584));
#89282=CARTESIAN_POINT('Ctrl Pts',(-9.81940602022508,18.5968506442323,4.95232721989833));
#89283=CARTESIAN_POINT('Ctrl Pts',(-9.82538550133075,18.5965153391574,4.9530582622521));
#89284=CARTESIAN_POINT('Ctrl Pts',(-9.86960229252743,18.5940240749958,4.95818727339153));
#89285=CARTESIAN_POINT('Ctrl Pts',(-9.90799242254303,18.5917964330933,4.96111183710114));
#89286=CARTESIAN_POINT('Ctrl Pts',(-10.0381681247916,18.5841209538749,4.96587823235985));
#89287=CARTESIAN_POINT('Ctrl Pts',(-10.1299984413347,18.5785163252143,4.96060145746879));
#89288=CARTESIAN_POINT('Ctrl Pts',(-10.3004774010799,18.5682509548979,4.93459163435388));
#89289=CARTESIAN_POINT('Ctrl Pts',(-10.3790904158726,18.5635738346236,4.91585084707607));
#89290=CARTESIAN_POINT('Ctrl Pts',(-10.4666057508596,18.5584746346053,4.88717028308612));
#89291=CARTESIAN_POINT('Ctrl Pts',(-10.4774017884599,18.5578472853668,4.88349190953207));
#89292=CARTESIAN_POINT('Ctrl Pts',(-10.493840810038,18.5568944361162,4.87767553992463));
#89293=CARTESIAN_POINT('Ctrl Pts',(-10.4995152382987,18.5565659728823,4.87562828089422));
#89294=CARTESIAN_POINT('Ctrl Pts',(-10.5093889127066,18.5559951648206,4.87199683907327));
#89295=CARTESIAN_POINT('Ctrl Pts',(-10.5135938029111,18.5557523068487,4.87042832612619));
#89296=CARTESIAN_POINT('Ctrl Pts',(-10.5230490322838,18.5552067048538,4.86685169544319));
#89297=CARTESIAN_POINT('Ctrl Pts',(-10.5282951676456,18.5549043287108,4.86483261411838));
#89298=CARTESIAN_POINT('Ctrl Pts',(-10.5423744106431,18.5540936903237,4.85932059137314));
#89299=CARTESIAN_POINT('Ctrl Pts',(-10.5511854447853,18.5535872945577,4.85577176641991));
#89300=CARTESIAN_POINT('Ctrl Pts',(-10.5910026463331,18.5513023723958,4.83928224505634));
#89301=CARTESIAN_POINT('Ctrl Pts',(-10.6215933144883,18.5495568946276,4.82536147420745));
#89302=CARTESIAN_POINT('Ctrl Pts',(-10.6661529404654,18.5470154986339,4.8032013678181));
#89303=CARTESIAN_POINT('Ctrl Pts',(-10.6805065703623,18.5461969780945,4.79576401164056));
#89304=CARTESIAN_POINT('Ctrl Pts',(-10.814775093416,18.5385283747616,4.72334598477918));
#89305=CARTESIAN_POINT('Ctrl Pts',(-10.9251604654451,18.5322037135823,4.64214936086016));
#89306=CARTESIAN_POINT('Ctrl Pts',(-11.0438952489654,18.5237400798321,4.52615435144233));
#89307=CARTESIAN_POINT('Ctrl Pts',(-11.0644532018346,18.5221988623762,4.50481301125365));
#89308=CARTESIAN_POINT('Ctrl Pts',(-11.0883064659294,18.5202958253574,4.47849682116792));
#89309=CARTESIAN_POINT('Ctrl Pts',(-11.0922385022404,18.5199782060204,4.47410576667655));
#89310=CARTESIAN_POINT('Ctrl Pts',(-11.0983042536294,18.5194818877506,4.46724901029832));
#89311=CARTESIAN_POINT('Ctrl Pts',(-11.1004564798394,18.5193045277037,4.46479967714465));
#89312=CARTESIAN_POINT('Ctrl Pts',(-11.1044333140265,18.5189744189999,4.46024323688067));
#89313=CARTESIAN_POINT('Ctrl Pts',(-11.1062600974178,18.5188218336919,4.45813809838841));
#89314=CARTESIAN_POINT('Ctrl Pts',(-11.1103919138853,18.51847456447,4.45334912995422));
#89315=CARTESIAN_POINT('Ctrl Pts',(-11.1126932255873,18.5182796159138,4.45066216459677));
#89316=CARTESIAN_POINT('Ctrl Pts',(-11.1196657734697,18.5176843588288,4.44246115626137));
#89317=CARTESIAN_POINT('Ctrl Pts',(-11.1243058575673,18.5172818937623,4.43692091960949));
#89318=CARTESIAN_POINT('Ctrl Pts',(-11.1676255132608,18.513466196205,4.38441226581151));
#89319=CARTESIAN_POINT('Ctrl Pts',(-11.2033780175825,18.5098764432556,4.3351133024829));
#89320=CARTESIAN_POINT('Ctrl Pts',(-11.2753617041683,18.5018308010741,4.22159508366675));
#89321=CARTESIAN_POINT('Ctrl Pts',(-11.3100266684528,18.4973654266722,4.15656508946262));
#89322=CARTESIAN_POINT('Ctrl Pts',(-11.3600685296333,18.4899878363907,4.04278647233013));
#89323=CARTESIAN_POINT('Ctrl Pts',(-11.3780586971039,18.4870275331359,3.99533680351693));
#89324=CARTESIAN_POINT('Ctrl Pts',(-11.4026314683836,18.4824508258297,3.91873740137572));
#89325=CARTESIAN_POINT('Ctrl Pts',(-11.4108482702535,18.4807858785617,3.89015815636262));
#89326=CARTESIAN_POINT('Ctrl Pts',(-11.4203467654776,18.4786676477986,3.85287912080897));
#89327=CARTESIAN_POINT('Ctrl Pts',(-11.4224284561605,18.478188933693,3.84439207287755));
#89328=CARTESIAN_POINT('Ctrl Pts',(-11.4256856256605,18.4774154160204,3.83057901533335));
#89329=CARTESIAN_POINT('Ctrl Pts',(-11.4269075458637,18.4771191377824,3.8252642698995));
#89330=CARTESIAN_POINT('Ctrl Pts',(-11.4291981885138,18.476551693937,3.81503973443032));
#89331=CARTESIAN_POINT('Ctrl Pts',(-11.4302713862357,18.4762803895147,3.81013103505893));
#89332=CARTESIAN_POINT('Ctrl Pts',(-11.432669081689,18.4756614494362,3.79888700442992));
#89333=CARTESIAN_POINT('Ctrl Pts',(-11.4339768810146,18.4753143472781,3.7925481936284));
#89334=CARTESIAN_POINT('Ctrl Pts',(-11.4373392798564,18.4743957516364,3.77568640533997));
#89335=CARTESIAN_POINT('Ctrl Pts',(-11.4393203886253,18.4738265766896,3.76514906469495));
#89336=CARTESIAN_POINT('Ctrl Pts',(-11.456032501873,18.4687580889258,3.67054523624139));
#89337=CARTESIAN_POINT('Ctrl Pts',(-11.4634999999972,18.4645009776468,3.58535927216356));
#89338=CARTESIAN_POINT('Ctrl Pts',(-11.4635,18.4603263886907,3.50000000004768));
#89339=CARTESIAN_POINT('Ctrl Pts',(-11.4635,18.3899253605917,3.49999999994518));
#89340=CARTESIAN_POINT('Ctrl Pts',(-11.4635000000029,18.3945771388639,3.57822134916453));
#89341=CARTESIAN_POINT('Ctrl Pts',(-11.4572289891273,18.3991090574555,3.65632582354247));
#89342=CARTESIAN_POINT('Ctrl Pts',(-11.4430408401938,18.4040355085825,3.74408811969543));
#89343=CARTESIAN_POINT('Ctrl Pts',(-11.441224692596,18.4046226067156,3.75459236153278));
#89344=CARTESIAN_POINT('Ctrl Pts',(-11.4381247168033,18.4055594387835,3.77142442432346));
#89345=CARTESIAN_POINT('Ctrl Pts',(-11.4369135242059,18.4059114447033,3.77776508964052));
#89346=CARTESIAN_POINT('Ctrl Pts',(-11.4346852373581,18.4065350251148,3.78902552666228));
#89347=CARTESIAN_POINT('Ctrl Pts',(-11.4336846945519,18.406807117627,3.79394843567765));
#89348=CARTESIAN_POINT('Ctrl Pts',(-11.4315429299953,18.4073735045454,3.80421529925514));
#89349=CARTESIAN_POINT('Ctrl Pts',(-11.4303970847225,18.4076676477889,3.80955821722363));
#89350=CARTESIAN_POINT('Ctrl Pts',(-11.4273315913403,18.4084321024381,3.82347165981112));
#89351=CARTESIAN_POINT('Ctrl Pts',(-11.4253646544717,18.4089009072752,3.83203161393671));
#89352=CARTESIAN_POINT('Ctrl Pts',(-11.4163051351005,18.4109682836516,3.86989305352903));
#89353=CARTESIAN_POINT('Ctrl Pts',(-11.4083849675585,18.4125403953376,3.89899004593538));
#89354=CARTESIAN_POINT('Ctrl Pts',(-11.3844419289713,18.4167442984087,3.97731679489139));
#89355=CARTESIAN_POINT('Ctrl Pts',(-11.3666971787622,18.4193239430853,4.02597542888947));
#89356=CARTESIAN_POINT('Ctrl Pts',(-11.305566318069,18.4269863086776,4.16946930926579));
#89357=CARTESIAN_POINT('Ctrl Pts',(-11.2546020226093,18.4319185081065,4.26069904141007));
#89358=CARTESIAN_POINT('Ctrl Pts',(-11.1768742706503,18.4387644485129,4.370469811124));
#89359=CARTESIAN_POINT('Ctrl Pts',(-11.1585976051872,18.4403382749099,4.39465193214756));
#89360=CARTESIAN_POINT('Ctrl Pts',(-11.1360490403333,18.4422614959794,4.4226356729963));
#89361=CARTESIAN_POINT('Ctrl Pts',(-11.1324879819438,18.4425647110403,4.42700322320252));
#89362=CARTESIAN_POINT('Ctrl Pts',(-11.1266490361908,18.4430612477817,4.43408068757959));
#89363=CARTESIAN_POINT('Ctrl Pts',(-11.1243863505771,18.4432535110348,4.43680313607298));
#89364=CARTESIAN_POINT('Ctrl Pts',(-11.1203238155486,18.4435984923092,4.44165523050985));
#89365=CARTESIAN_POINT('Ctrl Pts',(-11.1185277360159,18.4437509386556,4.44378796794327));
#89366=CARTESIAN_POINT('Ctrl Pts',(-11.1146178009627,18.4440826588219,4.44840394467078));
#89367=CARTESIAN_POINT('Ctrl Pts',(-11.1125017663161,18.4442620878345,4.45088522125727));
#89368=CARTESIAN_POINT('Ctrl Pts',(-11.1065384325569,18.4447674274733,4.45783071488683));
#89369=CARTESIAN_POINT('Ctrl Pts',(-11.1026724804649,18.4450946607164,4.46227874314975));
#89370=CARTESIAN_POINT('Ctrl Pts',(-11.0792379011744,18.447075400211,4.48891509090154));
#89371=CARTESIAN_POINT('Ctrl Pts',(-11.0590282504532,18.4487714992823,4.51052779486213));
#89372=CARTESIAN_POINT('Ctrl Pts',(-10.9424796200404,18.4584142138015,4.62782976782654));
#89373=CARTESIAN_POINT('Ctrl Pts',(-10.8338396162752,18.4668191002877,4.71036626633017));
#89374=CARTESIAN_POINT('Ctrl Pts',(-10.6732575175743,18.4775151120482,4.80034081350232));
#89375=CARTESIAN_POINT('Ctrl Pts',(-10.6300057613722,18.4802576589133,4.82183789131803));
#89376=CARTESIAN_POINT('Ctrl Pts',(-10.5769585323694,18.4834581943366,4.84500687276494));
#89377=CARTESIAN_POINT('Ctrl Pts',(-10.5681124353432,18.4839866977325,4.84876717889631));
#89378=CARTESIAN_POINT('Ctrl Pts',(-10.5534924103709,18.4848517409329,4.8548125137176));
#89379=CARTESIAN_POINT('Ctrl Pts',(-10.5477399386922,18.4851899806868,4.85714839162369));
#89380=CARTESIAN_POINT('Ctrl Pts',(-10.5373443873484,18.485797458194,4.86129279932157));
#89381=CARTESIAN_POINT('Ctrl Pts',(-10.5327066289094,18.4860671278402,4.8631143475392));
#89382=CARTESIAN_POINT('Ctrl Pts',(-10.5227766826792,18.4866416893098,4.86695606252127));
#89383=CARTESIAN_POINT('Ctrl Pts',(-10.5174818756021,18.4869463460354,4.86896926425603));
#89384=CARTESIAN_POINT('Ctrl Pts',(-10.5030983226591,18.4877694109149,4.87434283278086));
#89385=CARTESIAN_POINT('Ctrl Pts',(-10.4939875869587,18.4882858516315,4.87764379077817));
#89386=CARTESIAN_POINT('Ctrl Pts',(-10.4463860301156,18.4909595575676,4.89435761860032));
#89387=CARTESIAN_POINT('Ctrl Pts',(-10.4073782491194,18.493066615075,4.90624926980271));
#89388=CARTESIAN_POINT('Ctrl Pts',(-10.2222492191598,18.502760558043,4.95433484845058));
#89389=CARTESIAN_POINT('Ctrl Pts',(-10.0716367098282,18.5096711303314,4.9694700847652));
#89390=CARTESIAN_POINT('Ctrl Pts',(-9.89708857762196,18.5186534628246,4.96007991369904));
#89391=CARTESIAN_POINT('Ctrl Pts',(-9.87283316913323,18.5199260337265,4.95816754039881));
#89392=CARTESIAN_POINT('Ctrl Pts',(-9.84289620320358,18.5215389859063,4.95505462900815));
#89393=CARTESIAN_POINT('Ctrl Pts',(-9.83715794117221,18.5218500844385,4.95442361023682));
#89394=CARTESIAN_POINT('Ctrl Pts',(-9.82817577117257,18.5223402833644,4.95338204716033));
#89395=CARTESIAN_POINT('Ctrl Pts',(-9.82492918699121,18.5225181271451,4.952994545972));
#89396=CARTESIAN_POINT('Ctrl Pts',(-9.81891721500178,18.5228487275864,4.95225653560759));
#89397=CARTESIAN_POINT('Ctrl Pts',(-9.81615151501714,18.5230013175686,4.95190900349485));
#89398=CARTESIAN_POINT('Ctrl Pts',(-9.80988714944279,18.523348072093,4.95110365039489));
#89399=CARTESIAN_POINT('Ctrl Pts',(-9.80638915329023,18.5235424973962,4.95064107884556));
#89400=CARTESIAN_POINT('Ctrl Pts',(-9.79578203754632,18.5241344147196,4.94919935562773));
#89401=CARTESIAN_POINT('Ctrl Pts',(-9.78867852484275,18.5245340281366,4.94818057520031));
#89402=CARTESIAN_POINT('Ctrl Pts',(-9.69523325299222,18.5298305984014,4.93407657012682));
#89403=CARTESIAN_POINT('Ctrl Pts',(-9.61023158522235,18.5350858865448,4.91334214191407));
#89404=CARTESIAN_POINT('Ctrl Pts',(-9.41941685056852,18.547227291252,4.84826518681616));
#89405=CARTESIAN_POINT('Ctrl Pts',(-9.31591476615047,18.5540493253382,4.7988193632697));
#89406=CARTESIAN_POINT('Ctrl Pts',(-9.20508493694049,18.5613752325927,4.72891060719764));
#89407=CARTESIAN_POINT('Ctrl Pts',(-9.1911108736851,18.5623003254658,4.71975803001214));
#89408=CARTESIAN_POINT('Ctrl Pts',(-9.17191033486806,18.5635738081848,4.70670715784962));
#89409=CARTESIAN_POINT('Ctrl Pts',(-9.16654897057532,18.563929670229,4.70301040800854));
#89410=CARTESIAN_POINT('Ctrl Pts',(-9.1573409695375,18.5645413678452,4.69657023532857));
#89411=CARTESIAN_POINT('Ctrl Pts',(-9.1534826439643,18.5647978382758,4.6938437654709));
#89412=CARTESIAN_POINT('Ctrl Pts',(-9.14552091471016,18.5653274245818,4.68815963879319));
#89413=CARTESIAN_POINT('Ctrl Pts',(-9.14141950202428,18.5656004331313,4.68519929287771));
#89414=CARTESIAN_POINT('Ctrl Pts',(-9.13184673438077,18.5662381456105,4.67821402612228));
#89415=CARTESIAN_POINT('Ctrl Pts',(-9.12638786262747,18.5666021917373,4.6741721421963));
#89416=CARTESIAN_POINT('Ctrl Pts',(-9.10870704111983,18.5677827480732,4.6608892610103));
#89417=CARTESIAN_POINT('Ctrl Pts',(-9.09660181337867,18.5685932725393,4.65149414009487));
#89418=CARTESIAN_POINT('Ctrl Pts',(-9.03430284268052,18.5727801824782,4.60155536321842));
#89419=CARTESIAN_POINT('Ctrl Pts',(-8.98668079926833,18.5760300968124,4.55791333902873));
#89420=CARTESIAN_POINT('Ctrl Pts',(-8.87247084567277,18.5841820677194,4.43843568637325));
#89421=CARTESIAN_POINT('Ctrl Pts',(-8.81056274972724,18.5889550555506,4.35861539172998));
#89422=CARTESIAN_POINT('Ctrl Pts',(-8.73648141049508,18.596003882923,4.23953583888169));
#89423=CARTESIAN_POINT('Ctrl Pts',(-8.71698421076062,18.5980335030499,4.2051683867065));
#89424=CARTESIAN_POINT('Ctrl Pts',(-8.69612600058251,18.60046779899,4.16466654462355));
#89425=CARTESIAN_POINT('Ctrl Pts',(-8.69338321127876,18.6007937005894,4.15925836118495));
#89426=CARTESIAN_POINT('Ctrl Pts',(-8.6890527411901,18.6013178794442,4.15058643261032));
#89427=CARTESIAN_POINT('Ctrl Pts',(-8.68744342486895,18.6015148623385,4.14733349842246));
#89428=CARTESIAN_POINT('Ctrl Pts',(-8.68461239035154,18.6018653441285,4.14155712659661));
#89429=CARTESIAN_POINT('Ctrl Pts',(-8.68338580361434,18.6020185400425,4.13903612424483));
#89430=CARTESIAN_POINT('Ctrl Pts',(-8.68079052281459,18.6023455791189,4.13366285486749));
#89431=CARTESIAN_POINT('Ctrl Pts',(-8.67942385268337,18.6025195366235,4.13080971543014));
#89432=CARTESIAN_POINT('Ctrl Pts',(-8.6757285313285,18.6029946185873,4.12303050980669));
#89433=CARTESIAN_POINT('Ctrl Pts',(-8.67341814666634,18.6032968278426,4.1180958852591));
#89434=CARTESIAN_POINT('Ctrl Pts',(-8.66160051125302,18.6048693130499,4.09248376055741));
#89435=CARTESIAN_POINT('Ctrl Pts',(-8.65254946860621,18.6061646506607,4.07160051174937));
#89436=CARTESIAN_POINT('Ctrl Pts',(-8.62671914249961,18.6101321803157,4.00797621518228));
#89437=CARTESIAN_POINT('Ctrl Pts',(-8.61146111572676,18.6128614491138,3.96464976342717));
#89438=CARTESIAN_POINT('Ctrl Pts',(-8.581325859582,18.6191491171178,3.86423724445855));
#89439=CARTESIAN_POINT('Ctrl Pts',(-8.56781060561573,18.6227161704226,3.80682056626437));
#89440=CARTESIAN_POINT('Ctrl Pts',(-8.5434141997546,18.6312813780389,3.66537208161505));
#89441=CARTESIAN_POINT('Ctrl Pts',(-8.53628922971168,18.6362024089687,3.58089939650866));
#89442=CARTESIAN_POINT('Ctrl Pts',(-8.53653204370949,18.6414866062904,3.48555390740052));
#89443=CARTESIAN_POINT('Ctrl Pts',(-8.53667710508559,18.6420770352681,3.47483529261879));
#89444=CARTESIAN_POINT('Ctrl Pts',(-8.53709860769564,18.6430181332781,3.45764836303294));
#89445=CARTESIAN_POINT('Ctrl Pts',(-8.5373002250128,18.6433711072986,3.45117874544495));
#89446=CARTESIAN_POINT('Ctrl Pts',(-8.53773463689923,18.643995797825,3.43968815245667));
#89447=CARTESIAN_POINT('Ctrl Pts',(-8.53795038803866,18.644268038691,3.4346666691707));
#89448=CARTESIAN_POINT('Ctrl Pts',(-8.53845428893852,18.6448341366366,3.42419661686861));
#89449=CARTESIAN_POINT('Ctrl Pts',(-8.53874704881716,18.6451278462459,3.41874834042412));
#89450=CARTESIAN_POINT('Ctrl Pts',(-8.53958834237091,18.6458898780341,3.40457191647122));
#89451=CARTESIAN_POINT('Ctrl Pts',(-8.54018465753275,18.6463567116404,3.39584675119378));
#89452=CARTESIAN_POINT('Ctrl Pts',(-8.54315578744952,18.6484026668579,3.35743801304619));
#89453=CARTESIAN_POINT('Ctrl Pts',(-8.54635810963059,18.649956016134,3.32782452149933));
#89454=CARTESIAN_POINT('Ctrl Pts',(-8.55746592606879,18.654095307351,3.24798598949941));
#89455=CARTESIAN_POINT('Ctrl Pts',(-8.56708800104811,18.6566311889731,3.19804081191957));
#89456=CARTESIAN_POINT('Ctrl Pts',(-8.59003794673595,18.66133169548,3.10522910337996));
#89457=CARTESIAN_POINT('Ctrl Pts',(-8.60277512639161,18.6635024111371,3.06227887389326));
#89458=CARTESIAN_POINT('Ctrl Pts',(-8.64478818450335,18.6697332921894,2.94127417799491));
#89459=CARTESIAN_POINT('Ctrl Pts',(-8.67878299831601,18.6737960375407,2.86505429119046));
#89460=CARTESIAN_POINT('Ctrl Pts',(-8.72454675093081,18.6787867304896,2.78223997708675));
#89461=CARTESIAN_POINT('Ctrl Pts',(-8.73013757597537,18.6793899617017,2.77239444100173));
#89462=CARTESIAN_POINT('Ctrl Pts',(-8.73804558528531,18.6802358052865,2.75883710669789));
#89463=CARTESIAN_POINT('Ctrl Pts',(-8.74026616993627,18.680472538678,2.75506909338957));
#89464=CARTESIAN_POINT('Ctrl Pts',(-8.74385160213527,18.6808536262899,2.74904700813513));
#89465=CARTESIAN_POINT('Ctrl Pts',(-8.74520572331474,18.6809972942244,2.74678653993729));
#89466=CARTESIAN_POINT('Ctrl Pts',(-8.7480469901349,18.6812982320707,2.74207246856585));
#89467=CARTESIAN_POINT('Ctrl Pts',(-8.74953524924617,18.6814555770695,2.73961957648321));
#89468=CARTESIAN_POINT('Ctrl Pts',(-8.75316399382042,18.6818385023396,2.73367828263712));
#89469=CARTESIAN_POINT('Ctrl Pts',(-8.75531191171081,18.6820645603632,2.73019446426505));
#89470=CARTESIAN_POINT('Ctrl Pts',(-8.76294593512555,18.6828657638731,2.71792792887253));
#89471=CARTESIAN_POINT('Ctrl Pts',(-8.76851048461643,18.6834457354618,2.70919468584696));
#89472=CARTESIAN_POINT('Ctrl Pts',(-8.82812234263739,18.6896108577193,2.61779238159771));
#89473=CARTESIAN_POINT('Ctrl Pts',(-8.89030968622555,18.695616987207,2.54074391230127));
#89474=CARTESIAN_POINT('Ctrl Pts',(-9.02838495177893,18.7074193181971,2.40122341709625));
#89475=CARTESIAN_POINT('Ctrl Pts',(-9.10376226169663,18.7131836117415,2.33891898377669));
#89476=CARTESIAN_POINT('Ctrl Pts',(-9.19904284257417,18.7196024029165,2.27501247650816));
#89477=CARTESIAN_POINT('Ctrl Pts',(-9.2134636367918,18.7205534098203,2.26570368819759));
#89478=CARTESIAN_POINT('Ctrl Pts',(-9.23426110936365,18.7218965228191,2.2527912238526));
#89479=CARTESIAN_POINT('Ctrl Pts',(-9.24050586496314,18.722296236083,2.2489786406692));
#89480=CARTESIAN_POINT('Ctrl Pts',(-9.25115308112507,18.722971768689,2.24258735156718));
#89481=CARTESIAN_POINT('Ctrl Pts',(-9.25554086963213,18.7232484572739,2.23998457133406));
#89482=CARTESIAN_POINT('Ctrl Pts',(-9.26443476749019,18.7238058991792,2.23477150055442));
#89483=CARTESIAN_POINT('Ctrl Pts',(-9.26894137932951,18.7240866138239,2.2321622102194));
#89484=CARTESIAN_POINT('Ctrl Pts',(-9.28004891647597,18.724774270396,2.225809956376));
#89485=CARTESIAN_POINT('Ctrl Pts',(-9.28666525024447,18.7251802395231,2.22209414757217));
#89486=CARTESIAN_POINT('Ctrl Pts',(-9.31106422645601,18.7266642803851,2.20863994313104));
#89487=CARTESIAN_POINT('Ctrl Pts',(-9.32902022793352,18.7277311395461,2.19921965917409));
#89488=CARTESIAN_POINT('Ctrl Pts',(-9.42725372019766,18.7334418551944,2.15025884621249));
#89489=CARTESIAN_POINT('Ctrl Pts',(-9.5108347760018,18.7378373903956,2.11777028976397));
#89490=CARTESIAN_POINT('Ctrl Pts',(-9.69528033882753,18.7471738754549,2.06491864368276));
#89491=CARTESIAN_POINT('Ctrl Pts',(-9.79636786818284,18.7520789374639,2.04712660131601));
#89492=CARTESIAN_POINT('Ctrl Pts',(-9.90911196850621,18.7580496802623,2.03928597871431));
#89493=CARTESIAN_POINT('Ctrl Pts',(-9.91976313814106,18.7586187716164,2.03866221595384));
#89494=CARTESIAN_POINT('Ctrl Pts',(-9.93468121458127,18.7594240320447,2.03795215313455));
#89495=CARTESIAN_POINT('Ctrl Pts',(-9.93894337795214,18.7596550335478,2.03776796019554));
#89496=CARTESIAN_POINT('Ctrl Pts',(-9.94581894463226,18.7600292700937,2.03750094023769));
#89497=CARTESIAN_POINT('Ctrl Pts',(-9.94843190391166,18.7601718642918,2.03740647553399));
#89498=CARTESIAN_POINT('Ctrl Pts',(-9.95393194051589,18.7604728184479,2.03722239312029));
#89499=CARTESIAN_POINT('Ctrl Pts',(-9.95681904118807,18.7606312658007,2.03713432002078));
#89500=CARTESIAN_POINT('Ctrl Pts',(-9.96389610477852,18.7610207822941,2.03693939765707));
#89501=CARTESIAN_POINT('Ctrl Pts',(-9.96808628506719,18.7612523679918,2.03684200057313));
#89502=CARTESIAN_POINT('Ctrl Pts',(-9.98327034169327,18.7620949101606,2.03655431584109));
#89503=CARTESIAN_POINT('Ctrl Pts',(-9.99426557663278,18.7627113619199,2.0364699341982));
#89504=CARTESIAN_POINT('Ctrl Pts',(-10.0649999890705,18.7667133959952,2.03672418211309));
#89505=CARTESIAN_POINT('Ctrl Pts',(-10.1246652906782,18.7702536171005,2.04059656495621));
#89506=CARTESIAN_POINT('Ctrl Pts',(-10.1982460606775,18.7747011000034,2.0499175013927));
#89507=CARTESIAN_POINT('Ctrl Pts',(-10.2125434928297,18.7755692801554,2.05194405787678));
#89508=CARTESIAN_POINT('Ctrl Pts',(-10.3481711280124,18.7838322218326,2.07322024615524));
#89509=CARTESIAN_POINT('Ctrl Pts',(-10.4666778091345,18.7911997754611,2.10746778044932));
#89510=CARTESIAN_POINT('Ctrl Pts',(-10.5942714054837,18.7989601922179,2.16249047262196));
#89511=CARTESIAN_POINT('Ctrl Pts',(-10.608915178728,18.7998491676177,2.16909332663192));
#89512=CARTESIAN_POINT('Ctrl Pts',(-10.6292422630092,18.8010811854801,2.17866452195563));
#89513=CARTESIAN_POINT('Ctrl Pts',(-10.6350189046432,18.801431082406,2.1814309787995));
#89514=CARTESIAN_POINT('Ctrl Pts',(-10.6449999453007,18.802035303737,2.18629174450317));
#89515=CARTESIAN_POINT('Ctrl Pts',(-10.6492127355964,18.8022902272634,2.18836852178129));
#89516=CARTESIAN_POINT('Ctrl Pts',(-10.6578669933686,18.8028137202805,2.19268671755451));
#89517=CARTESIAN_POINT('Ctrl Pts',(-10.6623071797158,18.8030822008843,2.19493057657343));
#89518=CARTESIAN_POINT('Ctrl Pts',(-10.6726808868895,18.8037092529278,2.20023953197276));
#89519=CARTESIAN_POINT('Ctrl Pts',(-10.6786050677288,18.8040671891047,2.20332270248199));
#89520=CARTESIAN_POINT('Ctrl Pts',(-10.6910908468669,18.8048213386004,2.20992978505063));
#89521=CARTESIAN_POINT('Ctrl Pts',(-10.6976470814831,18.8052172005832,2.21346345930166));
#89522=CARTESIAN_POINT('Ctrl Pts',(-10.7152721691126,18.8062812227657,2.22313736538282));
#89523=CARTESIAN_POINT('Ctrl Pts',(-10.7262889344517,18.8069461135178,2.2293714704402));
#89524=CARTESIAN_POINT('Ctrl Pts',(-10.8197795298147,18.8125906660714,2.28388866377502));
#89525=CARTESIAN_POINT('Ctrl Pts',(-10.8974235835359,18.8172722031773,2.34000061921834));
#89526=CARTESIAN_POINT('Ctrl Pts',(-11.0426344495342,18.8266961752259,2.46830809838115));
#89527=CARTESIAN_POINT('Ctrl Pts',(-11.1094805591221,18.8314191755474,2.54056120241384));
#89528=CARTESIAN_POINT('Ctrl Pts',(-11.1751087459218,18.8371759796641,2.62760717380487));
#89529=CARTESIAN_POINT('Ctrl Pts',(-11.1815394503109,18.837754124242,2.6363366850984));
#89530=CARTESIAN_POINT('Ctrl Pts',(-11.1903814953133,18.8385701870271,2.64862311681924));
#89531=CARTESIAN_POINT('Ctrl Pts',(-11.1928752185691,18.8388027536703,2.65212063736747));
#89532=CARTESIAN_POINT('Ctrl Pts',(-11.1968651964447,18.8391788572451,2.65776914276756));
#89533=CARTESIAN_POINT('Ctrl Pts',(-11.1983711543682,18.8393217410231,2.65991328335112));
#89534=CARTESIAN_POINT('Ctrl Pts',(-11.2015219394555,18.8396226689237,2.66442499444997));
#89535=CARTESIAN_POINT('Ctrl Pts',(-11.2031655345118,18.8397807970039,2.66679338876023));
#89536=CARTESIAN_POINT('Ctrl Pts',(-11.2071655744408,18.8401684281312,2.67259389759016));
#89537=CARTESIAN_POINT('Ctrl Pts',(-11.2095143835328,18.8403984366162,2.67603122779192));
#89538=CARTESIAN_POINT('Ctrl Pts',(-11.2179091213831,18.8412290166541,2.68842962325464));
#89539=CARTESIAN_POINT('Ctrl Pts',(-11.2238702373381,18.8418348851805,2.69744736471882));
#89540=CARTESIAN_POINT('Ctrl Pts',(-11.2610278974344,18.8457108417614,2.75503482030055));
#89541=CARTESIAN_POINT('Ctrl Pts',(-11.2894251684542,18.8491258879651,2.80534468732222));
#89542=CARTESIAN_POINT('Ctrl Pts',(-11.3603170823029,18.8587955058051,2.95034487485124));
#89543=CARTESIAN_POINT('Ctrl Pts',(-11.3958362314279,18.8650966776298,3.04808334101784));
#89544=CARTESIAN_POINT('Ctrl Pts',(-11.428530157041,18.8729875691269,3.18032639978974));
#89545=CARTESIAN_POINT('Ctrl Pts',(-11.4352804511279,18.8748428025503,3.21214608978472));
#89546=CARTESIAN_POINT('Ctrl Pts',(-11.4441814339091,18.8776969539278,3.26228020459244));
#89547=CARTESIAN_POINT('Ctrl Pts',(-11.4470557275583,18.8787176641047,3.2804539230847));
#89548=CARTESIAN_POINT('Ctrl Pts',(-11.4506210494256,18.8801404540088,3.30612540022741));
#89549=CARTESIAN_POINT('Ctrl Pts',(-11.4515980169538,18.880551428578,3.31358114470718));
#89550=CARTESIAN_POINT('Ctrl Pts',(-11.4530890471029,18.881214955985,3.32568327950151));
#89551=CARTESIAN_POINT('Ctrl Pts',(-11.453638377954,18.8814686072157,3.33032512059649));
#89552=CARTESIAN_POINT('Ctrl Pts',(-11.4546996683609,18.881977937171,3.33967667889566));
#89553=CARTESIAN_POINT('Ctrl Pts',(-11.455211016886,18.8822335939466,3.34438640971473));
#89554=CARTESIAN_POINT('Ctrl Pts',(-11.4562112003746,18.8827556143257,3.3540348715201));
#89555=CARTESIAN_POINT('Ctrl Pts',(-11.4566978010851,18.8830219053279,3.3589737755919));
#89556=CARTESIAN_POINT('Ctrl Pts',(-11.4577688305633,18.8836381435864,3.37044206157947));
#89557=CARTESIAN_POINT('Ctrl Pts',(-11.4583345328788,18.8839875075812,3.37697311326332));
#89558=CARTESIAN_POINT('Ctrl Pts',(-11.4600523568521,18.8851332574215,3.39848578774896));
#89559=CARTESIAN_POINT('Ctrl Pts',(-11.4610176633964,18.885923903218,3.41348162672928));
#89560=CARTESIAN_POINT('Ctrl Pts',(-11.4629170959972,18.8879521529579,3.45230837672371));
#89561=CARTESIAN_POINT('Ctrl Pts',(-11.4635,18.8891793096102,3.47615209647377));
#89562=CARTESIAN_POINT('Ctrl Pts',(-11.4635,18.8903920399481,3.49999999999848));
#89563=CARTESIAN_POINT('Origin',(-10.,13.2,3.5));
#89564=CARTESIAN_POINT('',(-11.4635,19.4617257853095,3.50000000002413));
#89565=CARTESIAN_POINT('',(-11.4635,19.3881255777082,3.49999999999758));
#89566=CARTESIAN_POINT('',(-11.4635,13.2,3.5));
#89567=CARTESIAN_POINT('',(-11.4634997839299,18.9595020917114,3.50079525917368));
#89568=CARTESIAN_POINT('Ctrl Pts',(-11.4635,19.4617257853095,3.50000000002413));
#89569=CARTESIAN_POINT('Ctrl Pts',(-11.4635000000026,19.4524485230724,3.3412217020481));
#89570=CARTESIAN_POINT('Ctrl Pts',(-11.4376650484514,19.4425861276583,3.18348540399603));
#89571=CARTESIAN_POINT('Ctrl Pts',(-11.3783221719652,19.4320345915534,3.00725738649133));
#89572=CARTESIAN_POINT('Ctrl Pts',(-11.3689573148942,19.4305183273054,2.98180766057932));
#89573=CARTESIAN_POINT('Ctrl Pts',(-11.3556309158342,19.4285418047488,2.94848015531596));
#89574=CARTESIAN_POINT('Ctrl Pts',(-11.3522981584465,19.4280608332659,2.94035813735574));
#89575=CARTESIAN_POINT('Ctrl Pts',(-11.3467735026669,19.42728457902,2.92723196774772));
#89576=CARTESIAN_POINT('Ctrl Pts',(-11.3446263481021,19.426987802169,2.92220931872042));
#89577=CARTESIAN_POINT('Ctrl Pts',(-11.3404513020567,19.4264200030463,2.91259232618528));
#89578=CARTESIAN_POINT('Ctrl Pts',(-11.3384277875086,19.4261488379691,2.90799617658701));
#89579=CARTESIAN_POINT('Ctrl Pts',(-11.3337052068178,19.4255251255251,2.89741743638549));
#89580=CARTESIAN_POINT('Ctrl Pts',(-11.330989462413,19.425173150328,2.89144237945448));
#89581=CARTESIAN_POINT('Ctrl Pts',(-11.3223227572006,19.4240704968521,2.87270984642012));
#89582=CARTESIAN_POINT('Ctrl Pts',(-11.3162277773467,19.4233247416354,2.86001963517606));
#89583=CARTESIAN_POINT('Ctrl Pts',(-11.2854568896411,19.4196983183261,2.79825206581243));
#89584=CARTESIAN_POINT('Ctrl Pts',(-11.2582133820865,19.4169077474748,2.75050050609355));
#89585=CARTESIAN_POINT('Ctrl Pts',(-11.1709614261774,19.4089267219041,2.61579165080753));
#89586=CARTESIAN_POINT('Ctrl Pts',(-11.104162486679,19.4039360201529,2.533667497967));
#89587=CARTESIAN_POINT('Ctrl Pts',(-11.0219259393998,19.3981646355012,2.45233504232117));
#89588=CARTESIAN_POINT('Ctrl Pts',(-11.0146633423629,19.3976575064748,2.44529967053531));
#89589=CARTESIAN_POINT('Ctrl Pts',(-10.9907607225171,19.3959945233693,2.4226202853351));
#89590=CARTESIAN_POINT('Ctrl Pts',(-10.9738279133202,19.3948258907295,2.40729099817625));
#89591=CARTESIAN_POINT('Ctrl Pts',(-10.9443044568649,19.3927904753356,2.38179479541691));
#89592=CARTESIAN_POINT('Ctrl Pts',(-10.9318909066807,19.3919352733111,2.37142874323844));
#89593=CARTESIAN_POINT('Ctrl Pts',(-10.9153873143281,19.3907953094447,2.35810520901328));
#89594=CARTESIAN_POINT('Ctrl Pts',(-10.9114496992113,19.3905231053712,2.35495978532642));
#89595=CARTESIAN_POINT('Ctrl Pts',(-10.905085867791,19.3900826875053,2.34992988941526));
#89596=CARTESIAN_POINT('Ctrl Pts',(-10.9026697915969,19.3899153665694,2.34803258105276));
#89597=CARTESIAN_POINT('Ctrl Pts',(-10.8980167565477,19.3895928744069,2.3444022489014));
#89598=CARTESIAN_POINT('Ctrl Pts',(-10.8957807317323,19.3894377844098,2.34266809534273));
#89599=CARTESIAN_POINT('Ctrl Pts',(-10.8904696340765,19.3890691566503,2.33857367523647));
#89600=CARTESIAN_POINT('Ctrl Pts',(-10.8873901956392,19.3888552246634,2.33621912842635));
#89601=CARTESIAN_POINT('Ctrl Pts',(-10.8770896045394,19.3881390797345,2.32840792248312));
#89602=CARTESIAN_POINT('Ctrl Pts',(-10.8698273382458,19.3876332749473,2.32300613268513));
#89603=CARTESIAN_POINT('Ctrl Pts',(-10.8296007985981,19.3848288110455,2.29366061717046));
#89604=CARTESIAN_POINT('Ctrl Pts',(-10.7957001677799,19.3824556870078,2.27103584444739));
#89605=CARTESIAN_POINT('Ctrl Pts',(-10.680352843892,19.3744595974338,2.20082939784806));
#89606=CARTESIAN_POINT('Ctrl Pts',(-10.5952523625627,19.3687001125254,2.15970152865512));
#89607=CARTESIAN_POINT('Ctrl Pts',(-10.4393901202397,19.3588591008574,2.10216979943314));
#89608=CARTESIAN_POINT('Ctrl Pts',(-10.3702500096279,19.3547139126427,2.08228696008173));
#89609=CARTESIAN_POINT('Ctrl Pts',(-10.2896331116339,19.3501511161827,2.06540759108002));
#89610=CARTESIAN_POINT('Ctrl Pts',(-10.2793226725288,19.349572366234,2.06336449584378));
#89611=CARTESIAN_POINT('Ctrl Pts',(-10.262689972495,19.3486462973541,2.06025442578539));
#89612=CARTESIAN_POINT('Ctrl Pts',(-10.2563812790387,19.3482967877577,2.05911763779681));
#89613=CARTESIAN_POINT('Ctrl Pts',(-10.2451233704981,19.347676136775,2.05716531096991));
#89614=CARTESIAN_POINT('Ctrl Pts',(-10.2401770770362,19.3474044932385,2.05633370228128));
#89615=CARTESIAN_POINT('Ctrl Pts',(-10.2298145000246,19.3468375495628,2.05464619807104));
#89616=CARTESIAN_POINT('Ctrl Pts',(-10.2243974771326,19.3465424097218,2.05379528055222));
#89617=CARTESIAN_POINT('Ctrl Pts',(-10.2102011380848,19.345772091221,2.05164697379681));
#89618=CARTESIAN_POINT('Ctrl Pts',(-10.2014145054314,19.34529846393,2.05039894845542));
#89619=CARTESIAN_POINT('Ctrl Pts',(-10.1617971925706,19.3431765931866,2.0451390037453));
#89620=CARTESIAN_POINT('Ctrl Pts',(-10.1308536167949,19.3415566083917,2.0420300541232));
#89621=CARTESIAN_POINT('Ctrl Pts',(-10.0457844723548,19.3371853026616,2.03621349773804));
#89622=CARTESIAN_POINT('Ctrl Pts',(-9.99157003237367,19.334491790305,2.03552170208954));
#89623=CARTESIAN_POINT('Ctrl Pts',(-9.84606763351743,19.327350877629,2.04174722922775));
#89624=CARTESIAN_POINT('Ctrl Pts',(-9.75526945254689,19.3229954474432,2.05421250553614));
#89625=CARTESIAN_POINT('Ctrl Pts',(-9.62850193768208,19.3164453316802,2.08390563547147));
#89626=CARTESIAN_POINT('Ctrl Pts',(-9.5911389195793,19.3144523968771,2.09423821785307));
#89627=CARTESIAN_POINT('Ctrl Pts',(-9.54848556310275,19.3120593214827,2.10787810299123));
#89628=CARTESIAN_POINT('Ctrl Pts',(-9.54274950552511,19.3117349894782,2.10975158850731));
#89629=CARTESIAN_POINT('Ctrl Pts',(-9.53359123633073,19.311212893273,2.11280563028858));
#89630=CARTESIAN_POINT('Ctrl Pts',(-9.53016147366375,19.3110164077606,2.11396352400709));
#89631=CARTESIAN_POINT('Ctrl Pts',(-9.52408498371202,19.3106665310475,2.11604010304071));
#89632=CARTESIAN_POINT('Ctrl Pts',(-9.52143655692601,19.3105134396495,2.11695367757221));
#89633=CARTESIAN_POINT('Ctrl Pts',(-9.51579965186166,19.3101863049149,2.11891625747655));
#89634=CARTESIAN_POINT('Ctrl Pts',(-9.51281199829518,19.3100121453022,2.11996734400902));
#89635=CARTESIAN_POINT('Ctrl Pts',(-9.50467564682918,19.3095357894121,2.12285950827203));
#89636=CARTESIAN_POINT('Ctrl Pts',(-9.49953387137099,19.3092324982303,2.12471973730548));
#89637=CARTESIAN_POINT('Ctrl Pts',(-9.4727914080038,19.3076437406707,2.13456464942518));
#89638=CARTESIAN_POINT('Ctrl Pts',(-9.45137210010414,19.3063326011449,2.14302914507264));
#89639=CARTESIAN_POINT('Ctrl Pts',(-9.38707003955389,19.3022973956454,2.17021132186913));
#89640=CARTESIAN_POINT('Ctrl Pts',(-9.34487815567612,19.2995141595237,2.19048256889337));
#89641=CARTESIAN_POINT('Ctrl Pts',(-9.26719040448947,19.2942146194269,2.23250312849887));
#89642=CARTESIAN_POINT('Ctrl Pts',(-9.23150672551661,19.2917055362684,2.25381529490041));
#89643=CARTESIAN_POINT('Ctrl Pts',(-9.11231676879165,19.2831434999268,2.3320703966411));
#89644=CARTESIAN_POINT('Ctrl Pts',(-9.03381295054377,19.2772076913192,2.39612953280818));
#89645=CARTESIAN_POINT('Ctrl Pts',(-8.95504591408695,19.2710198370259,2.47529725484498));
#89646=CARTESIAN_POINT('Ctrl Pts',(-8.94764654684068,19.2704356845538,2.48289775560714));
#89647=CARTESIAN_POINT('Ctrl Pts',(-8.93588943315622,19.2695026889125,2.49524012478654));
#89648=CARTESIAN_POINT('Ctrl Pts',(-8.93147930777664,19.2691516022992,2.49993138362786));
#89649=CARTESIAN_POINT('Ctrl Pts',(-8.92368628174116,19.2685291501771,2.50833159424205));
#89650=CARTESIAN_POINT('Ctrl Pts',(-8.92029125487751,19.2682572722157,2.51202911294484));
#89651=CARTESIAN_POINT('Ctrl Pts',(-8.91323696348129,19.2676908354403,2.51979172308752));
#89652=CARTESIAN_POINT('Ctrl Pts',(-8.90958132329648,19.2673964307516,2.52386001296781));
#89653=CARTESIAN_POINT('Ctrl Pts',(-8.90009630243397,19.2666302150475,2.53453547971394));
#89654=CARTESIAN_POINT('Ctrl Pts',(-8.89430358326092,19.2661599246375,2.54117503034391));
#89655=CARTESIAN_POINT('Ctrl Pts',(-8.86876223180642,19.2640752308194,2.57098954588913));
#89656=CARTESIAN_POINT('Ctrl Pts',(-8.84967898401814,19.2624878547055,2.59472598410348));
#89657=CARTESIAN_POINT('Ctrl Pts',(-8.79973351710246,19.2582307599563,2.66098202371571));
#89658=CARTESIAN_POINT('Ctrl Pts',(-8.77039700663102,19.2556149532308,2.70459579877185));
#89659=CARTESIAN_POINT('Ctrl Pts',(-8.68913403800723,19.2478329577494,2.84068649317437));
#89660=CARTESIAN_POINT('Ctrl Pts',(-8.64485016577919,19.2428200578731,2.93730197707057));
#89661=CARTESIAN_POINT('Ctrl Pts',(-8.60263873539193,19.2359892470634,3.06413137353829));
#89662=CARTESIAN_POINT('Ctrl Pts',(-8.59463785285838,19.2345459040571,3.09066272712875));
#89663=CARTESIAN_POINT('Ctrl Pts',(-8.58596164926306,19.2327688523476,3.12269658637106));
#89664=CARTESIAN_POINT('Ctrl Pts',(-8.58455779865475,19.2324736600671,3.12799772037629));
#89665=CARTESIAN_POINT('Ctrl Pts',(-8.58230852278426,19.2319877130592,3.13668838656857));
#89666=CARTESIAN_POINT('Ctrl Pts',(-8.58144536897563,19.2317979435292,3.14007332509899));
#89667=CARTESIAN_POINT('Ctrl Pts',(-8.57991601569942,19.2314556609791,3.14616178783846));
#89668=CARTESIAN_POINT('Ctrl Pts',(-8.57924540527199,19.2313034021861,3.14886415132922));
#89669=CARTESIAN_POINT('Ctrl Pts',(-8.57779804676516,19.2309699834298,3.15476861290011));
#89670=CARTESIAN_POINT('Ctrl Pts',(-8.57702440897239,19.2307886541447,3.15797138522856));
#89671=CARTESIAN_POINT('Ctrl Pts',(-8.57486018795554,19.230272497008,3.16706546068466));
#89672=CARTESIAN_POINT('Ctrl Pts',(-8.57349534783142,19.2299362558809,3.17296274512755));
#89673=CARTESIAN_POINT('Ctrl Pts',(-8.56499619218746,19.227772651871,3.21075213362819));
#89674=CARTESIAN_POINT('Ctrl Pts',(-8.55889572602779,19.2258932815956,3.24286500192575));
#89675=CARTESIAN_POINT('Ctrl Pts',(-8.54132305107115,19.2191989107634,3.35588505618728));
#89676=CARTESIAN_POINT('Ctrl Pts',(-8.53555341202188,19.2142297614304,3.43752451107034));
#89677=CARTESIAN_POINT('Ctrl Pts',(-8.5378977806997,19.2035218500461,3.61605195314118));
#89678=CARTESIAN_POINT('Ctrl Pts',(-8.54877797047256,19.1978466268146,3.71253515469245));
#89679=CARTESIAN_POINT('Ctrl Pts',(-8.571360226001,19.1918855814505,3.81770263479479));
#89680=CARTESIAN_POINT('Ctrl Pts',(-8.5737194396154,19.191296671026,3.82813158886203));
#89681=CARTESIAN_POINT('Ctrl Pts',(-8.57768790715829,19.1903575797684,3.84482218291235));
#89682=CARTESIAN_POINT('Ctrl Pts',(-8.5792246970207,19.1900051085473,3.85110050924547));
#89683=CARTESIAN_POINT('Ctrl Pts',(-8.58202967401712,19.1893810704679,3.86223975230408));
#89684=CARTESIAN_POINT('Ctrl Pts',(-8.58328138306868,19.1891089820984,3.86710467830216));
#89685=CARTESIAN_POINT('Ctrl Pts',(-8.58594517343029,19.1885429674895,3.87724127615743));
#89686=CARTESIAN_POINT('Ctrl Pts',(-8.58736174575787,19.1882491900568,3.88251169490943));
#89687=CARTESIAN_POINT('Ctrl Pts',(-8.59112800416835,19.1874864777828,3.89621790774856));
#89688=CARTESIAN_POINT('Ctrl Pts',(-8.5935239999163,19.1870190374626,3.90464082436167));
#89689=CARTESIAN_POINT('Ctrl Pts',(-8.60443687727148,19.1849655295444,3.94173568266471));
#89690=CARTESIAN_POINT('Ctrl Pts',(-8.61375624750092,19.1834054797222,3.97016514612553));
#89691=CARTESIAN_POINT('Ctrl Pts',(-8.64136026491014,19.1792429169887,4.04639531394243));
#89692=CARTESIAN_POINT('Ctrl Pts',(-8.66129102499622,19.176691217273,4.09355588507725));
#89693=CARTESIAN_POINT('Ctrl Pts',(-8.72434143447789,19.1696000335026,4.22332311603181));
#89694=CARTESIAN_POINT('Ctrl Pts',(-8.77292702672683,19.1651715642419,4.30298900748788));
#89695=CARTESIAN_POINT('Ctrl Pts',(-8.85354707607167,19.1584286167577,4.41059800253315));
#89696=CARTESIAN_POINT('Ctrl Pts',(-8.8797370631283,19.1563077281068,4.4426311048685));
#89697=CARTESIAN_POINT('Ctrl Pts',(-8.91171439053565,19.1537396173159,4.47852532434047));
#89698=CARTESIAN_POINT('Ctrl Pts',(-8.91621738480605,19.1533784387528,4.48351035464096));
#89699=CARTESIAN_POINT('Ctrl Pts',(-8.92310438865228,19.1528264175971,4.49102986714121));
#89700=CARTESIAN_POINT('Ctrl Pts',(-8.92546344206393,19.1526373957696,4.4935872082774));
#89701=CARTESIAN_POINT('Ctrl Pts',(-8.92972627462679,19.152295897515,4.49817541120781));
#89702=CARTESIAN_POINT('Ctrl Pts',(-8.93162674771857,19.1521436699795,4.50020927428896));
#89703=CARTESIAN_POINT('Ctrl Pts',(-8.93579729643342,19.1518096454743,4.50464709607204));
#89704=CARTESIAN_POINT('Ctrl Pts',(-8.93806969200833,19.1516276745681,4.50704875872401));
#89705=CARTESIAN_POINT('Ctrl Pts',(-8.94456210899373,19.1511079040361,4.51386409220888));
#89706=CARTESIAN_POINT('Ctrl Pts',(-8.94880159119083,19.1507686604302,4.5182590249448));
#89707=CARTESIAN_POINT('Ctrl Pts',(-8.97668493832947,19.1485392716742,4.54680506536336));
#89708=CARTESIAN_POINT('Ctrl Pts',(-9.001130224203,19.1465934988796,4.5701557736849));
#89709=CARTESIAN_POINT('Ctrl Pts',(-9.09645481502427,19.1391112196426,4.65509872569979));
#89710=CARTESIAN_POINT('Ctrl Pts',(-9.17239646759694,19.1333745877624,4.71066900008591));
#89711=CARTESIAN_POINT('Ctrl Pts',(-9.3249163251688,19.1227978244221,4.80117668905939));
#89712=CARTESIAN_POINT('Ctrl Pts',(-9.400215424835,19.1179466887933,4.83755780285789));
#89713=CARTESIAN_POINT('Ctrl Pts',(-9.48819707202169,19.112728041925,4.87113242719118));
#89714=CARTESIAN_POINT('Ctrl Pts',(-9.49821931849686,19.1121396501248,4.87483181741007));
#89715=CARTESIAN_POINT('Ctrl Pts',(-9.51436658934363,19.1112012230839,4.88059196818485));
#89716=CARTESIAN_POINT('Ctrl Pts',(-9.52046618965083,19.1108489025931,4.882722430124));
#89717=CARTESIAN_POINT('Ctrl Pts',(-9.53133260169763,19.1102250373651,4.88643728645773));
#89718=CARTESIAN_POINT('Ctrl Pts',(-9.53609380961473,19.1099529721035,4.88803765327444));
#89719=CARTESIAN_POINT('Ctrl Pts',(-9.54604628235298,19.1093869125499,4.89132601113578));
#89720=CARTESIAN_POINT('Ctrl Pts',(-9.55123894862432,19.1090930676393,4.89300953582749));
#89721=CARTESIAN_POINT('Ctrl Pts',(-9.56479141957688,19.108329978341,4.89731976470854));
#89722=CARTESIAN_POINT('Ctrl Pts',(-9.57316567954627,19.1078622312734,4.89990053243183));
#89723=CARTESIAN_POINT('Ctrl Pts',(-9.61027892796517,19.1058053915191,4.91097404920086));
#89724=CARTESIAN_POINT('Ctrl Pts',(-9.63925266202821,19.1042424234472,4.91865845208204));
#89725=CARTESIAN_POINT('Ctrl Pts',(-9.71841524391045,19.1000698153711,4.93707152551713));
#89726=CARTESIAN_POINT('Ctrl Pts',(-9.76896607511278,19.0975113124651,4.94605961588683));
#89727=CARTESIAN_POINT('Ctrl Pts',(-9.91584444952054,19.090237691633,4.96427439282175));
#89728=CARTESIAN_POINT('Ctrl Pts',(-10.0127380826137,19.0856460104106,4.96663467823313));
#89729=CARTESIAN_POINT('Ctrl Pts',(-10.1468527378634,19.0788719116609,4.95660425529117));
#89730=CARTESIAN_POINT('Ctrl Pts',(-10.1844289326779,19.0769255190811,4.9523247553457));
#89731=CARTESIAN_POINT('Ctrl Pts',(-10.2277217809414,19.0745846396972,4.94568703522324));
#89732=CARTESIAN_POINT('Ctrl Pts',(-10.2336437132274,19.0742622841533,4.94474178528179));
#89733=CARTESIAN_POINT('Ctrl Pts',(-10.243119913875,19.0737427682739,4.94316942267513));
#89734=CARTESIAN_POINT('Ctrl Pts',(-10.2466780244964,19.0735468667013,4.9425655017117));
#89735=CARTESIAN_POINT('Ctrl Pts',(-10.2529928539392,19.0731976463438,4.94146963455314));
#89736=CARTESIAN_POINT('Ctrl Pts',(-10.255750436706,19.0730446233236,4.94098293033323));
#89737=CARTESIAN_POINT('Ctrl Pts',(-10.2616304624845,19.0727171926923,4.93992771469341));
#89738=CARTESIAN_POINT('Ctrl Pts',(-10.264752408592,19.0725426660079,4.93935696899386));
#89739=CARTESIAN_POINT('Ctrl Pts',(-10.2732771284898,19.0720642940924,4.93776983005245));
#89740=CARTESIAN_POINT('Ctrl Pts',(-10.2786760139853,19.0717593386902,4.93673315212822));
#89741=CARTESIAN_POINT('Ctrl Pts',(-10.3070503523027,19.0701465902986,4.93111884847474));
#89742=CARTESIAN_POINT('Ctrl Pts',(-10.3299180609175,19.0688122148497,4.92602069479193));
#89743=CARTESIAN_POINT('Ctrl Pts',(-10.3993143190696,19.0646768191767,4.90879093602591));
#89744=CARTESIAN_POINT('Ctrl Pts',(-10.4453745519343,19.0618134842561,4.89491389567479));
#89745=CARTESIAN_POINT('Ctrl Pts',(-10.6015533422794,19.0518610518198,4.83933534920191));
#89746=CARTESIAN_POINT('Ctrl Pts',(-10.7072956744309,19.0447358639228,4.78663373496802));
#89747=CARTESIAN_POINT('Ctrl Pts',(-10.8292061074749,19.0364373843041,4.70625445152632));
#89748=CARTESIAN_POINT('Ctrl Pts',(-10.8523689734237,19.0348536701358,4.68999994114569));
#89749=CARTESIAN_POINT('Ctrl Pts',(-10.882197461977,19.0328038014142,4.66774974224451));
#89750=CARTESIAN_POINT('Ctrl Pts',(-10.8892988438916,19.0323149617858,4.66235080489159));
#89751=CARTESIAN_POINT('Ctrl Pts',(-10.9006930869062,19.0315291687146,4.6535226011869));
#89752=CARTESIAN_POINT('Ctrl Pts',(-10.9050167034869,19.0312306527563,4.65013355563903));
#89753=CARTESIAN_POINT('Ctrl Pts',(-10.9131080895021,19.0306713149452,4.64371728376321));
#89754=CARTESIAN_POINT('Ctrl Pts',(-10.9168801345462,19.03041028001,4.64069558951642));
#89755=CARTESIAN_POINT('Ctrl Pts',(-10.9255125347198,19.0298122083475,4.63370989805401));
#89756=CARTESIAN_POINT('Ctrl Pts',(-10.9303625348391,19.0294756835999,4.62973321643136));
#89757=CARTESIAN_POINT('Ctrl Pts',(-10.9404648942874,19.0287735690889,4.62134076687125));
#89758=CARTESIAN_POINT('Ctrl Pts',(-10.9457120712773,19.0284082311885,4.61691898238927));
#89759=CARTESIAN_POINT('Ctrl Pts',(-10.9594608528606,19.0274490641185,4.60516656268905));
#89760=CARTESIAN_POINT('Ctrl Pts',(-10.9679096354125,19.0268577074367,4.5977746609398));
#89761=CARTESIAN_POINT('Ctrl Pts',(-10.9931424155635,19.0250847871176,4.57518052432145));
#89762=CARTESIAN_POINT('Ctrl Pts',(-11.0096597861465,19.0239150240216,4.55968495370579));
#89763=CARTESIAN_POINT('Ctrl Pts',(-11.0707156452118,19.0195438407297,4.49968198920872));
#89764=CARTESIAN_POINT('Ctrl Pts',(-11.1127274369591,19.0164407865026,4.45269854547398));
#89765=CARTESIAN_POINT('Ctrl Pts',(-11.2162224705601,19.008261125164,4.32073501696944));
#89766=CARTESIAN_POINT('Ctrl Pts',(-11.271818271681,19.0032752039734,4.23162581080527));
#89767=CARTESIAN_POINT('Ctrl Pts',(-11.324354224812,18.9969774402849,4.12303404272962));
#89768=CARTESIAN_POINT('Ctrl Pts',(-11.331050762151,18.9961355313254,4.108596219519));
#89769=CARTESIAN_POINT('Ctrl Pts',(-11.3395433659732,18.9950109244557,4.08947511250625));
#89770=CARTESIAN_POINT('Ctrl Pts',(-11.3415529367248,18.9947403690034,4.08488721483336));
#89771=CARTESIAN_POINT('Ctrl Pts',(-11.3447542327214,18.9943019813114,4.0774752796125));
#89772=CARTESIAN_POINT('Ctrl Pts',(-11.3459607238252,18.994135027147,4.07465761506311));
#89773=CARTESIAN_POINT('Ctrl Pts',(-11.3482650872044,18.9938127460461,4.06922888860492));
#89774=CARTESIAN_POINT('Ctrl Pts',(-11.3493642377146,18.9936574970333,4.06661841345753));
#89775=CARTESIAN_POINT('Ctrl Pts',(-11.3519561614253,18.9932877782613,4.06041229886672));
#89776=CARTESIAN_POINT('Ctrl Pts',(-11.3534421735571,18.9930729078479,4.0568138730817));
#89777=CARTESIAN_POINT('Ctrl Pts',(-11.3583717677595,18.9923504038943,4.04474037484503));
#89778=CARTESIAN_POINT('Ctrl Pts',(-11.3617501698118,18.9918390926783,4.0362391273953));
#89779=CARTESIAN_POINT('Ctrl Pts',(-11.3800447281281,18.9889807957476,3.98891559194911));
#89780=CARTESIAN_POINT('Ctrl Pts',(-11.3933793656938,18.9865563240167,3.94950559920582));
#89781=CARTESIAN_POINT('Ctrl Pts',(-11.4437290608436,18.9758948947297,3.7767888706231));
#89782=CARTESIAN_POINT('Ctrl Pts',(-11.463424603677,18.9673935543336,3.63914799684217));
#89783=CARTESIAN_POINT('Ctrl Pts',(-11.4634997839299,18.9595020917114,3.50079525917368));
#89784=CARTESIAN_POINT('Ctrl Pts',(-11.463499784802,18.9595020000746,3.50079365260118));
#89785=CARTESIAN_POINT('Ctrl Pts',(-11.4634999282675,18.9594869104204,3.50052910137612));
#89786=CARTESIAN_POINT('Ctrl Pts',(-11.4635,18.9594718228119,3.50026455050034));
#89787=CARTESIAN_POINT('Ctrl Pts',(-11.4635,18.9594567372512,3.50000000000276));
#89788=CARTESIAN_POINT('',(-11.4634994779773,18.8904305419548,3.50076815470882));
#89789=CARTESIAN_POINT('Ctrl Pts',(-11.4635,18.8903920399481,3.49999999999848));
#89790=CARTESIAN_POINT('Ctrl Pts',(-11.4635,18.8904050895196,3.50025661510164));
#89791=CARTESIAN_POINT('Ctrl Pts',(-11.4634999325063,18.8904181374306,3.50051323068873));
#89792=CARTESIAN_POINT('Ctrl Pts',(-11.4634997975183,18.8904311836853,3.50076984673329));
#89793=CARTESIAN_POINT('Ctrl Pts',(-11.4634997984221,18.890431096239,3.50076812669027));
#89794=CARTESIAN_POINT('Ctrl Pts',(-11.4634937883446,18.8910132559842,3.51221903341649));
#89795=CARTESIAN_POINT('Ctrl Pts',(-11.4633533849326,18.8915920540778,3.52366969261506));
#89796=CARTESIAN_POINT('Ctrl Pts',(-11.4597985251028,18.8990413693994,3.67177255314227));
#89797=CARTESIAN_POINT('Ctrl Pts',(-11.4373908907185,18.9053791212155,3.80727533817238));
#89798=CARTESIAN_POINT('Ctrl Pts',(-11.387649115658,18.9138592895339,3.96598437396818));
#89799=CARTESIAN_POINT('Ctrl Pts',(-11.3779237119127,18.9154017383441,3.99400152961883));
#89800=CARTESIAN_POINT('Ctrl Pts',(-11.3652526854024,18.9173062261339,4.02721165613559));
#89801=CARTESIAN_POINT('Ctrl Pts',(-11.3631172800626,18.9176239920481,4.03270846040276));
#89802=CARTESIAN_POINT('Ctrl Pts',(-11.3597492183937,18.9181205272658,4.04122541780645));
#89803=CARTESIAN_POINT('Ctrl Pts',(-11.3585395619885,18.918297956365,4.04425467190385));
#89804=CARTESIAN_POINT('Ctrl Pts',(-11.3562771197782,18.9186281866594,4.04986580073081));
#89805=CARTESIAN_POINT('Ctrl Pts',(-11.3552270771593,18.918780824336,4.05244872467638));
#89806=CARTESIAN_POINT('Ctrl Pts',(-11.3528275386992,18.9191282071699,4.05830316529903));
#89807=CARTESIAN_POINT('Ctrl Pts',(-11.3514735598145,18.919323217104,4.06157278283855));
#89808=CARTESIAN_POINT('Ctrl Pts',(-11.3473178487401,18.9199186452004,4.07150600877889));
#89809=CARTESIAN_POINT('Ctrl Pts',(-11.3444786363621,18.9203212209716,4.07815369547151));
#89810=CARTESIAN_POINT('Ctrl Pts',(-11.3119708262875,18.9248815707213,4.15273245892959));
#89811=CARTESIAN_POINT('Ctrl Pts',(-11.2772342277427,18.9292997755313,4.21832970371251));
#89812=CARTESIAN_POINT('Ctrl Pts',(-11.1869509978999,18.9394720120493,4.36140421947868));
#89813=CARTESIAN_POINT('Ctrl Pts',(-11.1284992205411,18.9452158305324,4.4366765185587));
#89814=CARTESIAN_POINT('Ctrl Pts',(-11.0434421340565,18.952368274697,4.52658830911708));
#89815=CARTESIAN_POINT('Ctrl Pts',(-11.0231203673566,18.9540035229907,4.54684283129346));
#89816=CARTESIAN_POINT('Ctrl Pts',(-10.9925357526582,18.9563592854659,4.57558424463029));
#89817=CARTESIAN_POINT('Ctrl Pts',(-10.9827325184723,18.9570994036766,4.58454852404956));
#89818=CARTESIAN_POINT('Ctrl Pts',(-10.9648557884184,18.9584226203781,4.60045393613906));
#89819=CARTESIAN_POINT('Ctrl Pts',(-10.9568261076936,18.9590076642827,4.60744271457308));
#89820=CARTESIAN_POINT('Ctrl Pts',(-10.9443106959637,18.9599054731251,4.61809798537478));
#89821=CARTESIAN_POINT('Ctrl Pts',(-10.9398783596608,18.9602207615261,4.62182639735366));
#89822=CARTESIAN_POINT('Ctrl Pts',(-10.9319542137566,18.9607797477126,4.62841213584912));
#89823=CARTESIAN_POINT('Ctrl Pts',(-10.9284711232963,18.9610238615502,4.63127979682628));
#89824=CARTESIAN_POINT('Ctrl Pts',(-10.9205854667354,18.9615729843872,4.63771118041038));
#89825=CARTESIAN_POINT('Ctrl Pts',(-10.916175346408,18.9618776168836,4.64126555519157));
#89826=CARTESIAN_POINT('Ctrl Pts',(-10.9041665594707,18.9627005464271,4.65082967305957));
#89827=CARTESIAN_POINT('Ctrl Pts',(-10.8965286005457,18.9632168771588,4.65678977265509));
#89828=CARTESIAN_POINT('Ctrl Pts',(-10.8605850313518,18.9656146365331,4.68426763776586));
#89829=CARTESIAN_POINT('Ctrl Pts',(-10.8315593563729,18.9674587825877,4.70482601898135));
#89830=CARTESIAN_POINT('Ctrl Pts',(-10.6768666882513,18.9768794888153,4.80613585849699));
#89831=CARTESIAN_POINT('Ctrl Pts',(-10.5401525374523,18.9837566537663,4.8683442937853));
#89832=CARTESIAN_POINT('Ctrl Pts',(-10.3670465804022,18.9929137665057,4.91705305941306));
#89833=CARTESIAN_POINT('Ctrl Pts',(-10.3374365873845,18.994498786133,4.92439420731395));
#89834=CARTESIAN_POINT('Ctrl Pts',(-10.3018105211813,18.9964509132998,4.93205376371408));
#89835=CARTESIAN_POINT('Ctrl Pts',(-10.2959925379804,18.9967711333796,4.93326759116886));
#89836=CARTESIAN_POINT('Ctrl Pts',(-10.2869604908855,18.9972706829159,4.93509464214676));
#89837=CARTESIAN_POINT('Ctrl Pts',(-10.283751424121,18.9974486458808,4.93573259492423));
#89838=CARTESIAN_POINT('Ctrl Pts',(-10.2778046587712,18.9977793533087,4.93689407774314));
#89839=CARTESIAN_POINT('Ctrl Pts',(-10.2750675889424,18.9979319301875,4.93742055092653));
#89840=CARTESIAN_POINT('Ctrl Pts',(-10.2688650878725,18.9982785068563,4.93859523278231));
#89841=CARTESIAN_POINT('Ctrl Pts',(-10.2653988252634,18.9984727662671,4.93923873706635));
#89842=CARTESIAN_POINT('Ctrl Pts',(-10.256432914147,18.9989766672973,4.94086974844446));
#89843=CARTESIAN_POINT('Ctrl Pts',(-10.2509299264486,18.9992873297414,4.94183828545735));
#89844=CARTESIAN_POINT('Ctrl Pts',(-10.2163927309197,19.0012451604467,4.94771319515197));
#89845=CARTESIAN_POINT('Ctrl Pts',(-10.1872233581509,19.0029344011007,4.95177356486003));
#89846=CARTESIAN_POINT('Ctrl Pts',(-10.0535486374856,19.0107787775643,4.9662856637501));
#89847=CARTESIAN_POINT('Ctrl Pts',(-9.94822832933526,19.0172197176339,4.96634968180547));
#89848=CARTESIAN_POINT('Ctrl Pts',(-9.79225596596759,19.0265398495859,4.94960780672466));
#89849=CARTESIAN_POINT('Ctrl Pts',(-9.74103198219931,19.0295698839666,4.94133852745841));
#89850=CARTESIAN_POINT('Ctrl Pts',(-9.66085017601027,19.034239965734,4.92398059414231));
#89851=CARTESIAN_POINT('Ctrl Pts',(-9.63155259575886,19.0359310381326,4.91668275754192));
#89852=CARTESIAN_POINT('Ctrl Pts',(-9.59404390717099,19.0380772404299,4.90609711711246));
#89853=CARTESIAN_POINT('Ctrl Pts',(-9.58560927897287,19.0385586326944,4.90363449199275));
#89854=CARTESIAN_POINT('Ctrl Pts',(-9.57196510455479,19.0393354629141,4.89951714745544));
#89855=CARTESIAN_POINT('Ctrl Pts',(-9.56674183718933,19.0396323981674,4.89790896814791));
#89856=CARTESIAN_POINT('Ctrl Pts',(-9.55673517191959,19.0402004335404,4.8947665664988));
#89857=CARTESIAN_POINT('Ctrl Pts',(-9.55195043284844,19.0404716770047,4.89323690343059));
#89858=CARTESIAN_POINT('Ctrl Pts',(-9.54103686331703,19.0410895632117,4.88968584079911));
#89859=CARTESIAN_POINT('Ctrl Pts',(-9.53491331329074,19.0414356797211,4.88764846867514));
#89860=CARTESIAN_POINT('Ctrl Pts',(-9.51871695434973,19.0423497153297,4.88214050717547));
#89861=CARTESIAN_POINT('Ctrl Pts',(-9.50866812255637,19.0429153539751,4.87860028499092));
#89862=CARTESIAN_POINT('Ctrl Pts',(-9.40731908370013,19.0486076081573,4.84164589325476));
#89863=CARTESIAN_POINT('Ctrl Pts',(-9.3195223628312,19.0534120451214,4.79932197213555));
#89864=CARTESIAN_POINT('Ctrl Pts',(-9.16706909048235,19.0621159110974,4.70610666531665));
#89865=CARTESIAN_POINT('Ctrl Pts',(-9.10124840789684,19.0660277432525,4.6578907662122));
#89866=CARTESIAN_POINT('Ctrl Pts',(-9.01515863151058,19.071818597797,4.58304412866461));
#89867=CARTESIAN_POINT('Ctrl Pts',(-8.99125698261388,19.0735101552157,4.56081776065816));
#89868=CARTESIAN_POINT('Ctrl Pts',(-8.96382802089867,19.0755814937634,4.53354560137138));
#89869=CARTESIAN_POINT('Ctrl Pts',(-8.95956273294129,19.0759074976781,4.52925175304407));
#89870=CARTESIAN_POINT('Ctrl Pts',(-8.95301641303678,19.0764141471231,4.52257932615369));
#89871=CARTESIAN_POINT('Ctrl Pts',(-8.95071652498853,19.0765933633167,4.52021924029947));
#89872=CARTESIAN_POINT('Ctrl Pts',(-8.94648741532887,19.0769252113112,4.51585000984714));
#89873=CARTESIAN_POINT('Ctrl Pts',(-8.94455594716732,19.0770776660609,4.51384311387529));
#89874=CARTESIAN_POINT('Ctrl Pts',(-8.94021358505153,19.0774224431619,4.50930531674216));
#89875=CARTESIAN_POINT('Ctrl Pts',(-8.93780603636744,19.0776150135029,4.50677130015311));
#89876=CARTESIAN_POINT('Ctrl Pts',(-8.93164132279362,19.0781116951501,4.50023602879445));
#89877=CARTESIAN_POINT('Ctrl Pts',(-8.92789758245441,19.0784167803251,4.4962222547278));
#89878=CARTESIAN_POINT('Ctrl Pts',(-8.90535140255819,19.0802746575577,4.47177555831482));
#89879=CARTESIAN_POINT('Ctrl Pts',(-8.88711217990929,19.0818648600866,4.45083320471266));
#89880=CARTESIAN_POINT('Ctrl Pts',(-8.8635321302407,19.0840265088872,4.42215008601664));
#89881=CARTESIAN_POINT('Ctrl Pts',(-8.85765306791184,19.0845747830171,4.4148570822684));
#89882=CARTESIAN_POINT('Ctrl Pts',(-8.8512751973173,19.0851795038228,4.40678796896942));
#89883=CARTESIAN_POINT('Ctrl Pts',(-8.85070654763207,19.0852335085463,4.4060671350983));
#89884=CARTESIAN_POINT('Ctrl Pts',(-8.78803853945861,19.0911947704695,4.32647376028324));
#89885=CARTESIAN_POINT('Ctrl Pts',(-8.73421800636294,19.0973404764065,4.24142191718636));
#89886=CARTESIAN_POINT('Ctrl Pts',(-8.65971860638031,19.1072603280742,4.09157493574746));
#89887=CARTESIAN_POINT('Ctrl Pts',(-8.6340581858006,19.1111365537407,4.02964136141409));
#89888=CARTESIAN_POINT('Ctrl Pts',(-8.60775159136329,19.1157433380274,3.95135420443804));
#89889=CARTESIAN_POINT('Ctrl Pts',(-8.60301333184552,19.1166069801966,3.9364682403135));
#89890=CARTESIAN_POINT('Ctrl Pts',(-8.59654270853897,19.1178379467534,3.91495389520153));
#89891=CARTESIAN_POINT('Ctrl Pts',(-8.59461723860037,19.1182114996025,3.90838511271655));
#89892=CARTESIAN_POINT('Ctrl Pts',(-8.59134680292386,19.1188589687067,3.89693084194802));
#89893=CARTESIAN_POINT('Ctrl Pts',(-8.58998100329481,19.1191335535903,3.89205146696607));
#89894=CARTESIAN_POINT('Ctrl Pts',(-8.58739436163082,19.1196618462301,3.88262220393595));
#89895=CARTESIAN_POINT('Ctrl Pts',(-8.58617009497762,19.1199156613013,3.87807332737975));
#89896=CARTESIAN_POINT('Ctrl Pts',(-8.58299832183356,19.120583404227,3.86605742954535));
#89897=CARTESIAN_POINT('Ctrl Pts',(-8.58108785826273,19.1209961414884,3.85858072281213));
#89898=CARTESIAN_POINT('Ctrl Pts',(-8.57454284315463,19.1224487940204,3.83209480668695));
#89899=CARTESIAN_POINT('Ctrl Pts',(-8.57023033370002,19.12347846433,3.81300769267559));
#89900=CARTESIAN_POINT('Ctrl Pts',(-8.54092946320679,19.1310750692854,3.67004308906951));
#89901=CARTESIAN_POINT('Ctrl Pts',(-8.53169769971814,19.1370953083661,3.54348802515119));
#89902=CARTESIAN_POINT('Ctrl Pts',(-8.54166438968115,19.1457266435962,3.36736227577759));
#89903=CARTESIAN_POINT('Ctrl Pts',(-8.54705071643975,19.148202546586,3.31759045860735));
#89904=CARTESIAN_POINT('Ctrl Pts',(-8.55877824828366,19.1520121436158,3.24448312088082));
#89905=CARTESIAN_POINT('Ctrl Pts',(-8.5631650262296,19.153269944864,3.22086895784399));
#89906=CARTESIAN_POINT('Ctrl Pts',(-8.56927640379195,19.154855427326,3.19195300619819));
#89907=CARTESIAN_POINT('Ctrl Pts',(-8.57045306931451,19.1551543153173,3.18653783302719));
#89908=CARTESIAN_POINT('Ctrl Pts',(-8.57235419992102,19.1556276343702,3.17802196037888));
#89909=CARTESIAN_POINT('Ctrl Pts',(-8.57305809094665,19.1558009199294,3.17491666257417));
#89910=CARTESIAN_POINT('Ctrl Pts',(-8.57439986899663,19.1561276532861,3.16908558009046));
#89911=CARTESIAN_POINT('Ctrl Pts',(-8.57503544610246,19.1562809699356,3.16635931527085));
#89912=CARTESIAN_POINT('Ctrl Pts',(-8.57650513764595,19.1566322088916,3.16013598000003));
#89913=CARTESIAN_POINT('Ctrl Pts',(-8.57734431823989,19.1568304159127,3.15664015111482));
#89914=CARTESIAN_POINT('Ctrl Pts',(-8.57960595807513,19.1573583946805,3.14736932954402));
#89915=CARTESIAN_POINT('Ctrl Pts',(-8.58105074023388,19.1576893814363,3.1415999165177));
#89916=CARTESIAN_POINT('Ctrl Pts',(-8.59163331127443,19.1600690277061,3.10040798792131));
#89917=CARTESIAN_POINT('Ctrl Pts',(-8.60206059883461,19.1621824920263,3.06533287829992));
#89918=CARTESIAN_POINT('Ctrl Pts',(-8.61648311195782,19.1648275370238,3.02273297786068));
#89919=CARTESIAN_POINT('Ctrl Pts',(-8.61924481892797,19.1653234336311,3.01480115795194));
#89920=CARTESIAN_POINT('Ctrl Pts',(-8.65469549692082,19.1715562243935,2.91573857354387));
#89921=CARTESIAN_POINT('Ctrl Pts',(-8.69628123895668,19.1774723926981,2.82804431797812));
#89922=CARTESIAN_POINT('Ctrl Pts',(-8.77891485928773,19.1869427957533,2.69080306282505));
#89923=CARTESIAN_POINT('Ctrl Pts',(-8.81509969616742,19.1906019529537,2.63868618083177));
#89924=CARTESIAN_POINT('Ctrl Pts',(-8.86400209389244,19.1949812342604,2.57719372387759));
#89925=CARTESIAN_POINT('Ctrl Pts',(-8.87363474025282,19.195820083828,2.56546054552569));
#89926=CARTESIAN_POINT('Ctrl Pts',(-8.88782299585406,19.197022309762,2.548716472269));
#89927=CARTESIAN_POINT('Ctrl Pts',(-8.8922333446231,19.197391519909,2.54358425458789));
#89928=CARTESIAN_POINT('Ctrl Pts',(-8.89999963880857,19.1980339402669,2.53467259539743));
#89929=CARTESIAN_POINT('Ctrl Pts',(-8.90333983768092,19.1983077894451,2.53087963494174));
#89930=CARTESIAN_POINT('Ctrl Pts',(-8.90984485028935,19.1988364275771,2.52356957022177));
#89931=CARTESIAN_POINT('Ctrl Pts',(-8.91300719940275,19.1990913135192,2.52005036516622));
#89932=CARTESIAN_POINT('Ctrl Pts',(-8.92144544953346,19.1997659187328,2.51075100433232));
#89933=CARTESIAN_POINT('Ctrl Pts',(-8.9267507830111,19.2001843997546,2.50499768079893));
#89934=CARTESIAN_POINT('Ctrl Pts',(-8.94597537156872,19.2016809536736,2.48448240777051));
#89935=CARTESIAN_POINT('Ctrl Pts',(-8.960155438753,19.2027479213745,2.46996736024903));
#89936=CARTESIAN_POINT('Ctrl Pts',(-9.09416318526745,19.212513616109,2.33838270915207));
#89937=CARTESIAN_POINT('Ctrl Pts',(-9.23293114521216,19.2201624705963,2.24242743545717));
#89938=CARTESIAN_POINT('Ctrl Pts',(-9.41337924357198,19.2302757766424,2.1588463684646));
#89939=CARTESIAN_POINT('Ctrl Pts',(-9.44226829587132,19.2319048116769,2.14657765513481));
#89940=CARTESIAN_POINT('Ctrl Pts',(-9.47711248687387,19.2339061901083,2.13308494326703));
#89941=CARTESIAN_POINT('Ctrl Pts',(-9.48271094969269,19.2342288598946,2.13095647999957));
#89942=CARTESIAN_POINT('Ctrl Pts',(-9.49139696378548,19.2347314172632,2.12771505430884));
#89943=CARTESIAN_POINT('Ctrl Pts',(-9.49447552512786,19.2349099118896,2.12657798711041));
#89944=CARTESIAN_POINT('Ctrl Pts',(-9.50017494028386,19.2352410997588,2.12449466596413));
#89945=CARTESIAN_POINT('Ctrl Pts',(-9.50279468647932,19.2353936213885,2.12354553648829));
#89946=CARTESIAN_POINT('Ctrl Pts',(-9.50872299227258,19.235739419123,2.12141685435759));
#89947=CARTESIAN_POINT('Ctrl Pts',(-9.51203307970919,19.2359329498355,2.12024173423697));
#89948=CARTESIAN_POINT('Ctrl Pts',(-9.52057935936852,19.2364337326745,2.11724230420256));
#89949=CARTESIAN_POINT('Ctrl Pts',(-9.52582169825958,19.2367419852226,2.11543583315469));
#89950=CARTESIAN_POINT('Ctrl Pts',(-9.55827193135465,19.2386561109895,2.10445963208981));
#89951=CARTESIAN_POINT('Ctrl Pts',(-9.58573282842601,19.2403019849419,2.09606300294355));
#89952=CARTESIAN_POINT('Ctrl Pts',(-9.75525735872894,19.2505468179804,2.04963458489905));
#89953=CARTESIAN_POINT('Ctrl Pts',(-9.90214634706315,19.2596741607257,2.03238455393682));
#89954=CARTESIAN_POINT('Ctrl Pts',(-10.0885523410539,19.2704053424228,2.03864992541802));
#89955=CARTESIAN_POINT('Ctrl Pts',(-10.1278748760657,19.2726288003457,2.04156454008032));
#89956=CARTESIAN_POINT('Ctrl Pts',(-10.1765625422358,19.2753323780346,2.04715799267027));
#89957=CARTESIAN_POINT('Ctrl Pts',(-10.1860796339814,19.2758585277891,2.04834625149376));
#89958=CARTESIAN_POINT('Ctrl Pts',(-10.2011765746972,19.2766895919647,2.05038209326492));
#89959=CARTESIAN_POINT('Ctrl Pts',(-10.2067642747135,19.276996408987,2.05116853095995));
#89960=CARTESIAN_POINT('Ctrl Pts',(-10.2172800088412,19.2775723958659,2.05271063632221));
#89961=CARTESIAN_POINT('Ctrl Pts',(-10.2222089888003,19.2778417837619,2.0534592053439));
#89962=CARTESIAN_POINT('Ctrl Pts',(-10.2332996623311,19.2784466382635,2.05520158150741));
#89963=CARTESIAN_POINT('Ctrl Pts',(-10.2394590390122,19.2787816522177,2.05620965067414));
#89964=CARTESIAN_POINT('Ctrl Pts',(-10.2551924009508,19.2796351936729,2.05888809050786));
#89965=CARTESIAN_POINT('Ctrl Pts',(-10.2647566218842,19.2801519574655,2.06061449416049));
#89966=CARTESIAN_POINT('Ctrl Pts',(-10.3235700280896,19.2833177802144,2.07183674237607));
#89967=CARTESIAN_POINT('Ctrl Pts',(-10.3723237665449,19.2858888397729,2.08376430349396));
#89968=CARTESIAN_POINT('Ctrl Pts',(-10.5485961943378,19.2951170768274,2.13662394302789));
#89969=CARTESIAN_POINT('Ctrl Pts',(-10.6709215073448,19.3013339623607,2.19247949114761));
#89970=CARTESIAN_POINT('Ctrl Pts',(-10.8087960320802,19.3096615597938,2.27993951042481));
#89971=CARTESIAN_POINT('Ctrl Pts',(-10.8331682471934,19.3111930592952,2.29645147229864));
#89972=CARTESIAN_POINT('Ctrl Pts',(-10.8617947014911,19.3130852928861,2.31713197074493));
#89973=CARTESIAN_POINT('Ctrl Pts',(-10.8665441021854,19.3134024136174,2.32060685148671));
#89974=CARTESIAN_POINT('Ctrl Pts',(-10.8738910568082,19.3138981562282,2.32605055754707));
#89975=CARTESIAN_POINT('Ctrl Pts',(-10.8765032636626,19.3140754447768,2.32799961562743));
#89976=CARTESIAN_POINT('Ctrl Pts',(-10.88133830005,19.3144055503658,2.3316324093787));
#89977=CARTESIAN_POINT('Ctrl Pts',(-10.8835628398947,19.3145582049613,2.33331378103655));
#89978=CARTESIAN_POINT('Ctrl Pts',(-10.8886025084914,19.314905804154,2.33714558902756));
#89979=CARTESIAN_POINT('Ctrl Pts',(-10.8914146307227,19.3151010149067,2.33929988592921));
#89980=CARTESIAN_POINT('Ctrl Pts',(-10.8999555181905,19.315697651573,2.3458921929956));
#89981=CARTESIAN_POINT('Ctrl Pts',(-10.9056590770935,19.3161012476319,2.3503624934034));
#89982=CARTESIAN_POINT('Ctrl Pts',(-10.9604902932024,19.3200295040541,2.39399901880944));
#89983=CARTESIAN_POINT('Ctrl Pts',(-11.0070762572335,19.3237421819597,2.43624459523901));
#89984=CARTESIAN_POINT('Ctrl Pts',(-11.1311819647378,19.3344240649125,2.56426674279092));
#89985=CARTESIAN_POINT('Ctrl Pts',(-11.2014805075467,19.3414422403673,2.65642386488544));
#89986=CARTESIAN_POINT('Ctrl Pts',(-11.2721345744582,19.3494031036046,2.77608315948565));
#89987=CARTESIAN_POINT('Ctrl Pts',(-11.2835691043462,19.3507305312622,2.796556747927));
#89988=CARTESIAN_POINT('Ctrl Pts',(-11.3023707265818,19.3529831670557,2.83220744705339));
#89989=CARTESIAN_POINT('Ctrl Pts',(-11.3099762370591,19.3539164019355,2.84725296249905));
#89990=CARTESIAN_POINT('Ctrl Pts',(-11.3203946098345,19.3552275371098,2.86877886449836));
#89991=CARTESIAN_POINT('Ctrl Pts',(-11.3234229301527,19.3556128386323,2.87515298034299));
#89992=CARTESIAN_POINT('Ctrl Pts',(-11.3285619102496,19.3562740849912,2.88617465766563));
#89993=CARTESIAN_POINT('Ctrl Pts',(-11.3306945591667,19.3565507798328,2.89081177672277));
#89994=CARTESIAN_POINT('Ctrl Pts',(-11.3347288783223,19.3570786491562,2.8997060638848));
#89995=CARTESIAN_POINT('Ctrl Pts',(-11.3366345449189,19.3573299573574,2.90396134153322));
#89996=CARTESIAN_POINT('Ctrl Pts',(-11.341054118556,19.3579174673861,2.91395786716575));
#89997=CARTESIAN_POINT('Ctrl Pts',(-11.3435515561416,19.3582531088152,2.91970632607008));
#89998=CARTESIAN_POINT('Ctrl Pts',(-11.3520025916107,19.3594017330883,2.93950548259117));
#89999=CARTESIAN_POINT('Ctrl Pts',(-11.3577734314809,19.360208581783,2.95363341647211));
#90000=CARTESIAN_POINT('Ctrl Pts',(-11.4107130486128,19.3678399690638,3.08925999274087));
#90001=CARTESIAN_POINT('Ctrl Pts',(-11.4416727951722,19.3740590932737,3.21645087969917));
#90002=CARTESIAN_POINT('Ctrl Pts',(-11.4607906234388,19.382943268054,3.39720327065946));
#90003=CARTESIAN_POINT('Ctrl Pts',(-11.4635,19.385483219807,3.44858563713104));
#90004=CARTESIAN_POINT('Ctrl Pts',(-11.4635,19.3881255777082,3.49999999999758));
#90005=CARTESIAN_POINT('Origin',(-10.,13.2,3.5));
#90006=CARTESIAN_POINT('',(-11.4635,19.9607369088795,3.50000000007519));
#90007=CARTESIAN_POINT('',(-11.4635,19.889530718258,3.4999999999448));
#90008=CARTESIAN_POINT('',(-11.4635,13.2,3.5));
#90009=CARTESIAN_POINT('',(-11.4634994221272,19.9606728854432,3.49868359318153));
#90010=CARTESIAN_POINT('Ctrl Pts',(-11.4635,19.9607369088795,3.50000000007519));
#90011=CARTESIAN_POINT('Ctrl Pts',(-11.4635,19.9607155759167,3.49956121929246));
#90012=CARTESIAN_POINT('Ctrl Pts',(-11.4634998026698,19.9606942428785,3.49912243308542));
#90013=CARTESIAN_POINT('Ctrl Pts',(-11.4634994079946,19.9606729097263,3.49868364158582));
#90014=CARTESIAN_POINT('Ctrl Pts',(-11.4634994079501,19.9606729073219,3.49868359213058));
#90015=CARTESIAN_POINT('Ctrl Pts',(-11.4634137445551,19.956042766607,3.40344842169157));
#90016=CARTESIAN_POINT('Ctrl Pts',(-11.4540323528043,19.9514432767397,3.30845726190788));
#90017=CARTESIAN_POINT('Ctrl Pts',(-11.4341658037668,19.9460401280826,3.20837143954945));
#90018=CARTESIAN_POINT('Ctrl Pts',(-11.4327911374842,19.9456767153169,3.20169089370002));
#90019=CARTESIAN_POINT('Ctrl Pts',(-11.4302108123229,19.945012514577,3.18958057969233));
#90020=CARTESIAN_POINT('Ctrl Pts',(-11.4290207932211,19.9447125498405,3.18414757444547));
#90021=CARTESIAN_POINT('Ctrl Pts',(-11.4271000238858,19.9442379420016,3.17561144520711));
#90022=CARTESIAN_POINT('Ctrl Pts',(-11.4263900407649,19.9440644553884,3.17250364297565));
#90023=CARTESIAN_POINT('Ctrl Pts',(-11.4250379589305,19.9437376275442,3.1666729956909));
#90024=CARTESIAN_POINT('Ctrl Pts',(-11.4243982041104,19.9435844194613,3.16394965871794));
#90025=CARTESIAN_POINT('Ctrl Pts',(-11.4229205617866,19.9432337999986,3.15773959600882));
#90026=CARTESIAN_POINT('Ctrl Pts',(-11.4220776655418,19.9430361070718,3.15425410790757));
#90027=CARTESIAN_POINT('Ctrl Pts',(-11.4198096605747,19.9425102691521,3.14502421632571));
#90028=CARTESIAN_POINT('Ctrl Pts',(-11.4183625154802,19.9421809238922,3.13928535998554));
#90029=CARTESIAN_POINT('Ctrl Pts',(-11.4079209669034,19.9398478477394,3.09891245365048));
#90030=CARTESIAN_POINT('Ctrl Pts',(-11.3976944448366,19.9377821047575,3.06461223919841));
#90031=CARTESIAN_POINT('Ctrl Pts',(-11.38183488504,19.9348756600818,3.01776372784465));
#90032=CARTESIAN_POINT('Ctrl Pts',(-11.3772659615998,19.9340663509738,3.00486574745594));
#90033=CARTESIAN_POINT('Ctrl Pts',(-11.3597237666308,19.9310626316199,2.95746698529145));
#90034=CARTESIAN_POINT('Ctrl Pts',(-11.3456295550546,19.9288454497048,2.92339634274777));
#90035=CARTESIAN_POINT('Ctrl Pts',(-11.310057537937,19.9237069969352,2.84583561283726));
#90036=CARTESIAN_POINT('Ctrl Pts',(-11.2876733885248,19.9207877383682,2.80280611264914));
#90037=CARTESIAN_POINT('Ctrl Pts',(-11.2361885363111,19.9147338877698,2.71480560047531));
#90038=CARTESIAN_POINT('Ctrl Pts',(-11.2066706959746,19.9116131402043,2.67015719906115));
#90039=CARTESIAN_POINT('Ctrl Pts',(-11.1581488717457,19.90699428837,2.60484614158327));
#90040=CARTESIAN_POINT('Ctrl Pts',(-11.1408889258023,19.9054352779286,2.58294937543069));
#90041=CARTESIAN_POINT('Ctrl Pts',(-11.1189225181921,19.9035496118399,2.55666265585356));
#90042=CARTESIAN_POINT('Ctrl Pts',(-11.1147998470305,19.9031997514125,2.55179419457049));
#90043=CARTESIAN_POINT('Ctrl Pts',(-11.1067320421034,19.9025228395713,2.54239227767872));
#90044=CARTESIAN_POINT('Ctrl Pts',(-11.1027905640002,19.9021956490416,2.53785586509849));
#90045=CARTESIAN_POINT('Ctrl Pts',(-11.0955700654623,19.9016025554382,2.52964815168607));
#90046=CARTESIAN_POINT('Ctrl Pts',(-11.0923002658052,19.901336278605,2.52596888755771));
#90047=CARTESIAN_POINT('Ctrl Pts',(-11.0851397353979,19.9007581160934,2.51799307471616));
#90048=CARTESIAN_POINT('Ctrl Pts',(-11.081241906057,19.9004465325133,2.51370299171305));
#90049=CARTESIAN_POINT('Ctrl Pts',(-11.0705330424237,19.8995989211419,2.50205623276338));
#90050=CARTESIAN_POINT('Ctrl Pts',(-11.0636716705296,19.8990650220827,2.49474613082253));
#90051=CARTESIAN_POINT('Ctrl Pts',(-11.0284196591286,19.8963672211087,2.45795372319157));
#90052=CARTESIAN_POINT('Ctrl Pts',(-10.9988750550461,19.8942536648422,2.42959986209388));
#90053=CARTESIAN_POINT('Ctrl Pts',(-10.9580828980211,19.8914994527891,2.39361369338931));
#90054=CARTESIAN_POINT('Ctrl Pts',(-10.9478645134338,19.8908222990557,2.38484692783403));
#90055=CARTESIAN_POINT('Ctrl Pts',(-10.878613658334,19.8863120066616,2.32707348482156));
#90056=CARTESIAN_POINT('Ctrl Pts',(-10.8159256284579,19.8826145921874,2.28263220323446));
#90057=CARTESIAN_POINT('Ctrl Pts',(-10.7006323312488,19.8760710428404,2.21382052309578));
#90058=CARTESIAN_POINT('Ctrl Pts',(-10.6495288245896,19.8732464083486,2.18727202957116));
#90059=CARTESIAN_POINT('Ctrl Pts',(-10.5731768054225,19.8689588293042,2.15315873190921));
#90060=CARTESIAN_POINT('Ctrl Pts',(-10.5490753068879,19.8675958605482,2.14315469114894));
#90061=CARTESIAN_POINT('Ctrl Pts',(-10.519523059989,19.8658985816823,2.13180445748483));
#90062=CARTESIAN_POINT('Ctrl Pts',(-10.5143139991395,19.8655984397398,2.12983783415813));
#90063=CARTESIAN_POINT('Ctrl Pts',(-10.5060393396881,19.8651199401288,2.12676766289083));
#90064=CARTESIAN_POINT('Ctrl Pts',(-10.5029810063627,19.8649427147344,2.12564452494672));
#90065=CARTESIAN_POINT('Ctrl Pts',(-10.4972990851735,19.8646127254945,2.12357941005239));
#90066=CARTESIAN_POINT('Ctrl Pts',(-10.4946765425452,19.8644601239696,2.12263471133655));
#90067=CARTESIAN_POINT('Ctrl Pts',(-10.4887162388068,19.8641126474312,2.12050689445962));
#90068=CARTESIAN_POINT('Ctrl Pts',(-10.4853768872018,19.863917506455,2.1193283999687));
#90069=CARTESIAN_POINT('Ctrl Pts',(-10.4751935299055,19.863321091338,2.11577608936369));
#90070=CARTESIAN_POINT('Ctrl Pts',(-10.4683362538154,19.8629176486511,2.11344099491087));
#90071=CARTESIAN_POINT('Ctrl Pts',(-10.4019544400507,19.8589964636457,2.09138473063548));
#90072=CARTESIAN_POINT('Ctrl Pts',(-10.341243309482,19.8552914177431,2.07545946536196));
#90073=CARTESIAN_POINT('Ctrl Pts',(-10.1662376355533,19.8446107443839,2.04138409722124));
#90074=CARTESIAN_POINT('Ctrl Pts',(-10.0505327944258,19.8375852254356,2.03280931865867));
#90075=CARTESIAN_POINT('Ctrl Pts',(-9.91158568035819,19.8296172167755,2.03898481855261));
#90076=CARTESIAN_POINT('Ctrl Pts',(-9.88817999193968,19.8282891892406,2.04058956244162));
#90077=CARTESIAN_POINT('Ctrl Pts',(-9.848032610309,19.826035703083,2.04431374517357));
#90078=CARTESIAN_POINT('Ctrl Pts',(-9.83127090189589,19.8251022078473,2.04616125897734));
#90079=CARTESIAN_POINT('Ctrl Pts',(-9.8075451563331,19.82379085329,2.04919223485169));
#90080=CARTESIAN_POINT('Ctrl Pts',(-9.80055243369569,19.8234055874896,2.05013700336749));
#90081=CARTESIAN_POINT('Ctrl Pts',(-9.78851523630969,19.8227444542812,2.05185205164295));
#90082=CARTESIAN_POINT('Ctrl Pts',(-9.78346749742927,19.822467836695,2.05259820303716));
#90083=CARTESIAN_POINT('Ctrl Pts',(-9.7738169798387,19.8219401503499,2.05407634665203));
#90084=CARTESIAN_POINT('Ctrl Pts',(-9.76921360123617,19.8216889477474,2.05480395490498));
#90085=CARTESIAN_POINT('Ctrl Pts',(-9.75843155802166,19.8211017384344,2.05656099118922));
#90086=CARTESIAN_POINT('Ctrl Pts',(-9.75225584398058,19.8207662912435,2.0576081256702));
#90087=CARTESIAN_POINT('Ctrl Pts',(-9.73107243551469,19.819618601982,2.06133998177758));
#90088=CARTESIAN_POINT('Ctrl Pts',(-9.71609979308382,19.8188124819635,2.06421959252592));
#90089=CARTESIAN_POINT('Ctrl Pts',(-9.57352180475279,19.8111780721326,2.09395848544571));
#90090=CARTESIAN_POINT('Ctrl Pts',(-9.45000568237654,19.8049559802393,2.13752264926429));
#90091=CARTESIAN_POINT('Ctrl Pts',(-9.28793193910559,19.7960589220608,2.22036909480593));
#90092=CARTESIAN_POINT('Ctrl Pts',(-9.24325251606778,19.7935092898169,2.24627406565687));
#90093=CARTESIAN_POINT('Ctrl Pts',(-9.17954064616634,19.7895976833154,2.28786227981394));
#90094=CARTESIAN_POINT('Ctrl Pts',(-9.15938345317736,19.7883164287226,2.30175332866223));
#90095=CARTESIAN_POINT('Ctrl Pts',(-9.13507714125785,19.7867046767838,2.31941889017696));
#90096=CARTESIAN_POINT('Ctrl Pts',(-9.13058783459079,19.7864041191722,2.32272102156282));
#90097=CARTESIAN_POINT('Ctrl Pts',(-9.12355842121665,19.7859287816161,2.32795367527048));
#90098=CARTESIAN_POINT('Ctrl Pts',(-9.12100553274142,19.7857551640983,2.329867035563));
#90099=CARTESIAN_POINT('Ctrl Pts',(-9.116226226158,19.7854282311601,2.33347353636971));
#90100=CARTESIAN_POINT('Ctrl Pts',(-9.11399839475503,19.7852750499323,2.33516472034014));
#90101=CARTESIAN_POINT('Ctrl Pts',(-9.10892851882197,19.7849246743868,2.33903630686234));
#90102=CARTESIAN_POINT('Ctrl Pts',(-9.10608962539454,19.7847271999829,2.34122076176553));
#90103=CARTESIAN_POINT('Ctrl Pts',(-9.09859191401106,19.7842023209756,2.34703400511823));
#90104=CARTESIAN_POINT('Ctrl Pts',(-9.09394703981038,19.783873722902,2.35068056930586));
#90105=CARTESIAN_POINT('Ctrl Pts',(-9.06144994665411,19.7815512663168,2.37651257704863));
#90106=CARTESIAN_POINT('Ctrl Pts',(-9.03439550496941,19.7794959846328,2.39967834202384));
#90107=CARTESIAN_POINT('Ctrl Pts',(-8.93277701436523,19.7713770799739,2.49332656360102));
#90108=CARTESIAN_POINT('Ctrl Pts',(-8.86485773304225,19.7650917927627,2.57058649450229));
#90109=CARTESIAN_POINT('Ctrl Pts',(-8.76714163505637,19.7550710224111,2.70859861163956));
#90110=CARTESIAN_POINT('Ctrl Pts',(-8.73245005455498,19.7512217740035,2.76544237865106));
#90111=CARTESIAN_POINT('Ctrl Pts',(-8.69455815663255,19.7466432912847,2.8382628181346));
#90112=CARTESIAN_POINT('Ctrl Pts',(-8.68759418546321,19.745782796896,2.85218404731595));
#90113=CARTESIAN_POINT('Ctrl Pts',(-8.67789397716318,19.7445555504022,2.87237382561336));
#90114=CARTESIAN_POINT('Ctrl Pts',(-8.67497767910233,19.7441826199879,2.87855426484827));
#90115=CARTESIAN_POINT('Ctrl Pts',(-8.66997603532699,19.7435359490749,2.88934940957531));
#90116=CARTESIAN_POINT('Ctrl Pts',(-8.66787116848844,19.7432615437805,2.89395489661097));
#90117=CARTESIAN_POINT('Ctrl Pts',(-8.66385410917567,19.7427333999446,2.90286634263372));
#90118=CARTESIAN_POINT('Ctrl Pts',(-8.66193872644397,19.7424795553122,2.90717078745172));
#90119=CARTESIAN_POINT('Ctrl Pts',(-8.65744415039595,19.7418790130687,2.9174042186559));
#90120=CARTESIAN_POINT('Ctrl Pts',(-8.65488338383103,19.7415329413859,2.92334122353582));
#90121=CARTESIAN_POINT('Ctrl Pts',(-8.64595508593005,19.7403121028983,2.94442412070779));
#90122=CARTESIAN_POINT('Ctrl Pts',(-8.63980321477142,19.7394445631679,2.95966036508148));
#90123=CARTESIAN_POINT('Ctrl Pts',(-8.59140912326885,19.732387321404,3.08558494065421));
#90124=CARTESIAN_POINT('Ctrl Pts',(-8.56249427169595,19.7266807330681,3.20092154506376));
#90125=CARTESIAN_POINT('Ctrl Pts',(-8.54043625200066,19.718018778119,3.37740081448873));
#90126=CARTESIAN_POINT('Ctrl Pts',(-8.53666505748933,19.715109854666,3.43670081049282));
#90127=CARTESIAN_POINT('Ctrl Pts',(-8.53643367992204,19.7107054397737,3.52267295556827));
#90128=CARTESIAN_POINT('Ctrl Pts',(-8.53708792427982,19.7093161068906,3.54928000082999));
#90129=CARTESIAN_POINT('Ctrl Pts',(-8.53876325220548,19.7075831411918,3.58156029283086));
#90130=CARTESIAN_POINT('Ctrl Pts',(-8.53909290005057,19.7072750264397,3.58726601642025));
#90131=CARTESIAN_POINT('Ctrl Pts',(-8.53966060707512,19.7067903910223,3.5961846457714));
#90132=CARTESIAN_POINT('Ctrl Pts',(-8.53987587326326,19.7066151096075,3.59939900764801));
#90133=CARTESIAN_POINT('Ctrl Pts',(-8.54029751129362,19.7062868036667,3.60539777016742));
#90134=CARTESIAN_POINT('Ctrl Pts',(-8.5405012387892,19.7061339264532,3.60818230491921));
#90135=CARTESIAN_POINT('Ctrl Pts',(-8.5409853945846,19.7057832689559,3.61454930745263));
#90136=CARTESIAN_POINT('Ctrl Pts',(-8.54127104922889,19.7055852026814,3.61813132636036));
#90137=CARTESIAN_POINT('Ctrl Pts',(-8.54205344756484,19.705064803885,3.62750650098825));
#90138=CARTESIAN_POINT('Ctrl Pts',(-8.54257152351526,19.7047413389941,3.63329775388379));
#90139=CARTESIAN_POINT('Ctrl Pts',(-8.54633798821459,19.7025248119698,3.67275021392144));
#90140=CARTESIAN_POINT('Ctrl Pts',(-8.55071754288131,19.7005762988811,3.70629079347159));
#90141=CARTESIAN_POINT('Ctrl Pts',(-8.57274777077938,19.6926873348225,3.83901128282558));
#90142=CARTESIAN_POINT('Ctrl Pts',(-8.59945464158742,19.6865190039527,3.93640689355828));
#90143=CARTESIAN_POINT('Ctrl Pts',(-8.66123117777454,19.6763924792935,4.09531280814216));
#90144=CARTESIAN_POINT('Ctrl Pts',(-8.69112913346795,19.6723451386725,4.1584515761339));
#90145=CARTESIAN_POINT('Ctrl Pts',(-8.73326238610005,19.6675603275407,4.23311842180967));
#90146=CARTESIAN_POINT('Ctrl Pts',(-8.7413300823713,19.6666778858602,4.24688477668963));
#90147=CARTESIAN_POINT('Ctrl Pts',(-8.75320814921338,19.6654252674149,4.26641370531577));
#90148=CARTESIAN_POINT('Ctrl Pts',(-8.75683650109319,19.6650485541611,4.2722851831776));
#90149=CARTESIAN_POINT('Ctrl Pts',(-8.76320472565336,19.6643974671863,4.28242920238383));
#90150=CARTESIAN_POINT('Ctrl Pts',(-8.76592551748704,19.6641224026863,4.28671353102732));
#90151=CARTESIAN_POINT('Ctrl Pts',(-8.7712058238074,19.6635944820704,4.29493343177462));
#90152=CARTESIAN_POINT('Ctrl Pts',(-8.77376209275742,19.6633415111051,4.29887100582407));
#90153=CARTESIAN_POINT('Ctrl Pts',(-8.77984790768838,19.6627453224624,4.30814731333391));
#90154=CARTESIAN_POINT('Ctrl Pts',(-8.78339363028139,19.662402708906,4.31347535386647));
#90155=CARTESIAN_POINT('Ctrl Pts',(-8.79594833690625,19.6612058817682,4.33207520032044));
#90156=CARTESIAN_POINT('Ctrl Pts',(-8.8051406373841,19.6603585221528,4.34522226464615));
#90157=CARTESIAN_POINT('Ctrl Pts',(-8.88672891227969,19.6530754119513,4.45792004475657));
#90158=CARTESIAN_POINT('Ctrl Pts',(-8.9711972824844,19.6471681364316,4.54811767146009));
#90159=CARTESIAN_POINT('Ctrl Pts',(-9.10927710602421,19.6384223693583,4.66258765575071));
#90160=CARTESIAN_POINT('Ctrl Pts',(-9.15461998962888,19.6356570423598,4.69596367807828));
#90161=CARTESIAN_POINT('Ctrl Pts',(-9.22337796836966,19.6314486811779,4.74070755531096));
#90162=CARTESIAN_POINT('Ctrl Pts',(-9.24535484239603,19.6301012552783,4.75419597445641));
#90163=CARTESIAN_POINT('Ctrl Pts',(-9.27257698301564,19.6284152641202,4.76992915519647));
#90164=CARTESIAN_POINT('Ctrl Pts',(-9.27749519327278,19.62810999518,4.77273371409891));
#90165=CARTESIAN_POINT('Ctrl Pts',(-9.28522700281274,19.6276288602635,4.77708344112295));
#90166=CARTESIAN_POINT('Ctrl Pts',(-9.28802967658596,19.6274542043595,4.77864804042013));
#90167=CARTESIAN_POINT('Ctrl Pts',(-9.29328133325388,19.6271264224067,4.78155717054276));
#90168=CARTESIAN_POINT('Ctrl Pts',(-9.29572903096472,19.6269734387705,4.78290391574854));
#90169=CARTESIAN_POINT('Ctrl Pts',(-9.30134956332321,19.626621677513,4.78597545041253));
#90170=CARTESIAN_POINT('Ctrl Pts',(-9.30452492844998,19.6264226070416,4.78769550593635));
#90171=CARTESIAN_POINT('Ctrl Pts',(-9.312882000565,19.6258978590131,4.7921824991193));
#90172=CARTESIAN_POINT('Ctrl Pts',(-9.31807400404919,19.6255710189273,4.79492999419432));
#90173=CARTESIAN_POINT('Ctrl Pts',(-9.35435626943737,19.6232820160773,4.81385106239168));
#90174=CARTESIAN_POINT('Ctrl Pts',(-9.38599995462256,19.6212603318344,4.82893340745466));
#90175=CARTESIAN_POINT('Ctrl Pts',(-9.42647382145323,19.6186703599349,4.84647028659164));
#90176=CARTESIAN_POINT('Ctrl Pts',(-9.43482917189611,19.6181354607806,4.84999868171311));
#90177=CARTESIAN_POINT('Ctrl Pts',(-9.53192056583963,19.6119211107036,4.88994024236719));
#90178=CARTESIAN_POINT('Ctrl Pts',(-9.62399757590105,19.6060601650186,4.91762324028468));
#90179=CARTESIAN_POINT('Ctrl Pts',(-9.78189222149721,19.5965359725163,4.94861458435281));
#90180=CARTESIAN_POINT('Ctrl Pts',(-9.8464282850424,19.5927793476797,4.95687085410545));
#90181=CARTESIAN_POINT('Ctrl Pts',(-9.92665579746746,19.5882978209831,4.96174188744806));
#90182=CARTESIAN_POINT('Ctrl Pts',(-9.94201915791696,19.587447841252,4.9624318667499));
#90183=CARTESIAN_POINT('Ctrl Pts',(-9.96418876775474,19.5862327767526,4.96307759704093));
#90184=CARTESIAN_POINT('Ctrl Pts',(-9.97098794581049,19.5858616818992,4.96322821262309));
#90185=CARTESIAN_POINT('Ctrl Pts',(-9.98284556306865,19.5852171469707,4.96340820007504));
#90186=CARTESIAN_POINT('Ctrl Pts',(-9.98790352509332,19.5849430546479,4.96345874931301));
#90187=CARTESIAN_POINT('Ctrl Pts',(-9.9976815048502,19.5844147732169,4.96350577440856));
#90188=CARTESIAN_POINT('Ctrl Pts',(-10.0024014371083,19.5841604823555,4.96350564090653));
#90189=CARTESIAN_POINT('Ctrl Pts',(-10.0136200536952,19.5835577342547,4.96345105098093));
#90190=CARTESIAN_POINT('Ctrl Pts',(-10.0201185694611,19.5832099140434,4.96337614080986));
#90191=CARTESIAN_POINT('Ctrl Pts',(-10.0432431867641,19.5819767828504,4.96295550748489));
#90192=CARTESIAN_POINT('Ctrl Pts',(-10.0598639858717,19.5810988942023,4.9623696943485));
#90193=CARTESIAN_POINT('Ctrl Pts',(-10.1918530276353,19.5741869576191,4.95546349157989));
#90194=CARTESIAN_POINT('Ctrl Pts',(-10.3061122785802,19.5686086371621,4.93578530808741));
#90195=CARTESIAN_POINT('Ctrl Pts',(-10.4757500310807,19.5599949949133,4.88537590617138));
#90196=CARTESIAN_POINT('Ctrl Pts',(-10.5334606689696,19.5569917345533,4.86419323565645));
#90197=CARTESIAN_POINT('Ctrl Pts',(-10.6145044553621,19.5524591462504,4.82851535953255));
#90198=CARTESIAN_POINT('Ctrl Pts',(-10.6390327584642,19.5510431795133,4.81689245328271));
#90199=CARTESIAN_POINT('Ctrl Pts',(-10.6683463656569,19.5492803730599,4.80199018009279));
#90200=CARTESIAN_POINT('Ctrl Pts',(-10.6734550912476,19.5489705023101,4.79935504440227));
#90201=CARTESIAN_POINT('Ctrl Pts',(-10.6814088694462,19.54848370746,4.79519289215716));
#90202=CARTESIAN_POINT('Ctrl Pts',(-10.6842646741082,19.5483080407645,4.7936864112331));
#90203=CARTESIAN_POINT('Ctrl Pts',(-10.6895797389374,19.5479794076285,4.79086010998411));
#90204=CARTESIAN_POINT('Ctrl Pts',(-10.6920402213336,19.5478265915004,4.78954269861279));
#90205=CARTESIAN_POINT('Ctrl Pts',(-10.6976504905862,19.5474765936178,4.78651812209661));
#90206=CARTESIAN_POINT('Ctrl Pts',(-10.7007977770161,19.5472791299922,4.7848064292587));
#90207=CARTESIAN_POINT('Ctrl Pts',(-10.7090049861787,19.5467613357898,4.78030370318974));
#90208=CARTESIAN_POINT('Ctrl Pts',(-10.7140546686712,19.5464398907297,4.77749425467367));
#90209=CARTESIAN_POINT('Ctrl Pts',(-10.7479026614091,19.5442666412832,4.75839915218622));
#90210=CARTESIAN_POINT('Ctrl Pts',(-10.7761562413337,19.5423617532052,4.74117201757062));
#90211=CARTESIAN_POINT('Ctrl Pts',(-10.8193709285459,19.5393318979977,4.71276985944076));
#90212=CARTESIAN_POINT('Ctrl Pts',(-10.8347449692665,19.5382298450131,4.70223968055702));
#90213=CARTESIAN_POINT('Ctrl Pts',(-10.9129777569391,19.5325109077971,4.64643137033179));
#90214=CARTESIAN_POINT('Ctrl Pts',(-10.972370871376,19.5278002291315,4.59650743157249));
#90215=CARTESIAN_POINT('Ctrl Pts',(-11.0860126013559,19.518292613268,4.48445584413692));
#90216=CARTESIAN_POINT('Ctrl Pts',(-11.1395405602359,19.5135267088618,4.42196936214456));
#90217=CARTESIAN_POINT('Ctrl Pts',(-11.1942331072658,19.5083448190035,4.34603211461871));
#90218=CARTESIAN_POINT('Ctrl Pts',(-11.2008083000543,19.5077156784156,4.33667346702114));
#90219=CARTESIAN_POINT('Ctrl Pts',(-11.2106867920785,19.5067606859864,4.32225677950704));
#90220=CARTESIAN_POINT('Ctrl Pts',(-11.2140695043242,19.5064318503367,4.31725391412741));
#90221=CARTESIAN_POINT('Ctrl Pts',(-11.2199122772675,19.5058606321388,4.30849640230696));
#90222=CARTESIAN_POINT('Ctrl Pts',(-11.2223861941975,19.5056177340641,4.30475113521458));
#90223=CARTESIAN_POINT('Ctrl Pts',(-11.2279167792504,19.5050723460416,4.29629402661117));
#90224=CARTESIAN_POINT('Ctrl Pts',(-11.2309636427519,19.5047702220696,4.29157583655084));
#90225=CARTESIAN_POINT('Ctrl Pts',(-11.2390783965571,19.5039609896041,4.27884965535902));
#90226=CARTESIAN_POINT('Ctrl Pts',(-11.2440958382738,19.5034557362017,4.27080971019543));
#90227=CARTESIAN_POINT('Ctrl Pts',(-11.2664278807289,19.5011837549075,4.23423869191108));
#90228=CARTESIAN_POINT('Ctrl Pts',(-11.2828422439138,19.4994496066057,4.2051680883371));
#90229=CARTESIAN_POINT('Ctrl Pts',(-11.3076118965672,19.4967086028152,4.15756731916387));
#90230=CARTESIAN_POINT('Ctrl Pts',(-11.316599815457,19.4956835424412,4.13938143373197));
#90231=CARTESIAN_POINT('Ctrl Pts',(-11.3815681658965,19.4880135176368,4.00074285838403));
#90232=CARTESIAN_POINT('Ctrl Pts',(-11.4212877154875,19.481841213713,3.87337494196798));
#90233=CARTESIAN_POINT('Ctrl Pts',(-11.4481455384831,19.4735699988697,3.71346696718282));
#90234=CARTESIAN_POINT('Ctrl Pts',(-11.4521348330697,19.4720427424521,3.68438503750852));
#90235=CARTESIAN_POINT('Ctrl Pts',(-11.4558703979341,19.4701553302202,3.64935927968659));
#90236=CARTESIAN_POINT('Ctrl Pts',(-11.4564586066254,19.4698385350959,3.64351005136787));
#90237=CARTESIAN_POINT('Ctrl Pts',(-11.457317924449,19.4693432293857,3.63441475582111));
#90238=CARTESIAN_POINT('Ctrl Pts',(-11.4576134706745,19.4691660489122,3.63117099217267));
#90239=CARTESIAN_POINT('Ctrl Pts',(-11.4581418553068,19.4688360994474,3.62514931416747));
#90240=CARTESIAN_POINT('Ctrl Pts',(-11.4583775869423,19.4686834924334,3.62237170649832));
#90241=CARTESIAN_POINT('Ctrl Pts',(-11.4588948555638,19.4683359463758,3.61606290907804));
#90242=CARTESIAN_POINT('Ctrl Pts',(-11.4591715072062,19.4681407409272,3.61253137547976));
#90243=CARTESIAN_POINT('Ctrl Pts',(-11.4598557787738,19.4676326704406,3.6033693563878));
#90244=CARTESIAN_POINT('Ctrl Pts',(-11.4602436426691,19.4673187565338,3.59773750866249));
#90245=CARTESIAN_POINT('Ctrl Pts',(-11.462518878454,19.4652979615535,3.56165634540871));
#90246=CARTESIAN_POINT('Ctrl Pts',(-11.4634862001066,19.4635459198122,3.53115852443362));
#90247=CARTESIAN_POINT('Ctrl Pts',(-11.4634999512113,19.4617513002721,3.50043670964679));
#90248=CARTESIAN_POINT('Ctrl Pts',(-11.4635,19.4617385435116,3.50021835384036));
#90249=CARTESIAN_POINT('Ctrl Pts',(-11.4635,19.4617257853095,3.50000000002413));
#90250=CARTESIAN_POINT('',(-11.4634993701123,19.8894511250131,3.49867606424249));
#90251=CARTESIAN_POINT('Ctrl Pts',(-11.4635,19.3881255777082,3.49999999999758));
#90252=CARTESIAN_POINT('Ctrl Pts',(-11.4635,19.3881370392299,3.50022301552205));
#90253=CARTESIAN_POINT('Ctrl Pts',(-11.4634999490457,19.3881485027067,3.50044603164707));
#90254=CARTESIAN_POINT('Ctrl Pts',(-11.4634888518949,19.3893964453504,3.52472008708722));
#90255=CARTESIAN_POINT('Ctrl Pts',(-11.4628849790811,19.3906549537311,3.54876585650265));
#90256=CARTESIAN_POINT('Ctrl Pts',(-11.461402976112,19.3922519923169,3.57852810566533));
#90257=CARTESIAN_POINT('Ctrl Pts',(-11.4610831222154,19.3925619190849,3.58426998126322));
#90258=CARTESIAN_POINT('Ctrl Pts',(-11.4605286576543,19.3930506651495,3.59326815002381));
#90259=CARTESIAN_POINT('Ctrl Pts',(-11.4603169743387,19.393228239904,3.59652586011211));
#90260=CARTESIAN_POINT('Ctrl Pts',(-11.4599233417494,19.3935433614148,3.60228577791062));
#90261=CARTESIAN_POINT('Ctrl Pts',(-11.4597458567251,19.3936806582384,3.60478825160784));
#90262=CARTESIAN_POINT('Ctrl Pts',(-11.4593129048901,19.3940047119826,3.61067806849549));
#90263=CARTESIAN_POINT('Ctrl Pts',(-11.4590520806128,19.3941917631619,3.61406495869504));
#90264=CARTESIAN_POINT('Ctrl Pts',(-11.4582552911372,19.3947403259567,3.62396135268497));
#90265=CARTESIAN_POINT('Ctrl Pts',(-11.4576875440557,19.3951035365753,3.63046812535771));
#90266=CARTESIAN_POINT('Ctrl Pts',(-11.4528571950243,19.3979907279391,3.68185272219291));
#90267=CARTESIAN_POINT('Ctrl Pts',(-11.4465669915753,19.4006133688458,3.72651188545727));
#90268=CARTESIAN_POINT('Ctrl Pts',(-11.4204208431472,19.4089837066789,3.86537225020693));
#90269=CARTESIAN_POINT('Ctrl Pts',(-11.3933312749514,19.4148632640615,3.9579536784888));
#90270=CARTESIAN_POINT('Ctrl Pts',(-11.3313501279308,19.4246668279097,4.11169738273552));
#90271=CARTESIAN_POINT('Ctrl Pts',(-11.3007869957119,19.4286730746124,4.17425678720106));
#90272=CARTESIAN_POINT('Ctrl Pts',(-11.2606401269891,19.4331044912688,4.24345681886297));
#90273=CARTESIAN_POINT('Ctrl Pts',(-11.2552964014634,19.4336801780356,4.25244436587787));
#90274=CARTESIAN_POINT('Ctrl Pts',(-11.2465297059245,19.4346023787075,4.26683560160738));
#90275=CARTESIAN_POINT('Ctrl Pts',(-11.2431668941995,19.4349510531361,4.2722753541504));
#90276=CARTESIAN_POINT('Ctrl Pts',(-11.2371035750247,19.4355708292823,4.28194126675532));
#90277=CARTESIAN_POINT('Ctrl Pts',(-11.2344168122376,19.43584242725,4.28617589286897));
#90278=CARTESIAN_POINT('Ctrl Pts',(-11.2287411675719,19.4364098883857,4.29502048830991));
#90279=CARTESIAN_POINT('Ctrl Pts',(-11.225747982341,19.436705587331,4.29962761247738));
#90280=CARTESIAN_POINT('Ctrl Pts',(-11.2178287923076,19.4374787240333,4.3116679108839));
#90281=CARTESIAN_POINT('Ctrl Pts',(-11.2128606297635,19.4379545900671,4.31907317282511));
#90282=CARTESIAN_POINT('Ctrl Pts',(-11.1900319996136,19.4401007504995,4.35243704071685));
#90283=CARTESIAN_POINT('Ctrl Pts',(-11.1714030771434,19.4417419697623,4.37786108729252));
#90284=CARTESIAN_POINT('Ctrl Pts',(-11.1178811024405,19.446188223003,4.44616497784161));
#90285=CARTESIAN_POINT('Ctrl Pts',(-11.0813571785017,19.4489328075118,4.4877011737487));
#90286=CARTESIAN_POINT('Ctrl Pts',(-11.0052302764448,19.4542473850178,4.5649766023865));
#90287=CARTESIAN_POINT('Ctrl Pts',(-10.9658521475789,19.4568164309644,4.6008145560141));
#90288=CARTESIAN_POINT('Ctrl Pts',(-10.8668395090666,19.4630566640221,4.68151429231231));
#90289=CARTESIAN_POINT('Ctrl Pts',(-10.8055630945377,19.466746884936,4.72411281085682));
#90290=CARTESIAN_POINT('Ctrl Pts',(-10.7350818208191,19.4711080266872,4.76551937648137));
#90291=CARTESIAN_POINT('Ctrl Pts',(-10.7288178976457,19.4714965995947,4.76913712550046));
#90292=CARTESIAN_POINT('Ctrl Pts',(-10.7194491340016,19.4720796198084,4.77445585424689));
#90293=CARTESIAN_POINT('Ctrl Pts',(-10.7163644282492,19.4722718768891,4.77619229986725));
#90294=CARTESIAN_POINT('Ctrl Pts',(-10.7108387369449,19.4726168515441,4.77927648100102));
#90295=CARTESIAN_POINT('Ctrl Pts',(-10.708400170501,19.4727692974872,4.78062844848033));
#90296=CARTESIAN_POINT('Ctrl Pts',(-10.703101075647,19.4731010220007,4.78354655640935));
#90297=CARTESIAN_POINT('Ctrl Pts',(-10.700239211046,19.4732804557987,4.78511008553037));
#90298=CARTESIAN_POINT('Ctrl Pts',(-10.6921906114133,19.4737858221446,4.78947242824774));
#90299=CARTESIAN_POINT('Ctrl Pts',(-10.6869922212927,19.4741130775286,4.79224946167871));
#90300=CARTESIAN_POINT('Ctrl Pts',(-10.6555926743018,19.4760942360078,4.80878041241338));
#90301=CARTESIAN_POINT('Ctrl Pts',(-10.6289977319239,19.4777907523757,4.82176757816664));
#90302=CARTESIAN_POINT('Ctrl Pts',(-10.4781876306072,19.4874393587972,4.88983076120671));
#90303=CARTESIAN_POINT('Ctrl Pts',(-10.3471619700783,19.495850140819,4.92820822716175));
#90304=CARTESIAN_POINT('Ctrl Pts',(-10.1650416887877,19.5065454620465,4.95496207001341));
#90305=CARTESIAN_POINT('Ctrl Pts',(-10.1170551277985,19.5092828107653,4.95960687560147));
#90306=CARTESIAN_POINT('Ctrl Pts',(-10.0593274835243,19.512478084001,4.96232854438822));
#90307=CARTESIAN_POINT('Ctrl Pts',(-10.0497279317456,19.5130062565214,4.96268645342303));
#90308=CARTESIAN_POINT('Ctrl Pts',(-10.0339210232831,19.51387087085,4.96312000098184));
#90309=CARTESIAN_POINT('Ctrl Pts',(-10.0277155739982,19.5142090097267,4.96325070364289));
#90310=CARTESIAN_POINT('Ctrl Pts',(-10.0165275235296,19.5148163776531,4.96341515488704));
#90311=CARTESIAN_POINT('Ctrl Pts',(-10.0115452504418,19.5150860379272,4.96346294200809));
#90312=CARTESIAN_POINT('Ctrl Pts',(-10.0008970811179,19.5156606557286,4.96351069217716));
#90313=CARTESIAN_POINT('Ctrl Pts',(-9.99523122172534,19.5159653776625,4.96350319810504));
#90314=CARTESIAN_POINT('Ctrl Pts',(-9.97987019197919,19.5167888067918,4.96339367378582));
#90315=CARTESIAN_POINT('Ctrl Pts',(-9.9701756660977,19.5173055435273,4.96322820121313));
#90316=CARTESIAN_POINT('Ctrl Pts',(-9.9196596332674,19.5199836623755,4.96186369627595));
#90317=CARTESIAN_POINT('Ctrl Pts',(-9.87889797126392,19.5220946326705,4.95905268307079));
#90318=CARTESIAN_POINT('Ctrl Pts',(-9.71378303553656,19.5305137133052,4.94069751926143));
#90319=CARTESIAN_POINT('Ctrl Pts',(-9.59156494624521,19.5363916492481,4.91092450988107));
#90320=CARTESIAN_POINT('Ctrl Pts',(-9.46399590928774,19.5432002307963,4.86185969258435));
#90321=CARTESIAN_POINT('Ctrl Pts',(-9.45340420836556,19.5437712795273,4.85764326680083));
#90322=CARTESIAN_POINT('Ctrl Pts',(-9.4089914721531,19.5461941632612,4.83935913776671));
#90323=CARTESIAN_POINT('Ctrl Pts',(-9.37565795690693,19.5480824121372,4.82414899976603));
#90324=CARTESIAN_POINT('Ctrl Pts',(-9.33761651227905,19.550358185318,4.80503477470672));
#90325=CARTESIAN_POINT('Ctrl Pts',(-9.33231667434938,19.5506780372347,4.80233122601178));
#90326=CARTESIAN_POINT('Ctrl Pts',(-9.32384050553403,19.5511943171159,4.79794203165456));
#90327=CARTESIAN_POINT('Ctrl Pts',(-9.32065359130019,19.5513895116015,4.79627683614106));
#90328=CARTESIAN_POINT('Ctrl Pts',(-9.31499648272897,19.5517379850783,4.79329434717067));
#90329=CARTESIAN_POINT('Ctrl Pts',(-9.31252389492118,19.5518909734596,4.79198169179796));
#90330=CARTESIAN_POINT('Ctrl Pts',(-9.30724730966148,19.5522189273376,4.78916100475393));
#90331=CARTESIAN_POINT('Ctrl Pts',(-9.30444450638144,19.5523940157872,4.78765093913189));
#90332=CARTESIAN_POINT('Ctrl Pts',(-9.29677816670136,19.5528753111136,4.78348821338989));
#90333=CARTESIAN_POINT('Ctrl Pts',(-9.29192478180408,19.5531826499434,4.78081709236763));
#90334=CARTESIAN_POINT('Ctrl Pts',(-9.26613317293796,19.5548295370464,4.76643096221526));
#90335=CARTESIAN_POINT('Ctrl Pts',(-9.24547137530858,19.5561969856439,4.75423056858856));
#90336=CARTESIAN_POINT('Ctrl Pts',(-9.18274248956905,19.5604770492784,4.71507935363373));
#90337=CARTESIAN_POINT('Ctrl Pts',(-9.14174932372667,19.5634566331956,4.68647918343862));
#90338=CARTESIAN_POINT('Ctrl Pts',(-9.00281137922814,19.5740262052301,4.57857127997811));
#90339=CARTESIAN_POINT('Ctrl Pts',(-8.913694079542,19.5816308322526,4.48876256262639));
#90340=CARTESIAN_POINT('Ctrl Pts',(-8.82508023407212,19.5898300087594,4.37280739379337));
#90341=CARTESIAN_POINT('Ctrl Pts',(-8.81330670353822,19.590937076438,4.35673115864341));
#90342=CARTESIAN_POINT('Ctrl Pts',(-8.79740260013003,19.5924584405785,4.33405762417671));
#90343=CARTESIAN_POINT('Ctrl Pts',(-8.79299119237502,19.5928833510243,4.32766078087798));
#90344=CARTESIAN_POINT('Ctrl Pts',(-8.7859818838541,19.5935633217146,4.31732157013319));
#90345=CARTESIAN_POINT('Ctrl Pts',(-8.78335178913591,19.5938195881298,4.31340129521907));
#90346=CARTESIAN_POINT('Ctrl Pts',(-8.77794177869087,19.5943490871375,4.30525248276169));
#90347=CARTESIAN_POINT('Ctrl Pts',(-8.77516473087381,19.5946222105868,4.30102211059117));
#90348=CARTESIAN_POINT('Ctrl Pts',(-8.76870427074262,19.5952607680451,4.29106851671943));
#90349=CARTESIAN_POINT('Ctrl Pts',(-8.76503871221338,19.5956255390292,4.28533380853693));
#90350=CARTESIAN_POINT('Ctrl Pts',(-8.7532103196746,19.5968109109581,4.26654085692686));
#90351=CARTESIAN_POINT('Ctrl Pts',(-8.74521341125689,19.597625456764,4.25337907639385));
#90352=CARTESIAN_POINT('Ctrl Pts',(-8.70448043466346,19.6018487188167,4.18388996682947));
#90353=CARTESIAN_POINT('Ctrl Pts',(-8.6753231438874,19.6051283561073,4.12554688264944));
#90354=CARTESIAN_POINT('Ctrl Pts',(-8.61451511102962,19.6128869849944,3.98038489203253));
#90355=CARTESIAN_POINT('Ctrl Pts',(-8.58700399490199,19.617274622955,3.89214672512127));
#90356=CARTESIAN_POINT('Ctrl Pts',(-8.56575899711584,19.6224075666015,3.79137753656668));
#90357=CARTESIAN_POINT('Ctrl Pts',(-8.56365467278365,19.6229469505714,3.78082061390514));
#90358=CARTESIAN_POINT('Ctrl Pts',(-8.55488996320356,19.6253411738116,3.73417135393701));
#90359=CARTESIAN_POINT('Ctrl Pts',(-8.54947265648821,19.6272329671384,3.69786168250997));
#90360=CARTESIAN_POINT('Ctrl Pts',(-8.54476954666823,19.6295127124965,3.65547350828073));
#90361=CARTESIAN_POINT('Ctrl Pts',(-8.54414922163953,19.6298327248091,3.64955331097293));
#90362=CARTESIAN_POINT('Ctrl Pts',(-8.54321206155058,19.6303492142427,3.64005030628945));
#90363=CARTESIAN_POINT('Ctrl Pts',(-8.54287228152534,19.6305444562879,3.63646976732252));
#90364=CARTESIAN_POINT('Ctrl Pts',(-8.5422915002884,19.6308929829265,3.6301000290468));
#90365=CARTESIAN_POINT('Ctrl Pts',(-8.54204529980753,19.6310459765809,3.62731134974793));
#90366=CARTESIAN_POINT('Ctrl Pts',(-8.54153625737361,19.6313739050152,3.62135029494992));
#90367=CARTESIAN_POINT('Ctrl Pts',(-8.54127576742497,19.6315489625135,3.61817781322907));
#90368=CARTESIAN_POINT('Ctrl Pts',(-8.54059049117699,19.6320300875497,3.60948423908685));
#90369=CARTESIAN_POINT('Ctrl Pts',(-8.54018669145509,19.6323372857366,3.60396160461855));
#90370=CARTESIAN_POINT('Ctrl Pts',(-8.53820280922318,19.6339820770236,3.57453324519177));
#90371=CARTESIAN_POINT('Ctrl Pts',(-8.53717867091092,19.6353474883183,3.55059500034907));
#90372=CARTESIAN_POINT('Ctrl Pts',(-8.53583524222462,19.639618535893,3.47681521411126));
#90373=CARTESIAN_POINT('Ctrl Pts',(-8.53747382767058,19.642590846011,3.42697553874008));
#90374=CARTESIAN_POINT('Ctrl Pts',(-8.55216402382087,19.6531194160634,3.25234704689363));
#90375=CARTESIAN_POINT('Ctrl Pts',(-8.57870044642372,19.6606919054296,3.12921815587786));
#90376=CARTESIAN_POINT('Ctrl Pts',(-8.62745632911001,19.6688958815603,2.99169449324787));
#90377=CARTESIAN_POINT('Ctrl Pts',(-8.63469464575175,19.6700329964928,2.97256093634037));
#90378=CARTESIAN_POINT('Ctrl Pts',(-8.64526378429456,19.671588346472,2.94629999243609));
#90379=CARTESIAN_POINT('Ctrl Pts',(-8.64825424920253,19.6720178284821,2.93903891303143));
#90380=CARTESIAN_POINT('Ctrl Pts',(-8.65314190456953,19.6727032078373,2.92743738037344));
#90381=CARTESIAN_POINT('Ctrl Pts',(-8.65500194937244,19.6729603474446,2.92308152468217));
#90382=CARTESIAN_POINT('Ctrl Pts',(-8.65888926558614,19.6734902370097,2.91409918844373));
#90383=CARTESIAN_POINT('Ctrl Pts',(-8.66091941059574,19.6737628855044,2.90947401504536));
#90384=CARTESIAN_POINT('Ctrl Pts',(-8.66571773557392,19.6743979113802,2.89869422989448));
#90385=CARTESIAN_POINT('Ctrl Pts',(-8.66850463347723,19.6747596475565,2.89254804195705));
#90386=CARTESIAN_POINT('Ctrl Pts',(-8.67765512759769,19.6759249468962,2.87273322402547));
#90387=CARTESIAN_POINT('Ctrl Pts',(-8.68418757119051,19.6767227413814,2.85914335120469));
#90388=CARTESIAN_POINT('Ctrl Pts',(-8.71890115548597,19.6807957758188,2.78969581140663));
#90389=CARTESIAN_POINT('Ctrl Pts',(-8.7504341805923,19.683952514362,2.73558343377593));
#90390=CARTESIAN_POINT('Ctrl Pts',(-8.83560972332474,19.6914952616717,2.60884892028306));
#90391=CARTESIAN_POINT('Ctrl Pts',(-8.89268249415985,19.6957880909552,2.5388537987157));
#90392=CARTESIAN_POINT('Ctrl Pts',(-8.99212286210712,19.7028272091799,2.43759752579814));
#90393=CARTESIAN_POINT('Ctrl Pts',(-9.03035017278664,19.7054532030893,2.40259692823344));
#90394=CARTESIAN_POINT('Ctrl Pts',(-9.07584518979355,19.7085970225304,2.36517807434153));
#90395=CARTESIAN_POINT('Ctrl Pts',(-9.0813754294384,19.7089794808208,2.36069678731107));
#90396=CARTESIAN_POINT('Ctrl Pts',(-9.08968648324077,19.7095550756271,2.35406199147379));
#90397=CARTESIAN_POINT('Ctrl Pts',(-9.09244281079923,19.7097461028654,2.35187780877597));
#90398=CARTESIAN_POINT('Ctrl Pts',(-9.0973972836655,19.7100897646473,2.34798075005767));
#90399=CARTESIAN_POINT('Ctrl Pts',(-9.0995924731048,19.710242136298,2.34626419787403));
#90400=CARTESIAN_POINT('Ctrl Pts',(-9.10438099917312,19.7105747542419,2.34254174847796));
#90401=CARTESIAN_POINT('Ctrl Pts',(-9.10697614331696,19.7107551628563,2.34053831903817));
#90402=CARTESIAN_POINT('Ctrl Pts',(-9.11431900084161,19.7112659798729,2.33490897095393));
#90403=CARTESIAN_POINT('Ctrl Pts',(-9.11908215842843,19.7115977561718,2.33130342170295));
#90404=CARTESIAN_POINT('Ctrl Pts',(-9.14876356574491,19.7136670950381,2.30912014208308));
#90405=CARTESIAN_POINT('Ctrl Pts',(-9.17424466770942,19.7154516879571,2.29131221813473));
#90406=CARTESIAN_POINT('Ctrl Pts',(-9.33457789607275,19.7266358461978,2.18669750910278));
#90407=CARTESIAN_POINT('Ctrl Pts',(-9.48238553957991,19.7365995753722,2.12172398753755));
#90408=CARTESIAN_POINT('Ctrl Pts',(-9.6629788467985,19.7471601878114,2.07559729912238));
#90409=CARTESIAN_POINT('Ctrl Pts',(-9.68830152301704,19.7486107833966,2.06984249380475));
#90410=CARTESIAN_POINT('Ctrl Pts',(-9.72223535808229,19.7505155864279,2.06307493148943));
#90411=CARTESIAN_POINT('Ctrl Pts',(-9.73072052486733,19.7509886690149,2.06146066526613));
#90412=CARTESIAN_POINT('Ctrl Pts',(-9.74456490866533,19.7517554262881,2.05895361863814));
#90413=CARTESIAN_POINT('Ctrl Pts',(-9.74991559927502,19.7520505272024,2.05801541175204));
#90414=CARTESIAN_POINT('Ctrl Pts',(-9.76023446564596,19.752617280279,2.05626523255056));
#90415=CARTESIAN_POINT('Ctrl Pts',(-9.76520184284659,19.752889060973,2.05544906061482));
#90416=CARTESIAN_POINT('Ctrl Pts',(-9.77672822323623,19.7535173202494,2.05361622792713));
#90417=CARTESIAN_POINT('Ctrl Pts',(-9.78329015722995,19.7538731994404,2.05261852007167));
#90418=CARTESIAN_POINT('Ctrl Pts',(-9.80417626518422,19.7550004063593,2.04958811980506));
#90419=CARTESIAN_POINT('Ctrl Pts',(-9.81852413989434,19.755766488904,2.04772313614655));
#90420=CARTESIAN_POINT('Ctrl Pts',(-9.89035499686071,19.7595635307535,2.03946750216789));
#90421=CARTESIAN_POINT('Ctrl Pts',(-9.94815623199775,19.7624940727064,2.03627517345835));
#90422=CARTESIAN_POINT('Ctrl Pts',(-10.1262541280899,19.7713268299521,2.03700527146272));
#90423=CARTESIAN_POINT('Ctrl Pts',(-10.2459761815924,19.7769596538143,2.05231754779553));
#90424=CARTESIAN_POINT('Ctrl Pts',(-10.3904950169908,19.7845676826105,2.08926157923564));
#90425=CARTESIAN_POINT('Ctrl Pts',(-10.4183041668185,19.7860725025643,2.09725602705258));
#90426=CARTESIAN_POINT('Ctrl Pts',(-10.4511554702649,19.7879187716305,2.10776368868606));
#90427=CARTESIAN_POINT('Ctrl Pts',(-10.4564449131565,19.7882181921252,2.10948885507311));
#90428=CARTESIAN_POINT('Ctrl Pts',(-10.4650628657661,19.7887097380655,2.11235409454352));
#90429=CARTESIAN_POINT('Ctrl Pts',(-10.4683973768328,19.7889008401202,2.11347610013684));
#90430=CARTESIAN_POINT('Ctrl Pts',(-10.4743658418246,19.7892445814191,2.11550837330259));
#90431=CARTESIAN_POINT('Ctrl Pts',(-10.4770012714212,19.789396957238,2.11641415041444));
#90432=CARTESIAN_POINT('Ctrl Pts',(-10.4827305618842,19.7897295192493,2.11840157925402));
#90433=CARTESIAN_POINT('Ctrl Pts',(-10.4858233404175,19.7899098673236,2.11948608371518));
#90434=CARTESIAN_POINT('Ctrl Pts',(-10.4945384575337,19.7904203452318,2.12257501380342));
#90435=CARTESIAN_POINT('Ctrl Pts',(-10.5001521463365,19.7907518401392,2.12460343660886));
#90436=CARTESIAN_POINT('Ctrl Pts',(-10.5344870476136,19.7927951232602,2.13724783812309));
#90437=CARTESIAN_POINT('Ctrl Pts',(-10.5628797707166,19.7945525210164,2.1487280238192));
#90438=CARTESIAN_POINT('Ctrl Pts',(-10.6610882482114,19.8008204992774,2.19206948588274));
#90439=CARTESIAN_POINT('Ctrl Pts',(-10.7287392971688,19.8054753552094,2.2285212655474));
#90440=CARTESIAN_POINT('Ctrl Pts',(-10.8645873012179,19.8151904104543,2.31613627882895));
#90441=CARTESIAN_POINT('Ctrl Pts',(-10.9318223407228,19.8202184239716,2.36829552523978));
#90442=CARTESIAN_POINT('Ctrl Pts',(-11.0125920698612,19.8264473289293,2.44306083109441));
#90443=CARTESIAN_POINT('Ctrl Pts',(-11.0305827273165,19.8278496410744,2.46059514210448));
#90444=CARTESIAN_POINT('Ctrl Pts',(-11.0540655613569,19.8297013682571,2.48469179009598));
#90445=CARTESIAN_POINT('Ctrl Pts',(-11.0599637430919,19.8301683602617,2.49085093450522));
#90446=CARTESIAN_POINT('Ctrl Pts',(-11.069514070692,19.8309277364672,2.5009999244755));
#90447=CARTESIAN_POINT('Ctrl Pts',(-11.0731984714005,19.8312214956212,2.50495902577625));
#90448=CARTESIAN_POINT('Ctrl Pts',(-11.0802756890719,19.831787360392,2.51264894088238));
#90449=CARTESIAN_POINT('Ctrl Pts',(-11.0836713308142,19.832059583447,2.51637704073608));
#90450=CARTESIAN_POINT('Ctrl Pts',(-11.0915302243543,19.8326913494294,2.52509547051751));
#90451=CARTESIAN_POINT('Ctrl Pts',(-11.0959786566836,19.8330502712902,2.53009904711472));
#90452=CARTESIAN_POINT('Ctrl Pts',(-11.1097075710606,19.8341622704137,2.545756331416));
#90453=CARTESIAN_POINT('Ctrl Pts',(-11.1188683708862,19.834910435979,2.55651419759801));
#90454=CARTESIAN_POINT('Ctrl Pts',(-11.1683195161835,19.8389866024002,2.6163198669558));
#90455=CARTESIAN_POINT('Ctrl Pts',(-11.2055438973363,19.8421909595547,2.66781842694425));
#90456=CARTESIAN_POINT('Ctrl Pts',(-11.2664674218612,19.8478496029484,2.76481327483067));
#90457=CARTESIAN_POINT('Ctrl Pts',(-11.2913443219007,19.8503251223025,2.80944280029376));
#90458=CARTESIAN_POINT('Ctrl Pts',(-11.3511495750143,19.8569277173582,2.93131679114062));
#90459=CARTESIAN_POINT('Ctrl Pts',(-11.3817860003093,19.861052370121,3.01043908276629));
#90460=CARTESIAN_POINT('Ctrl Pts',(-11.408564591399,19.8661158509983,3.10262587747066));
#90461=CARTESIAN_POINT('Ctrl Pts',(-11.4115960946363,19.8667189906883,3.11353285858365));
#90462=CARTESIAN_POINT('Ctrl Pts',(-11.4156228675866,19.8675647257246,3.12870056083994));
#90463=CARTESIAN_POINT('Ctrl Pts',(-11.4167260951719,19.8678014440579,3.13293250345685));
#90464=CARTESIAN_POINT('Ctrl Pts',(-11.4184635892592,19.868182513626,3.13972199746729));
#90465=CARTESIAN_POINT('Ctrl Pts',(-11.4191099545004,19.8683261786957,3.14227646153254));
#90466=CARTESIAN_POINT('Ctrl Pts',(-11.420445710445,19.8686271163107,3.14761602510535));
#90467=CARTESIAN_POINT('Ctrl Pts',(-11.4211338110559,19.8687844639743,3.15040141206348));
#90468=CARTESIAN_POINT('Ctrl Pts',(-11.4227836461558,19.8691674054795,3.15716520154111));
#90469=CARTESIAN_POINT('Ctrl Pts',(-11.4237368868074,19.8693934771686,3.16114563730735));
#90470=CARTESIAN_POINT('Ctrl Pts',(-11.4257351832887,19.8698777726327,3.16964720387249));
#90471=CARTESIAN_POINT('Ctrl Pts',(-11.4267754564191,19.8701362499985,3.17416940202215));
#90472=CARTESIAN_POINT('Ctrl Pts',(-11.4317038490203,19.871391970386,3.1960699675285));
#90473=CARTESIAN_POINT('Ctrl Pts',(-11.4352959031073,19.8724040590828,3.21351267192146));
#90474=CARTESIAN_POINT('Ctrl Pts',(-11.4550740134502,19.8785960252534,3.31928901210277));
#90475=CARTESIAN_POINT('Ctrl Pts',(-11.4634181561964,19.8840564920709,3.40888654081214));
#90476=CARTESIAN_POINT('Ctrl Pts',(-11.4634994008935,19.8894511611806,3.49867577028773));
#90477=CARTESIAN_POINT('Ctrl Pts',(-11.4634994011565,19.8894511786466,3.49867606099216));
#90478=CARTESIAN_POINT('Ctrl Pts',(-11.4634998003887,19.889477693589,3.49911737745962));
#90479=CARTESIAN_POINT('Ctrl Pts',(-11.4635,19.8895042068034,3.49955869048854));
#90480=CARTESIAN_POINT('Ctrl Pts',(-11.4635,19.889530718258,3.4999999999448));
#90481=CARTESIAN_POINT('Origin',(-10.,13.2,3.5));
#90482=CARTESIAN_POINT('',(-11.4635,20.459317028952,3.50000000000019));
#90483=CARTESIAN_POINT('',(-11.4635,20.390600218991,3.49999999999975));
#90484=CARTESIAN_POINT('',(-11.4635,13.2,3.5));
#90485=CARTESIAN_POINT('Ctrl Pts',(-11.4635,20.459317028952,3.5000000000001));
#90486=CARTESIAN_POINT('Ctrl Pts',(-11.4635,20.4585861607261,3.48684366450097));
#90487=CARTESIAN_POINT('Ctrl Pts',(-11.4633225942004,20.457860760563,3.47368763253133));
#90488=CARTESIAN_POINT('Ctrl Pts',(-11.4627948065494,20.4567898065315,3.45412231023958));
#90489=CARTESIAN_POINT('Ctrl Pts',(-11.4625796377616,20.4564400819949,3.44771029236232));
#90490=CARTESIAN_POINT('Ctrl Pts',(-11.4621216643936,20.4558199937918,3.43630138831388));
#90491=CARTESIAN_POINT('Ctrl Pts',(-11.4618953899615,20.4555491216085,3.43130397179102));
#90492=CARTESIAN_POINT('Ctrl Pts',(-11.4613647468365,20.4549801729395,3.42077896701188));
#90493=CARTESIAN_POINT('Ctrl Pts',(-11.4610546289448,20.4546822793544,3.41525173889905));
#90494=CARTESIAN_POINT('Ctrl Pts',(-11.4601510936625,20.4538966131438,3.40063168220289));
#90495=CARTESIAN_POINT('Ctrl Pts',(-11.4595040997807,20.4534105090671,3.39154232769414));
#90496=CARTESIAN_POINT('Ctrl Pts',(-11.4560719320678,20.4511428547768,3.34894637463714));
#90497=CARTESIAN_POINT('Ctrl Pts',(-11.4522174412442,20.4493946878353,3.31553482727249));
#90498=CARTESIAN_POINT('Ctrl Pts',(-11.438138932602,20.4445582981249,3.22195134093262));
#90499=CARTESIAN_POINT('Ctrl Pts',(-11.4252983366242,20.4415455503876,3.16224261081665));
#90500=CARTESIAN_POINT('Ctrl Pts',(-11.3822214179042,20.433783059304,3.00918732932115));
#90501=CARTESIAN_POINT('Ctrl Pts',(-11.3462729364702,20.4291146075255,2.91778108706047));
#90502=CARTESIAN_POINT('Ctrl Pts',(-11.2905274834118,20.4228469200063,2.80938922834438));
#90503=CARTESIAN_POINT('Ctrl Pts',(-11.2790682285419,20.4215950503575,2.78839002263734));
#90504=CARTESIAN_POINT('Ctrl Pts',(-11.2642284884675,20.42000559209,2.76271341011662));
#90505=CARTESIAN_POINT('Ctrl Pts',(-11.2613275828113,20.4196962904609,2.75776155224647));
#90506=CARTESIAN_POINT('Ctrl Pts',(-11.2567326861606,20.4192083558283,2.75002277285764));
#90507=CARTESIAN_POINT('Ctrl Pts',(-11.2550583449591,20.4190309611882,2.74722417943978));
#90508=CARTESIAN_POINT('Ctrl Pts',(-11.2519356941978,20.4187008217362,2.74204417256937));
#90509=CARTESIAN_POINT('Ctrl Pts',(-11.2504899281503,20.4185482405374,2.73966128735058));
#90510=CARTESIAN_POINT('Ctrl Pts',(-11.2471940631138,20.418201024319,2.73426393011264));
#90511=CARTESIAN_POINT('Ctrl Pts',(-11.2453398462278,20.4180061249949,2.73125203958135));
#90512=CARTESIAN_POINT('Ctrl Pts',(-11.2396661928984,20.4174111640023,2.72211045666386));
#90513=CARTESIAN_POINT('Ctrl Pts',(-11.2358123425125,20.4170089488611,2.71600238446182));
#90514=CARTESIAN_POINT('Ctrl Pts',(-11.1836711101133,20.4115950902546,2.63470207207895));
#90515=CARTESIAN_POINT('Ctrl Pts',(-11.1286450767361,20.4062093218945,2.56406460363401));
#90516=CARTESIAN_POINT('Ctrl Pts',(-10.9909043473901,20.3940826678966,2.41718499056907));
#90517=CARTESIAN_POINT('Ctrl Pts',(-10.9051396337102,20.3874055017354,2.34453036920985));
#90518=CARTESIAN_POINT('Ctrl Pts',(-10.7979156082569,20.3801990584344,2.27303384144496));
#90519=CARTESIAN_POINT('Ctrl Pts',(-10.7837583681777,20.3792671828579,2.2639425071447));
#90520=CARTESIAN_POINT('Ctrl Pts',(-10.7638920337555,20.3779860184665,2.25166356376414));
#90521=CARTESIAN_POINT('Ctrl Pts',(-10.7583139976357,20.3776291379109,2.24826728883624));
#90522=CARTESIAN_POINT('Ctrl Pts',(-10.7486585644598,20.3770162174819,2.24247665681609));
#90523=CARTESIAN_POINT('Ctrl Pts',(-10.7445919847818,20.3767595362859,2.24006453271567));
#90524=CARTESIAN_POINT('Ctrl Pts',(-10.7361552218653,20.3762300004168,2.23511531218163));
#90525=CARTESIAN_POINT('Ctrl Pts',(-10.7317834402164,20.3759572503516,2.23258105518874));
#90526=CARTESIAN_POINT('Ctrl Pts',(-10.721524047013,20.3753209769279,2.22670461715346));
#90527=CARTESIAN_POINT('Ctrl Pts',(-10.7156261688355,20.3749581033805,2.22338053008284));
#90528=CARTESIAN_POINT('Ctrl Pts',(-10.6964076928092,20.3737848954022,2.2127238940706));
#90529=CARTESIAN_POINT('Ctrl Pts',(-10.6829956023699,20.3729804432523,2.20555785084485));
#90530=CARTESIAN_POINT('Ctrl Pts',(-10.6129199208088,20.3688472271292,2.16950904821246));
#90531=CARTESIAN_POINT('Ctrl Pts',(-10.5545268275638,20.3656411487338,2.14413194679851));
#90532=CARTESIAN_POINT('Ctrl Pts',(-10.40210321424,20.3576476321263,2.08939108164212));
#90533=CARTESIAN_POINT('Ctrl Pts',(-10.3064346172044,20.3529829476257,2.06556611554445));
#90534=CARTESIAN_POINT('Ctrl Pts',(-10.1996502540447,20.3475813911027,2.05015060114662));
#90535=CARTESIAN_POINT('Ctrl Pts',(-10.190182601987,20.3471006733265,2.04887833867582));
#90536=CARTESIAN_POINT('Ctrl Pts',(-10.1470890727483,20.3449018132879,2.04351640419182));
#90537=CARTESIAN_POINT('Ctrl Pts',(-10.1133421801772,20.3431501199156,2.04050252794203));
#90538=CARTESIAN_POINT('Ctrl Pts',(-10.0737069406151,20.3410273455869,2.03834563840073));
#90539=CARTESIAN_POINT('Ctrl Pts',(-10.0678883553571,20.3407140648319,2.03806383353461));
#90540=CARTESIAN_POINT('Ctrl Pts',(-10.0584748490325,20.3402043410197,2.03766423880226));
#90541=CARTESIAN_POINT('Ctrl Pts',(-10.0548808469425,20.340009052094,2.03752494772663));
#90542=CARTESIAN_POINT('Ctrl Pts',(-10.0484957827406,20.3396608388582,2.03730105414115));
#90543=CARTESIAN_POINT('Ctrl Pts',(-10.0457049527783,20.3395082079309,2.0372111894317));
#90544=CARTESIAN_POINT('Ctrl Pts',(-10.0396958335017,20.3391786240388,2.03703490976044));
#90545=CARTESIAN_POINT('Ctrl Pts',(-10.0364775593377,20.3390015327322,2.0369511280516));
#90546=CARTESIAN_POINT('Ctrl Pts',(-10.0275552941409,20.3385090174946,2.03674831091788));
#90547=CARTESIAN_POINT('Ctrl Pts',(-10.0218509073033,20.3381923737394,2.03665201148477));
#90548=CARTESIAN_POINT('Ctrl Pts',(-9.98969365549149,20.3363980144065,2.03629721200639));
#90549=CARTESIAN_POINT('Ctrl Pts',(-9.96323970265074,20.334886298025,2.03672266032551));
#90550=CARTESIAN_POINT('Ctrl Pts',(-9.87810227136302,20.3299369259874,2.04040188642371));
#90551=CARTESIAN_POINT('Ctrl Pts',(-9.81960017659495,20.3264088661178,2.04647296012052));
#90552=CARTESIAN_POINT('Ctrl Pts',(-9.6438861012254,20.3156861790243,2.07548063515102));
#90553=CARTESIAN_POINT('Ctrl Pts',(-9.52894419341959,20.3085432518702,2.10924889192518));
#90554=CARTESIAN_POINT('Ctrl Pts',(-9.40434830473908,20.3009587714688,2.16310096173804));
#90555=CARTESIAN_POINT('Ctrl Pts',(-9.38943821841819,20.3000528708883,2.16984424897268));
#90556=CARTESIAN_POINT('Ctrl Pts',(-9.36880853794113,20.2988014639674,2.17959428735803));
#90557=CARTESIAN_POINT('Ctrl Pts',(-9.36299140740488,20.29844881634,2.18239081568749));
#90558=CARTESIAN_POINT('Ctrl Pts',(-9.35296298884173,20.2978412077954,2.18729381612792));
#90559=CARTESIAN_POINT('Ctrl Pts',(-9.34874304742762,20.2975856310286,2.18938228249713));
#90560=CARTESIAN_POINT('Ctrl Pts',(-9.34000415353803,20.2970565573425,2.19375982596258));
#90561=CARTESIAN_POINT('Ctrl Pts',(-9.33548685441311,20.2967831749257,2.19605207548404));
#90562=CARTESIAN_POINT('Ctrl Pts',(-9.32489338302851,20.2961422748894,2.20149695307174));
#90563=CARTESIAN_POINT('Ctrl Pts',(-9.31882721871617,20.2957754356686,2.20466886420272));
#90564=CARTESIAN_POINT('Ctrl Pts',(-9.29898410424006,20.2945758233606,2.21522248989186));
#90565=CARTESIAN_POINT('Ctrl Pts',(-9.28530287418127,20.2937493147883,2.22278248535166));
#90566=CARTESIAN_POINT('Ctrl Pts',(-9.21358644135855,20.2894159200497,2.26392493071262));
#90567=CARTESIAN_POINT('Ctrl Pts',(-9.15778651145136,20.2860462143296,2.30124830370249));
#90568=CARTESIAN_POINT('Ctrl Pts',(-9.02608012585929,20.2778500202053,2.4030956614309));
#90569=CARTESIAN_POINT('Ctrl Pts',(-8.9538313725829,20.273135691026,2.47177433908668));
#90570=CARTESIAN_POINT('Ctrl Pts',(-8.86439788531536,20.2662175017211,2.57605160217889));
#90571=CARTESIAN_POINT('Ctrl Pts',(-8.8408209205691,20.2642638759563,2.60580974911267));
#90572=CARTESIAN_POINT('Ctrl Pts',(-8.81488697556333,20.2619148859655,2.64129434408914));
#90573=CARTESIAN_POINT('Ctrl Pts',(-8.81137485014706,20.2615922180586,2.64616246577292));
#90574=CARTESIAN_POINT('Ctrl Pts',(-8.80579830310663,20.2610722943105,2.65399314736641));
#90575=CARTESIAN_POINT('Ctrl Pts',(-8.80371468763766,20.260876300372,2.65694203139851));
#90576=CARTESIAN_POINT('Ctrl Pts',(-8.80003445426928,20.2605269763263,2.66219167959683));
#90577=CARTESIAN_POINT('Ctrl Pts',(-8.79843350266798,20.2603739426225,2.66448935071331));
#90578=CARTESIAN_POINT('Ctrl Pts',(-8.79503284550171,20.2600465593963,2.66939993233331));
#90579=CARTESIAN_POINT('Ctrl Pts',(-8.79323506723848,20.2598720912459,2.67201406262575));
#90580=CARTESIAN_POINT('Ctrl Pts',(-8.78834803912353,20.2593940409363,2.67916996460683));
#90581=CARTESIAN_POINT('Ctrl Pts',(-8.78527586851363,20.2590893510475,2.68372326768473));
#90582=CARTESIAN_POINT('Ctrl Pts',(-8.76927150352025,20.2574804591513,2.70773397682981));
#90583=CARTESIAN_POINT('Ctrl Pts',(-8.7567816584149,20.2561498219653,2.72748067258661));
#90584=CARTESIAN_POINT('Ctrl Pts',(-8.72015780539824,20.2520306381704,2.78857350248166));
#90585=CARTESIAN_POINT('Ctrl Pts',(-8.6975756914836,20.2491802905592,2.83081088587004));
#90586=CARTESIAN_POINT('Ctrl Pts',(-8.63407573749567,20.2402673835883,2.96501845979466));
#90587=CARTESIAN_POINT('Ctrl Pts',(-8.60053390658912,20.2341704435879,3.06016707201283));
#90588=CARTESIAN_POINT('Ctrl Pts',(-8.56696162203014,20.2258660540496,3.19985729705873));
#90589=CARTESIAN_POINT('Ctrl Pts',(-8.55875445129622,20.2234295009587,3.2421309587808));
#90590=CARTESIAN_POINT('Ctrl Pts',(-8.55092430309774,20.220488760785,3.29477928035595));
#90591=CARTESIAN_POINT('Ctrl Pts',(-8.54953159768786,20.2199295246279,3.30486584004043));
#90592=CARTESIAN_POINT('Ctrl Pts',(-8.5475068873743,20.2190551502944,3.32075151269132));
#90593=CARTESIAN_POINT('Ctrl Pts',(-8.54680411210141,20.2187378088219,3.32654114263757));
#90594=CARTESIAN_POINT('Ctrl Pts',(-8.54562367785358,20.2181790684193,3.33677696801069));
#90595=CARTESIAN_POINT('Ctrl Pts',(-8.5451317563247,20.21793722717,3.34122141595275));
#90596=CARTESIAN_POINT('Ctrl Pts',(-8.54405002705769,20.2173838976553,3.35142205156006));
#90597=CARTESIAN_POINT('Ctrl Pts',(-8.54347396949103,20.2170728417907,3.35717964346401));
#90598=CARTESIAN_POINT('Ctrl Pts',(-8.54197193984876,20.2162135830915,3.37314760006469));
#90599=CARTESIAN_POINT('Ctrl Pts',(-8.54111907612931,20.2156676589603,3.38336461650375));
#90600=CARTESIAN_POINT('Ctrl Pts',(-8.5367643629416,20.2124973751532,3.44309819412834));
#90601=CARTESIAN_POINT('Ctrl Pts',(-8.53567605865511,20.2099491778866,3.49276067483508));
#90602=CARTESIAN_POINT('Ctrl Pts',(-8.54056124353831,20.201479750471,3.66136423339364));
#90603=CARTESIAN_POINT('Ctrl Pts',(-8.55850935500589,20.1958884282564,3.77946747108423));
#90604=CARTESIAN_POINT('Ctrl Pts',(-8.5927282984786,20.1895349614457,3.90185017331306));
#90605=CARTESIAN_POINT('Ctrl Pts',(-8.59496256707478,20.1891303024943,3.90959371669516));
#90606=CARTESIAN_POINT('Ctrl Pts',(-8.60764490262973,20.1868860310935,3.9522230724931));
#90607=CARTESIAN_POINT('Ctrl Pts',(-8.61932756751662,20.1850082975208,3.98672543146744));
#90608=CARTESIAN_POINT('Ctrl Pts',(-8.63439694046938,20.182744377329,4.02630391238361));
#90609=CARTESIAN_POINT('Ctrl Pts',(-8.63654401192042,20.1824250754662,4.03184141486891));
#90610=CARTESIAN_POINT('Ctrl Pts',(-8.64004362442416,20.1819095483078,4.04070676851005));
#90611=CARTESIAN_POINT('Ctrl Pts',(-8.64137483797195,20.1817145512693,4.0440430327879));
#90612=CARTESIAN_POINT('Ctrl Pts',(-8.64376489016373,20.1813663436337,4.04996945997589));
#90613=CARTESIAN_POINT('Ctrl Pts',(-8.64481888990078,20.1812134225456,4.0525615248878));
#90614=CARTESIAN_POINT('Ctrl Pts',(-8.64708815847951,20.1808855154591,4.05809670980613));
#90615=CARTESIAN_POINT('Ctrl Pts',(-8.64830558101838,20.1807104059678,4.06103884510556));
#90616=CARTESIAN_POINT('Ctrl Pts',(-8.65166925793434,20.1802288291927,4.06909331619036));
#90617=CARTESIAN_POINT('Ctrl Pts',(-8.65383495637173,20.1799212272831,4.07419741015248));
#90618=CARTESIAN_POINT('Ctrl Pts',(-8.66555934888172,20.178269422689,4.10139840502714));
#90619=CARTESIAN_POINT('Ctrl Pts',(-8.67563270323871,20.176897121994,4.12326801426323));
#90620=CARTESIAN_POINT('Ctrl Pts',(-8.70837821347617,20.1725951849505,4.18997791047985));
#90621=CARTESIAN_POINT('Ctrl Pts',(-8.73282264425357,20.1695978494516,4.23390551272138));
#90622=CARTESIAN_POINT('Ctrl Pts',(-8.82701899972409,20.1589299200293,4.38439481185877));
#90623=CARTESIAN_POINT('Ctrl Pts',(-8.90836851306369,20.1512486618383,4.48305168894253));
#90624=CARTESIAN_POINT('Ctrl Pts',(-9.01512649082637,20.1430598075018,4.58268430628366));
#90625=CARTESIAN_POINT('Ctrl Pts',(-9.02902516341687,20.1420232106957,4.59516621946138));
#90626=CARTESIAN_POINT('Ctrl Pts',(-9.0488836785362,20.1405822959859,4.61232514292157));
#90627=CARTESIAN_POINT('Ctrl Pts',(-9.05464625160571,20.1401687770694,4.61722682295983));
#90628=CARTESIAN_POINT('Ctrl Pts',(-9.06403595145289,20.1395023146433,4.62508909225015));
#90629=CARTESIAN_POINT('Ctrl Pts',(-9.06763968120551,20.1392482529777,4.62807730334386));
#90630=CARTESIAN_POINT('Ctrl Pts',(-9.07518761168055,20.138719682142,4.63427516671551));
#90631=CARTESIAN_POINT('Ctrl Pts',(-9.0791343320648,20.1384453018159,4.6374816613624));
#90632=CARTESIAN_POINT('Ctrl Pts',(-9.08852124092305,20.1377973932307,4.64502713607102));
#90633=CARTESIAN_POINT('Ctrl Pts',(-9.0939758484807,20.1374245867772,4.64934803681316));
#90634=CARTESIAN_POINT('Ctrl Pts',(-9.11229675865478,20.1361844614468,4.66364958310356));
#90635=CARTESIAN_POINT('Ctrl Pts',(-9.12529903177867,20.1353240185402,4.67345457564422));
#90636=CARTESIAN_POINT('Ctrl Pts',(-9.19713585962409,20.1306713734026,4.72576901378889));
#90637=CARTESIAN_POINT('Ctrl Pts',(-9.25890914353523,20.1270414561978,4.76407532114117));
#90638=CARTESIAN_POINT('Ctrl Pts',(-9.41089829175372,20.1186337239025,4.84333808502662));
#90639=CARTESIAN_POINT('Ctrl Pts',(-9.50291668369698,20.1139425395583,4.88003750392223));
#90640=CARTESIAN_POINT('Ctrl Pts',(-9.62922331045825,20.1072785057017,4.91612732635012));
#90641=CARTESIAN_POINT('Ctrl Pts',(-9.66081129649352,20.105592463459,4.9240234115604));
#90642=CARTESIAN_POINT('Ctrl Pts',(-9.69825775149512,20.1035436591159,4.93206737039526));
#90643=CARTESIAN_POINT('Ctrl Pts',(-9.70388864685603,20.1032342557305,4.93324226920779));
#90644=CARTESIAN_POINT('Ctrl Pts',(-9.71302981526673,20.1027296215998,4.93509342608285));
#90645=CARTESIAN_POINT('Ctrl Pts',(-9.71653595140138,20.1025355077801,4.93579008253647));
#90646=CARTESIAN_POINT('Ctrl Pts',(-9.7227833465373,20.1021885762415,4.93700764189391));
#90647=CARTESIAN_POINT('Ctrl Pts',(-9.7255235791595,20.102036043593,4.93753355789755));
#90648=CARTESIAN_POINT('Ctrl Pts',(-9.73144336653739,20.1017057291804,4.938652162645));
#90649=CARTESIAN_POINT('Ctrl Pts',(-9.73462334065085,20.101527802894,4.93924214040401));
#90650=CARTESIAN_POINT('Ctrl Pts',(-9.74348510040362,20.101030658394,4.94085588704509));
#90651=CARTESIAN_POINT('Ctrl Pts',(-9.74917096292433,20.1007101834854,4.94185657151965));
#90652=CARTESIAN_POINT('Ctrl Pts',(-9.78201888808637,20.0988507152992,4.94743747443672));
#90653=CARTESIAN_POINT('Ctrl Pts',(-9.80929839007174,20.0972748311089,4.95128346721581));
#90654=CARTESIAN_POINT('Ctrl Pts',(-9.89931083282583,20.0920064859197,4.96139232572001));
#90655=CARTESIAN_POINT('Ctrl Pts',(-9.96233935506856,20.0882114704415,4.96437246090669));
#90656=CARTESIAN_POINT('Ctrl Pts',(-10.1386103983788,20.0775941531258,4.96131753616541));
#90657=CARTESIAN_POINT('Ctrl Pts',(-10.2512695827667,20.0708375309667,4.94621357288375));
#90658=CARTESIAN_POINT('Ctrl Pts',(-10.3773087313069,20.063565625763,4.91412556522857));
#90659=CARTESIAN_POINT('Ctrl Pts',(-10.3934744215156,20.0626375772524,4.90971305781014));
#90660=CARTESIAN_POINT('Ctrl Pts',(-10.4158202280936,20.0613607852006,4.90319930561471));
#90661=CARTESIAN_POINT('Ctrl Pts',(-10.4220670027975,20.0610045171669,4.90133300840579));
#90662=CARTESIAN_POINT('Ctrl Pts',(-10.4328195102951,20.0603923662041,4.89804214858246));
#90663=CARTESIAN_POINT('Ctrl Pts',(-10.437331163193,20.0601358456546,4.89663740181011));
#90664=CARTESIAN_POINT('Ctrl Pts',(-10.4466549548152,20.0596063815475,4.89368473940844));
#90665=CARTESIAN_POINT('Ctrl Pts',(-10.4514660409754,20.0593335440106,4.89213369194642));
#90666=CARTESIAN_POINT('Ctrl Pts',(-10.4627116529755,20.058696620408,4.88844378794382));
#90667=CARTESIAN_POINT('Ctrl Pts',(-10.4691395721417,20.0583331881689,4.88628506809995));
#90668=CARTESIAN_POINT('Ctrl Pts',(-10.4895091464893,20.0571833440202,4.87928634947637));
#90669=CARTESIAN_POINT('Ctrl Pts',(-10.5033929463999,20.0564023830972,4.87428002997463));
#90670=CARTESIAN_POINT('Ctrl Pts',(-10.5359550749984,20.0545758419502,4.86197885583329));
#90671=CARTESIAN_POINT('Ctrl Pts',(-10.5545640838046,20.0535359986684,4.8545083872159));
#90672=CARTESIAN_POINT('Ctrl Pts',(-10.6209758989012,20.0498321984615,4.82624959486688));
#90673=CARTESIAN_POINT('Ctrl Pts',(-10.6678152016703,20.0472351762392,4.80329293425981));
#90674=CARTESIAN_POINT('Ctrl Pts',(-10.78354775598,20.0407257828274,4.73868949579091));
#90675=CARTESIAN_POINT('Ctrl Pts',(-10.8504108399234,20.0368799263507,4.69377529215694));
#90676=CARTESIAN_POINT('Ctrl Pts',(-10.9539521411974,20.0303095640824,4.61109020932959));
#90677=CARTESIAN_POINT('Ctrl Pts',(-10.9928912584495,20.027669381724,4.5764348661828));
#90678=CARTESIAN_POINT('Ctrl Pts',(-11.0349584116525,20.0245094367286,4.53476765629012));
#90679=CARTESIAN_POINT('Ctrl Pts',(-11.0399838036904,20.0241266062625,4.52971680587639));
#90680=CARTESIAN_POINT('Ctrl Pts',(-11.0474347170704,20.0235505979442,4.52211796604934));
#90681=CARTESIAN_POINT('Ctrl Pts',(-11.0498883331428,20.0233595345351,4.51959752375482));
#90682=CARTESIAN_POINT('Ctrl Pts',(-11.0542688719603,20.0230158831839,4.51506509973609));
#90683=CARTESIAN_POINT('Ctrl Pts',(-11.056199158364,20.0228635586798,4.51305643909112));
#90684=CARTESIAN_POINT('Ctrl Pts',(-11.0603868069784,20.0225311359013,4.50867378312491));
#90685=CARTESIAN_POINT('Ctrl Pts',(-11.062641907428,20.0223508760369,4.50629774784673));
#90686=CARTESIAN_POINT('Ctrl Pts',(-11.0672777317011,20.0219777739256,4.50138035720402));
#90687=CARTESIAN_POINT('Ctrl Pts',(-11.069657398808,20.02178485598,4.49883803744669));
#90688=CARTESIAN_POINT('Ctrl Pts',(-11.081242878703,20.0208388876541,4.48637179552282));
#90689=CARTESIAN_POINT('Ctrl Pts',(-11.0903194693153,20.020076852143,4.4763293038851));
#90690=CARTESIAN_POINT('Ctrl Pts',(-11.136606263325,20.0160875150725,4.42366633833537));
#90691=CARTESIAN_POINT('Ctrl Pts',(-11.1714587202384,20.0127314832471,4.37904306255321));
#90692=CARTESIAN_POINT('Ctrl Pts',(-11.232974669029,20.0062460173592,4.29010463783038));
#90693=CARTESIAN_POINT('Ctrl Pts',(-11.2600493420596,20.0031271227852,4.24616862571327));
#90694=CARTESIAN_POINT('Ctrl Pts',(-11.2866954006238,19.9997960348885,4.19732612616028));
#90695=CARTESIAN_POINT('Ctrl Pts',(-11.2886276758864,19.9995528138799,4.19374886908338));
#90696=CARTESIAN_POINT('Ctrl Pts',(-11.3320445888902,19.9940502250727,4.1125630727733));
#90697=CARTESIAN_POINT('Ctrl Pts',(-11.3664655914831,19.9889209772329,4.03136838411564));
#90698=CARTESIAN_POINT('Ctrl Pts',(-11.3966664999606,19.9834476899926,3.93734435758537));
#90699=CARTESIAN_POINT('Ctrl Pts',(-11.3998357262746,19.9828566074109,3.92709173171027));
#90700=CARTESIAN_POINT('Ctrl Pts',(-11.4047360157333,19.9819147347835,3.91059822267615));
#90701=CARTESIAN_POINT('Ctrl Pts',(-11.4065388782858,19.9815616327746,3.90437922810142));
#90702=CARTESIAN_POINT('Ctrl Pts',(-11.4096674852493,19.9809368708083,3.89331295607356));
#90703=CARTESIAN_POINT('Ctrl Pts',(-11.4110096396259,19.9806646852084,3.88847045980617));
#90704=CARTESIAN_POINT('Ctrl Pts',(-11.4137559568959,19.980098856048,3.87835970849104));
#90705=CARTESIAN_POINT('Ctrl Pts',(-11.4151556766407,19.9798053589016,3.87309031968845));
#90706=CARTESIAN_POINT('Ctrl Pts',(-11.4187206257387,19.9790442130742,3.85936095086765));
#90707=CARTESIAN_POINT('Ctrl Pts',(-11.4208396576202,19.9785780473065,3.85088912592739));
#90708=CARTESIAN_POINT('Ctrl Pts',(-11.4252784582874,19.9775703981376,3.83244310763236));
#90709=CARTESIAN_POINT('Ctrl Pts',(-11.4275696356019,19.9770298293959,3.82246247210452));
#90710=CARTESIAN_POINT('Ctrl Pts',(-11.4521868986626,19.970978501996,3.7098181246165));
#90711=CARTESIAN_POINT('Ctrl Pts',(-11.4634999999946,19.9658450492175,3.60506528518567));
#90712=CARTESIAN_POINT('Ctrl Pts',(-11.4635,19.9607369088795,3.50000000007519));
#90713=CARTESIAN_POINT('Ctrl Pts',(-11.4635,19.889530718258,3.4999999999448));
#90714=CARTESIAN_POINT('Ctrl Pts',(-11.4635000000029,19.894098071368,3.57602812264237));
#90715=CARTESIAN_POINT('Ctrl Pts',(-11.4575756192878,19.8986041100056,3.65195075480961));
#90716=CARTESIAN_POINT('Ctrl Pts',(-11.4415950904616,19.9044771054825,3.75369629780065));
#90717=CARTESIAN_POINT('Ctrl Pts',(-11.4366800211121,19.905992131755,3.78019433863034));
#90718=CARTESIAN_POINT('Ctrl Pts',(-11.4293252597365,19.9079367146872,3.81452861641016));
#90719=CARTESIAN_POINT('Ctrl Pts',(-11.4275477866545,19.908386892226,3.82250002989647));
#90720=CARTESIAN_POINT('Ctrl Pts',(-11.424440649886,19.9091418242089,3.83590530237781));
#90721=CARTESIAN_POINT('Ctrl Pts',(-11.4231464049553,19.9094476949911,3.84134710851949));
#90722=CARTESIAN_POINT('Ctrl Pts',(-11.4205283073341,19.9100499139078,3.85208143847751));
#90723=CARTESIAN_POINT('Ctrl Pts',(-11.4192059975401,19.910346305761,3.85737424211584));
#90724=CARTESIAN_POINT('Ctrl Pts',(-11.4166085922903,19.9109139535609,3.86752905926711));
#90725=CARTESIAN_POINT('Ctrl Pts',(-11.4153379857553,19.9111853485035,3.87239213217479));
#90726=CARTESIAN_POINT('Ctrl Pts',(-11.4123735237005,19.9118044773777,3.88350383624424));
#90727=CARTESIAN_POINT('Ctrl Pts',(-11.4106632012984,19.9121516775848,3.88974799191676));
#90728=CARTESIAN_POINT('Ctrl Pts',(-11.4060099170788,19.9130704975451,3.90630452154103));
#90729=CARTESIAN_POINT('Ctrl Pts',(-11.4029949176656,19.9136397978806,3.91659635172702));
#90730=CARTESIAN_POINT('Ctrl Pts',(-11.374848167005,19.9187311807119,4.00890351104174));
#90731=CARTESIAN_POINT('Ctrl Pts',(-11.3426634352935,19.923008432776,4.08859800525403));
#90732=CARTESIAN_POINT('Ctrl Pts',(-11.2813697121994,19.929604024528,4.20875538506209));
#90733=CARTESIAN_POINT('Ctrl Pts',(-11.2568745027884,19.9319766159394,4.25133813497436));
#90734=CARTESIAN_POINT('Ctrl Pts',(-11.2043916657069,19.9367111976816,4.33280185036871));
#90735=CARTESIAN_POINT('Ctrl Pts',(-11.1765449435219,19.9390692419126,4.37169930642364));
#90736=CARTESIAN_POINT('Ctrl Pts',(-11.1289817042751,19.9429781042925,4.43169713660158));
#90737=CARTESIAN_POINT('Ctrl Pts',(-11.1104576700371,19.9444754915997,4.45369952685649));
#90738=CARTESIAN_POINT('Ctrl Pts',(-11.0873876803285,19.946330771025,4.47951760536667));
#90739=CARTESIAN_POINT('Ctrl Pts',(-11.0834502446072,19.9466470988143,4.48387106455671));
#90740=CARTESIAN_POINT('Ctrl Pts',(-11.0772882471084,19.9471418672051,4.49060228352051));
#90741=CARTESIAN_POINT('Ctrl Pts',(-11.0750817145551,19.9473189829016,4.49299655491857));
#90742=CARTESIAN_POINT('Ctrl Pts',(-11.070970406837,19.9476489356556,4.49742789991519));
#90743=CARTESIAN_POINT('Ctrl Pts',(-11.0690677888058,19.9478016115908,4.49946690310272));
#90744=CARTESIAN_POINT('Ctrl Pts',(-11.0647321257125,19.9481494792712,4.50408681455575));
#90745=CARTESIAN_POINT('Ctrl Pts',(-11.0622955292365,19.9483449388795,4.50666431282053));
#90746=CARTESIAN_POINT('Ctrl Pts',(-11.0548368119417,19.9489430750938,4.51449711201356));
#90747=CARTESIAN_POINT('Ctrl Pts',(-11.0497849638866,19.9493479374495,4.51972379360995));
#90748=CARTESIAN_POINT('Ctrl Pts',(-10.9973166870003,19.9535480618291,4.57320476829084));
#90749=CARTESIAN_POINT('Ctrl Pts',(-10.9466519623634,19.9575607837162,4.61814901091992));
#90750=CARTESIAN_POINT('Ctrl Pts',(-10.8155309465143,19.9674944744758,4.71914738886183));
#90751=CARTESIAN_POINT('Ctrl Pts',(-10.7321900783782,19.9734276613691,4.77094935954187));
#90752=CARTESIAN_POINT('Ctrl Pts',(-10.6035892678925,19.981731678141,4.83400441758086));
#90753=CARTESIAN_POINT('Ctrl Pts',(-10.5619730248338,19.9843046070277,4.85206314072622));
#90754=CARTESIAN_POINT('Ctrl Pts',(-10.5098115728236,19.9873909470546,4.87187231149635));
#90755=CARTESIAN_POINT('Ctrl Pts',(-10.5000015117888,19.9879655865824,4.87547808961509));
#90756=CARTESIAN_POINT('Ctrl Pts',(-10.4844409418412,19.9888680814775,4.88100904412464));
#90757=CARTESIAN_POINT('Ctrl Pts',(-10.4787157788796,19.9891982280175,4.88300405302513));
#90758=CARTESIAN_POINT('Ctrl Pts',(-10.4682723614392,19.9897970412564,4.8865705804098));
#90759=CARTESIAN_POINT('Ctrl Pts',(-10.4635581995058,19.9900660861239,4.88815372904553));
#90760=CARTESIAN_POINT('Ctrl Pts',(-10.4533538328366,19.9906457840905,4.89152286464655));
#90761=CARTESIAN_POINT('Ctrl Pts',(-10.4478609314645,19.9909561594179,4.89330045860854));
#90762=CARTESIAN_POINT('Ctrl Pts',(-10.4329018083687,19.9917969707834,4.89804387500847));
#90763=CARTESIAN_POINT('Ctrl Pts',(-10.4234156256785,19.9923253363793,4.9009460612596));
#90764=CARTESIAN_POINT('Ctrl Pts',(-10.3759981773585,19.9949433026962,4.9149272425878));
#90765=CARTESIAN_POINT('Ctrl Pts',(-10.3376569643441,19.9969861760379,4.92456374435216));
#90766=CARTESIAN_POINT('Ctrl Pts',(-10.1933314996131,20.0044628337437,4.95468234666377));
#90767=CARTESIAN_POINT('Ctrl Pts',(-10.085582600919,20.0095961482466,4.96497560605187));
#90768=CARTESIAN_POINT('Ctrl Pts',(-9.93223798521164,20.0171259017573,4.96263666909413));
#90769=CARTESIAN_POINT('Ctrl Pts',(-9.88685558545205,20.0193869070532,4.95982722601458));
#90770=CARTESIAN_POINT('Ctrl Pts',(-9.81920132561252,20.0228969208704,4.95246528142579));
#90771=CARTESIAN_POINT('Ctrl Pts',(-9.79678290986956,20.0240832829943,4.94949862250487));
#90772=CARTESIAN_POINT('Ctrl Pts',(-9.76907088632763,20.0255884524901,4.94517596216321));
#90773=CARTESIAN_POINT('Ctrl Pts',(-9.76370308324525,20.025881813155,4.9443079943049));
#90774=CARTESIAN_POINT('Ctrl Pts',(-9.75522259962754,20.0263483268957,4.94288816855444));
#90775=CARTESIAN_POINT('Ctrl Pts',(-9.75210660161655,20.0265203889804,4.94235609519179));
#90776=CARTESIAN_POINT('Ctrl Pts',(-9.74622973931599,20.0268461714822,4.94133298314577));
#90777=CARTESIAN_POINT('Ctrl Pts',(-9.74346854891021,20.0269997706503,4.94084410247839));
#90778=CARTESIAN_POINT('Ctrl Pts',(-9.73713274226629,20.0273534286572,4.93970353108384));
#90779=CARTESIAN_POINT('Ctrl Pts',(-9.7335591358612,20.0275537865757,4.93904646135372));
#90780=CARTESIAN_POINT('Ctrl Pts',(-9.72401383756117,20.0280912465118,4.9372546180525));
#90781=CARTESIAN_POINT('Ctrl Pts',(-9.71804677158459,20.0284296321021,4.93609594851646));
#90782=CARTESIAN_POINT('Ctrl Pts',(-9.67297060853479,20.0310031405718,4.92705141391336));
#90783=CARTESIAN_POINT('Ctrl Pts',(-9.6341944705975,20.0333152283376,4.91760704557434));
#90784=CARTESIAN_POINT('Ctrl Pts',(-9.51498865217206,20.0406331690028,4.88335665986826));
#90785=CARTESIAN_POINT('Ctrl Pts',(-9.43627649046886,20.0457596692194,4.8531916083317));
#90786=CARTESIAN_POINT('Ctrl Pts',(-9.30808656344019,20.054269218602,4.79092806692027));
#90787=CARTESIAN_POINT('Ctrl Pts',(-9.257149914964,20.0577005568928,4.76230516518392));
#90788=CARTESIAN_POINT('Ctrl Pts',(-9.18058141997299,20.0628992716039,4.7130345388412));
#90789=CARTESIAN_POINT('Ctrl Pts',(-9.15370597226154,20.0647331819932,4.69443972641523));
#90790=CARTESIAN_POINT('Ctrl Pts',(-9.1202265976167,20.067030823902,4.66957791442647));
#90791=CARTESIAN_POINT('Ctrl Pts',(-9.11302914614311,20.0675256000719,4.66412905083237));
#90792=CARTESIAN_POINT('Ctrl Pts',(-9.10151379913323,20.0683186557842,4.65524250614175));
#90793=CARTESIAN_POINT('Ctrl Pts',(-9.09716420560889,20.0686185498206,4.65184644405158));
#90794=CARTESIAN_POINT('Ctrl Pts',(-9.08890345856685,20.0691887985716,4.64532110333304));
#90795=CARTESIAN_POINT('Ctrl Pts',(-9.0849889663023,20.0694593197919,4.64219619445404));
#90796=CARTESIAN_POINT('Ctrl Pts',(-9.0760668757816,20.0700766320864,4.63499845563891));
#90797=CARTESIAN_POINT('Ctrl Pts',(-9.07107000477661,20.0704228917358,4.63091245378506));
#90798=CARTESIAN_POINT('Ctrl Pts',(-9.05807529974231,20.0713248685701,4.62014228900869));
#90799=CARTESIAN_POINT('Ctrl Pts',(-9.05012147631755,20.0718784591431,4.61340544560104));
#90800=CARTESIAN_POINT('Ctrl Pts',(-8.99060649724521,20.0760338106523,4.56189462289946));
#90801=CARTESIAN_POINT('Ctrl Pts',(-8.94216107780299,20.0794856497431,4.51364379344618));
#90802=CARTESIAN_POINT('Ctrl Pts',(-8.82090775052224,20.088594213038,4.37467711684604));
#90803=CARTESIAN_POINT('Ctrl Pts',(-8.75525199999838,20.0940493923356,4.27840623879632));
#90804=CARTESIAN_POINT('Ctrl Pts',(-8.68883131744937,20.101408550492,4.15072465069198));
#90805=CARTESIAN_POINT('Ctrl Pts',(-8.67670198426008,20.1028585582181,4.12569005688965));
#90806=CARTESIAN_POINT('Ctrl Pts',(-8.66291862210883,20.1046595622595,4.09504552216817));
#90807=CARTESIAN_POINT('Ctrl Pts',(-8.66057460421397,20.1049716924913,4.08975027887022));
#90808=CARTESIAN_POINT('Ctrl Pts',(-8.65696872266202,20.1054613020736,4.08147203527022));
#90809=CARTESIAN_POINT('Ctrl Pts',(-8.65568520457998,20.1056375007327,4.07849846162943));
#90810=CARTESIAN_POINT('Ctrl Pts',(-8.65331407255141,20.105966652738,4.07295466815457));
#90811=CARTESIAN_POINT('Ctrl Pts',(-8.65222393429799,20.1061194520176,4.07038558472665));
#90812=CARTESIAN_POINT('Ctrl Pts',(-8.64975561755191,20.1064687898988,4.06452201956107));
#90813=CARTESIAN_POINT('Ctrl Pts',(-8.64838214960475,20.1066656056578,4.06122561313357));
#90814=CARTESIAN_POINT('Ctrl Pts',(-8.64483321232762,20.1071804903288,4.05261935804939));
#90815=CARTESIAN_POINT('Ctrl Pts',(-8.64267690451335,20.1074996534187,4.04730173538273));
#90816=CARTESIAN_POINT('Ctrl Pts',(-8.62860841617458,20.1096237828037,4.01201321328187));
#90817=CARTESIAN_POINT('Ctrl Pts',(-8.61765928472868,20.1114792022709,3.98167026739948));
#90818=CARTESIAN_POINT('Ctrl Pts',(-8.60155070411231,20.1145390255567,3.93194083336622));
#90819=CARTESIAN_POINT('Ctrl Pts',(-8.59577116960505,20.1157234148815,3.91276465707285));
#90820=CARTESIAN_POINT('Ctrl Pts',(-8.56598398722431,20.1223187691706,3.80605334431026));
#90821=CARTESIAN_POINT('Ctrl Pts',(-8.54976519530505,20.1278518134404,3.71654317708157));
#90822=CARTESIAN_POINT('Ctrl Pts',(-8.5365463112622,20.1369153886528,3.56370697262953));
#90823=CARTESIAN_POINT('Ctrl Pts',(-8.53516014243279,20.1405297619297,3.50101843937636));
#90824=CARTESIAN_POINT('Ctrl Pts',(-8.53843054103904,20.1448618922449,3.42335428389944));
#90825=CARTESIAN_POINT('Ctrl Pts',(-8.53929830524962,20.145695511967,3.40829159212638));
#90826=CARTESIAN_POINT('Ctrl Pts',(-8.54089122637371,20.1468916628035,3.3865125576196));
#90827=CARTESIAN_POINT('Ctrl Pts',(-8.54143018333722,20.1472599459972,3.37978392408118));
#90828=CARTESIAN_POINT('Ctrl Pts',(-8.54245381853221,20.1479012922292,3.36802691743868));
#90829=CARTESIAN_POINT('Ctrl Pts',(-8.54291801159393,20.1481749879302,3.36299691396326));
#90830=CARTESIAN_POINT('Ctrl Pts',(-8.54386784882309,20.1487037147638,3.35325588076138));
#90831=CARTESIAN_POINT('Ctrl Pts',(-8.54435033592137,20.1489588406352,3.34854461245758));
#90832=CARTESIAN_POINT('Ctrl Pts',(-8.54569334081858,20.149634973573,3.33603044422757));
#90833=CARTESIAN_POINT('Ctrl Pts',(-8.54659379200469,20.1500547317036,3.32823192388808));
#90834=CARTESIAN_POINT('Ctrl Pts',(-8.55006476100666,20.151560509562,3.30015545562132));
#90835=CARTESIAN_POINT('Ctrl Pts',(-8.55299733502293,20.1526352414854,3.27992414731093));
#90836=CARTESIAN_POINT('Ctrl Pts',(-8.57694637552225,20.1602196344993,3.13600974533993));
#90837=CARTESIAN_POINT('Ctrl Pts',(-8.61336381114822,20.1661953764286,3.01542606630461));
#90838=CARTESIAN_POINT('Ctrl Pts',(-8.68511682441223,20.1747735245407,2.85548579061879));
#90839=CARTESIAN_POINT('Ctrl Pts',(-8.70782597164135,20.1772404552128,2.81108639091288));
#90840=CARTESIAN_POINT('Ctrl Pts',(-8.74473829586202,20.1810376048559,2.74718904692318));
#90841=CARTESIAN_POINT('Ctrl Pts',(-8.75722984462729,20.1822925080247,2.72674164333686));
#90842=CARTESIAN_POINT('Ctrl Pts',(-8.77321883862008,20.1838747351751,2.70195808637215));
#90843=CARTESIAN_POINT('Ctrl Pts',(-8.77624714639873,20.1841734058537,2.69732206636208));
#90844=CARTESIAN_POINT('Ctrl Pts',(-8.78105755855642,20.1846464574002,2.69004833033907));
#90845=CARTESIAN_POINT('Ctrl Pts',(-8.78282211547801,20.1848196949302,2.68739900333979));
#90846=CARTESIAN_POINT('Ctrl Pts',(-8.7861548079016,20.1851463901751,2.6824304693737));
#90847=CARTESIAN_POINT('Ctrl Pts',(-8.78772096234364,20.1852997171273,2.68010999384232));
#90848=CARTESIAN_POINT('Ctrl Pts',(-8.79131437112047,20.1856510475614,2.67481866461764));
#90849=CARTESIAN_POINT('Ctrl Pts',(-8.79334592384373,20.1858493363044,2.67185078298052));
#90850=CARTESIAN_POINT('Ctrl Pts',(-8.79876878814064,20.1863776742684,2.66399087401409));
#90851=CARTESIAN_POINT('Ctrl Pts',(-8.80217900562572,20.1867089410639,2.65911204904806));
#90852=CARTESIAN_POINT('Ctrl Pts',(-8.82682714070199,20.1890954623381,2.62430339839722));
#90853=CARTESIAN_POINT('Ctrl Pts',(-8.84915291529124,20.1912159345142,2.59516319161518));
#90854=CARTESIAN_POINT('Ctrl Pts',(-8.87972668534691,20.1940364214541,2.55822151439551));
#90855=CARTESIAN_POINT('Ctrl Pts',(-8.88700499943113,20.194702149994,2.54963105271912));
#90856=CARTESIAN_POINT('Ctrl Pts',(-8.95147161846621,20.2005438771801,2.47529860735073));
#90857=CARTESIAN_POINT('Ctrl Pts',(-9.01432657908907,20.20585512046,2.41470124228506));
#90858=CARTESIAN_POINT('Ctrl Pts',(-9.14150650408248,20.2155483707541,2.31230548975715));
#90859=CARTESIAN_POINT('Ctrl Pts',(-9.20445396068216,20.2199500440195,2.26925280390683));
#90860=CARTESIAN_POINT('Ctrl Pts',(-9.2802683397965,20.2247912977481,2.22565851654451));
#90861=CARTESIAN_POINT('Ctrl Pts',(-9.29012705390789,20.22541263905,2.22014051957886));
#90862=CARTESIAN_POINT('Ctrl Pts',(-9.30532780934558,20.2263583645299,2.21186222408904));
#90863=CARTESIAN_POINT('Ctrl Pts',(-9.31062446141557,20.2266856428689,2.20901984891106));
#90864=CARTESIAN_POINT('Ctrl Pts',(-9.32029141185334,20.2272789147652,2.20390867235254));
#90865=CARTESIAN_POINT('Ctrl Pts',(-9.32465591580488,20.2275452821668,2.20162915037062));
#90866=CARTESIAN_POINT('Ctrl Pts',(-9.33418522465892,20.2281236643144,2.1967131706401));
#90867=CARTESIAN_POINT('Ctrl Pts',(-9.33935437557597,20.2284353765932,2.19408528804474));
#90868=CARTESIAN_POINT('Ctrl Pts',(-9.35350744191571,20.229283397555,2.18699572113506));
#90869=CARTESIAN_POINT('Ctrl Pts',(-9.36252191641759,20.229817575014,2.1825955201098));
#90870=CARTESIAN_POINT('Ctrl Pts',(-9.40858284789632,20.2325178573159,2.16069546385885));
#90871=CARTESIAN_POINT('Ctrl Pts',(-9.44630887479806,20.2346335084292,2.14466335553089));
#90872=CARTESIAN_POINT('Ctrl Pts',(-9.49715144604226,20.237383787494,2.12553512524404));
#90873=CARTESIAN_POINT('Ctrl Pts',(-9.50970634464722,20.238055059588,2.12100670681927));
#90874=CARTESIAN_POINT('Ctrl Pts',(-9.61741858922705,20.2437543062467,2.08381305978538));
#90875=CARTESIAN_POINT('Ctrl Pts',(-9.71564390338453,20.2485335490283,2.06087005775287));
#90876=CARTESIAN_POINT('Ctrl Pts',(-9.86780638118246,20.2561052832374,2.04152711392916));
#90877=CARTESIAN_POINT('Ctrl Pts',(-9.92048533613664,20.2587614331918,2.03770909016852));
#90878=CARTESIAN_POINT('Ctrl Pts',(-9.98358392284736,20.2621000305162,2.03655557374408));
#90879=CARTESIAN_POINT('Ctrl Pts',(-9.99391929905978,20.2626519388117,2.03647613981034));
#90880=CARTESIAN_POINT('Ctrl Pts',(-10.0083440081236,20.263430325154,2.03651807222002));
#90881=CARTESIAN_POINT('Ctrl Pts',(-10.0124335441541,20.2636519144459,2.03654710305693));
#90882=CARTESIAN_POINT('Ctrl Pts',(-10.019391160707,20.2640305366273,2.03662565926711));
#90883=CARTESIAN_POINT('Ctrl Pts',(-10.0222593511513,20.2641870898066,2.03666647704751));
#90884=CARTESIAN_POINT('Ctrl Pts',(-10.0277627432949,20.2644884120598,2.03676098084255));
#90885=CARTESIAN_POINT('Ctrl Pts',(-10.0303979413271,20.2646331031827,2.03681335365757));
#90886=CARTESIAN_POINT('Ctrl Pts',(-10.0374091493145,20.265019129146,2.03697164541255));
#90887=CARTESIAN_POINT('Ctrl Pts',(-10.041784814132,20.2652611459357,2.03709007827683));
#90888=CARTESIAN_POINT('Ctrl Pts',(-10.0574987389489,20.2661340674989,2.03758595327695));
#90889=CARTESIAN_POINT('Ctrl Pts',(-10.0688327591201,20.2667707669853,2.03807558877922));
#90890=CARTESIAN_POINT('Ctrl Pts',(-10.1604276562741,20.271967304551,2.04310001409775));
#90891=CARTESIAN_POINT('Ctrl Pts',(-10.2401898155471,20.2768026957063,2.05410883386141));
#90892=CARTESIAN_POINT('Ctrl Pts',(-10.3896838983912,20.2860268533023,2.08745705147466));
#90893=CARTESIAN_POINT('Ctrl Pts',(-10.4594546316017,20.2904020272699,2.10858559824966));
#90894=CARTESIAN_POINT('Ctrl Pts',(-10.5596304521911,20.296661804801,2.14728337512537));
#90895=CARTESIAN_POINT('Ctrl Pts',(-10.591443492704,20.2986475688073,2.16088709546936));
#90896=CARTESIAN_POINT('Ctrl Pts',(-10.6364614171583,20.3014516181678,2.18205508334331));
#90897=CARTESIAN_POINT('Ctrl Pts',(-10.6500757115573,20.302298871294,2.18871683751952));
#90898=CARTESIAN_POINT('Ctrl Pts',(-10.6742420256568,20.3038016939787,2.20101080816636));
#90899=CARTESIAN_POINT('Ctrl Pts',(-10.6848329770508,20.3044599242566,2.20656309193725));
#90900=CARTESIAN_POINT('Ctrl Pts',(-10.7007647087862,20.3054497143361,2.21516581931488));
#90901=CARTESIAN_POINT('Ctrl Pts',(-10.7061560943078,20.305784600662,2.21812105835928));
#90902=CARTESIAN_POINT('Ctrl Pts',(-10.7158787468092,20.3063884557543,2.22353039614543));
#90903=CARTESIAN_POINT('Ctrl Pts',(-10.7202163984983,20.3066578341839,2.22597277506286));
#90904=CARTESIAN_POINT('Ctrl Pts',(-10.7295002775941,20.3072343671388,2.23126276655002));
#90905=CARTESIAN_POINT('Ctrl Pts',(-10.7344424899993,20.3075412696311,2.23411728319668));
#90906=CARTESIAN_POINT('Ctrl Pts',(-10.7476810766338,20.30836340778,2.24186723688362));
#90907=CARTESIAN_POINT('Ctrl Pts',(-10.755946104479,20.3088767267961,2.24681584152321));
#90908=CARTESIAN_POINT('Ctrl Pts',(-10.7950240835078,20.3113047345628,2.27074068856318));
#90909=CARTESIAN_POINT('Ctrl Pts',(-10.8251763487629,20.3131806510007,2.29077461979789));
#90910=CARTESIAN_POINT('Ctrl Pts',(-10.8651413145503,20.3156867944579,2.31952011808858));
#90911=CARTESIAN_POINT('Ctrl Pts',(-10.8756239216902,20.3163461281453,2.3272745400654));
#90912=CARTESIAN_POINT('Ctrl Pts',(-10.9946079416295,20.3238613759719,2.4177769071366));
#90913=CARTESIAN_POINT('Ctrl Pts',(-11.0911133593024,20.3301888480836,2.515156556385));
#90914=CARTESIAN_POINT('Ctrl Pts',(-11.1904582184754,20.338656052466,2.64822558186085));
#90915=CARTESIAN_POINT('Ctrl Pts',(-11.2074599293953,20.340197590524,2.67250334696458));
#90916=CARTESIAN_POINT('Ctrl Pts',(-11.226945813418,20.3421010590452,2.7022086836613));
#90917=CARTESIAN_POINT('Ctrl Pts',(-11.2301498895593,20.3424187715151,2.7071581113905));
#90918=CARTESIAN_POINT('Ctrl Pts',(-11.2350798223213,20.3429152410791,2.71487534692116));
#90919=CARTESIAN_POINT('Ctrl Pts',(-11.2368265174964,20.3430926585387,2.71762984874807));
#90920=CARTESIAN_POINT('Ctrl Pts',(-11.2400493021347,20.3434228784913,2.72274987755209));
#90921=CARTESIAN_POINT('Ctrl Pts',(-11.2415278473529,20.3435755175543,2.72511379646284));
#90922=CARTESIAN_POINT('Ctrl Pts',(-11.2448678190451,20.3439229182395,2.7304878889549));
#90923=CARTESIAN_POINT('Ctrl Pts',(-11.2467250788109,20.3441179447524,2.7335005849578));
#90924=CARTESIAN_POINT('Ctrl Pts',(-11.2523432060185,20.3447134725718,2.74268829437434));
#90925=CARTESIAN_POINT('Ctrl Pts',(-11.2560691993536,20.3451161325203,2.74888437162551));
#90926=CARTESIAN_POINT('Ctrl Pts',(-11.2908077781177,20.3489419413125,2.80763365642851));
#90927=CARTESIAN_POINT('Ctrl Pts',(-11.3185479375074,20.3525426105373,2.86204570177406));
#90928=CARTESIAN_POINT('Ctrl Pts',(-11.3893517097413,20.363200834911,3.02541299193128));
#90929=CARTESIAN_POINT('Ctrl Pts',(-11.4228513669856,20.3703211528115,3.13801665847732));
#90930=CARTESIAN_POINT('Ctrl Pts',(-11.4465537972481,20.3783824205192,3.27668071001339));
#90931=CARTESIAN_POINT('Ctrl Pts',(-11.4499675176857,20.3797190755843,3.30004080417767));
#90932=CARTESIAN_POINT('Ctrl Pts',(-11.454858658206,20.3819857504721,3.34029510375796));
#90933=CARTESIAN_POINT('Ctrl Pts',(-11.456610268367,20.3829239293748,3.35715067641398));
#90934=CARTESIAN_POINT('Ctrl Pts',(-11.4586774587503,20.384240732325,3.3810784909363));
#90935=CARTESIAN_POINT('Ctrl Pts',(-11.4592350435477,20.3846268445503,3.38812800115375));
#90936=CARTESIAN_POINT('Ctrl Pts',(-11.4601072646536,20.3852890471085,3.4002748617643));
#90937=CARTESIAN_POINT('Ctrl Pts',(-11.4604463513216,20.3855658931273,3.40537028309883));
#90938=CARTESIAN_POINT('Ctrl Pts',(-11.461043816564,20.386093757596,3.41511816026283));
#90939=CARTESIAN_POINT('Ctrl Pts',(-11.4613066591182,20.3863449115146,3.41977027143469));
#90940=CARTESIAN_POINT('Ctrl Pts',(-11.4619313921308,20.3869952065732,3.43185177820457));
#90941=CARTESIAN_POINT('Ctrl Pts',(-11.4622588719079,20.3873932758838,3.4392828712037));
#90942=CARTESIAN_POINT('Ctrl Pts',(-11.4631764913181,20.3887362282574,3.46446963435414));
#90943=CARTESIAN_POINT('Ctrl Pts',(-11.4635,20.3896728624995,3.48223381506111));
#90944=CARTESIAN_POINT('Ctrl Pts',(-11.4635,20.390600218991,3.49999999999975));
#90945=CARTESIAN_POINT('Origin',(-10.,13.2,3.5));
#90946=CARTESIAN_POINT('',(-11.4635,20.9613838610471,3.50000000002865));
#90947=CARTESIAN_POINT('',(-11.4635,20.8884018418444,3.49999999996669));
#90948=CARTESIAN_POINT('',(-11.4635,13.2,3.5));
#90949=CARTESIAN_POINT('Ctrl Pts',(-11.4635,20.9613838610471,3.50000000002865));
#90950=CARTESIAN_POINT('Ctrl Pts',(-11.4635000000015,20.9566884958894,3.42124724916301));
#90951=CARTESIAN_POINT('Ctrl Pts',(-11.4571434721348,20.9518997548335,3.34261904798223));
#90952=CARTESIAN_POINT('Ctrl Pts',(-11.4331286661958,20.9430155565538,3.19508157007876));
#90953=CARTESIAN_POINT('Ctrl Pts',(-11.4167227184934,20.9389100987044,3.12619260529468));
#90954=CARTESIAN_POINT('Ctrl Pts',(-11.3905528339483,20.9340650164995,3.04343324048439));
#90955=CARTESIAN_POINT('Ctrl Pts',(-11.3854566224749,20.9331762716414,3.02819456757604));
#90956=CARTESIAN_POINT('Ctrl Pts',(-11.3778073980026,20.9319163802089,3.00651552347577));
#90957=CARTESIAN_POINT('Ctrl Pts',(-11.3754581361996,20.9315385925182,3.0000049275953));
#90958=CARTESIAN_POINT('Ctrl Pts',(-11.3713051704093,20.9308862479867,2.9887464709405));
#90959=CARTESIAN_POINT('Ctrl Pts',(-11.3695227892526,20.9306109929557,2.98399091869568));
#90960=CARTESIAN_POINT('Ctrl Pts',(-11.3660468584145,20.9300831216393,2.97486170757454));
#90961=CARTESIAN_POINT('Ctrl Pts',(-11.3643569703184,20.9298303880588,2.97048672934046));
#90962=CARTESIAN_POINT('Ctrl Pts',(-11.360317984819,20.9292353909773,2.96017784564874));
#90963=CARTESIAN_POINT('Ctrl Pts',(-11.3579510357184,20.9288937256505,2.95425100596183));
#90964=CARTESIAN_POINT('Ctrl Pts',(-11.3495391842833,20.9277034784807,2.93358131525659));
#90965=CARTESIAN_POINT('Ctrl Pts',(-11.3432922327071,20.92686165002,2.91892157149693));
#90966=CARTESIAN_POINT('Ctrl Pts',(-11.2862567703959,20.919524474884,2.79091435411472));
#90967=CARTESIAN_POINT('Ctrl Pts',(-11.2214726632592,20.9135689753299,2.68436174290968));
#90968=CARTESIAN_POINT('Ctrl Pts',(-11.1374322571354,20.9069960955733,2.57902704816759));
#90969=CARTESIAN_POINT('Ctrl Pts',(-11.1307707738241,20.9064810956157,2.57086019777578));
#90970=CARTESIAN_POINT('Ctrl Pts',(-11.093548450587,20.9036322660254,2.52621958308996));
#90971=CARTESIAN_POINT('Ctrl Pts',(-11.0613127912209,20.9012709048846,2.49118332353302));
#90972=CARTESIAN_POINT('Ctrl Pts',(-11.0164020946423,20.8980219838253,2.44690985430923));
#90973=CARTESIAN_POINT('Ctrl Pts',(-11.0052022405265,20.897214819632,2.43621407474553));
#90974=CARTESIAN_POINT('Ctrl Pts',(-10.9885461216265,20.8960151428804,2.42080551798409));
#90975=CARTESIAN_POINT('Ctrl Pts',(-10.9832211047394,20.8956317058716,2.41595183695281));
#90976=CARTESIAN_POINT('Ctrl Pts',(-10.9736336167589,20.8949410688944,2.40734172433269));
#90977=CARTESIAN_POINT('Ctrl Pts',(-10.969384666537,20.894634900307,2.40357038838521));
#90978=CARTESIAN_POINT('Ctrl Pts',(-10.9626836765125,20.8941516993163,2.39769203931977));
#90979=CARTESIAN_POINT('Ctrl Pts',(-10.9602463840394,20.8939758780837,2.39556820820464));
#90980=CARTESIAN_POINT('Ctrl Pts',(-10.9577922516998,20.8937987479549,2.39344396763952));
#90981=CARTESIAN_POINT('Ctrl Pts',(-10.9577824043896,20.8937980372112,2.39343544426394));
#90982=CARTESIAN_POINT('Ctrl Pts',(-10.9577625910322,20.8937966071508,2.39341829520226));
#90983=CARTESIAN_POINT('Ctrl Pts',(-10.9577526250649,20.8937958878398,2.39340966959089));
#90984=CARTESIAN_POINT('Ctrl Pts',(-10.9577325723636,20.8937944404981,2.39339231431746));
#90985=CARTESIAN_POINT('Ctrl Pts',(-10.9577224855433,20.8937937124611,2.39338358458646));
#90986=CARTESIAN_POINT('Ctrl Pts',(-10.9577021890507,20.8937922475169,2.39336601928647));
#90987=CARTESIAN_POINT('Ctrl Pts',(-10.9576919792924,20.8937915106034,2.39335718364902));
#90988=CARTESIAN_POINT('Ctrl Pts',(-10.9576714346564,20.8937900277423,2.39333940459143));
#90989=CARTESIAN_POINT('Ctrl Pts',(-10.9576610998094,20.8937892817969,2.39333046120418));
#90990=CARTESIAN_POINT('Ctrl Pts',(-10.955543813586,20.8936364606164,2.39149829332148));
#90991=CARTESIAN_POINT('Ctrl Pts',(-10.9534317135231,20.8934839401861,2.38968113558982));
#90992=CARTESIAN_POINT('Ctrl Pts',(-10.9486368968294,20.8931375324251,2.38557965608107));
#90993=CARTESIAN_POINT('Ctrl Pts',(-10.9459511253157,20.8929433859604,2.38329899572709));
#90994=CARTESIAN_POINT('Ctrl Pts',(-10.9389884904475,20.8924398564311,2.37742971949755));
#90995=CARTESIAN_POINT('Ctrl Pts',(-10.9346993211786,20.8921294545162,2.37385587209659));
#90996=CARTESIAN_POINT('Ctrl Pts',(-10.9077062966974,20.8901752461793,2.35162502672633));
#90997=CARTESIAN_POINT('Ctrl Pts',(-10.8844666890242,20.8884895356405,2.3336320316125));
#90998=CARTESIAN_POINT('Ctrl Pts',(-10.7739230435552,20.8805162809182,2.25324897094252));
#90999=CARTESIAN_POINT('Ctrl Pts',(-10.6804677286658,20.8739303276766,2.19988095798401));
#91000=CARTESIAN_POINT('Ctrl Pts',(-10.5193331488387,20.8635097544077,2.13003916366665));
#91001=CARTESIAN_POINT('Ctrl Pts',(-10.4548186481774,20.8595505648093,2.10728983163349));
#91002=CARTESIAN_POINT('Ctrl Pts',(-10.3737281073614,20.854857397976,2.08493510917998));
#91003=CARTESIAN_POINT('Ctrl Pts',(-10.3584457304731,20.8539846334208,2.08098695242332));
#91004=CARTESIAN_POINT('Ctrl Pts',(-10.3364215302781,20.8527431929175,2.07567558864699));
#91005=CARTESIAN_POINT('Ctrl Pts',(-10.3297296752626,20.8523681395848,2.07411156876902));
#91006=CARTESIAN_POINT('Ctrl Pts',(-10.3180819573915,20.8517189926481,2.07147564813582));
#91007=CARTESIAN_POINT('Ctrl Pts',(-10.3131311194847,20.8514442196876,2.07038226843804));
#91008=CARTESIAN_POINT('Ctrl Pts',(-10.3035783435721,20.8509162108358,2.06832456694155));
#91009=CARTESIAN_POINT('Ctrl Pts',(-10.2989772505817,20.8506628639093,2.06735665266818));
#91010=CARTESIAN_POINT('Ctrl Pts',(-10.2880746531643,20.8500647958731,2.06511792583211));
#91011=CARTESIAN_POINT('Ctrl Pts',(-10.2817692534615,20.8497206882825,2.0638664191107));
#91012=CARTESIAN_POINT('Ctrl Pts',(-10.2595367102829,20.8485134826897,2.05960572454648));
#91013=CARTESIAN_POINT('Ctrl Pts',(-10.243567702511,20.8476573987832,2.05681956271455));
#91014=CARTESIAN_POINT('Ctrl Pts',(-10.1078104846959,20.8404654213748,2.03545119233245));
#91015=CARTESIAN_POINT('Ctrl Pts',(-9.98619094863813,20.8346392857349,2.03155249908111));
#91016=CARTESIAN_POINT('Ctrl Pts',(-9.80821563139624,20.8259285765369,2.04798154784805));
#91017=CARTESIAN_POINT('Ctrl Pts',(-9.75132118218259,20.8231057413387,2.0566369880701));
#91018=CARTESIAN_POINT('Ctrl Pts',(-9.66954216945178,20.818818723098,2.07405748298735));
#91019=CARTESIAN_POINT('Ctrl Pts',(-9.64414836847395,20.8174543131188,2.08018174105154));
#91020=CARTESIAN_POINT('Ctrl Pts',(-9.61344604106461,20.8157492806381,2.08846162265551));
#91021=CARTESIAN_POINT('Ctrl Pts',(-9.60796719937263,20.8154428458867,2.08997346302112));
#91022=CARTESIAN_POINT('Ctrl Pts',(-9.59940358505597,20.8149602768334,2.09239028976283));
#91023=CARTESIAN_POINT('Ctrl Pts',(-9.5963126919099,20.8147853645206,2.09327360837324));
#91024=CARTESIAN_POINT('Ctrl Pts',(-9.59054176420462,20.8144573688773,2.09494341597724));
#91025=CARTESIAN_POINT('Ctrl Pts',(-9.58786105753331,20.8143044299725,2.0957273972463));
#91026=CARTESIAN_POINT('Ctrl Pts',(-9.58172649798214,20.8139531261873,2.09754054755735));
#91027=CARTESIAN_POINT('Ctrl Pts',(-9.57827420040487,20.8137544712946,2.09857480127582));
#91028=CARTESIAN_POINT('Ctrl Pts',(-9.56922865056005,20.8132315245625,2.10132115537344));
#91029=CARTESIAN_POINT('Ctrl Pts',(-9.56364183803928,20.8129060827301,2.1030540389614));
#91030=CARTESIAN_POINT('Ctrl Pts',(-9.52513661950051,20.8106468455845,2.11525087553652));
#91031=CARTESIAN_POINT('Ctrl Pts',(-9.49258960908891,20.8086552152174,2.12684316490263));
#91032=CARTESIAN_POINT('Ctrl Pts',(-9.43313310578712,20.8049016749588,2.15042228365196));
#91033=CARTESIAN_POINT('Ctrl Pts',(-9.40611468908789,20.8031501745572,2.16209185516065));
#91034=CARTESIAN_POINT('Ctrl Pts',(-9.30617271356306,20.7965392716831,2.20888205228234));
#91035=CARTESIAN_POINT('Ctrl Pts',(-9.23584606064211,20.7916267791755,2.24921951193989));
#91036=CARTESIAN_POINT('Ctrl Pts',(-9.11908595498904,20.7832592713526,2.3297306721709));
#91037=CARTESIAN_POINT('Ctrl Pts',(-9.07115966331733,20.7797501902482,2.3673937441244));
#91038=CARTESIAN_POINT('Ctrl Pts',(-9.01462412332571,20.7755293273988,2.4178320225422));
#91039=CARTESIAN_POINT('Ctrl Pts',(-9.00368468848392,20.7747082759455,2.42789507383177));
#91040=CARTESIAN_POINT('Ctrl Pts',(-8.98803283551275,20.7735268174833,2.44273952670517));
#91041=CARTESIAN_POINT('Ctrl Pts',(-8.98319726108917,20.7731608519179,2.44738922548098));
#91042=CARTESIAN_POINT('Ctrl Pts',(-8.97478253016123,20.7725222597703,2.45559259637408));
#91043=CARTESIAN_POINT('Ctrl Pts',(-8.97118948139539,20.7722490158112,2.45913180329861));
#91044=CARTESIAN_POINT('Ctrl Pts',(-8.96425129159652,20.7717202398729,2.46603705007871));
#91045=CARTESIAN_POINT('Ctrl Pts',(-8.96090408995374,20.7714646185943,2.46940092216979));
#91046=CARTESIAN_POINT('Ctrl Pts',(-8.95202405150034,20.7707850189206,2.47841242772935));
#91047=CARTESIAN_POINT('Ctrl Pts',(-8.94652047382456,20.7703623145763,2.48408875992992));
#91048=CARTESIAN_POINT('Ctrl Pts',(-8.92671803572117,20.7688355584821,2.50484675792464));
#91049=CARTESIAN_POINT('Ctrl Pts',(-8.91269447507775,20.7677432137784,2.52018833319449));
#91050=CARTESIAN_POINT('Ctrl Pts',(-8.8165888678351,20.760163670269,2.62993186321281));
#91051=CARTESIAN_POINT('Ctrl Pts',(-8.74658411849937,20.7542053861851,2.73421258703406));
#91052=CARTESIAN_POINT('Ctrl Pts',(-8.66845912207229,20.7456481831522,2.89064997688716));
#91053=CARTESIAN_POINT('Ctrl Pts',(-8.64851249880959,20.7431848872761,2.93627183374724));
#91054=CARTESIAN_POINT('Ctrl Pts',(-8.62247140949482,20.7393928630961,3.00520704998095));
#91055=CARTESIAN_POINT('Ctrl Pts',(-8.61456445921144,20.7381392244046,3.02779950017673));
#91056=CARTESIAN_POINT('Ctrl Pts',(-8.605515885078,20.7365584842016,3.05584131981198));
#91057=CARTESIAN_POINT('Ctrl Pts',(-8.60384623578679,20.7362599762067,3.0611178465059));
#91058=CARTESIAN_POINT('Ctrl Pts',(-8.60126388452743,20.7357871614945,3.06944262469));
#91059=CARTESIAN_POINT('Ctrl Pts',(-8.60033110935933,20.7356139967324,3.07248465485085));
#91060=CARTESIAN_POINT('Ctrl Pts',(-8.59859655005347,20.7352874253576,3.07820804530214));
#91061=CARTESIAN_POINT('Ctrl Pts',(-8.59779253292075,20.7351341493173,3.08088867661833));
#91062=CARTESIAN_POINT('Ctrl Pts',(-8.59597308611298,20.7347829216217,3.08701863957445));
#91063=CARTESIAN_POINT('Ctrl Pts',(-8.59496267701831,20.7345846847845,3.09046941574758));
#91064=CARTESIAN_POINT('Ctrl Pts',(-8.59231364197492,20.7340564576069,3.09964167543322));
#91065=CARTESIAN_POINT('Ctrl Pts',(-8.59069720017489,20.733725249986,3.10536943026507));
#91066=CARTESIAN_POINT('Ctrl Pts',(-8.57936178000041,20.7313383910769,3.14649374141286));
#91067=CARTESIAN_POINT('Ctrl Pts',(-8.57094333208066,20.7292174935674,3.18223242306017));
#91068=CARTESIAN_POINT('Ctrl Pts',(-8.56183881258576,20.7264358883531,3.22863897155574));
#91069=CARTESIAN_POINT('Ctrl Pts',(-8.55991282253501,20.7258098789813,3.23905302617854));
#91070=CARTESIAN_POINT('Ctrl Pts',(-8.54307715898259,20.7199732890585,3.33595551281808));
#91071=CARTESIAN_POINT('Ctrl Pts',(-8.5358624844121,20.7146225471786,3.42360058363659));
#91072=CARTESIAN_POINT('Ctrl Pts',(-8.53713576986994,20.704889451098,3.5875411182641));
#91073=CARTESIAN_POINT('Ctrl Pts',(-8.54367389731852,20.700485462885,3.66356136209694));
#91074=CARTESIAN_POINT('Ctrl Pts',(-8.55794609596348,20.6956421867867,3.74988072813913));
#91075=CARTESIAN_POINT('Ctrl Pts',(-8.55991770669952,20.6950209413873,3.76100352300825));
#91076=CARTESIAN_POINT('Ctrl Pts',(-8.56313523722941,20.6940753987287,3.77800722371377));
#91077=CARTESIAN_POINT('Ctrl Pts',(-8.56428891014575,20.6937482079167,3.78390496808598));
#91078=CARTESIAN_POINT('Ctrl Pts',(-8.56645355672026,20.6931551140177,3.79462021795071));
#91079=CARTESIAN_POINT('Ctrl Pts',(-8.56745256653365,20.6928888371694,3.79944002664116));
#91080=CARTESIAN_POINT('Ctrl Pts',(-8.56968089652382,20.6923106748737,3.80992435984508));
#91081=CARTESIAN_POINT('Ctrl Pts',(-8.57091959411294,20.6919990915232,3.81558682074617));
#91082=CARTESIAN_POINT('Ctrl Pts',(-8.57439249473232,20.6911514813904,3.83102265485876));
#91083=CARTESIAN_POINT('Ctrl Pts',(-8.57669355626136,20.6906175833299,3.84078076678931));
#91084=CARTESIAN_POINT('Ctrl Pts',(-8.58889737310922,20.68791979675,3.89025221820011));
#91085=CARTESIAN_POINT('Ctrl Pts',(-8.60036311749825,20.6858062532142,3.92956304204687));
#91086=CARTESIAN_POINT('Ctrl Pts',(-8.61777109271493,20.6830520201436,3.98109953692637));
#91087=CARTESIAN_POINT('Ctrl Pts',(-8.62225551825075,20.6823748335203,3.9937951709245));
#91088=CARTESIAN_POINT('Ctrl Pts',(-8.67225012357295,20.6751493674886,4.12934643792311));
#91089=CARTESIAN_POINT('Ctrl Pts',(-8.73387908575262,20.6690544698455,4.24560600476089));
#91090=CARTESIAN_POINT('Ctrl Pts',(-8.82714833275273,20.6608812035185,4.37584471751621));
#91091=CARTESIAN_POINT('Ctrl Pts',(-8.84485643189269,20.6593613638933,4.39907069331645));
#91092=CARTESIAN_POINT('Ctrl Pts',(-8.86694345872554,20.6574822527619,4.42630966016178));
#91093=CARTESIAN_POINT('Ctrl Pts',(-8.87066816095837,20.6571658993751,4.43084709121206));
#91094=CARTESIAN_POINT('Ctrl Pts',(-8.87650062091459,20.6566711363923,4.4378656582528));
#91095=CARTESIAN_POINT('Ctrl Pts',(-8.87858957183165,20.6564940522166,4.44036242954924));
#91096=CARTESIAN_POINT('Ctrl Pts',(-8.88248287099121,20.6561641878848,4.44498438530276));
#91097=CARTESIAN_POINT('Ctrl Pts',(-8.8842849705884,20.6560115689693,4.44711139516433));
#91098=CARTESIAN_POINT('Ctrl Pts',(-8.888392346421,20.6556638732756,4.45193132131147));
#91099=CARTESIAN_POINT('Ctrl Pts',(-8.89070132633105,20.6554685291409,4.45462100754157));
#91100=CARTESIAN_POINT('Ctrl Pts',(-8.89777042974374,20.6548708900156,4.46279539122287));
#91101=CARTESIAN_POINT('Ctrl Pts',(-8.90256155219291,20.6544664137501,4.46825298333638));
#91102=CARTESIAN_POINT('Ctrl Pts',(-8.95554832763693,20.6500016622017,4.5277119891248));
#91103=CARTESIAN_POINT('Ctrl Pts',(-9.0076414177821,20.6456930284718,4.57809716581572));
#91104=CARTESIAN_POINT('Ctrl Pts',(-9.10628639507191,20.6379762913093,4.66027895616951));
#91105=CARTESIAN_POINT('Ctrl Pts',(-9.15135727437918,20.634589900873,4.69364026220984));
#91106=CARTESIAN_POINT('Ctrl Pts',(-9.26645628537517,20.6263961081862,4.76901410465484));
#91107=CARTESIAN_POINT('Ctrl Pts',(-9.3383047623977,20.6216650822126,4.80791667775934));
#91108=CARTESIAN_POINT('Ctrl Pts',(-9.42349604610924,20.6165156476931,4.84521595332661));
#91109=CARTESIAN_POINT('Ctrl Pts',(-9.4340149421953,20.6158871999292,4.84967540345245));
#91110=CARTESIAN_POINT('Ctrl Pts',(-9.45017003179515,20.6149330363354,4.85630221363035));
#91111=CARTESIAN_POINT('Ctrl Pts',(-9.45576904773861,20.6146043446668,4.8585585599309));
#91112=CARTESIAN_POINT('Ctrl Pts',(-9.46600310121169,20.6140071459131,4.86260935821819));
#91113=CARTESIAN_POINT('Ctrl Pts',(-9.47063360558834,20.6137382698475,4.8644149560642));
#91114=CARTESIAN_POINT('Ctrl Pts',(-9.48067947328153,20.6131577882854,4.86827335688927));
#91115=CARTESIAN_POINT('Ctrl Pts',(-9.48609801795175,20.6128464680661,4.87031767952266));
#91116=CARTESIAN_POINT('Ctrl Pts',(-9.5009089159111,20.6120002778584,4.87580536758673));
#91117=CARTESIAN_POINT('Ctrl Pts',(-9.51032476145337,20.6114675245657,4.87918471826834));
#91118=CARTESIAN_POINT('Ctrl Pts',(-9.55816219279598,20.6087861884441,4.89580192552832));
#91119=CARTESIAN_POINT('Ctrl Pts',(-9.59709031072738,20.6066871940358,4.90753253259805));
#91120=CARTESIAN_POINT('Ctrl Pts',(-9.64964362236174,20.6039393299958,4.92100947640338));
#91121=CARTESIAN_POINT('Ctrl Pts',(-9.66287522881874,20.603254541555,4.92420659445815));
#91122=CARTESIAN_POINT('Ctrl Pts',(-9.80407915310314,20.5960121157417,4.95624718476087));
#91123=CARTESIAN_POINT('Ctrl Pts',(-9.93531412083742,20.5899100079538,4.96794086071377));
#91124=CARTESIAN_POINT('Ctrl Pts',(-10.0955230028228,20.5817276127359,4.96067148000949));
#91125=CARTESIAN_POINT('Ctrl Pts',(-10.1246607228169,20.5802070729755,4.95847361732146));
#91126=CARTESIAN_POINT('Ctrl Pts',(-10.1595498760166,20.5783271782173,4.95478883641113));
#91127=CARTESIAN_POINT('Ctrl Pts',(-10.1653847818272,20.5780107830154,4.95413706131149));
#91128=CARTESIAN_POINT('Ctrl Pts',(-10.174448739469,20.5775159686562,4.95306933287671));
#91129=CARTESIAN_POINT('Ctrl Pts',(-10.1776806587125,20.5773388753632,4.95267767654967));
#91130=CARTESIAN_POINT('Ctrl Pts',(-10.1836776592562,20.577009002979,4.95193062488643));
#91131=CARTESIAN_POINT('Ctrl Pts',(-10.1864430465042,20.5768563851983,4.95157811088977));
#91132=CARTESIAN_POINT('Ctrl Pts',(-10.192722281388,20.5765087037073,4.95075943442791));
#91133=CARTESIAN_POINT('Ctrl Pts',(-10.1962354381214,20.576313372731,4.95028840807772));
#91134=CARTESIAN_POINT('Ctrl Pts',(-10.2053465379557,20.5758047631845,4.94903312643694));
#91135=CARTESIAN_POINT('Ctrl Pts',(-10.2109416565452,20.5754904321555,4.94822920063906));
#91136=CARTESIAN_POINT('Ctrl Pts',(-10.2468386063077,20.5734615595297,4.94285896966273));
#91137=CARTESIAN_POINT('Ctrl Pts',(-10.2769933771252,20.5717014538664,4.93737458772868));
#91138=CARTESIAN_POINT('Ctrl Pts',(-10.4488422888724,20.5614328355315,4.90051142392588));
#91139=CARTESIAN_POINT('Ctrl Pts',(-10.5854259286604,20.5524375547913,4.84914025540655));
#91140=CARTESIAN_POINT('Ctrl Pts',(-10.7465100432677,20.5418302924739,4.75940242629095));
#91141=CARTESIAN_POINT('Ctrl Pts',(-10.7800064589469,20.5396170533657,4.73893585454775));
#91142=CARTESIAN_POINT('Ctrl Pts',(-10.8206055595114,20.5369241247869,4.71182938158522));
#91143=CARTESIAN_POINT('Ctrl Pts',(-10.828516701172,20.5363988326869,4.70643442274162));
#91144=CARTESIAN_POINT('Ctrl Pts',(-10.8410011135454,20.5355688725945,4.69774002388942));
#91145=CARTESIAN_POINT('Ctrl Pts',(-10.8456091523379,20.5352623096942,4.69449118897344));
#91146=CARTESIAN_POINT('Ctrl Pts',(-10.8542551316687,20.5346866513018,4.68832035284328));
#91147=CARTESIAN_POINT('Ctrl Pts',(-10.8582971328054,20.5344173389875,4.68540420263811));
#91148=CARTESIAN_POINT('Ctrl Pts',(-10.8673684293265,20.5338124608504,4.67878888435012));
#91149=CARTESIAN_POINT('Ctrl Pts',(-10.8723891279557,20.5334773488524,4.67507805576253));
#91150=CARTESIAN_POINT('Ctrl Pts',(-10.8851720995358,20.5326231910664,4.66550299960771));
#91151=CARTESIAN_POINT('Ctrl Pts',(-10.8928999931483,20.5321059142689,4.65959324601958));
#91152=CARTESIAN_POINT('Ctrl Pts',(-10.9402818909444,20.5289277042012,4.62260434650245));
#91153=CARTESIAN_POINT('Ctrl Pts',(-10.9783700193084,20.5263455139822,4.58957025861108));
#91154=CARTESIAN_POINT('Ctrl Pts',(-11.1109874611881,20.5171190844727,4.4619768639741));
#91155=CARTESIAN_POINT('Ctrl Pts',(-11.194136314116,20.5109117001381,4.35657726243979));
#91156=CARTESIAN_POINT('Ctrl Pts',(-11.2767249500379,20.5025961367532,4.21601040281057));
#91157=CARTESIAN_POINT('Ctrl Pts',(-11.2908568794953,20.501065591186,4.19020705515303));
#91158=CARTESIAN_POINT('Ctrl Pts',(-11.3068697369986,20.4991744977396,4.15875514703171));
#91159=CARTESIAN_POINT('Ctrl Pts',(-11.3095069588764,20.4988575075804,4.15349703558725));
#91160=CARTESIAN_POINT('Ctrl Pts',(-11.313555429092,20.4983619622567,4.14530225429773));
#91161=CARTESIAN_POINT('Ctrl Pts',(-11.3149887210578,20.4981847392783,4.14237646887631));
#91162=CARTESIAN_POINT('Ctrl Pts',(-11.31763019005,20.4978547521786,4.13693853929639));
#91163=CARTESIAN_POINT('Ctrl Pts',(-11.3188409658966,20.4977021503595,4.1344277160232));
#91164=CARTESIAN_POINT('Ctrl Pts',(-11.3215736284869,20.4973546700867,4.12871928174073));
#91165=CARTESIAN_POINT('Ctrl Pts',(-11.3230910803971,20.4971595256465,4.1255196105431));
#91166=CARTESIAN_POINT('Ctrl Pts',(-11.326995846302,20.4966517170909,4.11720831331439));
#91167=CARTESIAN_POINT('Ctrl Pts',(-11.3293652196803,20.4963380058488,4.11208838310404));
#91168=CARTESIAN_POINT('Ctrl Pts',(-11.3443299348688,20.4943211291711,4.0792546713723));
#91169=CARTESIAN_POINT('Ctrl Pts',(-11.3560867670352,20.4925729981713,4.05116908989277));
#91170=CARTESIAN_POINT('Ctrl Pts',(-11.4034028041339,20.4848353898071,3.92743813517331));
#91171=CARTESIAN_POINT('Ctrl Pts',(-11.4297807441703,20.478584085687,3.82858823475624));
#91172=CARTESIAN_POINT('Ctrl Pts',(-11.4575117149778,20.4679876099714,3.65260042666487));
#91173=CARTESIAN_POINT('Ctrl Pts',(-11.4634769354391,20.4635722569285,3.57658548729573));
#91174=CARTESIAN_POINT('Ctrl Pts',(-11.4634999778476,20.4593334002854,3.50029468859335));
#91175=CARTESIAN_POINT('Ctrl Pts',(-11.4635,20.459325214305,3.50014734427607));
#91176=CARTESIAN_POINT('Ctrl Pts',(-11.4635,20.459317028952,3.5000000000001));
#91177=CARTESIAN_POINT('Ctrl Pts',(-11.4635,20.390600218991,3.49999999999975));
#91178=CARTESIAN_POINT('Ctrl Pts',(-11.4635,20.390607428758,3.50013812385499));
#91179=CARTESIAN_POINT('Ctrl Pts',(-11.4634999805033,20.3906146379989,3.50027624782956));
#91180=CARTESIAN_POINT('Ctrl Pts',(-11.4634741169183,20.3953818886303,3.59162099111268));
#91181=CARTESIAN_POINT('Ctrl Pts',(-11.4549227392133,20.3998676312033,3.68262807373579));
#91182=CARTESIAN_POINT('Ctrl Pts',(-11.4187105930484,20.4093415908848,3.87388767578039));
#91183=CARTESIAN_POINT('Ctrl Pts',(-11.3887498446853,20.4142928448941,3.97318077703706));
#91184=CARTESIAN_POINT('Ctrl Pts',(-11.3444555861568,20.4203180210045,4.07825967081919));
#91185=CARTESIAN_POINT('Ctrl Pts',(-11.3402234602025,20.4208846136783,4.08800181442585));
#91186=CARTESIAN_POINT('Ctrl Pts',(-11.3341467485738,20.4216868979981,4.10158360618573));
#91187=CARTESIAN_POINT('Ctrl Pts',(-11.3323907713043,20.4219174723696,4.10546280941432));
#91188=CARTESIAN_POINT('Ctrl Pts',(-11.3295298988873,20.4222911999234,4.11171016563223));
#91189=CARTESIAN_POINT('Ctrl Pts',(-11.3284355327981,20.4224337156073,4.11408314889006));
#91190=CARTESIAN_POINT('Ctrl Pts',(-11.3261174822221,20.4227346799665,4.11907432974894));
#91191=CARTESIAN_POINT('Ctrl Pts',(-11.3248923929248,20.4228932169853,4.12169184420796));
#91192=CARTESIAN_POINT('Ctrl Pts',(-11.3218682669134,20.4232832599149,4.12810362848368));
#91193=CARTESIAN_POINT('Ctrl Pts',(-11.3200606450264,20.423515285491,4.13189380100151));
#91194=CARTESIAN_POINT('Ctrl Pts',(-11.3134381352104,20.4243611882083,4.1456272667948));
#91195=CARTESIAN_POINT('Ctrl Pts',(-11.3085271303932,20.4249806170377,4.15552348290582));
#91196=CARTESIAN_POINT('Ctrl Pts',(-11.2760832204036,20.4290186013033,4.21908397511318));
#91197=CARTESIAN_POINT('Ctrl Pts',(-11.245369281037,20.4325946070711,4.27105394129202));
#91198=CARTESIAN_POINT('Ctrl Pts',(-11.1793753163977,20.4396507046261,4.36844336828949));
#91199=CARTESIAN_POINT('Ctrl Pts',(-11.1444473983025,20.4431207221245,4.41398050987996));
#91200=CARTESIAN_POINT('Ctrl Pts',(-11.0506532432454,20.4516826729866,4.52243007014784));
#91201=CARTESIAN_POINT('Ctrl Pts',(-10.9887326843839,20.4566917543782,4.58242651751467));
#91202=CARTESIAN_POINT('Ctrl Pts',(-10.9135597045607,20.4620560648074,4.64339666730071));
#91203=CARTESIAN_POINT('Ctrl Pts',(-10.9051559833319,20.4626468172799,4.65006083623498));
#91204=CARTESIAN_POINT('Ctrl Pts',(-10.891562833795,20.4635883294865,4.66059893161671));
#91205=CARTESIAN_POINT('Ctrl Pts',(-10.8864197407251,20.4639413974254,4.66453175646391));
#91206=CARTESIAN_POINT('Ctrl Pts',(-10.8772377663721,20.4645661957537,4.67145696243838));
#91207=CARTESIAN_POINT('Ctrl Pts',(-10.8732092729814,20.4648384511188,4.67446289002655));
#91208=CARTESIAN_POINT('Ctrl Pts',(-10.8647763577664,20.4654045215651,4.68068787611257));
#91209=CARTESIAN_POINT('Ctrl Pts',(-10.860369256452,20.4656981895318,4.68390318582672));
#91210=CARTESIAN_POINT('Ctrl Pts',(-10.8488536213085,20.4664599885719,4.69220643994294));
#91211=CARTESIAN_POINT('Ctrl Pts',(-10.8417172389066,20.466926632797,4.69725551159592));
#91212=CARTESIAN_POINT('Ctrl Pts',(-10.8101027530645,20.4689705427825,4.71920072681514));
#91213=CARTESIAN_POINT('Ctrl Pts',(-10.7851572419888,20.4705221013258,4.73541294661557));
#91214=CARTESIAN_POINT('Ctrl Pts',(-10.7163672564936,20.4746552512933,4.77719404635434));
#91215=CARTESIAN_POINT('Ctrl Pts',(-10.6716583565793,20.4771869779718,4.80126179547164));
#91216=CARTESIAN_POINT('Ctrl Pts',(-10.5646561713394,20.4830070221092,4.85187603736339));
#91217=CARTESIAN_POINT('Ctrl Pts',(-10.501595306771,20.4862581184921,4.87652004682003));
#91218=CARTESIAN_POINT('Ctrl Pts',(-10.3734075435223,20.4928459924698,4.91663227259763));
#91219=CARTESIAN_POINT('Ctrl Pts',(-10.3084779367331,20.4961747805824,4.93217300959891));
#91220=CARTESIAN_POINT('Ctrl Pts',(-10.2355561858,20.5001194633601,4.94443703883215));
#91221=CARTESIAN_POINT('Ctrl Pts',(-10.2283799741315,20.5005098602532,4.94558903526506));
#91222=CARTESIAN_POINT('Ctrl Pts',(-10.2176896406082,20.5010950938128,4.94722356589499));
#91223=CARTESIAN_POINT('Ctrl Pts',(-10.2141817533489,20.5012877158291,4.94774687197062));
#91224=CARTESIAN_POINT('Ctrl Pts',(-10.2079122320455,20.5016330823566,4.9486588733908));
#91225=CARTESIAN_POINT('Ctrl Pts',(-10.2051513554318,20.5017855526473,4.94905243138268));
#91226=CARTESIAN_POINT('Ctrl Pts',(-10.1991644832941,20.5021170224225,4.94988839604609));
#91227=CARTESIAN_POINT('Ctrl Pts',(-10.1959381761234,20.50229617508,4.95032792261136));
#91228=CARTESIAN_POINT('Ctrl Pts',(-10.1868909573308,20.5027999731771,4.95152970492334));
#91229=CARTESIAN_POINT('Ctrl Pts',(-10.1810669544135,20.503125928615,4.95226769909673));
#91230=CARTESIAN_POINT('Ctrl Pts',(-10.1462682291114,20.505082690734,4.95646467718328));
#91231=CARTESIAN_POINT('Ctrl Pts',(-10.1172015960127,20.50675492819,4.95909125854797));
#91232=CARTESIAN_POINT('Ctrl Pts',(-9.95760060590718,20.5160741420751,4.96871399136899));
#91233=CARTESIAN_POINT('Ctrl Pts',(-9.82665405767403,20.524156189074,4.95906653258119));
#91234=CARTESIAN_POINT('Ctrl Pts',(-9.68508252089366,20.5326020000613,4.92928423180258));
#91235=CARTESIAN_POINT('Ctrl Pts',(-9.67148740649836,20.5334108003078,4.92622085454221));
#91236=CARTESIAN_POINT('Ctrl Pts',(-9.61829535026342,20.5365654978466,4.91343416850989));
#91237=CARTESIAN_POINT('Ctrl Pts',(-9.57906601780826,20.5388699583677,4.9022516289793));
#91238=CARTESIAN_POINT('Ctrl Pts',(-9.5308430606685,20.5416752396865,4.88629878870084));
#91239=CARTESIAN_POINT('Ctrl Pts',(-9.52136650552922,20.5422252158763,4.88305551235554));
#91240=CARTESIAN_POINT('Ctrl Pts',(-9.50646033397564,20.5430883796072,4.87778243317299));
#91241=CARTESIAN_POINT('Ctrl Pts',(-9.50100832000851,20.5434036778963,4.87581726248366));
#91242=CARTESIAN_POINT('Ctrl Pts',(-9.49090108904287,20.5439874763804,4.872106142382));
#91243=CARTESIAN_POINT('Ctrl Pts',(-9.48624283371902,20.5442562544251,4.87036876133388));
#91244=CARTESIAN_POINT('Ctrl Pts',(-9.47594870545084,20.5448496231285,4.86646951150331));
#91245=CARTESIAN_POINT('Ctrl Pts',(-9.470317154656,20.5451738368501,4.86429643773945));
#91246=CARTESIAN_POINT('Ctrl Pts',(-9.45407307548177,20.5461079710779,4.85791251409775));
#91247=CARTESIAN_POINT('Ctrl Pts',(-9.44349603986617,20.5467149063497,4.853612187833));
#91248=CARTESIAN_POINT('Ctrl Pts',(-9.35820410394262,20.5516007166158,4.8177661434215));
#91249=CARTESIAN_POINT('Ctrl Pts',(-9.28617553206794,20.5556628084855,4.78018218264892));
#91250=CARTESIAN_POINT('Ctrl Pts',(-9.14259423546236,20.563991602126,4.68935691419776));
#91251=CARTESIAN_POINT('Ctrl Pts',(-9.07204243519726,20.5682245567197,4.63516859086689));
#91252=CARTESIAN_POINT('Ctrl Pts',(-8.97681467810198,20.5747301381891,4.54718435638437));
#91253=CARTESIAN_POINT('Ctrl Pts',(-8.94796796888357,20.5768273590472,4.51820003992412));
#91254=CARTESIAN_POINT('Ctrl Pts',(-8.91624730916446,20.5793374981187,4.48353938825117));
#91255=CARTESIAN_POINT('Ctrl Pts',(-8.91214838315707,20.5796660108317,4.47900382035431));
#91256=CARTESIAN_POINT('Ctrl Pts',(-8.90565199038369,20.5801935959356,4.47172422028032));
#91257=CARTESIAN_POINT('Ctrl Pts',(-8.90323610286555,20.5803913472762,4.46899663559176));
#91258=CARTESIAN_POINT('Ctrl Pts',(-8.89897815009931,20.5807426975999,4.46415299972927));
#91259=CARTESIAN_POINT('Ctrl Pts',(-8.8971319526628,20.5808959882856,4.46204063891472));
#91260=CARTESIAN_POINT('Ctrl Pts',(-8.893222217744,20.5812226597567,4.45754119839523));
#91261=CARTESIAN_POINT('Ctrl Pts',(-8.89116035575976,20.5813961513067,4.45515278824485));
#91262=CARTESIAN_POINT('Ctrl Pts',(-8.88558344190604,20.5818686783726,4.44865023425726));
#91263=CARTESIAN_POINT('Ctrl Pts',(-8.88208349447449,20.5821687795416,4.44452327483412));
#91264=CARTESIAN_POINT('Ctrl Pts',(-8.86429567523937,20.5837118523578,4.42331141813337));
#91265=CARTESIAN_POINT('Ctrl Pts',(-8.85037698899982,20.5849788071226,4.40592224239126));
#91266=CARTESIAN_POINT('Ctrl Pts',(-8.80992673116005,20.5888268944151,4.35295216074447));
#91267=CARTESIAN_POINT('Ctrl Pts',(-8.78461201156551,20.591461509597,4.31647616686375));
#91268=CARTESIAN_POINT('Ctrl Pts',(-8.72302006781919,20.5983965824194,4.21850232022926));
#91269=CARTESIAN_POINT('Ctrl Pts',(-8.68951184208899,20.6027228860264,4.15539663854157));
#91270=CARTESIAN_POINT('Ctrl Pts',(-8.63068859801709,20.6113792753365,4.02189406395155));
#91271=CARTESIAN_POINT('Ctrl Pts',(-8.60588773625279,20.6156872215042,3.95148729461855));
#91272=CARTESIAN_POINT('Ctrl Pts',(-8.58381486465399,20.6204035137354,3.86927462819662));
#91273=CARTESIAN_POINT('Ctrl Pts',(-8.58118338850067,20.6209858988318,3.85903136324673));
#91274=CARTESIAN_POINT('Ctrl Pts',(-8.57713071825249,20.6219166910244,3.8425151199075));
#91275=CARTESIAN_POINT('Ctrl Pts',(-8.57563947342048,20.6222673237693,3.83625985855487));
#91276=CARTESIAN_POINT('Ctrl Pts',(-8.5730575804616,20.6228893330799,3.82510426156666));
#91277=CARTESIAN_POINT('Ctrl Pts',(-8.57195083346964,20.6231612186845,3.82020778942869));
#91278=CARTESIAN_POINT('Ctrl Pts',(-8.56968944184591,20.6237280330903,3.8099579764735));
#91279=CARTESIAN_POINT('Ctrl Pts',(-8.56853960607608,20.6240228054133,3.80460364688229));
#91280=CARTESIAN_POINT('Ctrl Pts',(-8.56561291148635,20.6247907725627,3.79059254065567));
#91281=CARTESIAN_POINT('Ctrl Pts',(-8.56388434474194,20.6252624345873,3.7819258301705));
#91282=CARTESIAN_POINT('Ctrl Pts',(-8.55650421227616,20.6273612969774,3.74309274992734));
#91283=CARTESIAN_POINT('Ctrl Pts',(-8.55172368249318,20.6289610086887,3.71276761492174));
#91284=CARTESIAN_POINT('Ctrl Pts',(-8.54128046593888,20.6332608611351,3.62958874739014));
#91285=CARTESIAN_POINT('Ctrl Pts',(-8.53753699533784,20.6359056589259,3.57654061958454));
#91286=CARTESIAN_POINT('Ctrl Pts',(-8.53505787753058,20.6435130477447,3.42153402450689));
#91287=CARTESIAN_POINT('Ctrl Pts',(-8.54407055202662,20.6483421366308,3.31978159020635));
#91288=CARTESIAN_POINT('Ctrl Pts',(-8.56942674510398,20.6550802002476,3.18979546212704));
#91289=CARTESIAN_POINT('Ctrl Pts',(-8.57621761619831,20.6566671421376,3.15998505918496));
#91290=CARTESIAN_POINT('Ctrl Pts',(-8.5853630790576,20.6586050550509,3.1249446011584));
#91291=CARTESIAN_POINT('Ctrl Pts',(-8.58682148787257,20.6589090358855,3.1194863194484));
#91292=CARTESIAN_POINT('Ctrl Pts',(-8.58924618989976,20.6594065793754,3.11061779702304));
#91293=CARTESIAN_POINT('Ctrl Pts',(-8.59019334570668,20.6595990764697,3.10720232984749));
#91294=CARTESIAN_POINT('Ctrl Pts',(-8.59190785862227,20.6599443087391,3.10110584352167));
#91295=CARTESIAN_POINT('Ctrl Pts',(-8.59267048041607,20.6600967705797,3.09842354422595));
#91296=CARTESIAN_POINT('Ctrl Pts',(-8.59434067521794,20.6604283270342,3.09261231465354));
#91297=CARTESIAN_POINT('Ctrl Pts',(-8.59525101833033,20.6606075755217,3.08948427363875));
#91298=CARTESIAN_POINT('Ctrl Pts',(-8.5978332724912,20.6611119079906,3.08072052891734));
#91299=CARTESIAN_POINT('Ctrl Pts',(-8.59952868664254,20.6614383063382,3.07509188679085));
#91300=CARTESIAN_POINT('Ctrl Pts',(-8.60988310904659,20.6634033344892,3.04145127872989));
#91301=CARTESIAN_POINT('Ctrl Pts',(-8.61934786459483,20.6650837938046,3.01369624477323));
#91302=CARTESIAN_POINT('Ctrl Pts',(-8.67612115789244,20.6745116480617,2.86226201702805));
#91303=CARTESIAN_POINT('Ctrl Pts',(-8.73921435087696,20.6827019219361,2.74515532452553));
#91304=CARTESIAN_POINT('Ctrl Pts',(-8.82807916098557,20.6914976447893,2.62320204860877));
#91305=CARTESIAN_POINT('Ctrl Pts',(-8.83923344717261,20.6925653345078,2.6084877180643));
#91306=CARTESIAN_POINT('Ctrl Pts',(-8.87249719250457,20.6956448575536,2.56629044576023));
#91307=CARTESIAN_POINT('Ctrl Pts',(-8.89532612903876,20.6976301705083,2.53938975045291));
#91308=CARTESIAN_POINT('Ctrl Pts',(-8.92561928826648,20.7001093439909,2.50620340853799));
#91309=CARTESIAN_POINT('Ctrl Pts',(-8.93220292176351,20.7006393978413,2.49913288347314));
#91310=CARTESIAN_POINT('Ctrl Pts',(-8.94275277289437,20.7014751867949,2.4880254129426));
#91311=CARTESIAN_POINT('Ctrl Pts',(-8.94667314485928,20.7017828616776,2.48394547313304));
#91312=CARTESIAN_POINT('Ctrl Pts',(-8.95374333634529,20.7023325946614,2.47667240868098));
#91313=CARTESIAN_POINT('Ctrl Pts',(-8.95688434492712,20.7025750277356,2.47347084982523));
#91314=CARTESIAN_POINT('Ctrl Pts',(-8.96425265302893,20.7031396020369,2.46602924113074));
#91315=CARTESIAN_POINT('Ctrl Pts',(-8.96849137052845,20.703461239446,2.46180057516005));
#91316=CARTESIAN_POINT('Ctrl Pts',(-8.98072226529886,20.7043804699136,2.44974753450614));
#91317=CARTESIAN_POINT('Ctrl Pts',(-8.98877844041387,20.7049752258136,2.44198851215169));
#91318=CARTESIAN_POINT('Ctrl Pts',(-9.04941482937833,20.7093747666153,2.38491405071674));
#91319=CARTESIAN_POINT('Ctrl Pts',(-9.10548822072992,20.7130112826272,2.33944874008731));
#91320=CARTESIAN_POINT('Ctrl Pts',(-9.23322487295998,20.720678567297,2.25065831475121));
#91321=CARTESIAN_POINT('Ctrl Pts',(-9.30570694708112,20.7246657501089,2.20897122993276));
#91322=CARTESIAN_POINT('Ctrl Pts',(-9.43116367535788,20.7315127742817,2.15045215543675));
#91323=CARTESIAN_POINT('Ctrl Pts',(-9.4822472535904,20.7342903161352,2.1300419667088));
#91324=CARTESIAN_POINT('Ctrl Pts',(-9.54114592350192,20.7376055436466,2.11027465027035));
#91325=CARTESIAN_POINT('Ctrl Pts',(-9.54795667965244,20.7379905752628,2.10804438161724));
#91326=CARTESIAN_POINT('Ctrl Pts',(-9.55814282197562,20.738569296075,2.10479144179286));
#91327=CARTESIAN_POINT('Ctrl Pts',(-9.56150607290425,20.7387608421014,2.10373077021889));
#91328=CARTESIAN_POINT('Ctrl Pts',(-9.56753440712326,20.7391050562114,2.10185353757106));
#91329=CARTESIAN_POINT('Ctrl Pts',(-9.57019802028452,20.7392574577136,2.10103242443278));
#91330=CARTESIAN_POINT('Ctrl Pts',(-9.5759926749828,20.7395896920806,2.09926421535745));
#91331=CARTESIAN_POINT('Ctrl Pts',(-9.57912450888576,20.7397696842417,2.09832001848));
#91332=CARTESIAN_POINT('Ctrl Pts',(-9.58795197318773,20.7402781701645,2.09569093401207));
#91333=CARTESIAN_POINT('Ctrl Pts',(-9.59365466579339,20.7406080124679,2.09403022930265));
#91334=CARTESIAN_POINT('Ctrl Pts',(-9.62863724511608,20.7426389753466,2.08407341532358));
#91335=CARTESIAN_POINT('Ctrl Pts',(-9.65815800719362,20.7443851764392,2.0766580957713));
#91336=CARTESIAN_POINT('Ctrl Pts',(-9.8326517368111,20.7548110116127,2.03856834994767));
#91337=CARTESIAN_POINT('Ctrl Pts',(-9.98138562376467,20.7640040227649,2.02913157191114));
#91338=CARTESIAN_POINT('Ctrl Pts',(-10.1654734906761,20.7746119914218,2.04542457667391));
#91339=CARTESIAN_POINT('Ctrl Pts',(-10.2017900367449,20.7766738084385,2.05001646427287));
#91340=CARTESIAN_POINT('Ctrl Pts',(-10.2474402060859,20.7792271579078,2.05753713884985));
#91341=CARTESIAN_POINT('Ctrl Pts',(-10.2569660585743,20.7797578687801,2.05920361867682));
#91342=CARTESIAN_POINT('Ctrl Pts',(-10.2720951432256,20.7805975396543,2.06200516211635));
#91343=CARTESIAN_POINT('Ctrl Pts',(-10.2777093373958,20.7809084241285,2.06307883098469));
#91344=CARTESIAN_POINT('Ctrl Pts',(-10.2882001191804,20.7814880679398,2.06514888820618));
#91345=CARTESIAN_POINT('Ctrl Pts',(-10.2930781787321,20.7817570743469,2.0661373135095));
#91346=CARTESIAN_POINT('Ctrl Pts',(-10.3039590643816,20.7823559902763,2.06839991860104));
#91347=CARTESIAN_POINT('Ctrl Pts',(-10.3099591297369,20.782685485763,2.06968701140548));
#91348=CARTESIAN_POINT('Ctrl Pts',(-10.3275710386278,20.7836505010516,2.07358102539579));
#91349=CARTESIAN_POINT('Ctrl Pts',(-10.339159539298,20.7842827170908,2.07629192090537));
#91350=CARTESIAN_POINT('Ctrl Pts',(-10.4588240031204,20.7907856780798,2.10582903841884));
#91351=CARTESIAN_POINT('Ctrl Pts',(-10.5635364984254,20.7962222471104,2.14476489767079));
#91352=CARTESIAN_POINT('Ctrl Pts',(-10.7449222954545,20.8061132140168,2.23690800791843));
#91353=CARTESIAN_POINT('Ctrl Pts',(-10.8228865963402,20.8105666921341,2.2862602645948));
#91354=CARTESIAN_POINT('Ctrl Pts',(-10.9044833827044,20.8160115108662,2.3494063526567));
#91355=CARTESIAN_POINT('Ctrl Pts',(-10.9132003774872,20.8166042377049,2.35631254854431));
#91356=CARTESIAN_POINT('Ctrl Pts',(-10.9252092026642,20.8174376134264,2.36605157696715));
#91357=CARTESIAN_POINT('Ctrl Pts',(-10.9285686244638,20.8176726070618,2.36880090015919));
#91358=CARTESIAN_POINT('Ctrl Pts',(-10.9339426610799,20.8180516113993,2.37323903759915));
#91359=CARTESIAN_POINT('Ctrl Pts',(-10.9359650706279,20.8181949497142,2.3749184265511));
#91360=CARTESIAN_POINT('Ctrl Pts',(-10.9400062855384,20.8184828163387,2.37829264902925));
#91361=CARTESIAN_POINT('Ctrl Pts',(-10.9420250465688,20.8186273472463,2.37998749589648));
#91362=CARTESIAN_POINT('Ctrl Pts',(-10.9469971891729,20.8189851032353,2.38418480086848));
#91363=CARTESIAN_POINT('Ctrl Pts',(-10.9499452310026,20.8191987802106,2.38669353172425));
#91364=CARTESIAN_POINT('Ctrl Pts',(-10.9596720352538,20.8199088649679,2.39503763041493));
#91365=CARTESIAN_POINT('Ctrl Pts',(-10.9664071176315,20.8204087596367,2.4009233291967));
#91366=CARTESIAN_POINT('Ctrl Pts',(-10.9825368114719,20.8216250210738,2.41528173979945));
#91367=CARTESIAN_POINT('Ctrl Pts',(-10.991876214188,20.8223451929125,2.42381514348535));
#91368=CARTESIAN_POINT('Ctrl Pts',(-11.0265092178773,20.8250723718442,2.45629307432812));
#91369=CARTESIAN_POINT('Ctrl Pts',(-11.0510549080209,20.8271206907293,2.48101588986008));
#91370=CARTESIAN_POINT('Ctrl Pts',(-11.1684397018811,20.8374108297976,2.60800534651693));
#91371=CARTESIAN_POINT('Ctrl Pts',(-11.2473802239159,20.8458690277799,2.72220760261087));
#91372=CARTESIAN_POINT('Ctrl Pts',(-11.3210755620005,20.855218854551,2.86967875371017));
#91373=CARTESIAN_POINT('Ctrl Pts',(-11.3323584045408,20.8567119818949,2.89389214853392));
#91374=CARTESIAN_POINT('Ctrl Pts',(-11.3464424278588,20.8586633473753,2.92641368162881));
#91375=CARTESIAN_POINT('Ctrl Pts',(-11.3498403391074,20.8591416409647,2.93445642102651));
#91376=CARTESIAN_POINT('Ctrl Pts',(-11.3552432092668,20.859914714751,2.94757097524141));
#91377=CARTESIAN_POINT('Ctrl Pts',(-11.3572921162346,20.860210965593,2.95262435568503));
#91378=CARTESIAN_POINT('Ctrl Pts',(-11.3611755624191,20.8607785138527,2.96235828891635));
#91379=CARTESIAN_POINT('Ctrl Pts',(-11.3630143189916,20.8610499491327,2.96703706665562));
#91380=CARTESIAN_POINT('Ctrl Pts',(-11.3672077934773,20.8616753694391,2.97787115544829));
#91381=CARTESIAN_POINT('Ctrl Pts',(-11.3695451253283,20.8620287726436,2.98403310911999));
#91382=CARTESIAN_POINT('Ctrl Pts',(-11.3767921804142,20.8631401235808,3.00353490312667));
#91383=CARTESIAN_POINT('Ctrl Pts',(-11.3815493058924,20.8638930363262,3.01693081798758));
#91384=CARTESIAN_POINT('Ctrl Pts',(-11.4040587939898,20.8675785694212,3.08337088947177));
#91385=CARTESIAN_POINT('Ctrl Pts',(-11.4189560792206,20.8704175947892,3.13733565928366));
#91386=CARTESIAN_POINT('Ctrl Pts',(-11.4525167466992,20.8783406135788,3.29324514767279));
#91387=CARTESIAN_POINT('Ctrl Pts',(-11.4634999999976,20.8832405801403,3.39647993126226));
#91388=CARTESIAN_POINT('Ctrl Pts',(-11.4635,20.8884018418444,3.4999999999667));
#91389=CARTESIAN_POINT('Origin',(-10.,13.2,3.5));
#91390=CARTESIAN_POINT('',(-11.4635,21.4611504451332,3.50000000000115));
#91391=CARTESIAN_POINT('',(-11.4635,21.3891087006547,3.49999999989906));
#91392=CARTESIAN_POINT('',(-11.4635,13.2,3.5));
#91393=CARTESIAN_POINT('',(-11.4634996681794,20.9614426132404,3.50098551447728));
#91394=CARTESIAN_POINT('Ctrl Pts',(-11.4635,21.4611504451332,3.50000000000115));
#91395=CARTESIAN_POINT('Ctrl Pts',(-11.4635,21.4611301311275,3.49958402536292));
#91396=CARTESIAN_POINT('Ctrl Pts',(-11.463499822648,21.4611098150822,3.49916804479857));
#91397=CARTESIAN_POINT('Ctrl Pts',(-11.4634800403263,21.45997668514,3.47596872626212));
#91398=CARTESIAN_POINT('Ctrl Pts',(-11.4629285888914,21.4588587293667,3.453189353351));
#91399=CARTESIAN_POINT('Ctrl Pts',(-11.459355687562,21.4551326182292,3.37811065493419));
#91400=CARTESIAN_POINT('Ctrl Pts',(-11.4540587307172,21.4524786967789,3.32596506512405));
#91401=CARTESIAN_POINT('Ctrl Pts',(-11.4448804648682,21.4493035845956,3.26718370650074));
#91402=CARTESIAN_POINT('Ctrl Pts',(-11.443730267838,21.448920873213,3.2601544374043));
#91403=CARTESIAN_POINT('Ctrl Pts',(-11.4419355603834,21.4483450095766,3.24966730221917));
#91404=CARTESIAN_POINT('Ctrl Pts',(-11.4413298034892,21.4481539702018,3.24620280355885));
#91405=CARTESIAN_POINT('Ctrl Pts',(-11.4402218649907,21.4478103444058,3.23999809515392));
#91406=CARTESIAN_POINT('Ctrl Pts',(-11.4397243422751,21.4476580212517,3.2372571047446));
#91407=CARTESIAN_POINT('Ctrl Pts',(-11.438624679679,21.4473255805546,3.23129567464895));
#91408=CARTESIAN_POINT('Ctrl Pts',(-11.4380195591897,21.4471453012809,3.22807587382141));
#91409=CARTESIAN_POINT('Ctrl Pts',(-11.4362819450198,21.4466350371026,3.21899818148236));
#91410=CARTESIAN_POINT('Ctrl Pts',(-11.435124446602,21.4463036883464,3.21314521467631));
#91411=CARTESIAN_POINT('Ctrl Pts',(-11.4277385215497,21.4442414116689,3.17696177174206));
#91412=CARTESIAN_POINT('Ctrl Pts',(-11.4205850262114,21.4424638086071,3.14683022659087));
#91413=CARTESIAN_POINT('Ctrl Pts',(-11.3711499059412,21.4314313603784,2.96453989002991));
#91414=CARTESIAN_POINT('Ctrl Pts',(-11.3054224331949,21.4216221630225,2.81980899491061));
#91415=CARTESIAN_POINT('Ctrl Pts',(-11.2022685113024,21.4110553934255,2.66503399632583));
#91416=CARTESIAN_POINT('Ctrl Pts',(-11.1860571767917,21.4094867014405,2.64216182996881));
#91417=CARTESIAN_POINT('Ctrl Pts',(-11.1638515592825,21.4074531325712,2.61266645594961));
#91418=CARTESIAN_POINT('Ctrl Pts',(-11.1584403306633,21.4069660172414,2.60561346408241));
#91419=CARTESIAN_POINT('Ctrl Pts',(-11.1495858000748,21.4061823146069,2.59428766080702));
#91420=CARTESIAN_POINT('Ctrl Pts',(-11.1461821974204,21.4058841798824,2.58998421741162));
#91421=CARTESIAN_POINT('Ctrl Pts',(-11.1396215634412,21.40531538727,2.58178429023885));
#91422=CARTESIAN_POINT('Ctrl Pts',(-11.1364685535956,21.4050445758402,2.57788470077436));
#91423=CARTESIAN_POINT('Ctrl Pts',(-11.1291754280711,21.4044239488897,2.56895891380048));
#91424=CARTESIAN_POINT('Ctrl Pts',(-11.1250216691297,21.4040746863901,2.56394396673649));
#91425=CARTESIAN_POINT('Ctrl Pts',(-11.111958169909,21.4029891611793,2.54838461530554));
#91426=CARTESIAN_POINT('Ctrl Pts',(-11.1029324795768,21.4022576021341,2.53793826875781));
#91427=CARTESIAN_POINT('Ctrl Pts',(-11.0211719566985,21.3957878290582,2.44597166437074));
#91428=CARTESIAN_POINT('Ctrl Pts',(-10.939669528071,21.3904603760823,2.37270579807588));
#91429=CARTESIAN_POINT('Ctrl Pts',(-10.7888294885497,21.3814477690091,2.26493966676558));
#91430=CARTESIAN_POINT('Ctrl Pts',(-10.7235426742755,21.3777575031556,2.22559421903429));
#91431=CARTESIAN_POINT('Ctrl Pts',(-10.6346165643394,21.3726380238458,2.18104602627489));
#91432=CARTESIAN_POINT('Ctrl Pts',(-10.6134877345626,21.3714147880386,2.17108674239387));
#91433=CARTESIAN_POINT('Ctrl Pts',(-10.5869246875783,21.3698577586546,2.15933446708396));
#91434=CARTESIAN_POINT('Ctrl Pts',(-10.5817051795276,21.3695509025321,2.1570615270948));
#91435=CARTESIAN_POINT('Ctrl Pts',(-10.573484749764,21.3690660008817,2.15353869021256));
#91436=CARTESIAN_POINT('Ctrl Pts',(-10.5704926419175,21.3688891687441,2.15226821582951));
#91437=CARTESIAN_POINT('Ctrl Pts',(-10.5649261633307,21.3685595263574,2.1499265001712));
#91438=CARTESIAN_POINT('Ctrl Pts',(-10.5623529504834,21.3684068754176,2.14885264177258));
#91439=CARTESIAN_POINT('Ctrl Pts',(-10.5564953513437,21.3680587841313,2.14642776836013));
#91440=CARTESIAN_POINT('Ctrl Pts',(-10.5532091197796,21.3678630739183,2.14508135610378));
#91441=CARTESIAN_POINT('Ctrl Pts',(-10.5431573578577,21.367263225692,2.14100568209325));
#91442=CARTESIAN_POINT('Ctrl Pts',(-10.5363763988116,21.3668568833374,2.1383150783701));
#91443=CARTESIAN_POINT('Ctrl Pts',(-10.453761427734,21.361888389703,2.10624728187323));
#91444=CARTESIAN_POINT('Ctrl Pts',(-10.3756334230676,21.3570148277561,2.08319269281859));
#91445=CARTESIAN_POINT('Ctrl Pts',(-10.177714277955,21.3448484532469,2.04231712190961));
#91446=CARTESIAN_POINT('Ctrl Pts',(-10.056831455609,21.3376126476002,2.03262071543825));
#91447=CARTESIAN_POINT('Ctrl Pts',(-9.91988968774703,21.329954948038,2.03860393723804));
#91448=CARTESIAN_POINT('Ctrl Pts',(-9.90367376392719,21.3290557290481,2.0395831415249));
#91449=CARTESIAN_POINT('Ctrl Pts',(-9.88106183320187,21.3278120032122,2.04132684883454));
#91450=CARTESIAN_POINT('Ctrl Pts',(-9.87464990082434,21.3274604687251,2.04186385959931));
#91451=CARTESIAN_POINT('Ctrl Pts',(-9.8635574831246,21.3268542547662,2.04286657774157));
#91452=CARTESIAN_POINT('Ctrl Pts',(-9.85887535159832,21.3265989661006,2.04331259186927));
#91453=CARTESIAN_POINT('Ctrl Pts',(-9.84915162785144,21.3260700003851,2.04428618422934));
#91454=CARTESIAN_POINT('Ctrl Pts',(-9.84411045747146,21.3257964404922,2.04481740107011));
#91455=CARTESIAN_POINT('Ctrl Pts',(-9.83224791779711,21.3251542701545,2.04612977593453));
#91456=CARTESIAN_POINT('Ctrl Pts',(-9.8254290512644,21.3247863459649,2.04693276977572));
#91457=CARTESIAN_POINT('Ctrl Pts',(-9.80299025317935,21.3235794384284,2.0497354093413));
#91458=CARTESIAN_POINT('Ctrl Pts',(-9.78739664094299,21.3227468274616,2.05193920696695));
#91459=CARTESIAN_POINT('Ctrl Pts',(-9.70464902013932,21.3183570517546,2.064999197121));
#91460=CARTESIAN_POINT('Ctrl Pts',(-9.63827461380241,21.3149413213872,2.08027621668749));
#91461=CARTESIAN_POINT('Ctrl Pts',(-9.48633342006634,21.3071268913126,2.12660066633379));
#91462=CARTESIAN_POINT('Ctrl Pts',(-9.40212707427342,21.3028035137062,2.16111027112437));
#91463=CARTESIAN_POINT('Ctrl Pts',(-9.31338696659663,21.2978019485107,2.20752869420937));
#91464=CARTESIAN_POINT('Ctrl Pts',(-9.30515030113056,21.2973331095202,2.21193811280459));
#91465=CARTESIAN_POINT('Ctrl Pts',(-9.26521347672998,21.2950347291572,2.23381244510653));
#91466=CARTESIAN_POINT('Ctrl Pts',(-9.2341286938692,21.2931680878775,2.25236908693119));
#91467=CARTESIAN_POINT('Ctrl Pts',(-9.19878816219192,21.2909164287371,2.27528491478045));
#91468=CARTESIAN_POINT('Ctrl Pts',(-9.19382996878516,21.2905974628379,2.27854294901673));
#91469=CARTESIAN_POINT('Ctrl Pts',(-9.18590343993438,21.2900823746668,2.28382076549076));
#91470=CARTESIAN_POINT('Ctrl Pts',(-9.18292243759883,21.2898874773167,2.28582151393529));
#91471=CARTESIAN_POINT('Ctrl Pts',(-9.17763136852044,21.2895393809886,2.28940101074344));
#91472=CARTESIAN_POINT('Ctrl Pts',(-9.17531843361537,21.28938647083,2.29097543747345));
#91473=CARTESIAN_POINT('Ctrl Pts',(-9.17038203307026,21.2890585098531,2.2943564271401));
#91474=CARTESIAN_POINT('Ctrl Pts',(-9.16775998719448,21.2888833350482,2.29616489645935));
#91475=CARTESIAN_POINT('Ctrl Pts',(-9.16058560982151,21.2884013987963,2.30114782703011));
#91476=CARTESIAN_POINT('Ctrl Pts',(-9.15604544768949,21.2880934999663,2.30433961231346));
#91477=CARTESIAN_POINT('Ctrl Pts',(-9.13184662829229,21.2864372422295,2.32155815284345));
#91478=CARTESIAN_POINT('Ctrl Pts',(-9.11252034471343,21.2850606097371,2.3360433059577));
#91479=CARTESIAN_POINT('Ctrl Pts',(-9.05392142794344,21.2807394058507,2.38227151457293));
#91480=CARTESIAN_POINT('Ctrl Pts',(-9.01592757424103,21.277726499898,2.41557273939989));
#91481=CARTESIAN_POINT('Ctrl Pts',(-8.88752373856033,21.2669636947059,2.5404319031459));
#91482=CARTESIAN_POINT('Ctrl Pts',(-8.80751698747826,21.2592069482765,2.64187969540345));
#91483=CARTESIAN_POINT('Ctrl Pts',(-8.73286767803188,21.2510259388926,2.76752897205724));
#91484=CARTESIAN_POINT('Ctrl Pts',(-8.72420467963364,21.2500564955394,2.78272427479796));
#91485=CARTESIAN_POINT('Ctrl Pts',(-8.71228119170046,21.2486923203827,2.80453840291927));
#91486=CARTESIAN_POINT('Ctrl Pts',(-8.70879537338103,21.2482896493729,2.81103180244253));
#91487=CARTESIAN_POINT('Ctrl Pts',(-8.70319217737001,21.2476359411706,2.82166136237208));
#91488=CARTESIAN_POINT('Ctrl Pts',(-8.70104521444083,21.2473838679045,2.82578171049791));
#91489=CARTESIAN_POINT('Ctrl Pts',(-8.69657548545385,21.2468556751731,2.8344604012811));
#91490=CARTESIAN_POINT('Ctrl Pts',(-8.69425692330766,21.2465797050502,2.83902084664508));
#91491=CARTESIAN_POINT('Ctrl Pts',(-8.68876489988419,21.2459211681037,2.84996493775974));
#91492=CARTESIAN_POINT('Ctrl Pts',(-8.68561405781701,21.2455393893209,2.85635983084253));
#91493=CARTESIAN_POINT('Ctrl Pts',(-8.67497665685648,21.244236482752,2.87835320145688));
#91494=CARTESIAN_POINT('Ctrl Pts',(-8.66771988757726,21.2433232389886,2.89406160589563));
#91495=CARTESIAN_POINT('Ctrl Pts',(-8.65096439207781,21.2411512086961,2.93208861657945));
#91496=CARTESIAN_POINT('Ctrl Pts',(-8.64173847558102,21.2399013469183,2.95452211441172));
#91497=CARTESIAN_POINT('Ctrl Pts',(-8.60792953137675,21.2350830696333,3.04291566124165));
#91498=CARTESIAN_POINT('Ctrl Pts',(-8.5875591847026,21.231638108814,3.11038719020647));
#91499=CARTESIAN_POINT('Ctrl Pts',(-8.54994242726977,21.2232925582005,3.27774861985359));
#91500=CARTESIAN_POINT('Ctrl Pts',(-8.53805481268909,21.2184409491678,3.37845303050966));
#91501=CARTESIAN_POINT('Ctrl Pts',(-8.53649275767327,21.2125324444674,3.49029938558661));
#91502=CARTESIAN_POINT('Ctrl Pts',(-8.53646098064527,21.2119597726167,3.50103714852257));
#91503=CARTESIAN_POINT('Ctrl Pts',(-8.53658176970697,21.2111502896338,3.51605069394901));
#91504=CARTESIAN_POINT('Ctrl Pts',(-8.53663492389504,21.2109187189398,3.52032718952413));
#91505=CARTESIAN_POINT('Ctrl Pts',(-8.53675080086115,21.2105438379702,3.52721901810856));
#91506=CARTESIAN_POINT('Ctrl Pts',(-8.53680179307397,21.2104011731885,3.52983455635806));
#91507=CARTESIAN_POINT('Ctrl Pts',(-8.53692376803546,21.210100337392,3.53533430662061));
#91508=CARTESIAN_POINT('Ctrl Pts',(-8.53699626693786,21.2099420804834,3.53821845596389));
#91509=CARTESIAN_POINT('Ctrl Pts',(-8.53719463090444,21.209553498555,3.54527866660649));
#91510=CARTESIAN_POINT('Ctrl Pts',(-8.53732985103437,21.209322662046,3.54945442292691));
#91511=CARTESIAN_POINT('Ctrl Pts',(-8.53788283967565,21.2084855062561,3.56453484454326));
#91512=CARTESIAN_POINT('Ctrl Pts',(-8.53840468178118,21.2078737801958,3.57543505765787));
#91513=CARTESIAN_POINT('Ctrl Pts',(-8.54251979034078,21.2039274914821,3.64507607018328));
#91514=CARTESIAN_POINT('Ctrl Pts',(-8.54953136508475,21.2004425896762,3.70355615661841));
#91515=CARTESIAN_POINT('Ctrl Pts',(-8.57247777543465,21.1927434247547,3.82993566542132));
#91516=CARTESIAN_POINT('Ctrl Pts',(-8.58978333102514,21.1885242647581,3.89745032580979));
#91517=CARTESIAN_POINT('Ctrl Pts',(-8.63578567597808,21.179899157694,4.03523297328383));
#91518=CARTESIAN_POINT('Ctrl Pts',(-8.66527299870249,21.1755235017651,4.10503029413225));
#91519=CARTESIAN_POINT('Ctrl Pts',(-8.70489812915807,21.1707437526348,4.1816565936542));
#91520=CARTESIAN_POINT('Ctrl Pts',(-8.70986840195684,21.1701601018389,4.19101739165575));
#91521=CARTESIAN_POINT('Ctrl Pts',(-8.71801978183778,21.1692277491744,4.20597478114955));
#91522=CARTESIAN_POINT('Ctrl Pts',(-8.72113682998956,21.1688768087861,4.21160569532669));
#91523=CARTESIAN_POINT('Ctrl Pts',(-8.72675075627993,21.1682545239069,4.22159116309641));
#91524=CARTESIAN_POINT('Ctrl Pts',(-8.72923306840958,21.1679826679192,4.22595375179171));
#91525=CARTESIAN_POINT('Ctrl Pts',(-8.73446770029021,21.167416185326,4.23504433613493));
#91526=CARTESIAN_POINT('Ctrl Pts',(-8.7372241892471,21.1671217134128,4.23976984974173));
#91527=CARTESIAN_POINT('Ctrl Pts',(-8.74449223529763,21.1663551223996,4.25207063433728));
#91528=CARTESIAN_POINT('Ctrl Pts',(-8.7490459024572,21.1658845267094,4.25962085061249));
#91529=CARTESIAN_POINT('Ctrl Pts',(-8.76965800893085,21.1637964618045,4.29310872199924));
#91530=CARTESIAN_POINT('Ctrl Pts',(-8.78645744700883,21.1622061302865,4.3185826192565));
#91531=CARTESIAN_POINT('Ctrl Pts',(-8.83439914582753,21.1579387481391,4.38655572799235));
#91532=CARTESIAN_POINT('Ctrl Pts',(-8.86705939512393,21.155315953508,4.42792918338761));
#91533=CARTESIAN_POINT('Ctrl Pts',(-8.97150478951151,21.1475598476947,4.54648107798513));
#91534=CARTESIAN_POINT('Ctrl Pts',(-9.04944928307729,21.142576261814,4.61775433219206));
#91535=CARTESIAN_POINT('Ctrl Pts',(-9.15701541301805,21.1357631857022,4.696661533193));
#91536=CARTESIAN_POINT('Ctrl Pts',(-9.1801450907161,21.1343001148797,4.7126250711233));
#91537=CARTESIAN_POINT('Ctrl Pts',(-9.20833925665923,21.1325009723191,4.73090854663575));
#91538=CARTESIAN_POINT('Ctrl Pts',(-9.21297700116117,21.132204529286,4.73387899735192));
#91539=CARTESIAN_POINT('Ctrl Pts',(-9.22058963991437,21.1317169355873,4.73869447162572));
#91540=CARTESIAN_POINT('Ctrl Pts',(-9.22355462487179,21.1315267814213,4.74055515087622));
#91541=CARTESIAN_POINT('Ctrl Pts',(-9.22889032387238,21.1311840934668,4.74387695232787));
#91542=CARTESIAN_POINT('Ctrl Pts',(-9.23125855815697,21.1310318166463,4.74534196129335));
#91543=CARTESIAN_POINT('Ctrl Pts',(-9.23643311676034,21.1306987007447,4.74852260024066));
#91544=CARTESIAN_POINT('Ctrl Pts',(-9.23924101195282,21.1305176946732,4.75023550987749));
#91545=CARTESIAN_POINT('Ctrl Pts',(-9.24720989044726,21.1300033541549,4.75506000607419));
#91546=CARTESIAN_POINT('Ctrl Pts',(-9.25238429011887,21.1296686217544,4.75814916271871));
#91547=CARTESIAN_POINT('Ctrl Pts',(-9.28527290352683,21.1275370110273,4.77750939525265));
#91548=CARTESIAN_POINT('Ctrl Pts',(-9.31349580790314,21.1256898408835,4.79289472304763));
#91549=CARTESIAN_POINT('Ctrl Pts',(-9.41280254116626,21.1191873398328,4.84286190880665));
#91550=CARTESIAN_POINT('Ctrl Pts',(-9.48616447510012,21.1143860494115,4.8726075059821));
#91551=CARTESIAN_POINT('Ctrl Pts',(-9.65715228174409,21.103626519623,4.92629770037979));
#91552=CARTESIAN_POINT('Ctrl Pts',(-9.75558075408761,21.0977435122032,4.94642148469233));
#91553=CARTESIAN_POINT('Ctrl Pts',(-9.86590099355165,21.0916002502656,4.9573822535575));
#91554=CARTESIAN_POINT('Ctrl Pts',(-9.8765056875752,21.0910139409771,4.95831914879267));
#91555=CARTESIAN_POINT('Ctrl Pts',(-9.89355054844842,21.0900781815977,4.9596377514581));
#91556=CARTESIAN_POINT('Ctrl Pts',(-9.89998452372124,21.089726466836,4.96009272225645));
#91557=CARTESIAN_POINT('Ctrl Pts',(-9.91143240019448,21.0891032957391,4.96082621956821));
#91558=CARTESIAN_POINT('Ctrl Pts',(-9.91644509249127,21.0888313228433,4.96112150138762));
#91559=CARTESIAN_POINT('Ctrl Pts',(-9.92691524917671,21.0882650801918,4.961684207726));
#91560=CARTESIAN_POINT('Ctrl Pts',(-9.93237289838305,21.0879709621372,4.96194688007399));
#91561=CARTESIAN_POINT('Ctrl Pts',(-9.94661024148069,21.0872063470297,4.96255221497409));
#91562=CARTESIAN_POINT('Ctrl Pts',(-9.95539184863972,21.0867373586443,4.96284639152908));
#91563=CARTESIAN_POINT('Ctrl Pts',(-9.99436737631881,21.0846669755442,4.96380074024291));
#91564=CARTESIAN_POINT('Ctrl Pts',(-10.0245759197325,21.0830921422266,4.96360531750974));
#91565=CARTESIAN_POINT('Ctrl Pts',(-10.1066166978932,21.0788785685528,4.96053353149635));
#91566=CARTESIAN_POINT('Ctrl Pts',(-10.1583375172939,21.0762922994023,4.95583484762467));
#91567=CARTESIAN_POINT('Ctrl Pts',(-10.3009254274818,21.0692152413394,4.93519067490057));
#91568=CARTESIAN_POINT('Ctrl Pts',(-10.390691461434,21.0648288500034,4.91339552729158));
#91569=CARTESIAN_POINT('Ctrl Pts',(-10.5167660368826,21.0581387069485,4.86984818063788));
#91570=CARTESIAN_POINT('Ctrl Pts',(-10.5551363567249,21.0560248424622,4.8547524586733));
#91571=CARTESIAN_POINT('Ctrl Pts',(-10.5989521988299,21.0534646371539,4.83534024533925));
#91572=CARTESIAN_POINT('Ctrl Pts',(-10.6050704310159,21.0531037377691,4.83257910735675));
#91573=CARTESIAN_POINT('Ctrl Pts',(-10.6143296561969,21.0525520600224,4.82832353773122));
#91574=CARTESIAN_POINT('Ctrl Pts',(-10.6174847566823,21.0523630990202,4.82685979746426));
#91575=CARTESIAN_POINT('Ctrl Pts',(-10.6231554827871,21.0520216643432,4.82420438102518));
#91576=CARTESIAN_POINT('Ctrl Pts',(-10.6256729518529,21.0518694391256,4.82301676314877));
#91577=CARTESIAN_POINT('Ctrl Pts',(-10.6311141252355,21.0515390106314,4.82043088186607));
#91578=CARTESIAN_POINT('Ctrl Pts',(-10.6340365431695,21.0513606578538,4.81903010366078));
#91579=CARTESIAN_POINT('Ctrl Pts',(-10.642225513315,21.0508584641722,4.8150714503419));
#91580=CARTESIAN_POINT('Ctrl Pts',(-10.6474813424692,21.0505333196409,4.81249169073426));
#91581=CARTESIAN_POINT('Ctrl Pts',(-10.6593300903672,21.0497941432116,4.80658738727821));
#91582=CARTESIAN_POINT('Ctrl Pts',(-10.6659135729145,21.0493790838802,4.80324436605426));
#91583=CARTESIAN_POINT('Ctrl Pts',(-10.6867078973027,21.0480549089188,4.79248653360897));
#91584=CARTESIAN_POINT('Ctrl Pts',(-10.7008219654322,21.0471364632001,4.78488820900658));
#91585=CARTESIAN_POINT('Ctrl Pts',(-10.7586895583269,21.0432974234315,4.75249802229644));
#91586=CARTESIAN_POINT('Ctrl Pts',(-10.8012736386547,21.0402971342469,4.72569208732945));
#91587=CARTESIAN_POINT('Ctrl Pts',(-10.9467350795945,21.0296082615991,4.62330193253106));
#91588=CARTESIAN_POINT('Ctrl Pts',(-11.0410474002814,21.0219097677028,4.53650676924113));
#91589=CARTESIAN_POINT('Ctrl Pts',(-11.1347214881851,21.0137220141372,4.4244342244136));
#91590=CARTESIAN_POINT('Ctrl Pts',(-11.1462660878363,21.0127001152032,4.41007999121677));
#91591=CARTESIAN_POINT('Ctrl Pts',(-11.1621392883171,21.0112760471716,4.38956230495059));
#91592=CARTESIAN_POINT('Ctrl Pts',(-11.1666956752425,21.0108649597493,4.38357796722822));
#91593=CARTESIAN_POINT('Ctrl Pts',(-11.1740080984009,21.0102013610263,4.37381867430217));
#91594=CARTESIAN_POINT('Ctrl Pts',(-11.1767925016566,21.009947750139,4.37006522710676));
#91595=CARTESIAN_POINT('Ctrl Pts',(-11.1825727109988,21.0094192956094,4.36219484805808));
#91596=CARTESIAN_POINT('Ctrl Pts',(-11.1855651121342,21.009144585275,4.35807548538071));
#91597=CARTESIAN_POINT('Ctrl Pts',(-11.1926173576315,21.008494422858,4.34825999238966));
#91598=CARTESIAN_POINT('Ctrl Pts',(-11.196658003029,21.0081197065789,4.3425501780368));
#91599=CARTESIAN_POINT('Ctrl Pts',(-11.2100900803685,21.0068664097011,4.32327782704935));
#91600=CARTESIAN_POINT('Ctrl Pts',(-11.2192932903751,21.0059949104353,4.30958525443937));
#91601=CARTESIAN_POINT('Ctrl Pts',(-11.2687421622212,21.0012351319294,4.2332584867474));
#91602=CARTESIAN_POINT('Ctrl Pts',(-11.3043964994631,20.9975181250561,4.16777699043187));
#91603=CARTESIAN_POINT('Ctrl Pts',(-11.3597744263522,20.9908985377333,4.04454020773095));
#91604=CARTESIAN_POINT('Ctrl Pts',(-11.3811700748043,20.9879770697163,3.98772906042544));
#91605=CARTESIAN_POINT('Ctrl Pts',(-11.406670838702,20.983718731574,3.90471654848577));
#91606=CARTESIAN_POINT('Ctrl Pts',(-11.4136886518874,20.9824249091658,3.87947681474044));
#91607=CARTESIAN_POINT('Ctrl Pts',(-11.4239200913853,20.9803046684768,3.83844203636619));
#91608=CARTESIAN_POINT('Ctrl Pts',(-11.4275568608422,20.9794903835435,3.82275814532188));
#91609=CARTESIAN_POINT('Ctrl Pts',(-11.4365579543222,20.9772946049564,3.78080628546527));
#91610=CARTESIAN_POINT('Ctrl Pts',(-11.4414602383561,20.9758965958273,3.75444671073171));
#91611=CARTESIAN_POINT('Ctrl Pts',(-11.4464811884678,20.9741703166208,3.72260702659757));
#91612=CARTESIAN_POINT('Ctrl Pts',(-11.4472969071363,20.9738780694586,3.71724036833512));
#91613=CARTESIAN_POINT('Ctrl Pts',(-11.4485859946034,20.9733960013297,3.70842972611474));
#91614=CARTESIAN_POINT('Ctrl Pts',(-11.4490769890527,20.9732071391678,3.70498832595111));
#91615=CARTESIAN_POINT('Ctrl Pts',(-11.4499390431667,20.9728658077306,3.69878825181068));
#91616=CARTESIAN_POINT('Ctrl Pts',(-11.4503144977457,20.9727135862063,3.69603024099272));
#91617=CARTESIAN_POINT('Ctrl Pts',(-11.4510316633044,20.9724157252554,3.69064723748581));
#91618=CARTESIAN_POINT('Ctrl Pts',(-11.4513741176792,20.9722701355862,3.68802241189453));
#91619=CARTESIAN_POINT('Ctrl Pts',(-11.4521235011009,20.9719439083484,3.6821545241073));
#91620=CARTESIAN_POINT('Ctrl Pts',(-11.4525266894804,20.9717630680335,3.67891100868824));
#91621=CARTESIAN_POINT('Ctrl Pts',(-11.4535106169903,20.9713080933837,3.67077303471594));
#91622=CARTESIAN_POINT('Ctrl Pts',(-11.454077497768,20.9710332367512,3.66587697910149));
#91623=CARTESIAN_POINT('Ctrl Pts',(-11.4604998930407,20.9677627007257,3.60784340154265));
#91624=CARTESIAN_POINT('Ctrl Pts',(-11.4634636773972,20.9646285659503,3.55443221564043));
#91625=CARTESIAN_POINT('Ctrl Pts',(-11.4634996681794,20.9614426132404,3.50098551447728));
#91626=CARTESIAN_POINT('Ctrl Pts',(-11.4634996668985,20.9614427265142,3.50098741472866));
#91627=CARTESIAN_POINT('Ctrl Pts',(-11.4634998889677,20.9614231064952,3.50065827434728));
#91628=CARTESIAN_POINT('Ctrl Pts',(-11.4635,20.9614034846666,3.50032913609544));
#91629=CARTESIAN_POINT('Ctrl Pts',(-11.4635,20.9613838610471,3.50000000002865));
#91630=CARTESIAN_POINT('',(-11.4634999217228,20.8884519212361,3.50099524440106));
#91631=CARTESIAN_POINT('Ctrl Pts',(-11.4635,20.8884018418444,3.49999999996669));
#91632=CARTESIAN_POINT('Ctrl Pts',(-11.4635,20.8884183486207,3.5003310784354));
#91633=CARTESIAN_POINT('Ctrl Pts',(-11.4634998876533,20.8884348582932,3.500662159811));
#91634=CARTESIAN_POINT('Ctrl Pts',(-11.4634996629539,20.8884513708823,3.50099324403673));
#91635=CARTESIAN_POINT('Ctrl Pts',(-11.4634996615798,20.888451471758,3.50099526663525));
#91636=CARTESIAN_POINT('Ctrl Pts',(-11.4634678874633,20.8907817278273,3.54771783037357));
#91637=CARTESIAN_POINT('Ctrl Pts',(-11.4611986803181,20.8931652632148,3.59440894044376));
#91638=CARTESIAN_POINT('Ctrl Pts',(-11.4562447091829,20.8959151118543,3.6456229266027));
#91639=CARTESIAN_POINT('Ctrl Pts',(-11.4557657341047,20.8961694278967,3.65033567767033));
#91640=CARTESIAN_POINT('Ctrl Pts',(-11.4549259326783,20.8965970411513,3.6582180676293));
#91641=CARTESIAN_POINT('Ctrl Pts',(-11.4545776038289,20.8967696743937,3.6613890348129));
#91642=CARTESIAN_POINT('Ctrl Pts',(-11.4539232260965,20.8970856552067,3.66717182145757));
#91643=CARTESIAN_POINT('Ctrl Pts',(-11.4536204986812,20.8972288200656,3.6697840123862));
#91644=CARTESIAN_POINT('Ctrl Pts',(-11.4529817754272,20.8975248391498,3.67516851580173));
#91645=CARTESIAN_POINT('Ctrl Pts',(-11.4526448872473,20.8976777448881,3.67794066367647));
#91646=CARTESIAN_POINT('Ctrl Pts',(-11.4518567276296,20.8980282625831,3.68427474981859));
#91647=CARTESIAN_POINT('Ctrl Pts',(-11.4514002826456,20.8982261590924,3.68783599216815));
#91648=CARTESIAN_POINT('Ctrl Pts',(-11.4501719242579,20.8987457089006,3.69714793074098));
#91649=CARTESIAN_POINT('Ctrl Pts',(-11.4493789153753,20.8990684882368,3.70289572170898));
#91650=CARTESIAN_POINT('Ctrl Pts',(-11.4437702057706,20.9012687394216,3.74183630248317));
#91651=CARTESIAN_POINT('Ctrl Pts',(-11.4378491708847,20.9032007589316,3.77485746259861));
#91652=CARTESIAN_POINT('Ctrl Pts',(-11.4259168023662,20.9065282709584,3.83035297819525));
#91653=CARTESIAN_POINT('Ctrl Pts',(-11.4204940730595,20.9079057618472,3.85294240121919));
#91654=CARTESIAN_POINT('Ctrl Pts',(-11.3927160293921,20.9143703607978,3.95761432554385));
#91655=CARTESIAN_POINT('Ctrl Pts',(-11.3637668996709,20.9195462862548,4.03778230505363));
#91656=CARTESIAN_POINT('Ctrl Pts',(-11.3013152328085,20.9283333467417,4.17264315021601));
#91657=CARTESIAN_POINT('Ctrl Pts',(-11.2708837150819,20.9320027716621,4.22850968341083));
#91658=CARTESIAN_POINT('Ctrl Pts',(-11.2287883436083,20.936392852964,4.29507390705955));
#91659=CARTESIAN_POINT('Ctrl Pts',(-11.2204638517342,20.937232895955,4.30779410878638));
#91660=CARTESIAN_POINT('Ctrl Pts',(-11.208147160853,20.9384365075832,4.32598942359285));
#91661=CARTESIAN_POINT('Ctrl Pts',(-11.2043129491904,20.9388059287207,4.33156984837963));
#91662=CARTESIAN_POINT('Ctrl Pts',(-11.1975488724475,20.9394485937481,4.34126957450956));
#91663=CARTESIAN_POINT('Ctrl Pts',(-11.1946361562558,20.9397224780415,4.34540064700281));
#91664=CARTESIAN_POINT('Ctrl Pts',(-11.1889563335281,20.940251096742,4.35336830371731));
#91665=CARTESIAN_POINT('Ctrl Pts',(-11.1861919168658,20.9405059286469,4.3572067206404));
#91666=CARTESIAN_POINT('Ctrl Pts',(-11.1795643542736,20.9411111150987,4.36631569616052));
#91667=CARTESIAN_POINT('Ctrl Pts',(-11.1756844038229,20.9414608209053,4.37157394165595));
#91668=CARTESIAN_POINT('Ctrl Pts',(-11.1616796932645,20.9427069939652,4.390289927458));
#91669=CARTESIAN_POINT('Ctrl Pts',(-11.1513578176559,20.9435958298475,4.40359895483992));
#91670=CARTESIAN_POINT('Ctrl Pts',(-11.070888843521,20.9503116358383,4.50373743085783));
#91671=CARTESIAN_POINT('Ctrl Pts',(-10.9912456297667,20.9557177734446,4.58246317407575));
#91672=CARTESIAN_POINT('Ctrl Pts',(-10.8860507497717,20.9622218769823,4.66500375730469));
#91673=CARTESIAN_POINT('Ctrl Pts',(-10.8683754197174,20.9632972820162,4.67823758108123));
#91674=CARTESIAN_POINT('Ctrl Pts',(-10.8118772216963,20.9667004905346,4.71857664482065));
#91675=CARTESIAN_POINT('Ctrl Pts',(-10.7720369123503,20.9690505551201,4.74419937652244));
#91676=CARTESIAN_POINT('Ctrl Pts',(-10.7176537447061,20.9722849988975,4.77555622806802));
#91677=CARTESIAN_POINT('Ctrl Pts',(-10.7041587521399,20.9730897400513,4.78305534039246));
#91678=CARTESIAN_POINT('Ctrl Pts',(-10.6842089226722,20.9742861424566,4.79373184827651));
#91679=CARTESIAN_POINT('Ctrl Pts',(-10.6778449078585,20.9746687859607,4.79707756978428));
#91680=CARTESIAN_POINT('Ctrl Pts',(-10.6663603756657,20.9753615358747,4.8030076730888));
#91681=CARTESIAN_POINT('Ctrl Pts',(-10.6612487890496,20.9756706543867,4.80560912342843));
#91682=CARTESIAN_POINT('Ctrl Pts',(-10.6532502686896,20.976155782314,4.80962080724145));
#91683=CARTESIAN_POINT('Ctrl Pts',(-10.6503737019194,20.9763305381653,4.81105172275856));
#91684=CARTESIAN_POINT('Ctrl Pts',(-10.6449933449511,20.9766579782372,4.81370605566845));
#91685=CARTESIAN_POINT('Ctrl Pts',(-10.6424907621754,20.9768105166132,4.81493179894655));
#91686=CARTESIAN_POINT('Ctrl Pts',(-10.6368221945154,20.9771565557812,4.81768816823731));
#91687=CARTESIAN_POINT('Ctrl Pts',(-10.633654201036,20.9773503127382,4.81921452732917));
#91688=CARTESIAN_POINT('Ctrl Pts',(-10.6240584517716,20.9779382304224,4.8237952803805));
#91689=CARTESIAN_POINT('Ctrl Pts',(-10.6176139865872,20.978334471661,4.82681417499587));
#91690=CARTESIAN_POINT('Ctrl Pts',(-10.5361922965864,20.9833558613795,4.86423425519794));
#91691=CARTESIAN_POINT('Ctrl Pts',(-10.4584655685125,20.9883025126594,4.89228009642619));
#91692=CARTESIAN_POINT('Ctrl Pts',(-10.3179515557337,20.9970608168189,4.92993267866941));
#91693=CARTESIAN_POINT('Ctrl Pts',(-10.2561106916181,21.0008570900837,4.94229286519773));
#91694=CARTESIAN_POINT('Ctrl Pts',(-10.1346290331164,21.0080797808981,4.95851104418175));
#91695=CARTESIAN_POINT('Ctrl Pts',(-10.0751636212557,21.0115086470748,4.96278201794068));
#91696=CARTESIAN_POINT('Ctrl Pts',(-10.0009051341905,21.0156446676167,4.96357347421454));
#91697=CARTESIAN_POINT('Ctrl Pts',(-9.98621110586287,21.0164561883048,4.96350880497));
#91698=CARTESIAN_POINT('Ctrl Pts',(-9.96484275948789,21.0176266199279,4.96309289620649));
#91699=CARTESIAN_POINT('Ctrl Pts',(-9.95816625717915,21.017990943691,4.96291722066639));
#91700=CARTESIAN_POINT('Ctrl Pts',(-9.94645373087873,21.0186277170247,4.96252878610567));
#91701=CARTESIAN_POINT('Ctrl Pts',(-9.94141720272888,21.0189007724277,4.96233570354803));
#91702=CARTESIAN_POINT('Ctrl Pts',(-9.93097202981078,21.0194655051952,4.96188122279942));
#91703=CARTESIAN_POINT('Ctrl Pts',(-9.92556363038191,21.0197570538729,4.96161581758119));
#91704=CARTESIAN_POINT('Ctrl Pts',(-9.91161170355261,21.0205069859648,4.96085351604024));
#91705=CARTESIAN_POINT('Ctrl Pts',(-9.90307077020996,21.0209639694783,4.96031168415693));
#91706=CARTESIAN_POINT('Ctrl Pts',(-9.86925255558547,21.0227655107959,4.95786826988807));
#91707=CARTESIAN_POINT('Ctrl Pts',(-9.84402098433956,21.0240920134794,4.95538497804692));
#91708=CARTESIAN_POINT('Ctrl Pts',(-9.68033566857496,21.0326066645846,4.93496900683278));
#91709=CARTESIAN_POINT('Ctrl Pts',(-9.54500415439845,21.0391377933756,4.89796201794667));
#91710=CARTESIAN_POINT('Ctrl Pts',(-9.37405280195013,21.0483917719569,4.82371114732454));
#91711=CARTESIAN_POINT('Ctrl Pts',(-9.33206261267229,21.0507626284908,4.80302723947746));
#91712=CARTESIAN_POINT('Ctrl Pts',(-9.28263427905847,21.053756157782,4.77566185559158));
#91713=CARTESIAN_POINT('Ctrl Pts',(-9.27417705092004,21.0542758057067,4.77086890900552));
#91714=CARTESIAN_POINT('Ctrl Pts',(-9.26231644351195,21.055016027925,4.76399016799674));
#91715=CARTESIAN_POINT('Ctrl Pts',(-9.25887270545364,21.055232328876,4.76197405156413));
#91716=CARTESIAN_POINT('Ctrl Pts',(-9.25298365166132,21.0556046601951,4.75849392057858));
#91717=CARTESIAN_POINT('Ctrl Pts',(-9.25053425935228,21.0557602497611,4.75703678400076));
#91718=CARTESIAN_POINT('Ctrl Pts',(-9.24580739955322,21.0560619460629,4.75420606158851));
#91719=CARTESIAN_POINT('Ctrl Pts',(-9.24352940794893,21.0562079873464,4.75283341535161));
#91720=CARTESIAN_POINT('Ctrl Pts',(-9.23805000757893,21.0565608051909,4.74951130788908));
#91721=CARTESIAN_POINT('Ctrl Pts',(-9.23485233910362,21.0567679704366,4.74755575261467));
#91722=CARTESIAN_POINT('Ctrl Pts',(-9.22311419028167,21.0575330142122,4.74031510553916));
#91723=CARTESIAN_POINT('Ctrl Pts',(-9.21462086916275,21.0580955155457,4.73495454646749));
#91724=CARTESIAN_POINT('Ctrl Pts',(-9.11464645272156,21.0648169833118,4.6704072784527));
#91725=CARTESIAN_POINT('Ctrl Pts',(-9.03000131371245,21.0714836212155,4.60127390049134));
#91726=CARTESIAN_POINT('Ctrl Pts',(-8.9080712291999,21.0819379462725,4.47662860940969));
#91727=CARTESIAN_POINT('Ctrl Pts',(-8.86550869595354,21.0858063642649,4.42684563549367));
#91728=CARTESIAN_POINT('Ctrl Pts',(-8.80541468862294,21.091566023651,4.34618787342835));
#91729=CARTESIAN_POINT('Ctrl Pts',(-8.78543365341597,21.0935430123415,4.31724957676257));
#91730=CARTESIAN_POINT('Ctrl Pts',(-8.76153559450679,21.0959908875846,4.27982286610712));
#91731=CARTESIAN_POINT('Ctrl Pts',(-8.75663217437518,21.0964979933706,4.27198072637484));
#91732=CARTESIAN_POINT('Ctrl Pts',(-8.7488967042639,21.0973059929001,4.25934431402223));
#91733=CARTESIAN_POINT('Ctrl Pts',(-8.74601715621876,21.0976086121102,4.2545795336059));
#91734=CARTESIAN_POINT('Ctrl Pts',(-8.74060421071949,21.0981810357783,4.24550618761535));
#91735=CARTESIAN_POINT('Ctrl Pts',(-8.73806556517226,21.0984510274128,4.24120085866339));
#91736=CARTESIAN_POINT('Ctrl Pts',(-8.73234441442198,21.099063029358,4.23138367062301));
#91737=CARTESIAN_POINT('Ctrl Pts',(-8.72917569749857,21.099404541552,4.22586386548708));
#91738=CARTESIAN_POINT('Ctrl Pts',(-8.72106022233904,21.1002859795838,4.21151091729666));
#91739=CARTESIAN_POINT('Ctrl Pts',(-8.71616888545164,21.100823936604,4.2026467223897));
#91740=CARTESIAN_POINT('Ctrl Pts',(-8.68366004952092,21.1044468437323,4.14226051228089));
#91741=CARTESIAN_POINT('Ctrl Pts',(-8.65905745898278,21.1074240550001,4.08917191774264));
#91742=CARTESIAN_POINT('Ctrl Pts',(-8.6036309159947,21.1149730806284,3.94796951901581));
#91743=CARTESIAN_POINT('Ctrl Pts',(-8.57793780684316,21.1194139252313,3.85813677922145));
#91744=CARTESIAN_POINT('Ctrl Pts',(-8.55113998458815,21.1266717584984,3.71341964542923));
#91745=CARTESIAN_POINT('Ctrl Pts',(-8.54425828471586,21.1293831836728,3.6598695230222));
#91746=CARTESIAN_POINT('Ctrl Pts',(-8.53959128084539,21.1327888041901,3.59564432388117));
#91747=CARTESIAN_POINT('Ctrl Pts',(-8.53894556319771,21.1333467344117,3.5852137543083));
#91748=CARTESIAN_POINT('Ctrl Pts',(-8.5382017406495,21.1341322243204,3.57067511772246));
#91749=CARTESIAN_POINT('Ctrl Pts',(-8.53800913229654,21.1343547758547,3.56657195526271));
#91750=CARTESIAN_POINT('Ctrl Pts',(-8.5377112159965,21.1347345493512,3.55959874438));
#91751=CARTESIAN_POINT('Ctrl Pts',(-8.5375970761848,21.1348912844461,3.55672906172041));
#91752=CARTESIAN_POINT('Ctrl Pts',(-8.53739453182035,21.1351925653286,3.55122909891772));
#91753=CARTESIAN_POINT('Ctrl Pts',(-8.53730477424594,21.1353370309784,3.54859889354514));
#91754=CARTESIAN_POINT('Ctrl Pts',(-8.53708527353023,21.1357216754216,3.54161409050566));
#91755=CARTESIAN_POINT('Ctrl Pts',(-8.53696788040713,21.1359625274059,3.53725916656505));
#91756=CARTESIAN_POINT('Ctrl Pts',(-8.53661775649572,21.1368271055657,3.52169026017909));
#91757=CARTESIAN_POINT('Ctrl Pts',(-8.53649450725721,21.137456486465,3.51047449483913));
#91758=CARTESIAN_POINT('Ctrl Pts',(-8.53654515516309,21.1431198413276,3.41047310841816));
#91759=CARTESIAN_POINT('Ctrl Pts',(-8.5446694720475,21.1484889986286,3.32188275367972));
#91760=CARTESIAN_POINT('Ctrl Pts',(-8.57920590428533,21.1599541336159,3.13460802694218));
#91761=CARTESIAN_POINT('Ctrl Pts',(-8.60801224365818,21.1660005059439,3.03681198907617));
#91762=CARTESIAN_POINT('Ctrl Pts',(-8.65463390940712,21.1728843656703,2.92358584571164));
#91763=CARTESIAN_POINT('Ctrl Pts',(-8.6629456441163,21.174038080151,2.90455990508909));
#91764=CARTESIAN_POINT('Ctrl Pts',(-8.67487389436709,21.1755987136269,2.87876598986451));
#91765=CARTESIAN_POINT('Ctrl Pts',(-8.67814267310525,21.1760173772424,2.87184070361112));
#91766=CARTESIAN_POINT('Ctrl Pts',(-8.68373156924583,21.1767183812838,2.86023681370671));
#91767=CARTESIAN_POINT('Ctrl Pts',(-8.68602261885863,21.1770017134976,2.85554444748383));
#91768=CARTESIAN_POINT('Ctrl Pts',(-8.69059633297172,21.1775595060649,2.84630267495011));
#91769=CARTESIAN_POINT('Ctrl Pts',(-8.69287771301283,21.1778340057171,2.84175271837361));
#91770=CARTESIAN_POINT('Ctrl Pts',(-8.69795460357751,21.1784367805802,2.83175790666896));
#91771=CARTESIAN_POINT('Ctrl Pts',(-8.70076063566251,21.1787646846549,2.82631848374136));
#91772=CARTESIAN_POINT('Ctrl Pts',(-8.71073046053708,21.1799116385908,2.80728621738846));
#91773=CARTESIAN_POINT('Ctrl Pts',(-8.71807424922285,21.1807243901212,2.79378847143435));
#91774=CARTESIAN_POINT('Ctrl Pts',(-8.79051892301356,21.1884500206363,2.66549156394738));
#91775=CARTESIAN_POINT('Ctrl Pts',(-8.87064920523814,21.1947393068515,2.5598843986068));
#91776=CARTESIAN_POINT('Ctrl Pts',(-8.99962658011907,21.2036714996917,2.43058386451901));
#91777=CARTESIAN_POINT('Ctrl Pts',(-9.03723330910315,21.2061762982343,2.3966063830991));
#91778=CARTESIAN_POINT('Ctrl Pts',(-9.09529543359107,21.21002594748,2.3493795271473));
#91779=CARTESIAN_POINT('Ctrl Pts',(-9.11444297778402,21.2112930331554,2.33457885294272));
#91780=CARTESIAN_POINT('Ctrl Pts',(-9.13842508106681,21.2128889430654,2.31697347333036));
#91781=CARTESIAN_POINT('Ctrl Pts',(-9.14292130662893,21.2131885234483,2.31371200161458));
#91782=CARTESIAN_POINT('Ctrl Pts',(-9.1500262668751,21.2136626947862,2.3086196829808));
#91783=CARTESIAN_POINT('Ctrl Pts',(-9.15262264918451,21.213836133331,2.30677159281626));
#91784=CARTESIAN_POINT('Ctrl Pts',(-9.15751054449196,21.2141629884947,2.3033164156148));
#91785=CARTESIAN_POINT('Ctrl Pts',(-9.15980064230863,21.2143162727403,2.3017074135811));
#91786=CARTESIAN_POINT('Ctrl Pts',(-9.16503915312032,21.2146672221375,2.29804928294395));
#91787=CARTESIAN_POINT('Ctrl Pts',(-9.16799049834818,21.2148651702731,2.2960044308019));
#91788=CARTESIAN_POINT('Ctrl Pts',(-9.17583763242447,21.2153920116797,2.29061014164183));
#91789=CARTESIAN_POINT('Ctrl Pts',(-9.18074626022775,21.215722111854,2.28727960969383));
#91790=CARTESIAN_POINT('Ctrl Pts',(-9.2157394062011,21.2180784270235,2.26384596979193));
#91791=CARTESIAN_POINT('Ctrl Pts',(-9.24653791983643,21.2201680476056,2.24483628898403));
#91792=CARTESIAN_POINT('Ctrl Pts',(-9.28646677278156,21.2228666019121,2.22219047365839));
#91793=CARTESIAN_POINT('Ctrl Pts',(-9.29497465069798,21.2234410277182,2.21747666558154));
#91794=CARTESIAN_POINT('Ctrl Pts',(-9.31156780052904,21.2245594294929,2.20849819803641));
#91795=CARTESIAN_POINT('Ctrl Pts',(-9.31964733547032,21.2251031336573,2.20422376699748));
#91796=CARTESIAN_POINT('Ctrl Pts',(-9.41270439937898,21.2313516085068,2.15610275540327));
#91797=CARTESIAN_POINT('Ctrl Pts',(-9.50175063296573,21.2371801747724,2.12060678763121));
#91798=CARTESIAN_POINT('Ctrl Pts',(-9.63273521958418,21.2451899228687,2.0827469005947));
#91799=CARTESIAN_POINT('Ctrl Pts',(-9.67230370284899,21.2475431890549,2.07307837528896));
#91800=CARTESIAN_POINT('Ctrl Pts',(-9.72886736455619,21.2508075846401,2.06173458678877));
#91801=CARTESIAN_POINT('Ctrl Pts',(-9.74556544783553,21.251759264722,2.05868691909391));
#91802=CARTESIAN_POINT('Ctrl Pts',(-9.77522327567962,21.2534286327248,2.05380538734197));
#91803=CARTESIAN_POINT('Ctrl Pts',(-9.78816147435961,21.2541498958856,2.05185363717459));
#91804=CARTESIAN_POINT('Ctrl Pts',(-9.80743919165336,21.2552144475472,2.04920945282567));
#91805=CARTESIAN_POINT('Ctrl Pts',(-9.81375963213919,21.2555618639238,2.0483845537268));
#91806=CARTESIAN_POINT('Ctrl Pts',(-9.825046456361,21.2561794494475,2.04698640818088));
#91807=CARTESIAN_POINT('Ctrl Pts',(-9.83001073990744,21.2564501113165,2.04639727134377));
#91808=CARTESIAN_POINT('Ctrl Pts',(-9.84050440907031,21.2570202306539,2.04520642662856));
#91809=CARTESIAN_POINT('Ctrl Pts',(-9.84603441178467,21.257319494923,2.04461077939027));
#91810=CARTESIAN_POINT('Ctrl Pts',(-9.86074466905555,21.2581124958157,2.04311109059864));
#91811=CARTESIAN_POINT('Ctrl Pts',(-9.86993038601583,21.2586045076349,2.04226228618085));
#91812=CARTESIAN_POINT('Ctrl Pts',(-9.9099888736827,21.2607369351497,2.03894235154316));
#91813=CARTESIAN_POINT('Ctrl Pts',(-9.94092877728684,21.2623495723929,2.03736463017295));
#91814=CARTESIAN_POINT('Ctrl Pts',(-10.1263967790424,21.2718538287936,2.03380250583381));
#91815=CARTESIAN_POINT('Ctrl Pts',(-10.28036568849,21.2789508668227,2.05532114542294));
#91816=CARTESIAN_POINT('Ctrl Pts',(-10.457549551469,21.2883819563988,2.10952212768218));
#91817=CARTESIAN_POINT('Ctrl Pts',(-10.4866996657552,21.2899814742456,2.11945536942276));
#91818=CARTESIAN_POINT('Ctrl Pts',(-10.521089499703,21.2919498245786,2.132398636556));
#91819=CARTESIAN_POINT('Ctrl Pts',(-10.5266533148601,21.2922708612208,2.13453156774136));
#91820=CARTESIAN_POINT('Ctrl Pts',(-10.5352548308002,21.2927714134737,2.13788941596586));
#91821=CARTESIAN_POINT('Ctrl Pts',(-10.538301771078,21.2929495537965,2.139090679047));
#91822=CARTESIAN_POINT('Ctrl Pts',(-10.5439339579229,21.2932804209201,2.14133305521722));
#91823=CARTESIAN_POINT('Ctrl Pts',(-10.5465202772114,21.2934329787906,2.14237133072001));
#91824=CARTESIAN_POINT('Ctrl Pts',(-10.5523675219553,21.2937792930083,2.1447381178771));
#91825=CARTESIAN_POINT('Ctrl Pts',(-10.5556266116033,21.2939733072907,2.14607100762659));
#91826=CARTESIAN_POINT('Ctrl Pts',(-10.5654792519445,21.2945627631698,2.15014206735476));
#91827=CARTESIAN_POINT('Ctrl Pts',(-10.5720575049815,21.2949603009552,2.15291669542205));
#91828=CARTESIAN_POINT('Ctrl Pts',(-10.627314126559,21.2983315791153,2.17670100511284));
#91829=CARTESIAN_POINT('Ctrl Pts',(-10.6748336414272,21.3014397674838,2.20029168682407));
#91830=CARTESIAN_POINT('Ctrl Pts',(-10.8052601675048,21.3103728172256,2.27412426202323));
#91831=CARTESIAN_POINT('Ctrl Pts',(-10.8846184461138,21.31628014391,2.33009928968929));
#91832=CARTESIAN_POINT('Ctrl Pts',(-11.0001032064973,21.32525259741,2.43007146471581));
#91833=CARTESIAN_POINT('Ctrl Pts',(-11.0402177048261,21.3284599070218,2.46902873282656));
#91834=CARTESIAN_POINT('Ctrl Pts',(-11.087617682278,21.3323599827721,2.52065234540852));
#91835=CARTESIAN_POINT('Ctrl Pts',(-11.0970727983884,21.3331441487931,2.53125578897215));
#91836=CARTESIAN_POINT('Ctrl Pts',(-11.1106851418213,21.3342826344654,2.54697629879894));
#91837=CARTESIAN_POINT('Ctrl Pts',(-11.1149643751268,21.3346419604253,2.5519862324318));
#91838=CARTESIAN_POINT('Ctrl Pts',(-11.1224486011826,21.3352729999617,2.56086920156233));
#91839=CARTESIAN_POINT('Ctrl Pts',(-11.1256677222223,21.3355452857153,2.56473014648532));
#91840=CARTESIAN_POINT('Ctrl Pts',(-11.1323376596818,21.3361112989426,2.57281424938419));
#91841=CARTESIAN_POINT('Ctrl Pts',(-11.1357848957104,21.3364048800448,2.57704026985936));
#91842=CARTESIAN_POINT('Ctrl Pts',(-11.1446913057284,21.3371661935363,2.5880842423434));
#91843=CARTESIAN_POINT('Ctrl Pts',(-11.1501132559022,21.3376324426726,2.59493202601757));
#91844=CARTESIAN_POINT('Ctrl Pts',(-11.1718807051539,21.3395161900734,2.62293525407937));
#91845=CARTESIAN_POINT('Ctrl Pts',(-11.1877069256551,21.3409134331606,2.64448884740441));
#91846=CARTESIAN_POINT('Ctrl Pts',(-11.2937703485707,21.3505078083649,2.79755659716515));
#91847=CARTESIAN_POINT('Ctrl Pts',(-11.3625535910143,21.3578155085845,2.94258992024518));
#91848=CARTESIAN_POINT('Ctrl Pts',(-11.4151597132442,21.3675079728895,3.12567579722264));
#91849=CARTESIAN_POINT('Ctrl Pts',(-11.4227793757136,21.3691198930767,3.15577013325147));
#91850=CARTESIAN_POINT('Ctrl Pts',(-11.430717017823,21.3711021210456,3.19191441734161));
#91851=CARTESIAN_POINT('Ctrl Pts',(-11.4319622057151,21.3714238486354,3.19775481762025));
#91852=CARTESIAN_POINT('Ctrl Pts',(-11.4338354806062,21.3719252492649,3.20681267076338));
#91853=CARTESIAN_POINT('Ctrl Pts',(-11.4344885742218,21.3721035395539,3.21002495716689));
#91854=CARTESIAN_POINT('Ctrl Pts',(-11.435676907326,21.3724345421612,3.21597212489187));
#91855=CARTESIAN_POINT('Ctrl Pts',(-11.4362151306475,21.3725870844127,3.21870635592564));
#91856=CARTESIAN_POINT('Ctrl Pts',(-11.4374150468531,21.3729331787579,3.22489528229714));
#91857=CARTESIAN_POINT('Ctrl Pts',(-11.438072092779,21.3731269873723,3.22835081804142));
#91858=CARTESIAN_POINT('Ctrl Pts',(-11.4400216473243,21.3737152136708,3.23880923377225));
#91859=CARTESIAN_POINT('Ctrl Pts',(-11.4412754868841,21.374111715007,3.24581910410662));
#91860=CARTESIAN_POINT('Ctrl Pts',(-11.4563984470665,21.3791296586784,3.33407908000419));
#91861=CARTESIAN_POINT('Ctrl Pts',(-11.4634291991323,21.38407206109,3.41634335699287));
#91862=CARTESIAN_POINT('Ctrl Pts',(-11.4634998226655,21.3890586118033,3.49916806716909));
#91863=CARTESIAN_POINT('Ctrl Pts',(-11.4635,21.38908365615,3.49958403613083));
#91864=CARTESIAN_POINT('Ctrl Pts',(-11.4635,21.3891087006547,3.49999999989906));
#91865=CARTESIAN_POINT('Origin',(-10.,13.2,3.5));
#91866=CARTESIAN_POINT('',(-11.4634999989655,21.95929037674,3.50005409278718));
#91867=CARTESIAN_POINT('',(-11.4634995977471,21.8907054572846,3.50002669594524));
#91868=CARTESIAN_POINT('',(-11.4635,13.2,3.5));
#91869=CARTESIAN_POINT('Ctrl Pts',(-11.4634999989303,21.9592903521363,3.50005595443291));
#91870=CARTESIAN_POINT('Ctrl Pts',(-11.4635000837772,21.9591704883509,3.49783676651995));
#91871=CARTESIAN_POINT('Ctrl Pts',(-11.4634951210042,21.9590507810711,3.49561757043241));
#91872=CARTESIAN_POINT('Ctrl Pts',(-11.4634633356496,21.9586711814159,3.48857120664378));
#91873=CARTESIAN_POINT('Ctrl Pts',(-11.4634176777367,21.9584118738391,3.48374412844848));
#91874=CARTESIAN_POINT('Ctrl Pts',(-11.4632041962147,21.957618078178,3.46892637974804));
#91875=CARTESIAN_POINT('Ctrl Pts',(-11.4629579376394,21.9570860205732,3.45893701153549));
#91876=CARTESIAN_POINT('Ctrl Pts',(-11.4611625807412,21.954361214927,3.40749830568833));
#91877=CARTESIAN_POINT('Ctrl Pts',(-11.4579541439654,21.9522202978012,3.36612404212276));
#91878=CARTESIAN_POINT('Ctrl Pts',(-11.4410054772692,21.9450506786003,3.225451272886));
#91879=CARTESIAN_POINT('Ctrl Pts',(-11.4188333281464,21.9402629521516,3.12745979366409));
#91880=CARTESIAN_POINT('Ctrl Pts',(-11.3710145863942,21.9329358614462,2.98560701919107));
#91881=CARTESIAN_POINT('Ctrl Pts',(-11.3528394360572,21.9304854775702,2.93954843727851));
#91882=CARTESIAN_POINT('Ctrl Pts',(-11.3224999054142,21.9267113782372,2.87278779961937));
#91883=CARTESIAN_POINT('Ctrl Pts',(-11.3121029516317,21.925461926811,2.85131913981528));
#91884=CARTESIAN_POINT('Ctrl Pts',(-11.2986561562204,21.9238858904358,2.82520002798487));
#91885=CARTESIAN_POINT('Ctrl Pts',(-11.2960978165354,21.9235876976811,2.82029913761618));
#91886=CARTESIAN_POINT('Ctrl Pts',(-11.2920240379942,21.9231152710309,2.81260182493634));
#91887=CARTESIAN_POINT('Ctrl Pts',(-11.2905271190604,21.9229421759555,2.80979559519673));
#91888=CARTESIAN_POINT('Ctrl Pts',(-11.2876957141098,21.9226156597463,2.80452905750818));
#91889=CARTESIAN_POINT('Ctrl Pts',(-11.2863633113951,21.9224623686253,2.80206768620966));
#91890=CARTESIAN_POINT('Ctrl Pts',(-11.2833020514056,21.9221110076161,2.79645111107296));
#91891=CARTESIAN_POINT('Ctrl Pts',(-11.2815686155178,21.9219126517508,2.79329845238403));
#91892=CARTESIAN_POINT('Ctrl Pts',(-11.276933395061,21.9213839012366,2.78494135818655));
#91893=CARTESIAN_POINT('Ctrl Pts',(-11.2740114506032,21.9210522855656,2.77974825378787));
#91894=CARTESIAN_POINT('Ctrl Pts',(-11.252777994898,21.9186553468001,2.74254401312974));
#91895=CARTESIAN_POINT('Ctrl Pts',(-11.233295347001,21.9165241695375,2.7112196602872));
#91896=CARTESIAN_POINT('Ctrl Pts',(-11.2018455469214,21.9132194012611,2.66467242925011));
#91897=CARTESIAN_POINT('Ctrl Pts',(-11.1907235363588,21.9120736448428,2.64889348971784));
#91898=CARTESIAN_POINT('Ctrl Pts',(-11.1300698314428,21.9059605524687,2.56636002406667));
#91899=CARTESIAN_POINT('Ctrl Pts',(-11.0752268583977,21.9009041594141,2.50369200737933));
#91900=CARTESIAN_POINT('Ctrl Pts',(-10.9807191466828,21.893133951048,2.41264729949082));
#91901=CARTESIAN_POINT('Ctrl Pts',(-10.9444516243821,21.8903328228964,2.38100146087094));
#91902=CARTESIAN_POINT('Ctrl Pts',(-10.8841848114728,21.8859705980108,2.33343609705836));
#91903=CARTESIAN_POINT('Ctrl Pts',(-10.8611630631068,21.8843664054587,2.31633938058716));
#91904=CARTESIAN_POINT('Ctrl Pts',(-10.8305779474961,21.8823131895614,2.29499088734407));
#91905=CARTESIAN_POINT('Ctrl Pts',(-10.823459536086,21.8818406230474,2.29011525947487));
#91906=CARTESIAN_POINT('Ctrl Pts',(-10.8124149750886,21.8811154420045,2.28269311634664));
#91907=CARTESIAN_POINT('Ctrl Pts',(-10.8085191111315,21.8808611626428,2.28010205821046));
#91908=CARTESIAN_POINT('Ctrl Pts',(-10.8007541020377,21.8803573363245,2.27499125048678));
#91909=CARTESIAN_POINT('Ctrl Pts',(-10.7968853260594,21.8801077740617,2.27247104062598));
#91910=CARTESIAN_POINT('Ctrl Pts',(-10.7880757159549,21.8795427685242,2.26679145795087));
#91911=CARTESIAN_POINT('Ctrl Pts',(-10.7831276708928,21.8792277445854,2.26364337882923));
#91912=CARTESIAN_POINT('Ctrl Pts',(-10.7691422429803,21.87834376245,2.25486311910358));
#91913=CARTESIAN_POINT('Ctrl Pts',(-10.7600620194861,21.8777773151768,2.24929964554339));
#91914=CARTESIAN_POINT('Ctrl Pts',(-10.7071689109668,21.874519490189,2.21768070598441));
#91915=CARTESIAN_POINT('Ctrl Pts',(-10.6620771828199,21.8719082550391,2.19382805272781));
#91916=CARTESIAN_POINT('Ctrl Pts',(-10.4951779325324,21.8626900088065,2.11641052490169));
#91917=CARTESIAN_POINT('Ctrl Pts',(-10.3674773134903,21.8565101415634,2.07715951881793));
#91918=CARTESIAN_POINT('Ctrl Pts',(-10.2072676110131,21.8482293629933,2.05095389394188));
#91919=CARTESIAN_POINT('Ctrl Pts',(-10.1781547784743,21.8467013936436,2.04708736552379));
#91920=CARTESIAN_POINT('Ctrl Pts',(-10.1430983756158,21.8448131834933,2.0435008842159));
#91921=CARTESIAN_POINT('Ctrl Pts',(-10.1372458786108,21.8444963460496,2.04293775498961));
#91922=CARTESIAN_POINT('Ctrl Pts',(-10.1281460052437,21.8440009883469,2.0421174731926));
#91923=CARTESIAN_POINT('Ctrl Pts',(-10.1249008281039,21.8438237986499,2.0418358654302));
#91924=CARTESIAN_POINT('Ctrl Pts',(-10.1188767787523,21.8434938410214,2.04133337173733));
#91925=CARTESIAN_POINT('Ctrl Pts',(-10.11609820089,21.8433412351377,2.04110959003202));
#91926=CARTESIAN_POINT('Ctrl Pts',(-10.1097874907034,21.842993703369,2.04061947948288));
#91927=CARTESIAN_POINT('Ctrl Pts',(-10.1062550356974,21.8427985111697,2.0403580358101));
#91928=CARTESIAN_POINT('Ctrl Pts',(-10.0954909666558,21.8422017875704,2.03960064786574));
#91929=CARTESIAN_POINT('Ctrl Pts',(-10.0882566989605,21.8417980844197,2.03914561194563));
#91930=CARTESIAN_POINT('Ctrl Pts',(-10.0178409584893,21.8378446863776,2.03524140234865));
#91931=CARTESIAN_POINT('Ctrl Pts',(-9.95450786348122,21.8341043296183,2.03583987735351));
#91932=CARTESIAN_POINT('Ctrl Pts',(-9.77662597607295,21.8234162117968,2.04907380399863));
#91933=CARTESIAN_POINT('Ctrl Pts',(-9.66322180877623,21.8164226908135,2.071129844737));
#91934=CARTESIAN_POINT('Ctrl Pts',(-9.5197804533306,21.8077945664898,2.11707546265889));
#91935=CARTESIAN_POINT('Ctrl Pts',(-9.48639429982574,21.8057987001517,2.12912415599765));
#91936=CARTESIAN_POINT('Ctrl Pts',(-9.44487345930459,21.8033312202667,2.14583871379558));
#91937=CARTESIAN_POINT('Ctrl Pts',(-9.43630295065719,21.8028226744916,2.14938387860799));
#91938=CARTESIAN_POINT('Ctrl Pts',(-9.42263843260034,21.8020129959342,2.15518889263071));
#91939=CARTESIAN_POINT('Ctrl Pts',(-9.41752271992285,21.8017101241068,2.15739674013288));
#91940=CARTESIAN_POINT('Ctrl Pts',(-9.4078449461099,21.801137604408,2.16163921446936));
#91941=CARTESIAN_POINT('Ctrl Pts',(-9.40328046015303,21.8008677668167,2.16366808325395));
#91942=CARTESIAN_POINT('Ctrl Pts',(-9.39293606278555,21.8002566312356,2.16832963429322));
#91943=CARTESIAN_POINT('Ctrl Pts',(-9.38716270035744,21.79991582688,2.17097666210453));
#91944=CARTESIAN_POINT('Ctrl Pts',(-9.37226854095461,21.7990372387027,2.17792317343375));
#91945=CARTESIAN_POINT('Ctrl Pts',(-9.36317453618332,21.7985014031581,2.18227952303064));
#91946=CARTESIAN_POINT('Ctrl Pts',(-9.30256201159752,21.794932829543,2.21208910806198));
#91947=CARTESIAN_POINT('Ctrl Pts',(-9.25253335444661,21.7920039920107,2.2404648478235));
#91948=CARTESIAN_POINT('Ctrl Pts',(-9.12479569959115,21.7844232288834,2.32321496626206));
#91949=CARTESIAN_POINT('Ctrl Pts',(-9.05048359323231,21.7799135396216,2.38231325186151));
#91950=CARTESIAN_POINT('Ctrl Pts',(-8.94389758331957,21.772597821708,2.48543085389492));
#91951=CARTESIAN_POINT('Ctrl Pts',(-8.90746900772402,21.7699041182703,2.5247678055725));
#91952=CARTESIAN_POINT('Ctrl Pts',(-8.86663719053606,21.7665200602163,2.57402515624088));
#91953=CARTESIAN_POINT('Ctrl Pts',(-8.86007799601037,21.7659641256341,2.58211194492431));
#91954=CARTESIAN_POINT('Ctrl Pts',(-8.85105665554726,21.7651810341626,2.59348013883958));
#91955=CARTESIAN_POINT('Ctrl Pts',(-8.84852101844007,21.7649588460993,2.59670313758938));
#91956=CARTESIAN_POINT('Ctrl Pts',(-8.84423396366924,21.7645795469579,2.6021997127614));
#91957=CARTESIAN_POINT('Ctrl Pts',(-8.84247560453653,21.7644229202751,2.60446788986445));
#91958=CARTESIAN_POINT('Ctrl Pts',(-8.83911747621278,21.7641217335744,2.60882608692546));
#91959=CARTESIAN_POINT('Ctrl Pts',(-8.83751665971492,21.7639772529974,2.61091526797984));
#91960=CARTESIAN_POINT('Ctrl Pts',(-8.83327839690617,21.7635923442451,2.61647752188809));
#91961=CARTESIAN_POINT('Ctrl Pts',(-8.83065084553238,21.7633512408194,2.61995805645383));
#91962=CARTESIAN_POINT('Ctrl Pts',(-8.82130131040381,21.7624845753519,2.63245853469706));
#91963=CARTESIAN_POINT('Ctrl Pts',(-8.81466799124114,21.7618533224432,2.64154393933367));
#91964=CARTESIAN_POINT('Ctrl Pts',(-8.75731012902373,21.7562554192069,2.72203716607972));
#91965=CARTESIAN_POINT('Ctrl Pts',(-8.71299048644277,21.750962485745,2.79778323833706));
#91966=CARTESIAN_POINT('Ctrl Pts',(-8.63190202096214,21.7394924479113,2.97015808004315));
#91967=CARTESIAN_POINT('Ctrl Pts',(-8.59803190595747,21.7333671077691,3.06766204631052));
#91968=CARTESIAN_POINT('Ctrl Pts',(-8.56997984079086,21.726417681113,3.18806684238377));
#91969=CARTESIAN_POINT('Ctrl Pts',(-8.56571455021362,21.7252684047315,3.20830622112898));
#91970=CARTESIAN_POINT('Ctrl Pts',(-8.56046192414569,21.7237128192393,3.23614241599987));
#91971=CARTESIAN_POINT('Ctrl Pts',(-8.5591032104751,21.7232948614451,3.24366595716492));
#91972=CARTESIAN_POINT('Ctrl Pts',(-8.55691644360918,21.7225947730186,3.25634178628154));
#91973=CARTESIAN_POINT('Ctrl Pts',(-8.55605689004874,21.7223116554813,3.26148842366885));
#91974=CARTESIAN_POINT('Ctrl Pts',(-8.55441330065208,21.7217540848904,3.2716641734089));
#91975=CARTESIAN_POINT('Ctrl Pts',(-8.55362793958215,21.7214795937914,3.27669299432882));
#91976=CARTESIAN_POINT('Ctrl Pts',(-8.55195534342973,21.7208765989605,3.28778210446067));
#91977=CARTESIAN_POINT('Ctrl Pts',(-8.55107988310235,21.7205484680752,3.2938440905297));
#91978=CARTESIAN_POINT('Ctrl Pts',(-8.54813705709081,21.7193994443028,3.31516657127676));
#91979=CARTESIAN_POINT('Ctrl Pts',(-8.54627248442591,21.7185848820045,3.33045432602311));
#91980=CARTESIAN_POINT('Ctrl Pts',(-8.5307696184011,21.7108717779644,3.47674211733177));
#91981=CARTESIAN_POINT('Ctrl Pts',(-8.5346320052955,21.7045938192308,3.6089828561549));
#91982=CARTESIAN_POINT('Ctrl Pts',(-8.56443145441309,21.6956674857378,3.78906307213894));
#91983=CARTESIAN_POINT('Ctrl Pts',(-8.57533260239597,21.6931550187792,3.83872796592656));
#91984=CARTESIAN_POINT('Ctrl Pts',(-8.59521657054554,21.689294831275,3.91110046235463));
#91985=CARTESIAN_POINT('Ctrl Pts',(-8.60221936241023,21.6880253834705,3.93431466339828));
#91986=CARTESIAN_POINT('Ctrl Pts',(-8.61153150120847,21.6864268878782,3.96262117768541));
#91987=CARTESIAN_POINT('Ctrl Pts',(-8.61329796498304,21.6861272003435,3.96788950646745));
#91988=CARTESIAN_POINT('Ctrl Pts',(-8.61612462857936,21.6856529337003,3.97616316710048));
#91989=CARTESIAN_POINT('Ctrl Pts',(-8.617164734898,21.6854795083092,3.9791753692756));
#91990=CARTESIAN_POINT('Ctrl Pts',(-8.61913644347883,21.6851527294618,3.98482565490848));
#91991=CARTESIAN_POINT('Ctrl Pts',(-8.62006577670157,21.6849995086646,3.9874644769713));
#91992=CARTESIAN_POINT('Ctrl Pts',(-8.62220416428847,21.6846487744428,3.99348126361423));
#91993=CARTESIAN_POINT('Ctrl Pts',(-8.62341807661731,21.6844509787846,3.9968574545014));
#91994=CARTESIAN_POINT('Ctrl Pts',(-8.62666948528854,21.6839246898652,4.00579704458868));
#91995=CARTESIAN_POINT('Ctrl Pts',(-8.62872835079242,21.6835949931343,4.01135253456713));
#91996=CARTESIAN_POINT('Ctrl Pts',(-8.64348347251496,21.6812576560782,4.05043667013636));
#91997=CARTESIAN_POINT('Ctrl Pts',(-8.65737337855474,21.6791877722604,4.08349889889475));
#91998=CARTESIAN_POINT('Ctrl Pts',(-8.67815530924446,21.6762862395431,4.12828482984927));
#91999=CARTESIAN_POINT('Ctrl Pts',(-8.6840185595466,21.6754861918268,4.14047486141506));
#92000=CARTESIAN_POINT('Ctrl Pts',(-8.69247062771171,21.6743597327681,4.15744099693509));
#92001=CARTESIAN_POINT('Ctrl Pts',(-8.6949184427733,21.6740364957301,4.16228683522756));
#92002=CARTESIAN_POINT('Ctrl Pts',(-8.73762558518917,21.6684493261555,4.24567619112539));
#92003=CARTESIAN_POINT('Ctrl Pts',(-8.78488496736626,21.6630745406304,4.32043825290269));
#92004=CARTESIAN_POINT('Ctrl Pts',(-8.87651407117109,21.6541795756184,4.43994456728132));
#92005=CARTESIAN_POINT('Ctrl Pts',(-8.91755911770016,21.6505840065092,4.48693449851202));
#92006=CARTESIAN_POINT('Ctrl Pts',(-8.97208079597778,21.6462718136731,4.54184486128887));
#92007=CARTESIAN_POINT('Ctrl Pts',(-8.98284569741638,21.6454405151886,4.5523572366306));
#92008=CARTESIAN_POINT('Ctrl Pts',(-8.99866613351974,21.6442471374244,4.56733695801184));
#92009=CARTESIAN_POINT('Ctrl Pts',(-9.00359320981006,21.6438793415426,4.57193806010005));
#92010=CARTESIAN_POINT('Ctrl Pts',(-9.01226549975239,21.643238633391,4.57992513381734));
#92011=CARTESIAN_POINT('Ctrl Pts',(-9.0159967433852,21.642965091333,4.58332604948312));
#92012=CARTESIAN_POINT('Ctrl Pts',(-9.02374566792692,21.642401339232,4.59031589447885));
#92013=CARTESIAN_POINT('Ctrl Pts',(-9.02776572087343,21.6421112456479,4.59390208803307));
#92014=CARTESIAN_POINT('Ctrl Pts',(-9.03813221076957,21.6413691870973,4.60304749932841));
#92015=CARTESIAN_POINT('Ctrl Pts',(-9.04450713301085,21.6409185662689,4.60857422615282));
#92016=CARTESIAN_POINT('Ctrl Pts',(-9.06953990125163,21.6391707844506,4.62989997787011));
#92017=CARTESIAN_POINT('Ctrl Pts',(-9.0885452128395,21.6378903185369,4.64528608538948));
#92018=CARTESIAN_POINT('Ctrl Pts',(-9.23656008033713,21.6282404858106,4.75909503520879));
#92019=CARTESIAN_POINT('Ctrl Pts',(-9.38071950345847,21.6208150097395,4.83590486910357));
#92020=CARTESIAN_POINT('Ctrl Pts',(-9.56406785634892,21.6109769154887,4.89741423471858));
#92021=CARTESIAN_POINT('Ctrl Pts',(-9.59391954024016,21.6093587502289,4.90637895491126));
#92022=CARTESIAN_POINT('Ctrl Pts',(-9.62980857046062,21.6073696085137,4.91591888097632));
#92023=CARTESIAN_POINT('Ctrl Pts',(-9.6355940244763,21.6070476114953,4.91741887053334));
#92024=CARTESIAN_POINT('Ctrl Pts',(-9.64456689962912,21.6065459170461,4.91968669408182));
#92025=CARTESIAN_POINT('Ctrl Pts',(-9.64774805421934,21.6063676055274,4.9204793431988));
#92026=CARTESIAN_POINT('Ctrl Pts',(-9.65363707854226,21.6060366428554,4.92192571414978));
#92027=CARTESIAN_POINT('Ctrl Pts',(-9.65634416634114,21.6058841622806,4.92258239745361));
#92028=CARTESIAN_POINT('Ctrl Pts',(-9.66247058688416,21.605538313492,4.92405003234557));
#92029=CARTESIAN_POINT('Ctrl Pts',(-9.66589095760961,21.6053446897388,4.92485639508078));
#92030=CARTESIAN_POINT('Ctrl Pts',(-9.67472291917828,21.6048433972554,4.92690500711366));
#92031=CARTESIAN_POINT('Ctrl Pts',(-9.68013868450348,21.6045347243183,4.92812878112535));
#92032=CARTESIAN_POINT('Ctrl Pts',(-9.71366088548042,21.6026167781016,4.9355033847289));
#92033=CARTESIAN_POINT('Ctrl Pts',(-9.74193492165365,21.6009673426565,4.9408546929518));
#92034=CARTESIAN_POINT('Ctrl Pts',(-9.87335681296835,21.5932105017247,4.96173623535843));
#92035=CARTESIAN_POINT('Ctrl Pts',(-9.97782037657912,21.5868151459587,4.96704458156094));
#92036=CARTESIAN_POINT('Ctrl Pts',(-10.1347183405296,21.5774708125399,4.95824389699694));
#92037=CARTESIAN_POINT('Ctrl Pts',(-10.1872797823016,21.5743799517944,4.95242949126771));
#92038=CARTESIAN_POINT('Ctrl Pts',(-10.2695763298698,21.5696289932391,4.93878265627349));
#92039=CARTESIAN_POINT('Ctrl Pts',(-10.2995742953442,21.5679156448625,4.93283717432106));
#92040=CARTESIAN_POINT('Ctrl Pts',(-10.3379627827179,21.5657458300829,4.92397024585101));
#92041=CARTESIAN_POINT('Ctrl Pts',(-10.3465418902986,21.5652623794568,4.92190675736069));
#92042=CARTESIAN_POINT('Ctrl Pts',(-10.3604105106826,21.5644831196977,4.91843803443896));
#92043=CARTESIAN_POINT('Ctrl Pts',(-10.3657116359412,21.5641857950418,4.91708051790469));
#92044=CARTESIAN_POINT('Ctrl Pts',(-10.375859988453,21.563617599588,4.91442097978208));
#92045=CARTESIAN_POINT('Ctrl Pts',(-10.3807083675487,21.5633465816307,4.91312369547515));
#92046=CARTESIAN_POINT('Ctrl Pts',(-10.3917557101348,21.5627300095916,4.9101067676736));
#92047=CARTESIAN_POINT('Ctrl Pts',(-10.3979502253396,21.5623849747295,4.90837113454388));
#92048=CARTESIAN_POINT('Ctrl Pts',(-10.4143092511725,21.5614754990796,4.90367097117169));
#92049=CARTESIAN_POINT('Ctrl Pts',(-10.4244534816599,21.5609133028475,4.90063685537803));
#92050=CARTESIAN_POINT('Ctrl Pts',(-10.5063542370379,21.5563869209241,4.87516901454287));
#92051=CARTESIAN_POINT('Ctrl Pts',(-10.576321264917,21.5526068965931,4.84734557270202));
#92052=CARTESIAN_POINT('Ctrl Pts',(-10.7069695619628,21.5454541244459,4.78334211235957));
#92053=CARTESIAN_POINT('Ctrl Pts',(-10.7677810567725,21.5420785078132,4.74791225350963));
#92054=CARTESIAN_POINT('Ctrl Pts',(-10.8626912784255,21.5364304167027,4.683043357448));
#92055=CARTESIAN_POINT('Ctrl Pts',(-10.8983962151186,21.5342059077369,4.65616242828577));
#92056=CARTESIAN_POINT('Ctrl Pts',(-10.9500459305302,21.5307471609263,4.61343842373267));
#92057=CARTESIAN_POINT('Ctrl Pts',(-10.9669483947721,21.5295734454881,4.59879164848176));
#92058=CARTESIAN_POINT('Ctrl Pts',(-10.9875193033697,21.5280825743114,4.58012370661639));
#92059=CARTESIAN_POINT('Ctrl Pts',(-10.9915105942422,21.5277902961085,4.57646102380593));
#92060=CARTESIAN_POINT('Ctrl Pts',(-10.9977947669935,21.5273251518988,4.57062963387479));
#92061=CARTESIAN_POINT('Ctrl Pts',(-11.0001011667095,21.527153366573,4.56847548681762));
#92062=CARTESIAN_POINT('Ctrl Pts',(-11.0044436706111,21.5268278618063,4.56439326650314));
#92063=CARTESIAN_POINT('Ctrl Pts',(-11.0064812111677,21.526674261757,4.5624667920955));
#92064=CARTESIAN_POINT('Ctrl Pts',(-11.0111504217753,21.5263202823811,4.55802661542949));
#92065=CARTESIAN_POINT('Ctrl Pts',(-11.0137782615063,21.5261196015584,4.55550894374324));
#92066=CARTESIAN_POINT('Ctrl Pts',(-11.0207859005637,21.5255805939359,4.54874477863558));
#92067=CARTESIAN_POINT('Ctrl Pts',(-11.0251485363479,21.5252409716897,4.54448070412508));
#92068=CARTESIAN_POINT('Ctrl Pts',(-11.0583035737339,21.5226296032565,4.51166688618668));
#92069=CARTESIAN_POINT('Ctrl Pts',(-11.0859226772531,21.5202783802973,4.48196115951001));
#92070=CARTESIAN_POINT('Ctrl Pts',(-11.1690659715518,21.5127257572951,4.38473377712412));
#92071=CARTESIAN_POINT('Ctrl Pts',(-11.2197981970836,21.5073961710961,4.31336446490505));
#92072=CARTESIAN_POINT('Ctrl Pts',(-11.3016584975888,21.49772045675,4.17315479174647));
#92073=CARTESIAN_POINT('Ctrl Pts',(-11.3344301351383,21.493354600281,4.10559972713085));
#92074=CARTESIAN_POINT('Ctrl Pts',(-11.3679448482733,21.4882409043851,4.02041639713847));
#92075=CARTESIAN_POINT('Ctrl Pts',(-11.3737445244045,21.4873246453876,4.00490825665599));
#92076=CARTESIAN_POINT('Ctrl Pts',(-11.3816219359288,21.4860330771165,3.98270295460613));
#92077=CARTESIAN_POINT('Ctrl Pts',(-11.3839164890509,21.4856506608306,3.97608451975304));
#92078=CARTESIAN_POINT('Ctrl Pts',(-11.3877972302376,21.4849928836044,3.96462569746802));
#92079=CARTESIAN_POINT('Ctrl Pts',(-11.3894058160064,21.4847167923813,3.95979307341665));
#92080=CARTESIAN_POINT('Ctrl Pts',(-11.3924412842639,21.4841890668592,3.95051230878689));
#92081=CARTESIAN_POINT('Ctrl Pts',(-11.3938721597778,21.4839373049291,3.94606554830478));
#92082=CARTESIAN_POINT('Ctrl Pts',(-11.397184965174,21.4833472282806,3.93559867447005));
#92083=CARTESIAN_POINT('Ctrl Pts',(-11.3990493246379,21.4830094872735,3.92957306832552));
#92084=CARTESIAN_POINT('Ctrl Pts',(-11.40535960199,21.4818462163973,3.90870136534874));
#92085=CARTESIAN_POINT('Ctrl Pts',(-11.4096087122984,21.4810270358764,3.89379654555211));
#92086=CARTESIAN_POINT('Ctrl Pts',(-11.4467308269554,21.4735129762302,3.75527256097526));
#92087=CARTESIAN_POINT('Ctrl Pts',(-11.4634999999999,21.4673972845276,3.62791798927615));
#92088=CARTESIAN_POINT('Ctrl Pts',(-11.4635,21.4611504451332,3.50000000000115));
#92089=CARTESIAN_POINT('Ctrl Pts',(-11.4635,21.3891087006547,3.49999999989906));
#92090=CARTESIAN_POINT('Ctrl Pts',(-11.4635000000082,21.396299059564,3.61942455324135));
#92091=CARTESIAN_POINT('Ctrl Pts',(-11.4488819064457,21.4034476858667,3.73842431250034));
#92092=CARTESIAN_POINT('Ctrl Pts',(-11.4160045137088,21.4110348061065,3.87017551169755));
#92093=CARTESIAN_POINT('Ctrl Pts',(-11.4117876336054,21.411938487072,3.88594611052557));
#92094=CARTESIAN_POINT('Ctrl Pts',(-11.4055378386873,21.4131874124851,3.90784460544997));
#92095=CARTESIAN_POINT('Ctrl Pts',(-11.4037270149434,21.4135397598175,3.91403418646385));
#92096=CARTESIAN_POINT('Ctrl Pts',(-11.4005235009538,21.4141470489058,3.9247214841989));
#92097=CARTESIAN_POINT('Ctrl Pts',(-11.3991499195689,21.4144026044021,3.92922478860827));
#92098=CARTESIAN_POINT('Ctrl Pts',(-11.3962524959583,21.4149318192255,3.93856231961155));
#92099=CARTESIAN_POINT('Ctrl Pts',(-11.3947252210479,21.4152053629606,3.94339542094852));
#92100=CARTESIAN_POINT('Ctrl Pts',(-11.3910732724636,21.4158469655779,3.95474651993349));
#92101=CARTESIAN_POINT('Ctrl Pts',(-11.3889278380108,21.4162143426062,3.96125774760939));
#92102=CARTESIAN_POINT('Ctrl Pts',(-11.3817252394348,21.417417140065,3.98261109456256));
#92103=CARTESIAN_POINT('Ctrl Pts',(-11.3764752066174,21.4182462506883,3.99738731033037));
#92104=CARTESIAN_POINT('Ctrl Pts',(-11.3292636805123,21.4253175255697,4.12378725111242));
#92105=CARTESIAN_POINT('Ctrl Pts',(-11.2740437030693,21.4310658466671,4.22997794860489));
#92106=CARTESIAN_POINT('Ctrl Pts',(-11.1623467181847,21.4406756934843,4.39268199255192));
#92107=CARTESIAN_POINT('Ctrl Pts',(-11.1130695486394,21.4445030057006,4.45341727426985));
#92108=CARTESIAN_POINT('Ctrl Pts',(-11.0513696799749,21.4492189029787,4.51812694890517));
#92109=CARTESIAN_POINT('Ctrl Pts',(-11.0434542517006,21.4498227039456,4.52623773902712));
#92110=CARTESIAN_POINT('Ctrl Pts',(-11.0323535385172,21.4506692231751,4.53735122601047));
#92111=CARTESIAN_POINT('Ctrl Pts',(-11.0292475780893,21.4509060501968,4.54043299476479));
#92112=CARTESIAN_POINT('Ctrl Pts',(-11.0242488139958,21.4512872500056,4.54534853625745));
#92113=CARTESIAN_POINT('Ctrl Pts',(-11.0223647703632,21.4514309357564,4.54719122958526));
#92114=CARTESIAN_POINT('Ctrl Pts',(-11.0184194178687,21.4517318750698,4.55102919534127));
#92115=CARTESIAN_POINT('Ctrl Pts',(-11.0163572151585,21.4518892035245,4.55302349967875));
#92116=CARTESIAN_POINT('Ctrl Pts',(-11.011339869751,21.4522720279664,4.55784718001797));
#92117=CARTESIAN_POINT('Ctrl Pts',(-11.0083787098952,21.4524980011133,4.56067024329916));
#92118=CARTESIAN_POINT('Ctrl Pts',(-10.9978878319446,21.4532985824309,4.57058823076288));
#92119=CARTESIAN_POINT('Ctrl Pts',(-10.990294936522,21.4538780069786,4.57761552107226));
#92120=CARTESIAN_POINT('Ctrl Pts',(-10.9106348595005,21.4599508610021,4.64978870188361));
#92121=CARTESIAN_POINT('Ctrl Pts',(-10.8323310993438,21.4658523484903,4.70768048372725));
#92122=CARTESIAN_POINT('Ctrl Pts',(-10.6636701055125,21.4776595746329,4.80813222026336));
#92123=CARTESIAN_POINT('Ctrl Pts',(-10.5735132042922,21.4835265031393,4.85009488892858));
#92124=CARTESIAN_POINT('Ctrl Pts',(-10.4635806071914,21.4900367973308,4.88824339932996));
#92125=CARTESIAN_POINT('Ctrl Pts',(-10.4472708446001,21.4909876635815,4.89358370467582));
#92126=CARTESIAN_POINT('Ctrl Pts',(-10.4238786922607,21.4923306146242,4.90079000135828));
#92127=CARTESIAN_POINT('Ctrl Pts',(-10.4168708189894,21.4927303040876,4.90289147714915));
#92128=CARTESIAN_POINT('Ctrl Pts',(-10.4049500007657,21.4934058084196,4.90636900292444));
#92129=CARTESIAN_POINT('Ctrl Pts',(-10.4000451310839,21.4936824923587,4.90777205879353));
#92130=CARTESIAN_POINT('Ctrl Pts',(-10.3901188711676,21.4942399346962,4.91055543473153));
#92131=CARTESIAN_POINT('Ctrl Pts',(-10.3850972484291,21.4945206543603,4.91193465794634));
#92132=CARTESIAN_POINT('Ctrl Pts',(-10.3727400762796,21.4952083409809,4.9152578113658));
#92133=CARTESIAN_POINT('Ctrl Pts',(-10.3653965184493,21.4956143349415,4.91717155783715));
#92134=CARTESIAN_POINT('Ctrl Pts',(-10.3383769547443,21.4970985724304,4.92398892728958));
#92135=CARTESIAN_POINT('Ctrl Pts',(-10.318614034365,21.4981655994218,4.9285407165118));
#92136=CARTESIAN_POINT('Ctrl Pts',(-10.2109951546144,21.5038854037379,4.95098288513548));
#92137=CARTESIAN_POINT('Ctrl Pts',(-10.121729655085,21.5082887873556,4.96118249698326));
#92138=CARTESIAN_POINT('Ctrl Pts',(-9.92992853709821,21.5176239561816,4.96538836637921));
#92139=CARTESIAN_POINT('Ctrl Pts',(-9.82783213578223,21.5225206155021,4.95692344151619));
#92140=CARTESIAN_POINT('Ctrl Pts',(-9.71697043832576,21.5284816183374,4.9359110733186));
#92141=CARTESIAN_POINT('Ctrl Pts',(-9.706498229179,21.529051339805,4.93380718389019));
#92142=CARTESIAN_POINT('Ctrl Pts',(-9.69187516239833,21.5298573509298,4.93070246801058));
#92143=CARTESIAN_POINT('Ctrl Pts',(-9.68770398137463,21.5300884602971,4.92979777008576));
#92144=CARTESIAN_POINT('Ctrl Pts',(-9.68098368093543,21.5304628254161,4.928309377099));
#92145=CARTESIAN_POINT('Ctrl Pts',(-9.67843203204906,21.5306054394769,4.92773706623591));
#92146=CARTESIAN_POINT('Ctrl Pts',(-9.67306558853104,21.5309063912656,4.92651830749124));
#92147=CARTESIAN_POINT('Ctrl Pts',(-9.67025116274484,21.5310648161495,4.92587036399165));
#92148=CARTESIAN_POINT('Ctrl Pts',(-9.66335892770833,21.5314542005217,4.92426212100243));
#92149=CARTESIAN_POINT('Ctrl Pts',(-9.65928330527601,21.5316856757874,4.92329263818901));
#92150=CARTESIAN_POINT('Ctrl Pts',(-9.64453861928741,21.5325273759645,4.91971830705854));
#92151=CARTESIAN_POINT('Ctrl Pts',(-9.63389507014034,21.5331430820803,4.91701094919041));
#92152=CARTESIAN_POINT('Ctrl Pts',(-9.56569500565599,21.537136145647,4.89884351244477));
#92153=CARTESIAN_POINT('Ctrl Pts',(-9.50910243901627,21.5406674438585,4.88000083132761));
#92154=CARTESIAN_POINT('Ctrl Pts',(-9.39369499913671,21.5481262414772,4.83357666379679));
#92155=CARTESIAN_POINT('Ctrl Pts',(-9.33523932841442,21.5520520350159,4.80542181671792));
#92156=CARTESIAN_POINT('Ctrl Pts',(-9.20969095279338,21.5606384150614,4.73432540275917));
#92157=CARTESIAN_POINT('Ctrl Pts',(-9.14383671507622,21.5652461191646,4.68959455534421));
#92158=CARTESIAN_POINT('Ctrl Pts',(-9.07362143403438,21.5702425261918,4.63303526267893));
#92159=CARTESIAN_POINT('Ctrl Pts',(-9.06538328134277,21.5708303520168,4.6262494180452));
#92160=CARTESIAN_POINT('Ctrl Pts',(-9.05227971458969,21.5717681162534,4.61521308685246));
#92161=CARTESIAN_POINT('Ctrl Pts',(-9.0473670359062,21.5721203338421,4.61101953450838));
#92162=CARTESIAN_POINT('Ctrl Pts',(-9.03868272230908,21.5727441568008,4.60350649411708));
#92163=CARTESIAN_POINT('Ctrl Pts',(-9.03490013913785,21.5730162815768,4.60019986838014));
#92164=CARTESIAN_POINT('Ctrl Pts',(-9.0270405597478,21.5735826044486,4.59325752521818));
#92165=CARTESIAN_POINT('Ctrl Pts',(-9.02296673562821,21.5738766521926,4.58961832319621));
#92166=CARTESIAN_POINT('Ctrl Pts',(-9.012402450437,21.5746405733763,4.58007422033769));
#92167=CARTESIAN_POINT('Ctrl Pts',(-9.00594449612028,21.5751089442167,4.57413355830013));
#92168=CARTESIAN_POINT('Ctrl Pts',(-8.97759692328527,21.577171583483,4.54758204285154));
#92169=CARTESIAN_POINT('Ctrl Pts',(-8.95629125461885,21.5787395449588,4.52635686198655));
#92170=CARTESIAN_POINT('Ctrl Pts',(-8.90027272691854,21.5829291137524,4.46700021312388));
#92171=CARTESIAN_POINT('Ctrl Pts',(-8.86689569467471,21.5854990417828,4.42766624861666));
#92172=CARTESIAN_POINT('Ctrl Pts',(-8.77414649587277,21.5930211415696,4.30586928039764));
#92173=CARTESIAN_POINT('Ctrl Pts',(-8.72120955576969,21.5978324447365,4.21891187167456));
#92174=CARTESIAN_POINT('Ctrl Pts',(-8.66355289207488,21.6046531457452,4.09735365213714));
#92175=CARTESIAN_POINT('Ctrl Pts',(-8.65041864478409,21.6063621962531,4.06705564722612));
#92176=CARTESIAN_POINT('Ctrl Pts',(-8.63620402408808,21.6084368345276,4.03096718776663));
#92177=CARTESIAN_POINT('Ctrl Pts',(-8.63411891939832,21.6087475260663,4.02558014597852));
#92178=CARTESIAN_POINT('Ctrl Pts',(-8.63079238850586,21.6092538856038,4.01683227654651));
#92179=CARTESIAN_POINT('Ctrl Pts',(-8.629531295767,21.6094484246239,4.01347893395347));
#92180=CARTESIAN_POINT('Ctrl Pts',(-8.62730939922858,21.6097958659071,4.00750424542958));
#92181=CARTESIAN_POINT('Ctrl Pts',(-8.62634376999786,21.6099484803674,4.00488474547713));
#92182=CARTESIAN_POINT('Ctrl Pts',(-8.62427682545913,21.6102786854143,3.9992278391402));
#92183=CARTESIAN_POINT('Ctrl Pts',(-8.62317808708969,21.6104564187353,3.99618958882145));
#92184=CARTESIAN_POINT('Ctrl Pts',(-8.62015035700992,21.6109523238718,3.98772976874868));
#92185=CARTESIAN_POINT('Ctrl Pts',(-8.61824328994696,21.6112717419276,3.98230048367763));
#92186=CARTESIAN_POINT('Ctrl Pts',(-8.60749992970006,21.6131117352009,3.95112813176044));
#92187=CARTESIAN_POINT('Ctrl Pts',(-8.59935165171072,21.6146683185928,3.92515532070323));
#92188=CARTESIAN_POINT('Ctrl Pts',(-8.57510736430442,21.6198387214066,3.83959151156066));
#92189=CARTESIAN_POINT('Ctrl Pts',(-8.56205598451551,21.62355128336,3.77920893705136));
#92190=CARTESIAN_POINT('Ctrl Pts',(-8.53569718837198,21.6341987549722,3.60438159422973));
#92191=CARTESIAN_POINT('Ctrl Pts',(-8.53202029854842,21.6410713840203,3.48892978470404));
#92192=CARTESIAN_POINT('Ctrl Pts',(-8.54334599968473,21.6484386677781,3.35763137325285));
#92193=CARTESIAN_POINT('Ctrl Pts',(-8.54506075021879,21.6493611657897,3.34106128796563));
#92194=CARTESIAN_POINT('Ctrl Pts',(-8.54783797473983,21.6506316787789,3.31806591235982));
#92195=CARTESIAN_POINT('Ctrl Pts',(-8.54866094100329,21.6509871206973,3.31161343572553));
#92196=CARTESIAN_POINT('Ctrl Pts',(-8.55015559525731,21.6515982908575,3.30048620793536));
#92197=CARTESIAN_POINT('Ctrl Pts',(-8.55080693787177,21.6518546514241,3.29580886259368));
#92198=CARTESIAN_POINT('Ctrl Pts',(-8.55220296095287,21.6523841904108,3.2861271863853));
#92199=CARTESIAN_POINT('Ctrl Pts',(-8.5529509755268,21.6526572605281,3.2811233947266));
#92200=CARTESIAN_POINT('Ctrl Pts',(-8.55476508418211,21.6532954264855,3.26940398435029));
#92201=CARTESIAN_POINT('Ctrl Pts',(-8.55585206773396,21.6536598617201,3.2626916853773));
#92202=CARTESIAN_POINT('Ctrl Pts',(-8.5595474060199,21.654843001421,3.24083863497887));
#92203=CARTESIAN_POINT('Ctrl Pts',(-8.56234744738258,21.6556556829691,3.2257310623716));
#92204=CARTESIAN_POINT('Ctrl Pts',(-8.57820690049982,21.6598620696137,3.14709348702723));
#92205=CARTESIAN_POINT('Ctrl Pts',(-8.59524139441734,21.6631279102112,3.08443638661618));
#92206=CARTESIAN_POINT('Ctrl Pts',(-8.64832388837808,21.6711603447862,2.93042560695165));
#92207=CARTESIAN_POINT('Ctrl Pts',(-8.6894993367167,21.67581103413,2.84119087886284));
#92208=CARTESIAN_POINT('Ctrl Pts',(-8.74716094007279,21.6815026878103,2.74338440508356));
#92209=CARTESIAN_POINT('Ctrl Pts',(-8.75525056029391,21.6822869272086,2.730148276203));
#92210=CARTESIAN_POINT('Ctrl Pts',(-8.77821095889576,21.6844811522371,2.69388902718335));
#92211=CARTESIAN_POINT('Ctrl Pts',(-8.79351969635526,21.6859093181553,2.67115233702656));
#92212=CARTESIAN_POINT('Ctrl Pts',(-8.81263598908858,21.6876694369555,2.6444131599741));
#92213=CARTESIAN_POINT('Ctrl Pts',(-8.81584016799393,21.6879637192051,2.63998393874469));
#92214=CARTESIAN_POINT('Ctrl Pts',(-8.82112963502436,21.6884485014838,2.63275777127744));
#92215=CARTESIAN_POINT('Ctrl Pts',(-8.82320027096488,21.6886380247415,2.62995010607206));
#92216=CARTESIAN_POINT('Ctrl Pts',(-8.82694193964282,21.6889800981769,2.62491440790014));
#92217=CARTESIAN_POINT('Ctrl Pts',(-8.82860931044412,21.689132396177,2.62268371798023));
#92218=CARTESIAN_POINT('Ctrl Pts',(-8.83226681894093,21.6894661841141,2.61781954033371));
#92219=CARTESIAN_POINT('Ctrl Pts',(-8.83425947728678,21.6896478454222,2.61518805454251));
#92220=CARTESIAN_POINT('Ctrl Pts',(-8.83994636165077,21.690165697717,2.6077305653912));
#92221=CARTESIAN_POINT('Ctrl Pts',(-8.84366172616329,21.690503315778,2.6029208610141));
#92222=CARTESIAN_POINT('Ctrl Pts',(-8.86783893013152,21.6926950256579,2.57202215175352));
#92223=CARTESIAN_POINT('Ctrl Pts',(-8.88915098163295,21.6946026487201,2.546613562257));
#92224=CARTESIAN_POINT('Ctrl Pts',(-8.94321995279271,21.6993405190733,2.48642774225776));
#92225=CARTESIAN_POINT('Ctrl Pts',(-8.97685263418257,21.702203688261,2.45248777621627));
#92226=CARTESIAN_POINT('Ctrl Pts',(-9.10321776134156,21.7125115776972,2.33686951608614));
#92227=CARTESIAN_POINT('Ctrl Pts',(-9.20456201505614,21.7199226053434,2.26534213100808));
#92228=CARTESIAN_POINT('Ctrl Pts',(-9.32783209949298,21.7277166016019,2.19989288638051));
#92229=CARTESIAN_POINT('Ctrl Pts',(-9.34208462899249,21.7286019830116,2.19262263041452));
#92230=CARTESIAN_POINT('Ctrl Pts',(-9.36219656264053,21.7298298692306,2.18277568021352));
#92231=CARTESIAN_POINT('Ctrl Pts',(-9.36795763769513,21.7301791683883,2.18000167143456));
#92232=CARTESIAN_POINT('Ctrl Pts',(-9.3779793532746,21.7307826421209,2.17525677982484));
#92233=CARTESIAN_POINT('Ctrl Pts',(-9.3822316073647,21.7310374122636,2.17326849056468));
#92234=CARTESIAN_POINT('Ctrl Pts',(-9.39110404444629,21.7315663518774,2.16917177830147));
#92235=CARTESIAN_POINT('Ctrl Pts',(-9.3957257892238,21.7318403984058,2.16706687360271));
#92236=CARTESIAN_POINT('Ctrl Pts',(-9.40666453160325,21.7324855602976,2.16215357320406));
#92237=CARTESIAN_POINT('Ctrl Pts',(-9.41299068757409,21.7328559717701,2.15936578101823));
#92238=CARTESIAN_POINT('Ctrl Pts',(-9.43403285327849,21.734079284786,2.15027048020333));
#92239=CARTESIAN_POINT('Ctrl Pts',(-9.44883288276655,21.7349255695233,2.14415951407857));
#92240=CARTESIAN_POINT('Ctrl Pts',(-9.52906867994482,21.7394423698928,2.11256095026807));
#92241=CARTESIAN_POINT('Ctrl Pts',(-9.59617710057964,21.7429615978522,2.09156400279486));
#92242=CARTESIAN_POINT('Ctrl Pts',(-9.76691284034193,21.7515778549495,2.05135787362345));
#92243=CARTESIAN_POINT('Ctrl Pts',(-9.87157660648177,21.7565534298126,2.03835791657455));
#92244=CARTESIAN_POINT('Ctrl Pts',(-10.0060080229752,21.7634070930866,2.03621922122293));
#92245=CARTESIAN_POINT('Ctrl Pts',(-10.035301683776,21.764930057192,2.03663270926404));
#92246=CARTESIAN_POINT('Ctrl Pts',(-10.0701346239639,21.7667963509163,2.03817083469018));
#92247=CARTESIAN_POINT('Ctrl Pts',(-10.0757065422489,21.7670965755635,2.03844880640597));
#92248=CARTESIAN_POINT('Ctrl Pts',(-10.0847940716645,21.767589179462,2.03895426971784));
#92249=CARTESIAN_POINT('Ctrl Pts',(-10.0883107425056,21.7677805279407,2.03916261247456));
#92250=CARTESIAN_POINT('Ctrl Pts',(-10.0946082120583,21.7681245314717,2.0395585242061));
#92251=CARTESIAN_POINT('Ctrl Pts',(-10.0973892590605,21.7682769213467,2.03974134138634));
#92252=CARTESIAN_POINT('Ctrl Pts',(-10.1034360315283,21.768609300604,2.04015618786846));
#92253=CARTESIAN_POINT('Ctrl Pts',(-10.1067014622168,21.7687894504287,2.04039122845712));
#92254=CARTESIAN_POINT('Ctrl Pts',(-10.1159018366542,21.7692988184276,2.04108449595121));
#92255=CARTESIAN_POINT('Ctrl Pts',(-10.1218347422387,21.7696293924527,2.04156797320136));
#92256=CARTESIAN_POINT('Ctrl Pts',(-10.1583232370984,21.7716747568578,2.04476564937557));
#92257=CARTESIAN_POINT('Ctrl Pts',(-10.1887881843106,21.7734353545049,2.04840363262481));
#92258=CARTESIAN_POINT('Ctrl Pts',(-10.3697689285931,21.7841235796752,2.07580881393421));
#92259=CARTESIAN_POINT('Ctrl Pts',(-10.5159487183711,21.7935825196164,2.12200826181782));
#92260=CARTESIAN_POINT('Ctrl Pts',(-10.6817707313447,21.8041691130149,2.20458562574347));
#92261=CARTESIAN_POINT('Ctrl Pts',(-10.7106547921966,21.80601341701,2.22020324260207));
#92262=CARTESIAN_POINT('Ctrl Pts',(-10.7469615037909,21.808333028399,2.24144287583651));
#92263=CARTESIAN_POINT('Ctrl Pts',(-10.7548879323417,21.8088395520228,2.24618113827204));
#92264=CARTESIAN_POINT('Ctrl Pts',(-10.7675935307528,21.8096517765627,2.25394046005246));
#92265=CARTESIAN_POINT('Ctrl Pts',(-10.7724008833816,21.8099591637388,2.2569146923277));
#92266=CARTESIAN_POINT('Ctrl Pts',(-10.7813297440851,21.8105302554633,2.26251063071585));
#92267=CARTESIAN_POINT('Ctrl Pts',(-10.7854555803099,21.8107942135645,2.26512525321639));
#92268=CARTESIAN_POINT('Ctrl Pts',(-10.7936026256696,21.8113156044262,2.2703455441182));
#92269=CARTESIAN_POINT('Ctrl Pts',(-10.797624279808,21.8115730624537,2.27295040143109));
#92270=CARTESIAN_POINT('Ctrl Pts',(-10.8101128630608,21.8123728649195,2.28112669773267));
#92271=CARTESIAN_POINT('Ctrl Pts',(-10.8185348602932,21.8129126752935,2.28676644157736));
#92272=CARTESIAN_POINT('Ctrl Pts',(-10.8661469664403,21.815967985095,2.31937109987882));
#92273=CARTESIAN_POINT('Ctrl Pts',(-10.9040644797114,21.8184138817216,2.34814793507277));
#92274=CARTESIAN_POINT('Ctrl Pts',(-11.0289642439808,21.8266163543261,2.45291256216595));
#92275=CARTESIAN_POINT('Ctrl Pts',(-11.1083182141848,21.8320574296612,2.53730139872324));
#92276=CARTESIAN_POINT('Ctrl Pts',(-11.1863610599694,21.8385838297982,2.64289357858589));
#92277=CARTESIAN_POINT('Ctrl Pts',(-11.1955831183539,21.8393782718541,2.65580513673452));
#92278=CARTESIAN_POINT('Ctrl Pts',(-11.2242499692351,21.8419316305723,2.69735295202304));
#92279=CARTESIAN_POINT('Ctrl Pts',(-11.242888416667,21.8437200462267,2.72652841387841));
#92280=CARTESIAN_POINT('Ctrl Pts',(-11.2634485713923,21.845883648014,2.7613768014552));
#92281=CARTESIAN_POINT('Ctrl Pts',(-11.2663930179554,21.8461984518695,2.76643661230873));
#92282=CARTESIAN_POINT('Ctrl Pts',(-11.2711019299935,21.8467102080988,2.77464137372456));
#92283=CARTESIAN_POINT('Ctrl Pts',(-11.2728852969587,21.8469059918271,2.77777546887162));
#92284=CARTESIAN_POINT('Ctrl Pts',(-11.2760299051731,21.8472547940099,2.78334964032118));
#92285=CARTESIAN_POINT('Ctrl Pts',(-11.2773957614572,21.847407515856,2.78578705877666));
#92286=CARTESIAN_POINT('Ctrl Pts',(-11.2803184063214,21.8477369619707,2.79103782431816));
#92287=CARTESIAN_POINT('Ctrl Pts',(-11.2818728826596,21.8479138224963,2.79385235226335));
#92288=CARTESIAN_POINT('Ctrl Pts',(-11.2861494166674,21.848404893105,2.80165608051859));
#92289=CARTESIAN_POINT('Ctrl Pts',(-11.2888516748809,21.8487203110767,2.80665599457686));
#92290=CARTESIAN_POINT('Ctrl Pts',(-11.3037983379101,21.8504933316307,2.83470071834496));
#92291=CARTESIAN_POINT('Ctrl Pts',(-11.3154530729182,21.8519840091943,2.85805274384681));
#92292=CARTESIAN_POINT('Ctrl Pts',(-11.3507307212526,21.856831431449,2.93373630265889));
#92293=CARTESIAN_POINT('Ctrl Pts',(-11.371900796309,21.8602748106418,2.98714960778562));
#92294=CARTESIAN_POINT('Ctrl Pts',(-11.4216525001829,21.8698378809376,3.13801905024715));
#92295=CARTESIAN_POINT('Ctrl Pts',(-11.4433252705287,21.8759378400675,3.2374295162171));
#92296=CARTESIAN_POINT('Ctrl Pts',(-11.4563522824748,21.8826644899865,3.35460500502699));
#92297=CARTESIAN_POINT('Ctrl Pts',(-11.457891424295,21.8835931616838,3.37094845953377));
#92298=CARTESIAN_POINT('Ctrl Pts',(-11.4605892125318,21.8855578127953,3.40588199734631));
#92299=CARTESIAN_POINT('Ctrl Pts',(-11.4616686110426,21.8865912394602,3.42447541686786));
#92300=CARTESIAN_POINT('Ctrl Pts',(-11.4626808709883,21.8880202694117,3.45048475970381));
#92301=CARTESIAN_POINT('Ctrl Pts',(-11.4629126978096,21.8884250843579,3.45788669104469));
#92302=CARTESIAN_POINT('Ctrl Pts',(-11.4631998693633,21.8890841179268,3.46999153948444));
#92303=CARTESIAN_POINT('Ctrl Pts',(-11.4632887430357,21.8893393724585,3.4746934666286));
#92304=CARTESIAN_POINT('Ctrl Pts',(-11.4634130901352,21.8898174460827,3.48352485824998));
#92305=CARTESIAN_POINT('Ctrl Pts',(-11.4634537519943,21.8900404237556,3.48765419376562));
#92306=CARTESIAN_POINT('Ctrl Pts',(-11.4634923619222,21.8904108660782,3.49453132473303));
#92307=CARTESIAN_POINT('Ctrl Pts',(-11.4635000499487,21.8905586306153,3.49727902167419));
#92308=CARTESIAN_POINT('Ctrl Pts',(-11.4634999997558,21.890706156692,3.5000267339998));
#92309=CARTESIAN_POINT('Origin',(-10.,13.2,3.5));
#92310=CARTESIAN_POINT('',(-11.4635,22.4609791425484,3.50000000009405));
#92311=CARTESIAN_POINT('',(-11.4635,22.3887666433152,3.49999999992021));
#92312=CARTESIAN_POINT('',(-11.4635,13.2,3.5));
#92313=CARTESIAN_POINT('Ctrl Pts',(-11.4635,22.4609791425484,3.50000000009405));
#92314=CARTESIAN_POINT('Ctrl Pts',(-11.4635000000081,22.453441659244,3.3747282078163));
#92315=CARTESIAN_POINT('Ctrl Pts',(-11.4474152347156,22.4459190550057,3.24994710482719));
#92316=CARTESIAN_POINT('Ctrl Pts',(-11.4116157797429,22.438041381404,3.11344773460056));
#92317=CARTESIAN_POINT('Ctrl Pts',(-11.4073613069359,22.4371674081074,3.09823397015972));
#92318=CARTESIAN_POINT('Ctrl Pts',(-11.4010518680726,22.4359531013682,3.07700324437868));
#92319=CARTESIAN_POINT('Ctrl Pts',(-11.3992028591701,22.4356061589841,3.07092663451453));
#92320=CARTESIAN_POINT('Ctrl Pts',(-11.3959221543699,22.4350056870989,3.06039163690732));
#92321=CARTESIAN_POINT('Ctrl Pts',(-11.3945085224811,22.4347515756788,3.05592775880627));
#92322=CARTESIAN_POINT('Ctrl Pts',(-11.3915152500106,22.4342229910092,3.0466310449727));
#92323=CARTESIAN_POINT('Ctrl Pts',(-11.3899317967644,22.4339486461168,3.04179949624827));
#92324=CARTESIAN_POINT('Ctrl Pts',(-11.3861228901722,22.433300981241,3.03037893006756));
#92325=CARTESIAN_POINT('Ctrl Pts',(-11.3838755739913,22.4329283815508,3.02379729739795));
#92326=CARTESIAN_POINT('Ctrl Pts',(-11.3762175534057,22.4316896761417,3.00188164506415));
#92327=CARTESIAN_POINT('Ctrl Pts',(-11.370598120755,22.4308304244476,2.98662151481658));
#92328=CARTESIAN_POINT('Ctrl Pts',(-11.3385840571663,22.4261892278569,2.90395942239943));
#92329=CARTESIAN_POINT('Ctrl Pts',(-11.3074700823218,22.4225686245297,2.83849021529213));
#92330=CARTESIAN_POINT('Ctrl Pts',(-11.2233089145379,22.4142279840878,2.69075364256234));
#92331=CARTESIAN_POINT('Ctrl Pts',(-11.1666182671082,22.4095911108816,2.61097599619532));
#92332=CARTESIAN_POINT('Ctrl Pts',(-11.080156780591,22.4029344120636,2.5119521077098));
#92333=CARTESIAN_POINT('Ctrl Pts',(-11.0570249789257,22.4011844450203,2.48724377881045));
#92334=CARTESIAN_POINT('Ctrl Pts',(-11.028934403681,22.3990636016404,2.45925019332943));
#92335=CARTESIAN_POINT('Ctrl Pts',(-11.0247847753268,22.3987504059162,2.45516397020435));
#92336=CARTESIAN_POINT('Ctrl Pts',(-11.0180334921898,22.3982407936784,2.44859475378917));
#92337=CARTESIAN_POINT('Ctrl Pts',(-11.0154468391288,22.3980455304747,2.4460963519755));
#92338=CARTESIAN_POINT('Ctrl Pts',(-11.0108354820087,22.3976973453942,2.44167506161189));
#92339=CARTESIAN_POINT('Ctrl Pts',(-11.0088144552741,22.3975447167183,2.43974840646015));
#92340=CARTESIAN_POINT('Ctrl Pts',(-11.0044511092749,22.3972151172888,2.43561257730597));
#92341=CARTESIAN_POINT('Ctrl Pts',(-11.0021070449818,22.3970380080602,2.43340537855366));
#92342=CARTESIAN_POINT('Ctrl Pts',(-10.9955881333902,22.396545393596,2.42730755333567));
#92343=CARTESIAN_POINT('Ctrl Pts',(-10.9913978306028,22.3962286677509,2.42343362686863));
#92344=CARTESIAN_POINT('Ctrl Pts',(-10.9676386541808,22.3944329445069,2.40172466305618));
#92345=CARTESIAN_POINT('Ctrl Pts',(-10.9476124065932,22.3929198870113,2.38439979060911));
#92346=CARTESIAN_POINT('Ctrl Pts',(-10.8815916695705,22.3879639938376,2.33034532778859));
#92347=CARTESIAN_POINT('Ctrl Pts',(-10.8338495660784,22.3844305116281,2.29584466678645));
#92348=CARTESIAN_POINT('Ctrl Pts',(-10.683513713846,22.3737101406872,2.2004419133008));
#92349=CARTESIAN_POINT('Ctrl Pts',(-10.5754183893993,22.36657532429,2.14909454356247));
#92350=CARTESIAN_POINT('Ctrl Pts',(-10.4467432856713,22.3589972716214,2.10625657211431));
#92351=CARTESIAN_POINT('Ctrl Pts',(-10.4311229950802,22.358090810679,2.10134589702028));
#92352=CARTESIAN_POINT('Ctrl Pts',(-10.4092327263416,22.3568387600062,2.09486566298727));
#92353=CARTESIAN_POINT('Ctrl Pts',(-10.4030301979122,22.3564860194169,2.09307406349707));
#92354=CARTESIAN_POINT('Ctrl Pts',(-10.3922835171911,22.3558782943612,2.0900467861769));
#92355=CARTESIAN_POINT('Ctrl Pts',(-10.3877449159423,22.3556226934884,2.08879189914717));
#92356=CARTESIAN_POINT('Ctrl Pts',(-10.3783117710276,22.3550936105217,2.08623265329043));
#92357=CARTESIAN_POINT('Ctrl Pts',(-10.3734163480532,22.3548202427096,2.08493175478436));
#92358=CARTESIAN_POINT('Ctrl Pts',(-10.3618912112809,22.3541794477191,2.08193306398127));
#92359=CARTESIAN_POINT('Ctrl Pts',(-10.3552561155014,22.3538126982899,2.08025629834244));
#92360=CARTESIAN_POINT('Ctrl Pts',(-10.3334390649444,22.3526136883446,2.07490539839853));
#92361=CARTESIAN_POINT('Ctrl Pts',(-10.3182097489619,22.3517876834809,2.07142770083017));
#92362=CARTESIAN_POINT('Ctrl Pts',(-10.2374083315898,22.3474589229615,2.05433253577324));
#92363=CARTESIAN_POINT('Ctrl Pts',(-10.171011952334,22.3440930014806,2.04498337836854));
#92364=CARTESIAN_POINT('Ctrl Pts',(-10.0042365798917,22.3358614751077,2.0330785757467));
#92365=CARTESIAN_POINT('Ctrl Pts',(-9.90380919840749,22.3311116340162,2.03623041411179));
#92366=CARTESIAN_POINT('Ctrl Pts',(-9.80171056261637,22.3259191779904,2.04999259914285));
#92367=CARTESIAN_POINT('Ctrl Pts',(-9.79892377927207,22.325777154047,2.05037642236464));
#92368=CARTESIAN_POINT('Ctrl Pts',(-9.76176353436641,22.323879199411,2.05560371404392));
#92369=CARTESIAN_POINT('Ctrl Pts',(-9.72757437776214,22.3220857885533,2.06166027588769));
#92370=CARTESIAN_POINT('Ctrl Pts',(-9.68790742336772,22.319916638834,2.07015217974135));
#92371=CARTESIAN_POINT('Ctrl Pts',(-9.68218678228741,22.3196016383399,2.07141282315864));
#92372=CARTESIAN_POINT('Ctrl Pts',(-9.6729567178659,22.3190896583551,2.07350501289964));
#92373=CARTESIAN_POINT('Ctrl Pts',(-9.66944247320062,22.3188938496718,2.07431526012259));
#92374=CARTESIAN_POINT('Ctrl Pts',(-9.66321175375146,22.3185450665787,2.07577609567074));
#92375=CARTESIAN_POINT('Ctrl Pts',(-9.66049410744754,22.3183923892261,2.07642148046793));
#92376=CARTESIAN_POINT('Ctrl Pts',(-9.65465436318324,22.3180631150732,2.07782597250852));
#92377=CARTESIAN_POINT('Ctrl Pts',(-9.65153295967162,22.3178863826004,2.0785875705009));
#92378=CARTESIAN_POINT('Ctrl Pts',(-9.64290427639287,22.3173958528702,2.08072303197534));
#92379=CARTESIAN_POINT('Ctrl Pts',(-9.63740250363302,22.3170808514538,2.08211865050367));
#92380=CARTESIAN_POINT('Ctrl Pts',(-9.60674267061579,22.3153135029586,2.09008615795025));
#92381=CARTESIAN_POINT('Ctrl Pts',(-9.58175656738352,22.3138283183034,2.09729524541833));
#92382=CARTESIAN_POINT('Ctrl Pts',(-9.50258687594062,22.3090067414711,2.12244085344623));
#92383=CARTESIAN_POINT('Ctrl Pts',(-9.44925630694772,22.3055846408473,2.14288185052232));
#92384=CARTESIAN_POINT('Ctrl Pts',(-9.28622390353112,22.2948152270453,2.21656592506491));
#92385=CARTESIAN_POINT('Ctrl Pts',(-9.18186934398083,22.2875115529114,2.28042963453321));
#92386=CARTESIAN_POINT('Ctrl Pts',(-9.07401023684823,22.2798007898842,2.36658211836855));
#92387=CARTESIAN_POINT('Ctrl Pts',(-9.06155739252458,22.2789067510308,2.37687105026899));
#92388=CARTESIAN_POINT('Ctrl Pts',(-9.04439725640887,22.2776689847781,2.39153401257806));
#92389=CARTESIAN_POINT('Ctrl Pts',(-9.03954487961192,22.2773183172445,2.39573580498567));
#92390=CARTESIAN_POINT('Ctrl Pts',(-9.03118806519789,22.2767131887378,2.40306893188401));
#92391=CARTESIAN_POINT('Ctrl Pts',(-9.02767080347391,22.2764581237428,2.40618545104144));
#92392=CARTESIAN_POINT('Ctrl Pts',(-9.02038881961954,22.2759292380194,2.41270063545079));
#92393=CARTESIAN_POINT('Ctrl Pts',(-9.01662662693801,22.2756555365314,2.41610204220034));
#92394=CARTESIAN_POINT('Ctrl Pts',(-9.00780122110452,22.2750123606508,2.42416488415785));
#92395=CARTESIAN_POINT('Ctrl Pts',(-9.00275303176898,22.2746435787352,2.42884263533469));
#92396=CARTESIAN_POINT('Ctrl Pts',(-8.98619510306899,22.2734308818861,2.44440405381404));
#92397=CARTESIAN_POINT('Ctrl Pts',(-8.97482884685701,22.2725934256301,2.45543918166863));
#92398=CARTESIAN_POINT('Ctrl Pts',(-8.91506276222844,22.2681585679347,2.51537954698643));
#92399=CARTESIAN_POINT('Ctrl Pts',(-8.86997573435278,22.2647060572061,2.56746967331064));
#92400=CARTESIAN_POINT('Ctrl Pts',(-8.7881677395128,22.2579971754959,2.67667201586876));
#92401=CARTESIAN_POINT('Ctrl Pts',(-8.75141949705516,22.2547457390184,2.73354517203979));
#92402=CARTESIAN_POINT('Ctrl Pts',(-8.68650933204098,22.2481577662853,2.85113818227098));
#92403=CARTESIAN_POINT('Ctrl Pts',(-8.65831416395289,22.2448292432934,2.91164934895216));
#92404=CARTESIAN_POINT('Ctrl Pts',(-8.63173297742916,22.2408849473277,2.98064423941501));
#92405=CARTESIAN_POINT('Ctrl Pts',(-8.62917124271432,22.2404946401123,2.98744408602256));
#92406=CARTESIAN_POINT('Ctrl Pts',(-8.62543503637043,22.2399095542948,2.99758982636545));
#92407=CARTESIAN_POINT('Ctrl Pts',(-8.62422187668698,22.2397169894226,3.00092147242979));
#92408=CARTESIAN_POINT('Ctrl Pts',(-8.62207648328155,22.2393717323787,3.00688053734894));
#92409=CARTESIAN_POINT('Ctrl Pts',(-8.6211396383289,22.2392193143046,3.00950624343724));
#92410=CARTESIAN_POINT('Ctrl Pts',(-8.61912527683928,22.2388879693458,3.01520329747373));
#92411=CARTESIAN_POINT('Ctrl Pts',(-8.61805051695262,22.2387088894656,3.01827552509349));
#92412=CARTESIAN_POINT('Ctrl Pts',(-8.6150669486696,22.2382053270773,3.02689628697774));
#92413=CARTESIAN_POINT('Ctrl Pts',(-8.61318127026585,22.2378795359493,3.03245268857771));
#92414=CARTESIAN_POINT('Ctrl Pts',(-8.60212631219366,22.2359244690102,3.06568292527354));
#92415=CARTESIAN_POINT('Ctrl Pts',(-8.59375278051438,22.2342538378012,3.09361263443529));
#92416=CARTESIAN_POINT('Ctrl Pts',(-8.55251670032763,22.2249544152286,3.24774908013765));
#92417=CARTESIAN_POINT('Ctrl Pts',(-8.53580094404877,22.216891924607,3.37766880170769));
#92418=CARTESIAN_POINT('Ctrl Pts',(-8.53660320429906,22.2084222407454,3.5227053797132));
#92419=CARTESIAN_POINT('Ctrl Pts',(-8.53690280324924,22.2075742235998,3.53731390287786));
#92420=CARTESIAN_POINT('Ctrl Pts',(-8.53885701667855,22.204398525715,3.5923682498504));
#92421=CARTESIAN_POINT('Ctrl Pts',(-8.54197063521228,22.2021111663004,3.63274612247325));
#92422=CARTESIAN_POINT('Ctrl Pts',(-8.54793540193512,22.1993236021993,3.68286739055649));
#92423=CARTESIAN_POINT('Ctrl Pts',(-8.54921771331841,22.1987749797223,3.69277666635852));
#92424=CARTESIAN_POINT('Ctrl Pts',(-8.55140304503727,22.1979135307653,3.7084049396166));
#92425=CARTESIAN_POINT('Ctrl Pts',(-8.55223867610499,22.1975986064184,3.71413291937994));
#92426=CARTESIAN_POINT('Ctrl Pts',(-8.55385492399381,22.1970152637434,3.72476959656631));
#92427=CARTESIAN_POINT('Ctrl Pts',(-8.5546266027463,22.1967465695821,3.72967955014046));
#92428=CARTESIAN_POINT('Ctrl Pts',(-8.55639139683723,22.1961530966896,3.7405471452594));
#92429=CARTESIAN_POINT('Ctrl Pts',(-8.55739641309606,22.1958286967279,3.74650278044281));
#92430=CARTESIAN_POINT('Ctrl Pts',(-8.56041170243848,22.1948931580168,3.76372080297073));
#92431=CARTESIAN_POINT('Ctrl Pts',(-8.56251722499109,22.1942850197878,3.7749661976395));
#92432=CARTESIAN_POINT('Ctrl Pts',(-8.58084439463448,22.189335888439,3.86687842309058));
#92433=CARTESIAN_POINT('Ctrl Pts',(-8.60371115984457,22.1852185581605,3.94607416589016));
#92434=CARTESIAN_POINT('Ctrl Pts',(-8.66190954830837,22.1772388119776,4.09819678910241));
#92435=CARTESIAN_POINT('Ctrl Pts',(-8.69686769078022,22.1733841527389,4.17094762434115));
#92436=CARTESIAN_POINT('Ctrl Pts',(-8.74347906824812,22.1687953875763,4.25041379766014));
#92437=CARTESIAN_POINT('Ctrl Pts',(-8.74944188972407,22.1682167027023,4.260309229143));
#92438=CARTESIAN_POINT('Ctrl Pts',(-8.77477775253492,22.1657877883902,4.30125014612093));
#92439=CARTESIAN_POINT('Ctrl Pts',(-8.7951932255784,22.1639013047104,4.33163187179823));
#92440=CARTESIAN_POINT('Ctrl Pts',(-8.82022333003114,22.1616275792496,4.36602229928506));
#92441=CARTESIAN_POINT('Ctrl Pts',(-8.82375198188072,22.1613078790986,4.37080894077497));
#92442=CARTESIAN_POINT('Ctrl Pts',(-8.82946001563113,22.160791831555,4.3784539338452));
#92443=CARTESIAN_POINT('Ctrl Pts',(-8.83162096265796,22.1605967163792,4.38132604263797));
#92444=CARTESIAN_POINT('Ctrl Pts',(-8.83548318118876,22.1602483767575,4.38642013753526));
#92445=CARTESIAN_POINT('Ctrl Pts',(-8.83718027028188,22.1600954426378,4.38864523720031));
#92446=CARTESIAN_POINT('Ctrl Pts',(-8.84082115155021,22.1597675990558,4.39339060717344));
#92447=CARTESIAN_POINT('Ctrl Pts',(-8.84276675543991,22.159592566684,4.39590936872275));
#92448=CARTESIAN_POINT('Ctrl Pts',(-8.84812046434553,22.1591114142786,4.40279369671992));
#92449=CARTESIAN_POINT('Ctrl Pts',(-8.85154512261252,22.1588041628705,4.40714624845664));
#92450=CARTESIAN_POINT('Ctrl Pts',(-8.86993469438994,22.1571575962457,4.43024733951644));
#92451=CARTESIAN_POINT('Ctrl Pts',(-8.88533337436298,22.15579038881,4.44864423474454));
#92452=CARTESIAN_POINT('Ctrl Pts',(-8.93416628567594,22.151511040341,4.50415407153844));
#92453=CARTESIAN_POINT('Ctrl Pts',(-8.96905260893748,22.1485319418415,4.53993931794324));
#92454=CARTESIAN_POINT('Ctrl Pts',(-9.09811103967232,22.1379645422718,4.65943540509156));
#92455=CARTESIAN_POINT('Ctrl Pts',(-9.20120310006712,22.1303614756987,4.73273211345151));
#92456=CARTESIAN_POINT('Ctrl Pts',(-9.33003685209406,22.1221616190645,4.80129931551687));
#92457=CARTESIAN_POINT('Ctrl Pts',(-9.34784457455688,22.1210526730699,4.81031442199412));
#92458=CARTESIAN_POINT('Ctrl Pts',(-9.3728375928425,22.1195292855669,4.82233127214512));
#92459=CARTESIAN_POINT('Ctrl Pts',(-9.37987024524739,22.119104189983,4.82564390723366));
#92460=CARTESIAN_POINT('Ctrl Pts',(-9.39121516927925,22.1184240610725,4.83087774064756));
#92461=CARTESIAN_POINT('Ctrl Pts',(-9.39551085965176,22.1181678197877,4.83283435227153));
#92462=CARTESIAN_POINT('Ctrl Pts',(-9.40442898698283,22.1176384768501,4.83684441909221));
#92463=CARTESIAN_POINT('Ctrl Pts',(-9.40905275875837,22.1173654836952,4.83889476485651));
#92464=CARTESIAN_POINT('Ctrl Pts',(-9.4199168894195,22.1167274118548,4.84364506656454));
#92465=CARTESIAN_POINT('Ctrl Pts',(-9.42616564823459,22.116362994089,4.84632559915584));
#92466=CARTESIAN_POINT('Ctrl Pts',(-9.44659962658261,22.1151795524961,4.85492306052979));
#92467=CARTESIAN_POINT('Ctrl Pts',(-9.46085966915013,22.1143665575774,4.86066020758447));
#92468=CARTESIAN_POINT('Ctrl Pts',(-9.5358121100377,22.1101564696417,4.88945194186944));
#92469=CARTESIAN_POINT('Ctrl Pts',(-9.59790134507879,22.1068875170248,4.90867491018563));
#92470=CARTESIAN_POINT('Ctrl Pts',(-9.75557643684844,22.0988959128173,4.94621144036176));
#92471=CARTESIAN_POINT('Ctrl Pts',(-9.8520848686336,22.0942851976122,4.95924287508606));
#92472=CARTESIAN_POINT('Ctrl Pts',(-9.95996801387705,22.0888786143383,4.9629923048275));
#92473=CARTESIAN_POINT('Ctrl Pts',(-9.97077226603069,22.0883341632263,4.96324802263293));
#92474=CARTESIAN_POINT('Ctrl Pts',(-10.0139753732146,22.0861417915224,4.96379188538768));
#92475=CARTESIAN_POINT('Ctrl Pts',(-10.0463749145489,22.0844633937425,4.96312373410443));
#92476=CARTESIAN_POINT('Ctrl Pts',(-10.0844592918168,22.0824231496989,4.96107216693288));
#92477=CARTESIAN_POINT('Ctrl Pts',(-10.0901934839031,22.0821141558287,4.96072940076222));
#92478=CARTESIAN_POINT('Ctrl Pts',(-10.0994901061791,22.0816100594823,4.96011873853654));
#92479=CARTESIAN_POINT('Ctrl Pts',(-10.1030538898299,22.0814160700342,4.95987153787275));
#92480=CARTESIAN_POINT('Ctrl Pts',(-10.1093993832349,22.0810692735898,4.95940803397205));
#92481=CARTESIAN_POINT('Ctrl Pts',(-10.112181416177,22.0809167507836,4.95919682167899));
#92482=CARTESIAN_POINT('Ctrl Pts',(-10.1181887464026,22.0805863565253,4.95872346286045));
#92483=CARTESIAN_POINT('Ctrl Pts',(-10.121413736495,22.0804083398846,4.95845857844769));
#92484=CARTESIAN_POINT('Ctrl Pts',(-10.1303974613309,22.0799106936558,4.95769069705039));
#92485=CARTESIAN_POINT('Ctrl Pts',(-10.1361540684313,22.0795898033474,4.95716427816398));
#92486=CARTESIAN_POINT('Ctrl Pts',(-10.1694440945456,22.0777230917166,4.95392105031625));
#92487=CARTESIAN_POINT('Ctrl Pts',(-10.1968975041733,22.0761400504187,4.95045816582561));
#92488=CARTESIAN_POINT('Ctrl Pts',(-10.3376128891108,22.0678564580878,4.92864044099296));
#92489=CARTESIAN_POINT('Ctrl Pts',(-10.4485305027671,22.0607953565512,4.89779036562906));
#92490=CARTESIAN_POINT('Ctrl Pts',(-10.6192529357573,22.0498829116838,4.82786401519054));
#92491=CARTESIAN_POINT('Ctrl Pts',(-10.6818304502024,22.0458635700918,4.79684481337659));
#92492=CARTESIAN_POINT('Ctrl Pts',(-10.7517847537885,22.0413680693651,4.75569970496187));
#92493=CARTESIAN_POINT('Ctrl Pts',(-10.7615379957926,22.0407410631841,4.7498087679152));
#92494=CARTESIAN_POINT('Ctrl Pts',(-10.7763472171529,22.0397884781689,4.74062630162041));
#92495=CARTESIAN_POINT('Ctrl Pts',(-10.7814531447003,22.0394599440512,4.73741650466368));
#92496=CARTESIAN_POINT('Ctrl Pts',(-10.7906256409295,22.0388695228771,4.73157087815094));
#92497=CARTESIAN_POINT('Ctrl Pts',(-10.7946992159788,22.0386072299439,4.72894625143294));
#92498=CARTESIAN_POINT('Ctrl Pts',(-10.8026742588822,22.0380935338403,4.72375165335497));
#92499=CARTESIAN_POINT('Ctrl Pts',(-10.8065766027964,22.0378420811543,4.72118313920472));
#92500=CARTESIAN_POINT('Ctrl Pts',(-10.8175261332349,22.0371362335968,4.71390080025658));
#92501=CARTESIAN_POINT('Ctrl Pts',(-10.8245448181947,22.0366834317571,4.70914431655468));
#92502=CARTESIAN_POINT('Ctrl Pts',(-10.8539819317172,22.0347824029638,4.68881960158661));
#92503=CARTESIAN_POINT('Ctrl Pts',(-10.8760046323874,22.0333555619906,4.67268631540138));
#92504=CARTESIAN_POINT('Ctrl Pts',(-10.9329757461267,22.0296395929748,4.62844961090898));
#92505=CARTESIAN_POINT('Ctrl Pts',(-10.9671066525063,22.0273881298577,4.59933952514363));
#92506=CARTESIAN_POINT('Ctrl Pts',(-11.0598057092244,22.0211109455964,4.51261316555036));
#92507=CARTESIAN_POINT('Ctrl Pts',(-11.1149341768736,22.0171837786732,4.4515750286615));
#92508=CARTESIAN_POINT('Ctrl Pts',(-11.2016955977774,22.0101313039045,4.33755706769133));
#92509=CARTESIAN_POINT('Ctrl Pts',(-11.2356460165396,22.0070605143647,4.28660755910382));
#92510=CARTESIAN_POINT('Ctrl Pts',(-11.269930599622,22.003411907177,4.22743439232937));
#92511=CARTESIAN_POINT('Ctrl Pts',(-11.2735087064465,22.0030235261731,4.22115192110603));
#92512=CARTESIAN_POINT('Ctrl Pts',(-11.2787683912248,22.0024407777463,4.21175569702305));
#92513=CARTESIAN_POINT('Ctrl Pts',(-11.2804855179427,22.0022485982691,4.20866184350611));
#92514=CARTESIAN_POINT('Ctrl Pts',(-11.2835351856019,22.0019037550703,4.20311979535971));
#92515=CARTESIAN_POINT('Ctrl Pts',(-11.2848719687843,22.0017513627127,4.2006739919366));
#92516=CARTESIAN_POINT('Ctrl Pts',(-11.2877571490049,22.001419748754,4.19535919027451));
#92517=CARTESIAN_POINT('Ctrl Pts',(-11.2893029278831,22.0012403719883,4.19248887213935));
#92518=CARTESIAN_POINT('Ctrl Pts',(-11.2936154835886,22.0007351535464,4.18441650125373));
#92519=CARTESIAN_POINT('Ctrl Pts',(-11.2963604217629,22.0004079896983,4.17920293067916));
#92520=CARTESIAN_POINT('Ctrl Pts',(-11.3126994443173,21.9984271683819,4.14770968867428));
#92521=CARTESIAN_POINT('Ctrl Pts',(-11.3255246337247,21.9967309077959,4.12104095865997));
#92522=CARTESIAN_POINT('Ctrl Pts',(-11.3926644296615,21.987084682709,3.96986077497243));
#92523=CARTESIAN_POINT('Ctrl Pts',(-11.4302488217402,21.9786761397781,3.83864269421216));
#92524=CARTESIAN_POINT('Ctrl Pts',(-11.4559229522552,21.9679796483223,3.65635356779133));
#92525=CARTESIAN_POINT('Ctrl Pts',(-11.4602848338256,21.9652394749179,3.6082914467565));
#92526=CARTESIAN_POINT('Ctrl Pts',(-11.4626948800845,21.9619945793909,3.54965124027359));
#92527=CARTESIAN_POINT('Ctrl Pts',(-11.4630122637918,21.9614200016354,3.53920053386947));
#92528=CARTESIAN_POINT('Ctrl Pts',(-11.4633246277521,21.9605513674528,3.52330133005845));
#92529=CARTESIAN_POINT('Ctrl Pts',(-11.4634012166515,21.960254790277,3.51785492628046));
#92530=CARTESIAN_POINT('Ctrl Pts',(-11.4634713637882,21.9598057384796,3.50958161548477));
#92531=CARTESIAN_POINT('Ctrl Pts',(-11.4634871404727,21.9596525759417,3.50675498409382));
#92532=CARTESIAN_POINT('Ctrl Pts',(-11.4634981925777,21.9594298416703,3.50263751532071));
#92533=CARTESIAN_POINT('Ctrl Pts',(-11.4634999496205,21.9593600692025,3.50134671354812));
#92534=CARTESIAN_POINT('Ctrl Pts',(-11.4634999989321,21.9592903496774,3.50005590890961));
#92535=CARTESIAN_POINT('Ctrl Pts',(-11.4634999997572,21.8907061526447,3.50002665861792));
#92536=CARTESIAN_POINT('Ctrl Pts',(-11.4634998748308,21.8910743722622,3.50688484649636));
#92537=CARTESIAN_POINT('Ctrl Pts',(-11.463451542126,21.8914411004734,3.51374303113273));
#92538=CARTESIAN_POINT('Ctrl Pts',(-11.463197530598,21.892402160295,3.53178653891741));
#92539=CARTESIAN_POINT('Ctrl Pts',(-11.4629118060168,21.8929940237266,3.54297039138399));
#92540=CARTESIAN_POINT('Ctrl Pts',(-11.4602288213616,21.8968058150075,3.61543306443494));
#92541=CARTESIAN_POINT('Ctrl Pts',(-11.4541101003046,21.8999085988066,3.67651606038468));
#92542=CARTESIAN_POINT('Ctrl Pts',(-11.4274677810593,21.9080509034445,3.83883538003897));
#92543=CARTESIAN_POINT('Ctrl Pts',(-11.4000451466615,21.9129317401083,3.93857182873777));
#92544=CARTESIAN_POINT('Ctrl Pts',(-11.3517927132806,21.9195492143766,4.06153960555146));
#92545=CARTESIAN_POINT('Ctrl Pts',(-11.3404216078735,21.9210220395044,4.08816664706924));
#92546=CARTESIAN_POINT('Ctrl Pts',(-11.3235812573302,21.9231139835003,4.12457151651568));
#92547=CARTESIAN_POINT('Ctrl Pts',(-11.3187777212497,21.9237017266148,4.13465126820184));
#92548=CARTESIAN_POINT('Ctrl Pts',(-11.3102421852116,21.924732572778,4.1520468526634));
#92549=CARTESIAN_POINT('Ctrl Pts',(-11.3065630155415,21.9251727914233,4.15938817261978));
#92550=CARTESIAN_POINT('Ctrl Pts',(-11.301124435131,21.9258181911071,4.1700159296998));
#92551=CARTESIAN_POINT('Ctrl Pts',(-11.2994138747964,21.9260204407393,4.17332735211605));
#92552=CARTESIAN_POINT('Ctrl Pts',(-11.2963923507264,21.9263764614262,4.17912223430904));
#92553=CARTESIAN_POINT('Ctrl Pts',(-11.2950868638673,21.9265298901638,4.18160850281825));
#92554=CARTESIAN_POINT('Ctrl Pts',(-11.292304578325,21.9268560711533,4.18687044756367));
#92555=CARTESIAN_POINT('Ctrl Pts',(-11.2908260125752,21.9270289292762,4.18964508246653));
#92556=CARTESIAN_POINT('Ctrl Pts',(-11.2868024026863,21.9274979874139,4.19713740424601));
#92557=CARTESIAN_POINT('Ctrl Pts',(-11.2842403866769,21.9277952273199,4.20184586011237));
#92558=CARTESIAN_POINT('Ctrl Pts',(-11.2724562859347,21.9291555719528,4.223222034322));
#92559=CARTESIAN_POINT('Ctrl Pts',(-11.2629355871003,21.9302358839294,4.23972207080109));
#92560=CARTESIAN_POINT('Ctrl Pts',(-11.2003879433655,21.9371953382564,4.34339273009055));
#92561=CARTESIAN_POINT('Ctrl Pts',(-11.1386909554315,21.9434363486893,4.42499959528285));
#92562=CARTESIAN_POINT('Ctrl Pts',(-11.0085140950354,21.9548446394095,4.5642264468861));
#92563=CARTESIAN_POINT('Ctrl Pts',(-10.9422604566426,21.9600235828667,4.62331123269489));
#92564=CARTESIAN_POINT('Ctrl Pts',(-10.8600809710249,21.965709236107,4.68417888342102));
#92565=CARTESIAN_POINT('Ctrl Pts',(-10.8489886807373,21.9664629160807,4.69215650920394));
#92566=CARTESIAN_POINT('Ctrl Pts',(-10.8326263598107,21.9675550849795,4.70358015682235));
#92567=CARTESIAN_POINT('Ctrl Pts',(-10.8274434497495,21.9678982236067,4.70714919879279));
#92568=CARTESIAN_POINT('Ctrl Pts',(-10.8221661803877,21.968244795917,4.71073326099728));
#92569=CARTESIAN_POINT('Ctrl Pts',(-10.8220947328629,21.9682494875455,4.71078177540692));
#92570=CARTESIAN_POINT('Ctrl Pts',(-10.821951768276,21.968258874328,4.71087883295523));
#92571=CARTESIAN_POINT('Ctrl Pts',(-10.8218802512169,21.9682635694809,4.71092737607618));
#92572=CARTESIAN_POINT('Ctrl Pts',(-10.8217369152581,21.9682729785585,4.71102464864867));
#92573=CARTESIAN_POINT('Ctrl Pts',(-10.8216650963192,21.9682776924817,4.71107337805077));
#92574=CARTESIAN_POINT('Ctrl Pts',(-10.8215209097618,21.968287155287,4.71117119040635));
#92575=CARTESIAN_POINT('Ctrl Pts',(-10.8214485420768,21.9682919041657,4.71122027326418));
#92576=CARTESIAN_POINT('Ctrl Pts',(-10.8213029921463,21.968301454304,4.71131897240524));
#92577=CARTESIAN_POINT('Ctrl Pts',(-10.8212298098202,21.9683062555571,4.71136858853121));
#92578=CARTESIAN_POINT('Ctrl Pts',(-10.8210823402887,21.9683159294532,4.71146855036329));
#92579=CARTESIAN_POINT('Ctrl Pts',(-10.8210080529223,21.9683208020904,4.71151889588647));
#92580=CARTESIAN_POINT('Ctrl Pts',(-10.8208580517571,21.9683306397945,4.71162053351247));
#92581=CARTESIAN_POINT('Ctrl Pts',(-10.8207823377936,21.9683356048505,4.7116718253428));
#92582=CARTESIAN_POINT('Ctrl Pts',(-10.8206291222447,21.9683456510101,4.71177559906311));
#92583=CARTESIAN_POINT('Ctrl Pts',(-10.820551620425,21.9683507321014,4.71182808061982));
#92584=CARTESIAN_POINT('Ctrl Pts',(-10.8203944175345,21.9683610372319,4.71193451099511));
#92585=CARTESIAN_POINT('Ctrl Pts',(-10.8203147161731,21.9683662612553,4.71198845938921));
#92586=CARTESIAN_POINT('Ctrl Pts',(-10.8201526380789,21.9683768833484,4.71209814377574));
#92587=CARTESIAN_POINT('Ctrl Pts',(-10.8200702609818,21.9683822813983,4.7121538792355));
#92588=CARTESIAN_POINT('Ctrl Pts',(-10.8199022722045,21.968393288052,4.71226751367654));
#92589=CARTESIAN_POINT('Ctrl Pts',(-10.8198166600698,21.9683988966308,4.71232541198875));
#92590=CARTESIAN_POINT('Ctrl Pts',(-10.8196415337722,21.9684103678967,4.7124438204675));
#92591=CARTESIAN_POINT('Ctrl Pts',(-10.8195520190268,21.9684162305528,4.71250432979987));
#92592=CARTESIAN_POINT('Ctrl Pts',(-10.8193682770411,21.9684282628382,4.71262850432881));
#92593=CARTESIAN_POINT('Ctrl Pts',(-10.8192740491149,21.9684344324249,4.71269216843304));
#92594=CARTESIAN_POINT('Ctrl Pts',(-10.8190798781763,21.9684471439426,4.71282332501919));
#92595=CARTESIAN_POINT('Ctrl Pts',(-10.8189799342142,21.9684536858237,4.71289081614891));
#92596=CARTESIAN_POINT('Ctrl Pts',(-10.8187730647724,21.9684672244734,4.71303047572784));
#92597=CARTESIAN_POINT('Ctrl Pts',(-10.8186661381075,21.9684742211739,4.71310264238333));
#92598=CARTESIAN_POINT('Ctrl Pts',(-10.8184436652786,21.9684887761839,4.7132527503332));
#92599=CARTESIAN_POINT('Ctrl Pts',(-10.8183281174961,21.9684963344059,4.71333068927688));
#92600=CARTESIAN_POINT('Ctrl Pts',(-10.818086224307,21.9685121543227,4.7134938000734));
#92601=CARTESIAN_POINT('Ctrl Pts',(-10.8179598767135,21.9685204158973,4.7135789687137));
#92602=CARTESIAN_POINT('Ctrl Pts',(-10.8176933891285,21.9685378375021,4.71375854267936));
#92603=CARTESIAN_POINT('Ctrl Pts',(-10.8175532460828,21.968546997362,4.71385294347014));
#92604=CARTESIAN_POINT('Ctrl Pts',(-10.8136038127563,21.9688050796486,4.71651229979693));
#92605=CARTESIAN_POINT('Ctrl Pts',(-10.8097824573528,21.9690533301211,4.71905935545328));
#92606=CARTESIAN_POINT('Ctrl Pts',(-10.8010925827219,21.9696145841972,4.72479254432749));
#92607=CARTESIAN_POINT('Ctrl Pts',(-10.7962169081917,21.9699271783823,4.72796772725514));
#92608=CARTESIAN_POINT('Ctrl Pts',(-10.7825403764259,21.9707976723271,4.73675858462343));
#92609=CARTESIAN_POINT('Ctrl Pts',(-10.7736980794,21.9713531835782,4.74230935231646));
#92610=CARTESIAN_POINT('Ctrl Pts',(-10.7240156703094,21.9744351813889,4.77276136284784));
#92611=CARTESIAN_POINT('Ctrl Pts',(-10.6820313126561,21.9768916026595,4.79574459928614));
#92612=CARTESIAN_POINT('Ctrl Pts',(-10.5164223427695,21.9861438710776,4.876118669063));
#92613=CARTESIAN_POINT('Ctrl Pts',(-10.3861620492173,21.9924623938844,4.91819135349303));
#92614=CARTESIAN_POINT('Ctrl Pts',(-10.2228014318503,22.0009183102586,4.94674428002749));
#92615=CARTESIAN_POINT('Ctrl Pts',(-10.1934793515914,22.0024590523433,4.95095657868612));
#92616=CARTESIAN_POINT('Ctrl Pts',(-10.1581937435553,22.0043616300477,4.95493702358752));
#92617=CARTESIAN_POINT('Ctrl Pts',(-10.1523318822887,22.0046792957759,4.95556243369102));
#92618=CARTESIAN_POINT('Ctrl Pts',(-10.1432214159017,22.0051757079196,4.95647880628542));
#92619=CARTESIAN_POINT('Ctrl Pts',(-10.1399752791049,22.005353115199,4.95679436021216));
#92620=CARTESIAN_POINT('Ctrl Pts',(-10.1339520315398,22.0056833261085,4.95735955684384));
#92621=CARTESIAN_POINT('Ctrl Pts',(-10.1311752473293,22.0058359663863,4.95761211533821));
#92622=CARTESIAN_POINT('Ctrl Pts',(-10.1248719459341,22.0061833826945,4.9581672657449));
#92623=CARTESIAN_POINT('Ctrl Pts',(-10.121345058097,22.0063784237152,4.95846499927265));
#92624=CARTESIAN_POINT('Ctrl Pts',(-10.1106091762258,22.0069740388085,4.95933209178829));
#92625=CARTESIAN_POINT('Ctrl Pts',(-10.1033971230959,22.0073767724275,4.95986080656225));
#92626=CARTESIAN_POINT('Ctrl Pts',(-10.0351607744107,22.0112100412938,4.96435503330603));
#92627=CARTESIAN_POINT('Ctrl Pts',(-9.97395390869413,22.014818850994,4.96454498525115));
#92628=CARTESIAN_POINT('Ctrl Pts',(-9.85267291100218,22.0220921318146,4.95731595535349));
#92629=CARTESIAN_POINT('Ctrl Pts',(-9.79270372475452,22.0257479281469,4.95000120308259));
#92630=CARTESIAN_POINT('Ctrl Pts',(-9.67477066658229,22.032915489132,4.92814856277899));
#92631=CARTESIAN_POINT('Ctrl Pts',(-9.61689785912112,22.0364217347995,4.91372428260201));
#92632=CARTESIAN_POINT('Ctrl Pts',(-9.52848053384113,22.0417176537997,4.88585642973307));
#92633=CARTESIAN_POINT('Ctrl Pts',(-9.49724538710658,22.043576981709,4.87483333514987));
#92634=CARTESIAN_POINT('Ctrl Pts',(-9.45796564231367,22.0459014153428,4.85945328319706));
#92635=CARTESIAN_POINT('Ctrl Pts',(-9.44955285351882,22.0463984569333,4.85606873654565));
#92636=CARTESIAN_POINT('Ctrl Pts',(-9.43606349337157,22.0471942588067,4.85049561902494));
#92637=CARTESIAN_POINT('Ctrl Pts',(-9.43096700766257,22.0474946537564,4.84835613074385));
#92638=CARTESIAN_POINT('Ctrl Pts',(-9.42127744166367,22.0480652931244,4.84422375982401));
#92639=CARTESIAN_POINT('Ctrl Pts',(-9.41668223765199,22.0483357078916,4.84223608392613));
#92640=CARTESIAN_POINT('Ctrl Pts',(-9.40620211852893,22.0489519996026,4.83763887734628));
#92641=CARTESIAN_POINT('Ctrl Pts',(-9.40032401655242,22.0492973514997,4.83501401000542));
#92642=CARTESIAN_POINT('Ctrl Pts',(-9.38502669995551,22.0501953902724,4.82806157047441));
#92643=CARTESIAN_POINT('Ctrl Pts',(-9.37563571615882,22.050745981241,4.82367252111219));
#92644=CARTESIAN_POINT('Ctrl Pts',(-9.30670012967024,22.0547839013786,4.79055732755841));
#92645=CARTESIAN_POINT('Ctrl Pts',(-9.24911316879043,22.0581313113593,4.75792419203766));
#92646=CARTESIAN_POINT('Ctrl Pts',(-9.09528193418636,22.067248115937,4.65641051571358));
#92647=CARTESIAN_POINT('Ctrl Pts',(-9.0048977651671,22.0727919791811,4.57961413658884));
#92648=CARTESIAN_POINT('Ctrl Pts',(-8.90572674350895,22.0802644833843,4.4722055869489));
#92649=CARTESIAN_POINT('Ctrl Pts',(-8.88731182132546,22.0817251183974,4.45107438017727));
#92650=CARTESIAN_POINT('Ctrl Pts',(-8.86583040885561,22.0835380228467,4.42494609002167));
#92651=CARTESIAN_POINT('Ctrl Pts',(-8.86217150719607,22.0838508233243,4.42044133415475));
#92652=CARTESIAN_POINT('Ctrl Pts',(-8.85651087972144,22.0843412568194,4.41338676876146));
#92653=CARTESIAN_POINT('Ctrl Pts',(-8.8544906275482,22.0845176021297,4.4108518182182));
#92654=CARTESIAN_POINT('Ctrl Pts',(-8.85074691273074,22.0848468810217,4.40612216530549));
#92655=CARTESIAN_POINT('Ctrl Pts',(-8.84902129642667,22.0849996594038,4.40392923427325));
#92656=CARTESIAN_POINT('Ctrl Pts',(-8.84510405772229,22.0853487568711,4.39892176370605));
#92657=CARTESIAN_POINT('Ctrl Pts',(-8.84291645515684,22.0855453516001,4.39610414821671));
#92658=CARTESIAN_POINT('Ctrl Pts',(-8.83724472560966,22.0860592837821,4.38874360719605));
#92659=CARTESIAN_POINT('Ctrl Pts',(-8.8337769508376,22.0863777089599,4.38418822931801));
#92660=CARTESIAN_POINT('Ctrl Pts',(-8.81110553810187,22.0884867157653,4.35404094500185));
#92661=CARTESIAN_POINT('Ctrl Pts',(-8.7927201450553,22.0903269564238,4.32784722532375));
#92662=CARTESIAN_POINT('Ctrl Pts',(-8.76401506284007,22.0933957444598,4.28395900695168));
#92663=CARTESIAN_POINT('Ctrl Pts',(-8.75318117746453,22.094605200493,4.26661154681494));
#92664=CARTESIAN_POINT('Ctrl Pts',(-8.69632430617389,22.1012188882643,4.17117606652502));
#92665=CARTESIAN_POINT('Ctrl Pts',(-8.65726497784818,22.1067439338684,4.08916181754542));
#92666=CARTESIAN_POINT('Ctrl Pts',(-8.60447708175757,22.1157990278512,3.94527425252378));
#92667=CARTESIAN_POINT('Ctrl Pts',(-8.58670308899088,22.1194124833181,3.88515812811265));
#92668=CARTESIAN_POINT('Ctrl Pts',(-8.56949346164546,22.1237436465362,3.80937167794232));
#92669=CARTESIAN_POINT('Ctrl Pts',(-8.56638065445041,22.1245771586564,3.79461056906044));
#92670=CARTESIAN_POINT('Ctrl Pts',(-8.56220607494877,22.1257731844546,3.77317839827974));
#92671=CARTESIAN_POINT('Ctrl Pts',(-8.56096145088509,22.1261414485365,3.76654430119513));
#92672=CARTESIAN_POINT('Ctrl Pts',(-8.55886570598945,22.1267827726359,3.75493079787183));
#92673=CARTESIAN_POINT('Ctrl Pts',(-8.55799439364573,22.1270564651864,3.74995519040138));
#92674=CARTESIAN_POINT('Ctrl Pts',(-8.55635610290043,22.1275851939063,3.74030600803198));
#92675=CARTESIAN_POINT('Ctrl Pts',(-8.5555860168554,22.1278403247682,3.73563303068786));
#92676=CARTESIAN_POINT('Ctrl Pts',(-8.55380391283131,22.1284469758645,3.72448188544319));
#92677=CARTESIAN_POINT('Ctrl Pts',(-8.55281271422711,22.1287978399415,3.71800046153499));
#92678=CARTESIAN_POINT('Ctrl Pts',(-8.54941132236074,22.1300524204314,3.69471260025974));
#92679=CARTESIAN_POINT('Ctrl Pts',(-8.54725001769878,22.130948367659,3.67787082067707));
#92680=CARTESIAN_POINT('Ctrl Pts',(-8.53346270707527,22.1374989625693,3.55329989332224));
#92681=CARTESIAN_POINT('Ctrl Pts',(-8.53353908582426,22.1427605146645,3.44461420875881));
#92682=CARTESIAN_POINT('Ctrl Pts',(-8.55567232005459,22.1524191486553,3.24721974889649));
#92683=CARTESIAN_POINT('Ctrl Pts',(-8.57400707557569,22.1568058832743,3.15864926168474));
#92684=CARTESIAN_POINT('Ctrl Pts',(-8.60298181120139,22.1620708250013,3.06382129929687));
#92685=CARTESIAN_POINT('Ctrl Pts',(-8.60566384414128,22.1625479531297,3.05532218923868));
#92686=CARTESIAN_POINT('Ctrl Pts',(-8.60961632516433,22.1632375750851,3.04318457430629));
#92687=CARTESIAN_POINT('Ctrl Pts',(-8.61082383328572,22.1634465445029,3.0395255994677));
#92688=CARTESIAN_POINT('Ctrl Pts',(-8.61294220659321,22.1638102782918,3.03319070499079));
#92689=CARTESIAN_POINT('Ctrl Pts',(-8.61384640921342,22.1639646547203,3.0305125530506));
#92690=CARTESIAN_POINT('Ctrl Pts',(-8.61562919322852,22.1642673535614,3.02528218388922));
#92691=CARTESIAN_POINT('Ctrl Pts',(-8.61650707765149,22.1644156294216,3.02272977346037));
#92692=CARTESIAN_POINT('Ctrl Pts',(-8.61893326590075,22.164823265413,3.01573868085732));
#92693=CARTESIAN_POINT('Ctrl Pts',(-8.62049588907889,22.1650834491609,3.01130504815456));
#92694=CARTESIAN_POINT('Ctrl Pts',(-8.62664020650202,22.1660972600922,2.99413607666613));
#92695=CARTESIAN_POINT('Ctrl Pts',(-8.63137697641954,22.1668593317833,2.98145740412045));
#92696=CARTESIAN_POINT('Ctrl Pts',(-8.67507478130511,22.1737111459457,2.86926532623544));
#92697=CARTESIAN_POINT('Ctrl Pts',(-8.72464921269192,22.180252375855,2.7742372276203));
#92698=CARTESIAN_POINT('Ctrl Pts',(-8.83632298131635,22.1922710396534,2.60754051578375));
#92699=CARTESIAN_POINT('Ctrl Pts',(-8.89589738625106,22.197754551217,2.5348105436654));
#92700=CARTESIAN_POINT('Ctrl Pts',(-8.97024122864046,22.2035962071607,2.46001698198819));
#92701=CARTESIAN_POINT('Ctrl Pts',(-8.97854747885132,22.2042368512649,2.45185756550034));
#92702=CARTESIAN_POINT('Ctrl Pts',(-8.99134059085267,22.2052056625035,2.43958713164148));
#92703=CARTESIAN_POINT('Ctrl Pts',(-8.99575705178449,22.2055369466724,2.43540366449849));
#92704=CARTESIAN_POINT('Ctrl Pts',(-9.00348167530305,22.2061109446072,2.42817740343023));
#92705=CARTESIAN_POINT('Ctrl Pts',(-9.00677798641658,22.2063541891962,2.42512210817563));
#92706=CARTESIAN_POINT('Ctrl Pts',(-9.01420496614086,22.2068984856945,2.41830150221231));
#92707=CARTESIAN_POINT('Ctrl Pts',(-9.01834324826844,22.207199183005,2.41454456016516));
#92708=CARTESIAN_POINT('Ctrl Pts',(-9.02946012790565,22.2080001657881,2.40456766873976));
#92709=CARTESIAN_POINT('Ctrl Pts',(-9.0364770316985,22.2084986633406,2.39839066330193));
#92710=CARTESIAN_POINT('Ctrl Pts',(-9.06786861568483,22.2106982945188,2.37128595532881));
#92711=CARTESIAN_POINT('Ctrl Pts',(-9.09287021598116,22.2123693907942,2.35109614574636));
#92712=CARTESIAN_POINT('Ctrl Pts',(-9.13567363722489,22.2151126605051,2.31879972305439));
#92713=CARTESIAN_POINT('Ctrl Pts',(-9.15311334903888,22.2161996834704,2.30623402429931));
#92714=CARTESIAN_POINT('Ctrl Pts',(-9.28048285998501,22.2239450539178,2.21865798166779));
#92715=CARTESIAN_POINT('Ctrl Pts',(-9.39989846183862,22.2301283419472,2.15857761733415));
#92716=CARTESIAN_POINT('Ctrl Pts',(-9.55356135362848,22.2384134733811,2.1059456678371));
#92717=CARTESIAN_POINT('Ctrl Pts',(-9.58162668197631,22.2399418352708,2.09726749483232));
#92718=CARTESIAN_POINT('Ctrl Pts',(-9.61560074068774,22.2418305572055,2.08787250916541));
#92719=CARTESIAN_POINT('Ctrl Pts',(-9.62127869605408,22.2421474919794,2.086339145158));
#92720=CARTESIAN_POINT('Ctrl Pts',(-9.63011648693593,22.2426430061294,2.0840095147169));
#92721=CARTESIAN_POINT('Ctrl Pts',(-9.63327006507881,22.2428202541525,2.08318948971373));
#92722=CARTESIAN_POINT('Ctrl Pts',(-9.63912751994568,22.2431503238564,2.08168724199177));
#92723=CARTESIAN_POINT('Ctrl Pts',(-9.641830622287,22.2433029834021,2.08100221181624));
#92724=CARTESIAN_POINT('Ctrl Pts',(-9.64797307959817,22.243650645303,2.07946423702906));
#92725=CARTESIAN_POINT('Ctrl Pts',(-9.65141356980905,22.2438459142127,2.07861605936026));
#92726=CARTESIAN_POINT('Ctrl Pts',(-9.66190446529486,22.2444429011342,2.07607013860111));
#92727=CARTESIAN_POINT('Ctrl Pts',(-9.66896432947109,22.2448467929309,2.07441232427301));
#92728=CARTESIAN_POINT('Ctrl Pts',(-9.73795198291566,22.2488124938283,2.05875255543484));
#92729=CARTESIAN_POINT('Ctrl Pts',(-9.8007108636651,22.2525662347383,2.04874346243632));
#92730=CARTESIAN_POINT('Ctrl Pts',(-9.97833562145495,22.2632567738457,2.03215482531083));
#92731=CARTESIAN_POINT('Ctrl Pts',(-10.0936368131551,22.2702377785958,2.03498204341848));
#92732=CARTESIAN_POINT('Ctrl Pts',(-10.2425185400727,22.2788530377613,2.05629857679318));
#92733=CARTESIAN_POINT('Ctrl Pts',(-10.2774196446066,22.2808472449842,2.06259689452283));
#92734=CARTESIAN_POINT('Ctrl Pts',(-10.3211205628221,22.2833131071254,2.07213451551405));
#92735=CARTESIAN_POINT('Ctrl Pts',(-10.3301624534263,22.2838216298429,2.07419811419579));
#92736=CARTESIAN_POINT('Ctrl Pts',(-10.3446053664413,22.2846313462907,2.07763912880652));
#92737=CARTESIAN_POINT('Ctrl Pts',(-10.3500190957812,22.2849342784268,2.0789616682617));
#92738=CARTESIAN_POINT('Ctrl Pts',(-10.3602724792542,22.2855069592888,2.08152865394662));
#92739=CARTESIAN_POINT('Ctrl Pts',(-10.3651135606679,22.2857768975296,2.08276702424921));
#92740=CARTESIAN_POINT('Ctrl Pts',(-10.3760965938596,22.2863883258784,2.08563654434856));
#92741=CARTESIAN_POINT('Ctrl Pts',(-10.3822344778311,22.2867293214878,2.08728295887278));
#92742=CARTESIAN_POINT('Ctrl Pts',(-10.3980910677557,22.2876085329456,2.09164720785049));
#92743=CARTESIAN_POINT('Ctrl Pts',(-10.4077928232807,22.2881447967354,2.0944257026218));
#92744=CARTESIAN_POINT('Ctrl Pts',(-10.4725317784981,22.2917132561691,2.11369307768479));
#92745=CARTESIAN_POINT('Ctrl Pts',(-10.5265885218191,22.2946415962917,2.13331105761356));
#92746=CARTESIAN_POINT('Ctrl Pts',(-10.695529752119,22.3038047992147,2.20613950238704));
#92747=CARTESIAN_POINT('Ctrl Pts',(-10.8047054756562,22.3097066588664,2.27106549942956));
#92748=CARTESIAN_POINT('Ctrl Pts',(-10.9268237923954,22.3176351491507,2.367012671397));
#92749=CARTESIAN_POINT('Ctrl Pts',(-10.948950613736,22.3191355986231,2.38547986030676));
#92750=CARTESIAN_POINT('Ctrl Pts',(-10.9748949681556,22.3209930779516,2.40846609229575));
#92751=CARTESIAN_POINT('Ctrl Pts',(-10.9792501329606,22.3213083370287,2.41237154993949));
#92752=CARTESIAN_POINT('Ctrl Pts',(-10.9859894587572,22.3218017922268,2.41848827550402));
#92753=CARTESIAN_POINT('Ctrl Pts',(-10.9883899113329,22.3219786747619,2.42068160130729));
#92754=CARTESIAN_POINT('Ctrl Pts',(-10.9928359407773,22.3223084222953,2.42477126842293));
#92755=CARTESIAN_POINT('Ctrl Pts',(-10.9948834164606,22.3224611279589,2.42666546791513));
#92756=CARTESIAN_POINT('Ctrl Pts',(-10.9995266119369,22.3228093620652,2.4309857691967));
#92757=CARTESIAN_POINT('Ctrl Pts',(-11.0021189092997,22.3230051606963,2.43341546762361));
#92758=CARTESIAN_POINT('Ctrl Pts',(-11.0088310265022,22.3235156666897,2.43975264611415));
#92759=CARTESIAN_POINT('Ctrl Pts',(-11.0129369589023,22.3238314387093,2.44367466819873));
#92760=CARTESIAN_POINT('Ctrl Pts',(-11.0393808730648,22.3258872102307,2.4692300735727));
#92761=CARTESIAN_POINT('Ctrl Pts',(-11.0610458807732,22.3276741242561,2.49154543925271));
#92762=CARTESIAN_POINT('Ctrl Pts',(-11.0900548349518,22.330192460721,2.52339545628815));
#92763=CARTESIAN_POINT('Ctrl Pts',(-11.0980181964138,22.3308977523125,2.53235750035761));
#92764=CARTESIAN_POINT('Ctrl Pts',(-11.1696780201647,22.3373663805239,2.61502786914373));
#92765=CARTESIAN_POINT('Ctrl Pts',(-11.2259770888658,22.3433222520924,2.69482685579464));
#92766=CARTESIAN_POINT('Ctrl Pts',(-11.3058725866744,22.3529291419746,2.83611748346024));
#92767=CARTESIAN_POINT('Ctrl Pts',(-11.3340244891197,22.3566801773988,2.89467066488936));
#92768=CARTESIAN_POINT('Ctrl Pts',(-11.3639230564336,22.3611559624163,2.96916826968876));
#92769=CARTESIAN_POINT('Ctrl Pts',(-11.3694222003879,22.3620054171893,2.98352028870059));
#92770=CARTESIAN_POINT('Ctrl Pts',(-11.3770272454513,22.3632199489929,3.00434441316852));
#92771=CARTESIAN_POINT('Ctrl Pts',(-11.379315551355,22.3635910271429,3.0107484211073));
#92772=CARTESIAN_POINT('Ctrl Pts',(-11.3832283571807,22.3642356159443,3.02194439661502));
#92773=CARTESIAN_POINT('Ctrl Pts',(-11.3848727853526,22.3645097782961,3.02672923466602));
#92774=CARTESIAN_POINT('Ctrl Pts',(-11.388210587683,22.3650731223719,3.0366076983308));
#92775=CARTESIAN_POINT('Ctrl Pts',(-11.3899008200342,22.3653621978181,3.04170231014588));
#92776=CARTESIAN_POINT('Ctrl Pts',(-11.3941462061364,22.3660982067782,3.05473806132351));
#92777=CARTESIAN_POINT('Ctrl Pts',(-11.3966615808529,22.366543840011,3.06269201861919));
#92778=CARTESIAN_POINT('Ctrl Pts',(-11.4060733515762,22.3682493685352,3.09336307494882));
#92779=CARTESIAN_POINT('Ctrl Pts',(-11.4124848137888,22.369493601722,3.11622585638976));
#92780=CARTESIAN_POINT('Ctrl Pts',(-11.4483292668002,22.3770163013476,3.25714747176875));
#92781=CARTESIAN_POINT('Ctrl Pts',(-11.4634999999934,22.3828111295509,3.3783324018081));
#92782=CARTESIAN_POINT('Ctrl Pts',(-11.4635,22.3887666433152,3.49999999992021));
#92783=CARTESIAN_POINT('Origin',(-10.,13.2,3.5));
#92784=CARTESIAN_POINT('',(-11.4635,22.9615280277103,3.50000000002193));
#92785=CARTESIAN_POINT('',(-11.4635,22.8886966621701,3.49999999996283));
#92786=CARTESIAN_POINT('',(-11.4635,13.2,3.5));
#92787=CARTESIAN_POINT('',(-11.4634996241254,22.9614759749743,3.49895110311648));
#92788=CARTESIAN_POINT('Ctrl Pts',(-11.4635,22.9615280277103,3.50000000002193));
#92789=CARTESIAN_POINT('Ctrl Pts',(-11.4635,22.9615106796706,3.49965037019642));
#92790=CARTESIAN_POINT('Ctrl Pts',(-11.4634998747103,22.9614933287665,3.49930073787219));
#92791=CARTESIAN_POINT('Ctrl Pts',(-11.4634996241254,22.9614759749743,3.49895110311631));
#92792=CARTESIAN_POINT('Ctrl Pts',(-11.4634996227294,22.9614758783865,3.49894915711806));
#92793=CARTESIAN_POINT('Ctrl Pts',(-11.4634732452863,22.9596525387403,3.46221352449691));
#92794=CARTESIAN_POINT('Ctrl Pts',(-11.4620637099453,22.9577996109202,3.42549345045632));
#92795=CARTESIAN_POINT('Ctrl Pts',(-11.4581077419284,22.9550890724053,3.37354803891934));
#92796=CARTESIAN_POINT('Ctrl Pts',(-11.4566999901143,22.9542796794849,3.35824885081634));
#92797=CARTESIAN_POINT('Ctrl Pts',(-11.4545582938092,22.9532121376693,3.3384030684732));
#92798=CARTESIAN_POINT('Ctrl Pts',(-11.4540433356523,22.9529651037365,3.33383329060898));
#92799=CARTESIAN_POINT('Ctrl Pts',(-11.453141352384,22.9525478402738,3.32615444841089));
#92800=CARTESIAN_POINT('Ctrl Pts',(-11.4527658623536,22.9523782257767,3.32304403194678));
#92801=CARTESIAN_POINT('Ctrl Pts',(-11.4520582732807,22.9520658655692,3.31733671638442));
#92802=CARTESIAN_POINT('Ctrl Pts',(-11.4517291868762,22.95192328611,3.31473944852019));
#92803=CARTESIAN_POINT('Ctrl Pts',(-11.4510334839562,22.9516272991256,3.30936440807431));
#92804=CARTESIAN_POINT('Ctrl Pts',(-11.4506658617093,22.9514738333081,3.3065868213375));
#92805=CARTESIAN_POINT('Ctrl Pts',(-11.4498047599134,22.9511209672799,3.30022131027363));
#92806=CARTESIAN_POINT('Ctrl Pts',(-11.4493059364927,22.9509212721497,3.29663415084392));
#92807=CARTESIAN_POINT('Ctrl Pts',(-11.447939669845,22.9503866213018,3.28706938481767));
#92808=CARTESIAN_POINT('Ctrl Pts',(-11.447048535404,22.9500504020038,3.28109529924195));
#92809=CARTESIAN_POINT('Ctrl Pts',(-11.4401422078661,22.9475347194591,3.23668186635204));
#92810=CARTESIAN_POINT('Ctrl Pts',(-11.4326337019908,22.9452820229483,3.1984934683087));
#92811=CARTESIAN_POINT('Ctrl Pts',(-11.4178662325746,22.9415278490329,3.13654162919375));
#92812=CARTESIAN_POINT('Ctrl Pts',(-11.4115073323534,22.9400508489001,3.11258081753115));
#92813=CARTESIAN_POINT('Ctrl Pts',(-11.3850662966905,22.9344131355215,3.02226706459585));
#92814=CARTESIAN_POINT('Ctrl Pts',(-11.3608865634778,22.9302103812058,2.95720567509524));
#92815=CARTESIAN_POINT('Ctrl Pts',(-11.3105661700983,22.9229866428742,2.84656620096894));
#92816=CARTESIAN_POINT('Ctrl Pts',(-11.2864155588632,22.9199336403855,2.80021771283935));
#92817=CARTESIAN_POINT('Ctrl Pts',(-11.2444023432422,22.9152330577863,2.72914658989345));
#92818=CARTESIAN_POINT('Ctrl Pts',(-11.2281593016871,22.9135336143108,2.70352206951157));
#92819=CARTESIAN_POINT('Ctrl Pts',(-11.2061909941863,22.9113786000927,2.67113754909324));
#92820=CARTESIAN_POINT('Ctrl Pts',(-11.2011856138087,22.9108964959853,2.66390024344747));
#92821=CARTESIAN_POINT('Ctrl Pts',(-11.1929651611424,22.9101188686488,2.65224044703891));
#92822=CARTESIAN_POINT('Ctrl Pts',(-11.1897900964486,22.9098218415531,2.64779012980379));
#92823=CARTESIAN_POINT('Ctrl Pts',(-11.1836514842201,22.9092538621523,2.63928714501705));
#92824=CARTESIAN_POINT('Ctrl Pts',(-11.1806918777961,22.9089827650489,2.6352317389013));
#92825=CARTESIAN_POINT('Ctrl Pts',(-11.173885989987,22.9083655306467,2.62600603163217));
#92826=CARTESIAN_POINT('Ctrl Pts',(-11.1700262960853,22.9080199165649,2.62084572314555));
#92827=CARTESIAN_POINT('Ctrl Pts',(-11.1597125685023,22.9071078886038,2.6072447688895));
#92828=CARTESIAN_POINT('Ctrl Pts',(-11.1532004181785,22.9065437398669,2.5988485434561));
#92829=CARTESIAN_POINT('Ctrl Pts',(-11.0987936786368,22.9019237642244,2.53025672947721));
#92830=CARTESIAN_POINT('Ctrl Pts',(-11.0463106533937,22.8980613861498,2.47384916700088));
#92831=CARTESIAN_POINT('Ctrl Pts',(-10.939578223559,22.8909457544782,2.37588217397486));
#92832=CARTESIAN_POINT('Ctrl Pts',(-10.8863884780223,22.8876805205979,2.33348235656279));
#92833=CARTESIAN_POINT('Ctrl Pts',(-10.7933382059773,22.8821303986175,2.26935882031832));
#92834=CARTESIAN_POINT('Ctrl Pts',(-10.7550707615303,22.8798873171283,2.24551570384066));
#92835=CARTESIAN_POINT('Ctrl Pts',(-10.7027153707901,22.8767907665733,2.21615917451802));
#92836=CARTESIAN_POINT('Ctrl Pts',(-10.6895525526661,22.8760099747101,2.20904167230537));
#92837=CARTESIAN_POINT('Ctrl Pts',(-10.6700477227002,22.8748463254496,2.19887827618754));
#92838=CARTESIAN_POINT('Ctrl Pts',(-10.6637888450575,22.8744719303134,2.1956740988806));
#92839=CARTESIAN_POINT('Ctrl Pts',(-10.6524777643006,22.8737931111861,2.18998598875085));
#92840=CARTESIAN_POINT('Ctrl Pts',(-10.6474338192235,22.8734896216981,2.18748585141701));
#92841=CARTESIAN_POINT('Ctrl Pts',(-10.6395090463834,22.8730113792248,2.18361456706637));
#92842=CARTESIAN_POINT('Ctrl Pts',(-10.6366378915162,22.8728378218714,2.18222360655009));
#92843=CARTESIAN_POINT('Ctrl Pts',(-10.6337541194724,22.8726631896323,2.18083815771796));
#92844=CARTESIAN_POINT('Ctrl Pts',(-10.6337459992963,22.8726626978972,2.18083425663901));
#92845=CARTESIAN_POINT('Ctrl Pts',(-10.6337297220678,22.8726617121891,2.18082643695011));
#92846=CARTESIAN_POINT('Ctrl Pts',(-10.6337215651112,22.8726612182218,2.18082251838698));
#92847=CARTESIAN_POINT('Ctrl Pts',(-10.633705214225,22.8726602280431,2.18081466368569));
#92848=CARTESIAN_POINT('Ctrl Pts',(-10.6336970201241,22.8726597318214,2.18081072746609));
#92849=CARTESIAN_POINT('Ctrl Pts',(-10.633680594533,22.8726587371086,2.18080283725454));
#92850=CARTESIAN_POINT('Ctrl Pts',(-10.6336723632717,22.8726582386314,2.18079888337332));
#92851=CARTESIAN_POINT('Ctrl Pts',(-10.6336558631569,22.8726572393953,2.18079095774359));
#92852=CARTESIAN_POINT('Ctrl Pts',(-10.6336475942764,22.8726567386348,2.18078698598296));
#92853=CARTESIAN_POINT('Ctrl Pts',(-10.6336310188618,22.8726557348283,2.1807790245675));
#92854=CARTESIAN_POINT('Ctrl Pts',(-10.633622712158,22.8726552317721,2.18077503483202));
#92855=CARTESIAN_POINT('Ctrl Pts',(-10.6336060607994,22.872654223356,2.18076703732665));
#92856=CARTESIAN_POINT('Ctrl Pts',(-10.6335977161272,22.8726537179952,2.18076302954923));
#92857=CARTESIAN_POINT('Ctrl Pts',(-10.6335809884122,22.8726527049444,2.18075499576115));
#92858=CARTESIAN_POINT('Ctrl Pts',(-10.6335726055373,22.8726521972647,2.180750969832));
#92859=CARTESIAN_POINT('Ctrl Pts',(-10.6310480371142,22.8724993047404,2.17953855935238));
#92860=CARTESIAN_POINT('Ctrl Pts',(-10.6285284620908,22.8723464723902,2.17833740564742));
#92861=CARTESIAN_POINT('Ctrl Pts',(-10.6227644868692,22.8719962972652,2.17560976289968));
#92862=CARTESIAN_POINT('Ctrl Pts',(-10.6195179130081,22.8717986715108,2.1740879889186));
#92863=CARTESIAN_POINT('Ctrl Pts',(-10.6110157468355,22.8712801770037,2.17014079272056));
#92864=CARTESIAN_POINT('Ctrl Pts',(-10.6057513522915,22.8709581889716,2.16773461690217));
#92865=CARTESIAN_POINT('Ctrl Pts',(-10.5701233442704,22.8687733939266,2.15170508824438));
#92866=CARTESIAN_POINT('Ctrl Pts',(-10.539319037039,22.866856876712,2.13909058391791));
#92867=CARTESIAN_POINT('Ctrl Pts',(-10.490951763895,22.8638343877516,2.12118401036187));
#92868=CARTESIAN_POINT('Ctrl Pts',(-10.4736721816777,22.8627519898839,2.11515278938161));
#92869=CARTESIAN_POINT('Ctrl Pts',(-10.3712266359488,22.8563360105673,2.08153714905513));
#92870=CARTESIAN_POINT('Ctrl Pts',(-10.2837862196306,22.8508796704172,2.06148943069912));
#92871=CARTESIAN_POINT('Ctrl Pts',(-10.1249924508596,22.8414016889792,2.0401345461916));
#92872=CARTESIAN_POINT('Ctrl Pts',(-10.0543292150462,22.8373288740529,2.03580025987142));
#92873=CARTESIAN_POINT('Ctrl Pts',(-9.97248175545239,22.8327991070005,2.03671633227608));
#92874=CARTESIAN_POINT('Ctrl Pts',(-9.96134419308052,22.8321865598913,2.03696818754709));
#92875=CARTESIAN_POINT('Ctrl Pts',(-9.94423725542512,22.8312514399127,2.03755051856193));
#92876=CARTESIAN_POINT('Ctrl Pts',(-9.93826538179682,22.8309260714968,2.03779043641578));
#92877=CARTESIAN_POINT('Ctrl Pts',(-9.92737938139554,22.8303348767917,2.03829458792155));
#92878=CARTESIAN_POINT('Ctrl Pts',(-9.92246481877847,22.8300686888562,2.03854703721307));
#92879=CARTESIAN_POINT('Ctrl Pts',(-9.91173580259414,22.8294890904623,2.03915243354299));
#92880=CARTESIAN_POINT('Ctrl Pts',(-9.90592197901186,22.8291759931195,2.03951531734213));
#92881=CARTESIAN_POINT('Ctrl Pts',(-9.88998290910093,22.8283202026221,2.04060576395182));
#92882=CARTESIAN_POINT('Ctrl Pts',(-9.87986271825187,22.8277797080709,2.04140398431158));
#92883=CARTESIAN_POINT('Ctrl Pts',(-9.82731287488445,22.8249871155621,2.04609944596996));
#92884=CARTESIAN_POINT('Ctrl Pts',(-9.78505800028072,22.8227898373998,2.05174310309314));
#92885=CARTESIAN_POINT('Ctrl Pts',(-9.60357328982192,22.8134731653276,2.08410216307224));
#92886=CARTESIAN_POINT('Ctrl Pts',(-9.46841375493798,22.8069204477127,2.12911363783852));
#92887=CARTESIAN_POINT('Ctrl Pts',(-9.31503733309478,22.7981697349257,2.20633884689591));
#92888=CARTESIAN_POINT('Ctrl Pts',(-9.28865381232147,22.7966091742222,2.22065665692394));
#92889=CARTESIAN_POINT('Ctrl Pts',(-9.25762089799422,22.79468449035,2.23875438063674));
#92890=CARTESIAN_POINT('Ctrl Pts',(-9.2525290487486,22.794365744567,2.24176535650229));
#92891=CARTESIAN_POINT('Ctrl Pts',(-9.24465523892611,22.7938680426169,2.24648605775432));
#92892=CARTESIAN_POINT('Ctrl Pts',(-9.24186045141881,22.7936904373678,2.24817439875327));
#92893=CARTESIAN_POINT('Ctrl Pts',(-9.23669081958393,22.7933601102193,2.25132105340545));
#92894=CARTESIAN_POINT('Ctrl Pts',(-9.23431447778206,22.7932075535382,2.25277680535463));
#92895=CARTESIAN_POINT('Ctrl Pts',(-9.22893613498647,22.7928606577584,2.25609275334152));
#92896=CARTESIAN_POINT('Ctrl Pts',(-9.22593671453192,22.7926660564008,2.25795702499085));
#92897=CARTESIAN_POINT('Ctrl Pts',(-9.21819044690254,22.7921605777362,2.26281062828502));
#92898=CARTESIAN_POINT('Ctrl Pts',(-9.21345403206892,22.7918486687422,2.26581640058524));
#92899=CARTESIAN_POINT('Ctrl Pts',(-9.18361006114819,22.789865931455,2.2849972258552));
#92900=CARTESIAN_POINT('Ctrl Pts',(-9.1589869212381,22.788151817656,2.3019094252259));
#92901=CARTESIAN_POINT('Ctrl Pts',(-9.05050753570982,22.7803015469432,2.38140997779612));
#92902=CARTESIAN_POINT('Ctrl Pts',(-8.97299146723634,22.7738853242976,2.45212898819746));
#92903=CARTESIAN_POINT('Ctrl Pts',(-8.86936332633942,22.7645914861725,2.56931411253569));
#92904=CARTESIAN_POINT('Ctrl Pts',(-8.83713057946245,22.761564342947,2.60991515808132));
#92905=CARTESIAN_POINT('Ctrl Pts',(-8.78964159187339,22.7568982410933,2.67672931779638));
#92906=CARTESIAN_POINT('Ctrl Pts',(-8.77293022254313,22.7552083562166,2.70185086433013));
#92907=CARTESIAN_POINT('Ctrl Pts',(-8.75237036170699,22.7530635250058,2.7349315926207));
#92908=CARTESIAN_POINT('Ctrl Pts',(-8.74780157353129,22.7525823531225,2.7424325193172));
#92909=CARTESIAN_POINT('Ctrl Pts',(-8.74050076516666,22.7518058559297,2.75466532860033));
#92910=CARTESIAN_POINT('Ctrl Pts',(-8.73772728104875,22.7515090348037,2.75937210486224));
#92911=CARTESIAN_POINT('Ctrl Pts',(-8.73245515423332,22.7509412038779,2.76843487645601));
#92912=CARTESIAN_POINT('Ctrl Pts',(-8.72995245301274,22.7506700509194,2.77278841093122));
#92913=CARTESIAN_POINT('Ctrl Pts',(-8.72428563435984,22.7500523529439,2.78276452218088));
#92914=CARTESIAN_POINT('Ctrl Pts',(-8.72113617735537,22.7497063339397,2.78839533567326));
#92915=CARTESIAN_POINT('Ctrl Pts',(-8.71288610292295,22.7487925203549,2.80337706255747));
#92916=CARTESIAN_POINT('Ctrl Pts',(-8.7078501070075,22.7482270053733,2.81276324092941));
#92917=CARTESIAN_POINT('Ctrl Pts',(-8.66665355199016,22.7435332994342,2.89160013638136));
#92918=CARTESIAN_POINT('Ctrl Pts',(-8.63601583884849,22.7396060759652,2.96379818617022));
#92919=CARTESIAN_POINT('Ctrl Pts',(-8.59039816304495,22.7325125468467,3.10095008341315));
#92920=CARTESIAN_POINT('Ctrl Pts',(-8.57378661896455,22.7293279832478,3.16513674912525));
#92921=CARTESIAN_POINT('Ctrl Pts',(-8.55323254667196,22.7238525722675,3.27473036813422));
#92922=CARTESIAN_POINT('Ctrl Pts',(-8.54695636824686,22.7215994634492,3.31959447999967));
#92923=CARTESIAN_POINT('Ctrl Pts',(-8.54068423888189,22.7181005954297,3.38713465360805));
#92924=CARTESIAN_POINT('Ctrl Pts',(-8.53911811063888,22.7169170246536,3.4096392169471));
#92925=CARTESIAN_POINT('Ctrl Pts',(-8.53782097584902,22.715415061166,3.43759599882887));
#92926=CARTESIAN_POINT('Ctrl Pts',(-8.53759942493791,22.7151219897871,3.44302356436409));
#92927=CARTESIAN_POINT('Ctrl Pts',(-8.5372968229345,22.7146558688001,3.4516094364999));
#92928=CARTESIAN_POINT('Ctrl Pts',(-8.5371957717898,22.7144839075952,3.45476704325511));
#92929=CARTESIAN_POINT('Ctrl Pts',(-8.53702435003934,22.7141582699073,3.46072715173168));
#92930=CARTESIAN_POINT('Ctrl Pts',(-8.53695180727693,22.7140047142547,3.46352954220039));
#92931=CARTESIAN_POINT('Ctrl Pts',(-8.5368037273368,22.7136510993821,3.46996468298871));
#92932=CARTESIAN_POINT('Ctrl Pts',(-8.53673366710158,22.7134507408156,3.47359751861213));
#92933=CARTESIAN_POINT('Ctrl Pts',(-8.53658253141766,22.7129131589034,3.48331054085524));
#92934=CARTESIAN_POINT('Ctrl Pts',(-8.53652582146499,22.7125746505804,3.48939096868958));
#92935=CARTESIAN_POINT('Ctrl Pts',(-8.53638325076678,22.7099955052644,3.53546573631324));
#92936=CARTESIAN_POINT('Ctrl Pts',(-8.53789900869216,22.7076775240428,3.57544504617879));
#92937=CARTESIAN_POINT('Ctrl Pts',(-8.54849305359739,22.6997433998366,3.70948718960912));
#92938=CARTESIAN_POINT('Ctrl Pts',(-8.56503787126248,22.6939704175269,3.80272389431009));
#92939=CARTESIAN_POINT('Ctrl Pts',(-8.60423299226438,22.6853189730104,3.94304614335));
#92940=CARTESIAN_POINT('Ctrl Pts',(-8.62059246009301,22.682327538178,3.99162083570523));
#92941=CARTESIAN_POINT('Ctrl Pts',(-8.65049543517712,22.6777091455558,4.06706754963956));
#92942=CARTESIAN_POINT('Ctrl Pts',(-8.66237576933256,22.6760325416527,4.09455006417245));
#92943=CARTESIAN_POINT('Ctrl Pts',(-8.67881187770535,22.6739018708786,4.12957995242003));
#92944=CARTESIAN_POINT('Ctrl Pts',(-8.68260362463712,22.6734220032802,4.13747609041152));
#92945=CARTESIAN_POINT('Ctrl Pts',(-8.68887277207805,22.6726470872648,4.15023644212917));
#92946=CARTESIAN_POINT('Ctrl Pts',(-8.69130685921244,22.6723505542669,4.15512159394418));
#92947=CARTESIAN_POINT('Ctrl Pts',(-8.69603352162394,22.6717829295593,4.16447641434488));
#92948=CARTESIAN_POINT('Ctrl Pts',(-8.69832188873457,22.6715116969924,4.16894811268964));
#92949=CARTESIAN_POINT('Ctrl Pts',(-8.7036068643279,22.6708933435004,4.1791456775413));
#92950=CARTESIAN_POINT('Ctrl Pts',(-8.70661847914049,22.6705467525397,4.18486367757874));
#92951=CARTESIAN_POINT('Ctrl Pts',(-8.71471126413086,22.66963041481,4.19998525419879));
#92952=CARTESIAN_POINT('Ctrl Pts',(-8.71985779380491,22.6690629681527,4.20935353005815));
#92953=CARTESIAN_POINT('Ctrl Pts',(-8.77191907131174,22.6634691476678,4.30170894273364));
#92954=CARTESIAN_POINT('Ctrl Pts',(-8.82673462887108,22.658751251724,4.37998369660948));
#92955=CARTESIAN_POINT('Ctrl Pts',(-8.94276960040558,22.6500618603562,4.51537139454248));
#92956=CARTESIAN_POINT('Ctrl Pts',(-9.0020133400753,22.6460821487852,4.57365544564109));
#92957=CARTESIAN_POINT('Ctrl Pts',(-9.09121922817761,22.6402021306045,4.64762105758992));
#92958=CARTESIAN_POINT('Ctrl Pts',(-9.11726849491881,22.6384957524693,4.66777624396315));
#92959=CARTESIAN_POINT('Ctrl Pts',(-9.14889274793297,22.6364079045773,4.69058199347438));
#92960=CARTESIAN_POINT('Ctrl Pts',(-9.15383417936643,22.636081211939,4.69409900725277));
#92961=CARTESIAN_POINT('Ctrl Pts',(-9.16149559774753,22.6355737545293,4.69948050877862));
#92962=CARTESIAN_POINT('Ctrl Pts',(-9.16420032366015,22.6353944269104,4.70136673173851));
#92963=CARTESIAN_POINT('Ctrl Pts',(-9.16920047831088,22.6350625341961,4.70482868354144));
#92964=CARTESIAN_POINT('Ctrl Pts',(-9.17149404215828,22.6349101473326,4.7064070123273));
#92965=CARTESIAN_POINT('Ctrl Pts',(-9.17667281855228,22.6345657336821,4.70994908275563));
#92966=CARTESIAN_POINT('Ctrl Pts',(-9.17956054240587,22.6343734606614,4.71190904216155));
#92967=CARTESIAN_POINT('Ctrl Pts',(-9.18699497091596,22.6338779358729,4.71691619709011));
#92968=CARTESIAN_POINT('Ctrl Pts',(-9.19155176818449,22.6335737172127,4.71994822128145));
#92969=CARTESIAN_POINT('Ctrl Pts',(-9.21913457863256,22.6317297943003,4.73807900192011));
#92970=CARTESIAN_POINT('Ctrl Pts',(-9.24256455991984,22.6301533034055,4.75255010906952));
#92971=CARTESIAN_POINT('Ctrl Pts',(-9.35847478967007,22.6223572920333,4.81969836048252));
#92972=CARTESIAN_POINT('Ctrl Pts',(-9.45610518015055,22.6158270129194,4.86284161023424));
#92973=CARTESIAN_POINT('Ctrl Pts',(-9.62506051372539,22.6052915413896,4.91642809731541));
#92974=CARTESIAN_POINT('Ctrl Pts',(-9.694041148166,22.6011795437054,4.93291296673286));
#92975=CARTESIAN_POINT('Ctrl Pts',(-9.77982123375063,22.5963276866793,4.94693196239669));
#92976=CARTESIAN_POINT('Ctrl Pts',(-9.79573206100958,22.5954382363144,4.94926375481091));
#92977=CARTESIAN_POINT('Ctrl Pts',(-9.81854446093554,22.5941775312039,4.95222383668252));
#92978=CARTESIAN_POINT('Ctrl Pts',(-9.82541669103518,22.5937996235824,4.95306601881147));
#92979=CARTESIAN_POINT('Ctrl Pts',(-9.83734016167326,22.593147138594,4.95444141242383));
#92980=CARTESIAN_POINT('Ctrl Pts',(-9.84238863938118,22.5928718622089,4.95499714951122));
#92981=CARTESIAN_POINT('Ctrl Pts',(-9.85210384147005,22.5923439960224,4.95601544192326));
#92982=CARTESIAN_POINT('Ctrl Pts',(-9.85677008976282,22.592091288654,4.9564818688694));
#92983=CARTESIAN_POINT('Ctrl Pts',(-9.86778974556372,22.591496423386,4.95752989723281));
#92984=CARTESIAN_POINT('Ctrl Pts',(-9.8741449025253,22.5911548630033,4.95809240067142));
#92985=CARTESIAN_POINT('Ctrl Pts',(-9.8963724763953,22.5899653425686,4.95991338701998));
#92986=CARTESIAN_POINT('Ctrl Pts',(-9.9122618919183,22.5891241248389,4.96095441809888));
#92987=CARTESIAN_POINT('Ctrl Pts',(-10.0523400549234,22.5817811305488,4.96783831305953));
#92988=CARTESIAN_POINT('Ctrl Pts',(-10.1767821266354,22.5758204370791,4.95809436211311));
#92989=CARTESIAN_POINT('Ctrl Pts',(-10.352786077654,22.5670507395725,4.92142495588696));
#92990=CARTESIAN_POINT('Ctrl Pts',(-10.4063800518975,22.5643228853359,4.90703992533168));
#92991=CARTESIAN_POINT('Ctrl Pts',(-10.4832964210507,22.5601658805956,4.88163316941541));
#92992=CARTESIAN_POINT('Ctrl Pts',(-10.5073525058914,22.5588296684193,4.87298176333184));
#92993=CARTESIAN_POINT('Ctrl Pts',(-10.5364301773216,22.5571562520763,4.86165590506921));
#92994=CARTESIAN_POINT('Ctrl Pts',(-10.5416801496039,22.5568517623694,4.85957594579463));
#92995=CARTESIAN_POINT('Ctrl Pts',(-10.5498921626083,22.5563715861309,4.85626735636548));
#92996=CARTESIAN_POINT('Ctrl Pts',(-10.5528624832187,22.5561971017345,4.85505926316343));
#92997=CARTESIAN_POINT('Ctrl Pts',(-10.5584137120274,22.5558694618426,4.85278016852993));
#92998=CARTESIAN_POINT('Ctrl Pts',(-10.5609955360152,22.5557164474096,4.85171153220216));
#92999=CARTESIAN_POINT('Ctrl Pts',(-10.566911733211,22.555364376178,4.84924290427161));
#93000=CARTESIAN_POINT('Ctrl Pts',(-10.5702439808846,22.5551650246104,4.8478379463667));
#93001=CARTESIAN_POINT('Ctrl Pts',(-10.5789906386521,22.55463905706,4.84411189779674));
#93002=CARTESIAN_POINT('Ctrl Pts',(-10.5843962454322,22.5543112700257,4.84177046449532));
#93003=CARTESIAN_POINT('Ctrl Pts',(-10.6221557598251,22.5520031963805,4.82514350701536));
#93004=CARTESIAN_POINT('Ctrl Pts',(-10.6539943130848,22.549962301649,4.80972292829475));
#93005=CARTESIAN_POINT('Ctrl Pts',(-10.7254993130253,22.5452091159894,4.77183287634479));
#93006=CARTESIAN_POINT('Ctrl Pts',(-10.7647384705003,22.5424758684529,4.74863239749089));
#93007=CARTESIAN_POINT('Ctrl Pts',(-10.9060906270905,22.5323002412033,4.65589133514381));
#93008=CARTESIAN_POINT('Ctrl Pts',(-11.0003808480297,22.5248957318843,4.57532969754823));
#93009=CARTESIAN_POINT('Ctrl Pts',(-11.0940584743266,22.5171208528616,4.47217175681321));
#93010=CARTESIAN_POINT('Ctrl Pts',(-11.1044901012918,22.5162471505228,4.46030386526878));
#93011=CARTESIAN_POINT('Ctrl Pts',(-11.1191823929969,22.5150046261628,4.44303249467248));
#93012=CARTESIAN_POINT('Ctrl Pts',(-11.1236000810993,22.5146294114197,4.43776456257167));
#93013=CARTESIAN_POINT('Ctrl Pts',(-11.1312112287079,22.5139800759859,4.42855754616877));
#93014=CARTESIAN_POINT('Ctrl Pts',(-11.1344216149669,22.5137052748293,4.42463266268131));
#93015=CARTESIAN_POINT('Ctrl Pts',(-11.140568990456,22.5131772752128,4.41703692816707));
#93016=CARTESIAN_POINT('Ctrl Pts',(-11.1435088134412,22.5129239653447,4.41336846009926));
#93017=CARTESIAN_POINT('Ctrl Pts',(-11.1504248939997,22.512326082151,4.40465247469064));
#93018=CARTESIAN_POINT('Ctrl Pts',(-11.1543857051605,22.5119821214191,4.39959278688027));
#93019=CARTESIAN_POINT('Ctrl Pts',(-11.1682100304846,22.5107759287708,4.38169142327106));
#93020=CARTESIAN_POINT('Ctrl Pts',(-11.1778938225474,22.5099206952712,4.36871204172841));
#93021=CARTESIAN_POINT('Ctrl Pts',(-11.2583371411775,22.5027194438443,4.2570733205469));
#93022=CARTESIAN_POINT('Ctrl Pts',(-11.3167803750904,22.496885062275,4.15012633511043));
#93023=CARTESIAN_POINT('Ctrl Pts',(-11.3824075122001,22.4881708618385,3.98381162221937));
#93024=CARTESIAN_POINT('Ctrl Pts',(-11.400309287888,22.4853539038468,3.92925193913991));
#93025=CARTESIAN_POINT('Ctrl Pts',(-11.4216235868321,22.4810749154837,3.84856712176743));
#93026=CARTESIAN_POINT('Ctrl Pts',(-11.427609928413,22.4797122288226,3.82317547311844));
#93027=CARTESIAN_POINT('Ctrl Pts',(-11.4340697085064,22.4780091281776,3.79207635968033));
#93028=CARTESIAN_POINT('Ctrl Pts',(-11.4351927488141,22.4777028109347,3.78650706860523));
#93029=CARTESIAN_POINT('Ctrl Pts',(-11.4369003020955,22.4772203864281,3.77777707382073));
#93030=CARTESIAN_POINT('Ctrl Pts',(-11.4375068908089,22.47704549995,3.77462068270932));
#93031=CARTESIAN_POINT('Ctrl Pts',(-11.4386211642336,22.4767175259073,3.76871769088514));
#93032=CARTESIAN_POINT('Ctrl Pts',(-11.4391313865424,22.4765645825659,3.7659716214551));
#93033=CARTESIAN_POINT('Ctrl Pts',(-11.4402820754215,22.4762132330069,3.75967823707123));
#93034=CARTESIAN_POINT('Ctrl Pts',(-11.4409172976905,22.4760145364928,3.75613001431306));
#93035=CARTESIAN_POINT('Ctrl Pts',(-11.4425493561025,22.4754914094448,3.74681541708485));
#93036=CARTESIAN_POINT('Ctrl Pts',(-11.4435247157383,22.4751658276659,3.74104540572246));
#93037=CARTESIAN_POINT('Ctrl Pts',(-11.4500263477957,22.4729036216027,3.70112790356265));
#93038=CARTESIAN_POINT('Ctrl Pts',(-11.4543746179919,22.4709089950979,3.66680210651175));
#93039=CARTESIAN_POINT('Ctrl Pts',(-11.4614622886472,22.4663096565819,3.58875359134485));
#93040=CARTESIAN_POINT('Ctrl Pts',(-11.4634631165743,22.4636863066559,3.5449957527342));
#93041=CARTESIAN_POINT('Ctrl Pts',(-11.4634998316009,22.4610279215406,3.50081071340477));
#93042=CARTESIAN_POINT('Ctrl Pts',(-11.4635,22.4610035323129,3.50040535415972));
#93043=CARTESIAN_POINT('Ctrl Pts',(-11.4635,22.4609791425484,3.50000000009405));
#93044=CARTESIAN_POINT('',(-11.463499731436,22.8886344895975,3.49895700858923));
#93045=CARTESIAN_POINT('Ctrl Pts',(-11.4635,22.3887666433152,3.49999999992021));
#93046=CARTESIAN_POINT('Ctrl Pts',(-11.4635,22.3887864753112,3.50040515578243));
#93047=CARTESIAN_POINT('Ctrl Pts',(-11.4634998317572,22.3888063096356,3.50081031697022));
#93048=CARTESIAN_POINT('Ctrl Pts',(-11.4634414153931,22.3922499147876,3.5711463205363));
#93049=CARTESIAN_POINT('Ctrl Pts',(-11.4583710933305,22.3957287202161,3.64097534271047));
#93050=CARTESIAN_POINT('Ctrl Pts',(-11.4472875942407,22.3998459927665,3.71735608274318));
#93051=CARTESIAN_POINT('Ctrl Pts',(-11.4461906229825,22.4002362853658,3.72453891598871));
#93052=CARTESIAN_POINT('Ctrl Pts',(-11.444478747129,22.4008213923889,3.73521474365312));
#93053=CARTESIAN_POINT('Ctrl Pts',(-11.4439045419782,22.4010139935623,3.73871426361317));
#93054=CARTESIAN_POINT('Ctrl Pts',(-11.4428560750092,22.401359337681,3.74496198547646));
#93055=CARTESIAN_POINT('Ctrl Pts',(-11.4423866719365,22.4015118065534,3.7477109524882));
#93056=CARTESIAN_POINT('Ctrl Pts',(-11.441352114708,22.4018432907535,3.75366697789371));
#93057=CARTESIAN_POINT('Ctrl Pts',(-11.4407841210342,22.4020224593706,3.75687345210515));
#93058=CARTESIAN_POINT('Ctrl Pts',(-11.4391619377477,22.4025263464491,3.76585643968429));
#93059=CARTESIAN_POINT('Ctrl Pts',(-11.4380836895846,22.4028523756356,3.77162847594833));
#93060=CARTESIAN_POINT('Ctrl Pts',(-11.4314354600568,22.4048105108482,3.80606800764421));
#93061=CARTESIAN_POINT('Ctrl Pts',(-11.4250434955166,22.4064841137481,3.83456823090937));
#93062=CARTESIAN_POINT('Ctrl Pts',(-11.3853258268499,22.4158211782022,3.98975885778564));
#93063=CARTESIAN_POINT('Ctrl Pts',(-11.3359576300993,22.4239209942555,4.11173045469656));
#93064=CARTESIAN_POINT('Ctrl Pts',(-11.2643770012013,22.4323484510507,4.23713093768342));
#93065=CARTESIAN_POINT('Ctrl Pts',(-11.2575859048152,22.4331248972202,4.24865808397973));
#93066=CARTESIAN_POINT('Ctrl Pts',(-11.2293459393181,22.4362611205455,4.29512353940633));
#93067=CARTESIAN_POINT('Ctrl Pts',(-11.2065904314168,22.4385785969067,4.32924838239373));
#93068=CARTESIAN_POINT('Ctrl Pts',(-11.176518551953,22.4413972610217,4.37048090032699));
#93069=CARTESIAN_POINT('Ctrl Pts',(-11.1705235596547,22.4419481707111,4.37852575617457));
#93070=CARTESIAN_POINT('Ctrl Pts',(-11.1609334320775,22.4428124716891,4.39112257620886));
#93071=CARTESIAN_POINT('Ctrl Pts',(-11.1573932259788,22.4431279829346,4.39571580389915));
#93072=CARTESIAN_POINT('Ctrl Pts',(-11.1507968221072,22.4437094049003,4.40416987808131));
#93073=CARTESIAN_POINT('Ctrl Pts',(-11.1477482716439,22.4439756099944,4.40803656311885));
#93074=CARTESIAN_POINT('Ctrl Pts',(-11.1409351656734,22.4445650605231,4.41658896131871));
#93075=CARTESIAN_POINT('Ctrl Pts',(-11.1371611295861,22.4448879238874,4.42126703138382));
#93076=CARTESIAN_POINT('Ctrl Pts',(-11.1262122810549,22.4458142340023,4.43466877790436));
#93077=CARTESIAN_POINT('Ctrl Pts',(-11.1189650705888,22.44641477371,4.44333292464552));
#93078=CARTESIAN_POINT('Ctrl Pts',(-11.0621510974471,22.4510286227644,4.50967877619092));
#93079=CARTESIAN_POINT('Ctrl Pts',(-11.0082541199108,22.4548531801478,4.56350446287798));
#93080=CARTESIAN_POINT('Ctrl Pts',(-10.883461342075,22.4629211200718,4.67007675353308));
#93081=CARTESIAN_POINT('Ctrl Pts',(-10.8114919256778,22.4671179684292,4.7210910054779));
#93082=CARTESIAN_POINT('Ctrl Pts',(-10.72629793268,22.4720307904386,4.77060373689243));
#93083=CARTESIAN_POINT('Ctrl Pts',(-10.7171615562358,22.4725571427608,4.77578283379038));
#93084=CARTESIAN_POINT('Ctrl Pts',(-10.6758909548467,22.4749358702569,4.79859429861302));
#93085=CARTESIAN_POINT('Ctrl Pts',(-10.6431591778464,22.476825302443,4.81511276584703));
#93086=CARTESIAN_POINT('Ctrl Pts',(-10.6044353346551,22.4791024017168,4.83286367880385));
#93087=CARTESIAN_POINT('Ctrl Pts',(-10.5990109719022,22.4794223072308,4.8353102685113));
#93088=CARTESIAN_POINT('Ctrl Pts',(-10.5902849268182,22.4799386571361,4.83918217088102));
#93089=CARTESIAN_POINT('Ctrl Pts',(-10.5869925928706,22.480133867515,4.84062853803226));
#93090=CARTESIAN_POINT('Ctrl Pts',(-10.5811277770254,22.4804823587555,4.84317928589764));
#93091=CARTESIAN_POINT('Ctrl Pts',(-10.5785574194492,22.4806353488974,4.84428843616002));
#93092=CARTESIAN_POINT('Ctrl Pts',(-10.5730572266018,22.4809632942659,4.84664315986661));
#93093=CARTESIAN_POINT('Ctrl Pts',(-10.5701265510248,22.4811383723668,4.84788653097856));
#93094=CARTESIAN_POINT('Ctrl Pts',(-10.5620856910867,22.4816196107549,4.85126703776691));
#93095=CARTESIAN_POINT('Ctrl Pts',(-10.556967448217,22.4819269025589,4.85338471658757));
#93096=CARTESIAN_POINT('Ctrl Pts',(-10.5296264381595,22.4835730885363,4.86451573052521));
#93097=CARTESIAN_POINT('Ctrl Pts',(-10.5071978644269,22.4849398555446,4.87301039038172));
#93098=CARTESIAN_POINT('Ctrl Pts',(-10.4374726871198,22.4892169015712,4.89747679838489));
#93099=CARTESIAN_POINT('Ctrl Pts',(-10.389561225325,22.4921940506583,4.91158251923256));
#93100=CARTESIAN_POINT('Ctrl Pts',(-10.2187042126284,22.5027498596996,4.95252279674843));
#93101=CARTESIAN_POINT('Ctrl Pts',(-10.0930883918712,22.5103436952666,4.96594655266575));
#93102=CARTESIAN_POINT('Ctrl Pts',(-9.94719455106615,22.5185445538024,4.96268519073684));
#93103=CARTESIAN_POINT('Ctrl Pts',(-9.92710725936704,22.5196617784042,4.96182183850248));
#93104=CARTESIAN_POINT('Ctrl Pts',(-9.89926200125617,22.5211945809215,4.96004962279458));
#93105=CARTESIAN_POINT('Ctrl Pts',(-9.89148458351597,22.5216209854787,4.9594921901468));
#93106=CARTESIAN_POINT('Ctrl Pts',(-9.87900101644436,22.5223027231859,4.95849711321739));
#93107=CARTESIAN_POINT('Ctrl Pts',(-9.87429195693191,22.5225592742618,4.95809878675033));
#93108=CARTESIAN_POINT('Ctrl Pts',(-9.86454776042906,22.5230888957556,4.95722699548386));
#93109=CARTESIAN_POINT('Ctrl Pts',(-9.85951297723979,22.5233618595618,4.956750226667));
#93110=CARTESIAN_POINT('Ctrl Pts',(-9.84772754396771,22.5239992414438,4.95557253682056));
#93111=CARTESIAN_POINT('Ctrl Pts',(-9.84097906594481,22.5243630037593,4.95485073305045));
#93112=CARTESIAN_POINT('Ctrl Pts',(-9.81904237227039,22.525541678257,4.95234996691129));
#93113=CARTESIAN_POINT('Ctrl Pts',(-9.80387669397077,22.5263506316995,4.95037986800109));
#93114=CARTESIAN_POINT('Ctrl Pts',(-9.72514010678688,22.530523389766,4.93889397453724));
#93115=CARTESIAN_POINT('Ctrl Pts',(-9.66221303996137,22.5337617301061,4.92543502397663));
#93116=CARTESIAN_POINT('Ctrl Pts',(-9.50314940943004,22.5419183568554,4.88028440052389));
#93117=CARTESIAN_POINT('Ctrl Pts',(-9.40905612180236,22.5467051003403,4.84269456087022));
#93118=CARTESIAN_POINT('Ctrl Pts',(-9.28463538804256,22.5537686416941,4.77735843630602));
#93119=CARTESIAN_POINT('Ctrl Pts',(-9.25043951768621,22.5557974036299,4.75759678468063));
#93120=CARTESIAN_POINT('Ctrl Pts',(-9.21196450136535,22.5582307368725,4.73323520340183));
#93121=CARTESIAN_POINT('Ctrl Pts',(-9.20686201993588,22.5585566041021,4.72995981888036));
#93122=CARTESIAN_POINT('Ctrl Pts',(-9.19873835479184,22.5590807381084,4.72467350596726));
#93123=CARTESIAN_POINT('Ctrl Pts',(-9.19570398826674,22.5592777108738,4.72268284736137));
#93124=CARTESIAN_POINT('Ctrl Pts',(-9.19033865550719,22.5596281812374,4.71913437216778));
#93125=CARTESIAN_POINT('Ctrl Pts',(-9.18800472399327,22.559781375924,4.71758111919497));
#93126=CARTESIAN_POINT('Ctrl Pts',(-9.18304650777291,22.5601084199452,4.71426078359355));
#93127=CARTESIAN_POINT('Ctrl Pts',(-9.1804235274089,22.5602823836695,4.71249192336214));
#93128=CARTESIAN_POINT('Ctrl Pts',(-9.17329830821541,22.5607574997561,4.70765320234867));
#93129=CARTESIAN_POINT('Ctrl Pts',(-9.16880749336588,22.5610597371712,4.70456671020674));
#93130=CARTESIAN_POINT('Ctrl Pts',(-9.14564520508725,22.5626326197223,4.68845630205375));
#93131=CARTESIAN_POINT('Ctrl Pts',(-9.12726320025808,22.5639283412568,4.67502376884263));
#93132=CARTESIAN_POINT('Ctrl Pts',(-9.07275907440296,22.567897499983,4.63321063302459));
#93133=CARTESIAN_POINT('Ctrl Pts',(-9.03765364698384,22.5706280636724,4.60355383027538));
#93134=CARTESIAN_POINT('Ctrl Pts',(-8.96104735560925,22.576898838187,4.53239855890177));
#93135=CARTESIAN_POINT('Ctrl Pts',(-8.92052698077911,22.5804473722342,4.48995333718377));
#93136=CARTESIAN_POINT('Ctrl Pts',(-8.82784427719296,22.5890119061862,4.38039047884784));
#93137=CARTESIAN_POINT('Ctrl Pts',(-8.77876148970576,22.5939496597367,4.31093574509366));
#93138=CARTESIAN_POINT('Ctrl Pts',(-8.73056857989218,22.5992490905748,4.22834816152548));
#93139=CARTESIAN_POINT('Ctrl Pts',(-8.72526732849789,22.5998395876382,4.21902976263872));
#93140=CARTESIAN_POINT('Ctrl Pts',(-8.7169300870781,22.6007807728254,4.20399271866026));
#93141=CARTESIAN_POINT('Ctrl Pts',(-8.71382888898637,22.6011337666144,4.19831083655522));
#93142=CARTESIAN_POINT('Ctrl Pts',(-8.70838683153946,22.6017584798298,4.18818088804253));
#93143=CARTESIAN_POINT('Ctrl Pts',(-8.70603101286213,22.602030723746,4.18374101296351));
#93144=CARTESIAN_POINT('Ctrl Pts',(-8.70116572675879,22.6025968158955,4.17445648284007));
#93145=CARTESIAN_POINT('Ctrl Pts',(-8.69866038114204,22.6028905167333,4.16960974760642));
#93146=CARTESIAN_POINT('Ctrl Pts',(-8.69221027626545,22.6036524994976,4.156958715662));
#93147=CARTESIAN_POINT('Ctrl Pts',(-8.688308223726,22.6041192932145,4.14913280930692));
#93148=CARTESIAN_POINT('Ctrl Pts',(-8.67143169860479,22.6061648174623,4.11451184381907));
#93149=CARTESIAN_POINT('Ctrl Pts',(-8.65920596021384,22.6077177893871,4.08735852891814));
#93150=CARTESIAN_POINT('Ctrl Pts',(-8.62838014972795,22.6118557861262,4.01290614814757));
#93151=CARTESIAN_POINT('Ctrl Pts',(-8.61140075924212,22.6143907918847,3.96498001105964));
#93152=CARTESIAN_POINT('Ctrl Pts',(-8.5824091863414,22.6194021548061,3.86726182230662));
#93153=CARTESIAN_POINT('Ctrl Pts',(-8.57044768130865,22.621874729861,3.81752984479307));
#93154=CARTESIAN_POINT('Ctrl Pts',(-8.5470523962627,22.6281143211862,3.69157981223646));
#93155=CARTESIAN_POINT('Ctrl Pts',(-8.53898854594407,22.6318914986452,3.61490202496454));
#93156=CARTESIAN_POINT('Ctrl Pts',(-8.53669852566943,22.6365488222445,3.52663329570811));
#93157=CARTESIAN_POINT('Ctrl Pts',(-8.53653623689309,22.6371522753425,3.51530802586005));
#93158=CARTESIAN_POINT('Ctrl Pts',(-8.53649351503026,22.6379983820729,3.4996079979015));
#93159=CARTESIAN_POINT('Ctrl Pts',(-8.53650122439319,22.6382351519513,3.49523365804045));
#93160=CARTESIAN_POINT('Ctrl Pts',(-8.53654500298769,22.6386162832846,3.48822435302707));
#93161=CARTESIAN_POINT('Ctrl Pts',(-8.53656857841696,22.6387599581613,3.485589301262));
#93162=CARTESIAN_POINT('Ctrl Pts',(-8.53663268604307,22.6390608965735,3.48008554270168));
#93163=CARTESIAN_POINT('Ctrl Pts',(-8.53667453709305,22.63921823512,3.47721688554606));
#93164=CARTESIAN_POINT('Ctrl Pts',(-8.53679654829945,22.6396011210742,3.47025685106362));
#93165=CARTESIAN_POINT('Ctrl Pts',(-8.5368854341287,22.639827146003,3.46616566415688));
#93166=CARTESIAN_POINT('Ctrl Pts',(-8.53725972763587,22.6406281068654,3.45172679953076));
#93167=CARTESIAN_POINT('Ctrl Pts',(-8.53763775586047,22.6412078651074,3.44138207833712));
#93168=CARTESIAN_POINT('Ctrl Pts',(-8.54062012861015,22.6447838264441,3.37815679354885));
#93169=CARTESIAN_POINT('Ctrl Pts',(-8.54598259541785,22.6479030951848,3.32544983487339));
#93170=CARTESIAN_POINT('Ctrl Pts',(-8.5696521625787,22.657028497248,3.1745905257829));
#93171=CARTESIAN_POINT('Ctrl Pts',(-8.59515715009997,22.6631050551889,3.07785567250033));
#93172=CARTESIAN_POINT('Ctrl Pts',(-8.63541009758138,22.6697776582425,2.97090976213766));
#93173=CARTESIAN_POINT('Ctrl Pts',(-8.64071389204297,22.67061842507,2.95742892043499));
#93174=CARTESIAN_POINT('Ctrl Pts',(-8.66161464579819,22.6737902041093,2.90653585103432));
#93175=CARTESIAN_POINT('Ctrl Pts',(-8.6785640213756,22.6760806892185,2.8696965342615));
#93176=CARTESIAN_POINT('Ctrl Pts',(-8.7015746585457,22.6788715919741,2.82470463045362));
#93177=CARTESIAN_POINT('Ctrl Pts',(-8.70621819402671,22.6794205601664,2.8158502729913));
#93178=CARTESIAN_POINT('Ctrl Pts',(-8.71369423279636,22.6802824957722,2.80194322553294));
#93179=CARTESIAN_POINT('Ctrl Pts',(-8.71646656441212,22.680597564009,2.79685868547283));
#93180=CARTESIAN_POINT('Ctrl Pts',(-8.72167497630141,22.681181141717,2.78743975487316));
#93181=CARTESIAN_POINT('Ctrl Pts',(-8.72410309731634,22.6814499274489,2.78310107845231));
#93182=CARTESIAN_POINT('Ctrl Pts',(-8.72953039706457,22.6820435649402,2.77351825028911));
#93183=CARTESIAN_POINT('Ctrl Pts',(-8.73254004097025,22.682368037936,2.76828010933189));
#93184=CARTESIAN_POINT('Ctrl Pts',(-8.741343005884,22.6833036776209,2.75317625109079));
#93185=CARTESIAN_POINT('Ctrl Pts',(-8.74721975983142,22.683911843915,2.74335951700131));
#93186=CARTESIAN_POINT('Ctrl Pts',(-8.79624458086464,22.6888555074478,2.66360403823154));
#93187=CARTESIAN_POINT('Ctrl Pts',(-8.8450998973512,22.6929679573975,2.59734096251965));
#93188=CARTESIAN_POINT('Ctrl Pts',(-8.95081886252593,22.7008277252456,2.47668640122467));
#93189=CARTESIAN_POINT('Ctrl Pts',(-9.00700469158878,22.7045730324335,2.42208009176569));
#93190=CARTESIAN_POINT('Ctrl Pts',(-9.08007448707135,22.7092848832404,2.36164818997359));
#93191=CARTESIAN_POINT('Ctrl Pts',(-9.0930448151381,22.7101160606059,2.35128765136581));
#93192=CARTESIAN_POINT('Ctrl Pts',(-9.13327206936112,22.7126873021239,2.32026068537524));
#93193=CARTESIAN_POINT('Ctrl Pts',(-9.16107792589567,22.7144554446702,2.30032856113271));
#93194=CARTESIAN_POINT('Ctrl Pts',(-9.19441224937206,22.7165962941725,2.2781593124847));
#93195=CARTESIAN_POINT('Ctrl Pts',(-9.19928952173482,22.7169100458983,2.27495754467257));
#93196=CARTESIAN_POINT('Ctrl Pts',(-9.20720698261587,22.7174204218165,2.26982747478636));
#93197=CARTESIAN_POINT('Ctrl Pts',(-9.21023541875867,22.7176158875706,2.26788104638606));
#93198=CARTESIAN_POINT('Ctrl Pts',(-9.21562651509707,22.7179643411153,2.26444413730028));
#93199=CARTESIAN_POINT('Ctrl Pts',(-9.21798629426919,22.7181170345464,2.262949225944));
#93200=CARTESIAN_POINT('Ctrl Pts',(-9.22307474343982,22.7184466700936,2.2597460909196));
#93201=CARTESIAN_POINT('Ctrl Pts',(-9.22580473291283,22.7186237501001,2.25804013701011));
#93202=CARTESIAN_POINT('Ctrl Pts',(-9.23338518222181,22.7191160351367,2.25333786606279));
#93203=CARTESIAN_POINT('Ctrl Pts',(-9.23824750241473,22.7194324576396,2.25036089799427));
#93204=CARTESIAN_POINT('Ctrl Pts',(-9.26569853111618,22.721221998116,2.23377368023433));
#93205=CARTESIAN_POINT('Ctrl Pts',(-9.28863318567846,22.7227289026172,2.22074833709387));
#93206=CARTESIAN_POINT('Ctrl Pts',(-9.36349016166762,22.7276544911791,2.18087013012933));
#93207=CARTESIAN_POINT('Ctrl Pts',(-9.41667185743574,22.7311626819627,2.15650607990044));
#93208=CARTESIAN_POINT('Ctrl Pts',(-9.58286126871001,22.7418934069023,2.09210175433712));
#93209=CARTESIAN_POINT('Ctrl Pts',(-9.69947160524684,22.7490656316642,2.06268490817348));
#93210=CARTESIAN_POINT('Ctrl Pts',(-9.83457843120436,22.7566733659988,2.04578731457639));
#93211=CARTESIAN_POINT('Ctrl Pts',(-9.85081269514866,22.7575772843953,2.04403227773033));
#93212=CARTESIAN_POINT('Ctrl Pts',(-9.87349634966723,22.758826482709,2.04196341822132));
#93213=CARTESIAN_POINT('Ctrl Pts',(-9.87992316449001,22.7591788695553,2.0414200732242));
#93214=CARTESIAN_POINT('Ctrl Pts',(-9.89104746321068,22.7597862081531,2.04055361101967));
#93215=CARTESIAN_POINT('Ctrl Pts',(-9.89574326661374,22.7600417738813,2.04021064812564));
#93216=CARTESIAN_POINT('Ctrl Pts',(-9.90549741223821,22.7605709925661,2.03954555007214));
#93217=CARTESIAN_POINT('Ctrl Pts',(-9.91055594269594,22.7608445300248,2.03922701937872));
#93218=CARTESIAN_POINT('Ctrl Pts',(-9.92245935497029,22.7614860876628,2.03853953692759));
#93219=CARTESIAN_POINT('Ctrl Pts',(-9.9293054091789,22.7618534262664,2.03819238141261));
#93220=CARTESIAN_POINT('Ctrl Pts',(-9.95181444004333,22.7630559655072,2.03720947251223));
#93221=CARTESIAN_POINT('Ctrl Pts',(-9.9674855009764,22.7638848601518,2.0367772528237));
#93222=CARTESIAN_POINT('Ctrl Pts',(-10.1002298403708,22.7708421441393,2.03524978859578));
#93223=CARTESIAN_POINT('Ctrl Pts',(-10.217036074077,22.7764968213933,2.04795409076538));
#93224=CARTESIAN_POINT('Ctrl Pts',(-10.4092654661118,22.7861016063849,2.09259982242306));
#93225=CARTESIAN_POINT('Ctrl Pts',(-10.4858075344022,22.7900266848575,2.11715452202747));
#93226=CARTESIAN_POINT('Ctrl Pts',(-10.5704196880202,22.7948569382465,2.15219354125984));
#93227=CARTESIAN_POINT('Ctrl Pts',(-10.5808467652359,22.7954611601564,2.1566542178859));
#93228=CARTESIAN_POINT('Ctrl Pts',(-10.595224340333,22.7963081784401,2.1630035936448));
#93229=CARTESIAN_POINT('Ctrl Pts',(-10.5992200510468,22.7965450745061,2.1647896288009));
#93230=CARTESIAN_POINT('Ctrl Pts',(-10.6056089803002,22.7969263570545,2.16767985847276));
#93231=CARTESIAN_POINT('Ctrl Pts',(-10.6080073640733,22.7970700559468,2.16877265595065));
#93232=CARTESIAN_POINT('Ctrl Pts',(-10.6130099511688,22.7973709963732,2.17106836944284));
#93233=CARTESIAN_POINT('Ctrl Pts',(-10.6156135749375,22.7975283126558,2.17227246589962));
#93234=CARTESIAN_POINT('Ctrl Pts',(-10.6218463179888,22.7979065360459,2.17517719311851));
#93235=CARTESIAN_POINT('Ctrl Pts',(-10.6254720142168,22.7981278824866,2.17688508757524));
#93236=CARTESIAN_POINT('Ctrl Pts',(-10.6380206811357,22.7988984623876,2.1828592780222));
#93237=CARTESIAN_POINT('Ctrl Pts',(-10.6469071845318,22.799452061825,2.18720102271969));
#93238=CARTESIAN_POINT('Ctrl Pts',(-10.6685520949324,22.8008186578342,2.19804936736561));
#93239=CARTESIAN_POINT('Ctrl Pts',(-10.6812601242232,22.8016366628312,2.2046537265875));
#93240=CARTESIAN_POINT('Ctrl Pts',(-10.7309158696414,22.80488916689,2.23139261074237));
#93241=CARTESIAN_POINT('Ctrl Pts',(-10.767083292063,22.8073818547067,2.25292922879085));
#93242=CARTESIAN_POINT('Ctrl Pts',(-10.822896835068,22.8113754987719,2.28951196558835));
#93243=CARTESIAN_POINT('Ctrl Pts',(-10.8431781172665,22.8128595271252,2.30355061979335));
#93244=CARTESIAN_POINT('Ctrl Pts',(-10.9572840015759,22.8213679653181,2.38687726366919));
#93245=CARTESIAN_POINT('Ctrl Pts',(-11.0429303386377,22.8283385923076,2.4666848248111));
#93246=CARTESIAN_POINT('Ctrl Pts',(-11.1288827374588,22.8357853937335,2.56847960483394));
#93247=CARTESIAN_POINT('Ctrl Pts',(-11.1393511040777,22.836702425393,2.58131312470328));
#93248=CARTESIAN_POINT('Ctrl Pts',(-11.1536151227035,22.8379666762122,2.59941879867794));
#93249=CARTESIAN_POINT('Ctrl Pts',(-11.1575966367605,22.8383212274291,2.60454236282957));
#93250=CARTESIAN_POINT('Ctrl Pts',(-11.1644143085091,22.8389312797684,2.61343706924072));
#93251=CARTESIAN_POINT('Ctrl Pts',(-11.1672665234708,22.8391874078525,2.61719573179112));
#93252=CARTESIAN_POINT('Ctrl Pts',(-11.1731409083994,22.8397168490923,2.62501526753549));
#93253=CARTESIAN_POINT('Ctrl Pts',(-11.1761602901202,22.8399900518644,2.62907816318595));
#93254=CARTESIAN_POINT('Ctrl Pts',(-11.1831953719825,22.8406291894151,2.63864791676857));
#93255=CARTESIAN_POINT('Ctrl Pts',(-11.1871938235436,22.8409944575832,2.64416734869062));
#93256=CARTESIAN_POINT('Ctrl Pts',(-11.2001315268154,22.842183140367,2.66229160630215));
#93257=CARTESIAN_POINT('Ctrl Pts',(-11.2089098875799,22.843000451886,2.67501033811641));
#93258=CARTESIAN_POINT('Ctrl Pts',(-11.2538775766745,22.8472488226323,2.74242225251815));
#93259=CARTESIAN_POINT('Ctrl Pts',(-11.2865635122918,22.8505489835348,2.79936556394677));
#93260=CARTESIAN_POINT('Ctrl Pts',(-11.3338967311457,22.8558691003758,2.89638884000875));
#93261=CARTESIAN_POINT('Ctrl Pts',(-11.3508097537221,22.8579272232439,2.93525224182512));
#93262=CARTESIAN_POINT('Ctrl Pts',(-11.3822882437941,22.8621917575018,3.01712509042033));
#93263=CARTESIAN_POINT('Ctrl Pts',(-11.3965864969178,22.8643960686362,3.06018766095683));
#93264=CARTESIAN_POINT('Ctrl Pts',(-11.413960769318,22.8675830727605,3.12197619298645));
#93265=CARTESIAN_POINT('Ctrl Pts',(-11.4187089063772,22.8685263357334,3.14020553463525));
#93266=CARTESIAN_POINT('Ctrl Pts',(-11.4307820501429,22.8711499322043,3.19051999796195));
#93267=CARTESIAN_POINT('Ctrl Pts',(-11.4373783487565,22.8728536122414,3.2227666769586));
#93268=CARTESIAN_POINT('Ctrl Pts',(-11.4438471757254,22.8749222356935,3.26089565077517));
#93269=CARTESIAN_POINT('Ctrl Pts',(-11.4447788210633,22.875232644233,3.26659110412079));
#93270=CARTESIAN_POINT('Ctrl Pts',(-11.4462339212287,22.8757386322208,3.27582926369374));
#93271=CARTESIAN_POINT('Ctrl Pts',(-11.4467781107998,22.8759330853976,3.27936869786372));
#93272=CARTESIAN_POINT('Ctrl Pts',(-11.4477234132299,22.8762804332114,3.28567090130255));
#93273=CARTESIAN_POINT('Ctrl Pts',(-11.4481296171573,22.8764330406532,3.28843285808626));
#93274=CARTESIAN_POINT('Ctrl Pts',(-11.4489032929726,22.8767303498689,3.2938000495479));
#93275=CARTESIAN_POINT('Ctrl Pts',(-11.4492716379632,22.8768749935162,3.2964050808023));
#93276=CARTESIAN_POINT('Ctrl Pts',(-11.4500718859662,22.8771962038907,3.30217687069662));
#93277=CARTESIAN_POINT('Ctrl Pts',(-11.4505004425063,22.8773729526437,3.30534407059447));
#93278=CARTESIAN_POINT('Ctrl Pts',(-11.4515403440335,22.8778138430751,3.31322350615535));
#93279=CARTESIAN_POINT('Ctrl Pts',(-11.4521391158866,22.8780786431754,3.31793732979647));
#93280=CARTESIAN_POINT('Ctrl Pts',(-11.4546836389871,22.8792538586846,3.33878056841656));
#93281=CARTESIAN_POINT('Ctrl Pts',(-11.4563836145155,22.8801763564431,3.35493822620845));
#93282=CARTESIAN_POINT('Ctrl Pts',(-11.4615725124831,22.8835608832481,3.41363202851132));
#93283=CARTESIAN_POINT('Ctrl Pts',(-11.4634692177633,22.8860835649692,3.45628519631487));
#93284=CARTESIAN_POINT('Ctrl Pts',(-11.4634996283537,22.8886343115925,3.49895701930366));
#93285=CARTESIAN_POINT('Ctrl Pts',(-11.4634996286686,22.8886343380185,3.49895746138947));
#93286=CARTESIAN_POINT('Ctrl Pts',(-11.4634998762247,22.8886551110645,3.49930497676595));
#93287=CARTESIAN_POINT('Ctrl Pts',(-11.4635,22.8886758857888,3.49965248964563));
#93288=CARTESIAN_POINT('Ctrl Pts',(-11.4635,22.8886966621701,3.49999999996283));
#93289=CARTESIAN_POINT('Origin',(-10.,13.2,3.5));
#93290=CARTESIAN_POINT('',(-11.4635,23.4593691294935,3.50000000000014));
#93291=CARTESIAN_POINT('',(-11.4635,23.3906983315425,3.49999999997929));
#93292=CARTESIAN_POINT('',(-11.4635,13.2,3.5));
#93293=CARTESIAN_POINT('Ctrl Pts',(-11.4635,23.4593691294935,3.50000000000014));
#93294=CARTESIAN_POINT('Ctrl Pts',(-11.4635,23.4593632578606,3.49988815824253));
#93295=CARTESIAN_POINT('Ctrl Pts',(-11.4634999872435,23.4593573865652,3.49977631641766));
#93296=CARTESIAN_POINT('Ctrl Pts',(-11.4634862607233,23.4562145842122,3.43990509731606));
#93297=CARTESIAN_POINT('Ctrl Pts',(-11.4598124220148,23.4531917336194,3.38019956334097));
#93298=CARTESIAN_POINT('Ctrl Pts',(-11.4448085976956,23.4471221355299,3.25853176031568));
#93299=CARTESIAN_POINT('Ctrl Pts',(-11.4331130811415,23.4440884055884,3.19674123955496));
#93300=CARTESIAN_POINT('Ctrl Pts',(-11.3969745636183,23.4370116351706,3.05605230727827));
#93301=CARTESIAN_POINT('Ctrl Pts',(-11.3697592702726,23.4329623945494,2.97809621824932));
#93302=CARTESIAN_POINT('Ctrl Pts',(-11.3332284796358,23.4281841636351,2.89635710278226));
#93303=CARTESIAN_POINT('Ctrl Pts',(-11.3302765428507,23.4278016676637,2.88987932200807));
#93304=CARTESIAN_POINT('Ctrl Pts',(-11.3257961099855,23.4272260655346,2.88023448876226));
#93305=CARTESIAN_POINT('Ctrl Pts',(-11.324303222454,23.4270350694218,2.8770508940192));
#93306=CARTESIAN_POINT('Ctrl Pts',(-11.3216070504611,23.4266914894448,2.87135477826376));
#93307=CARTESIAN_POINT('Ctrl Pts',(-11.3204080520168,23.4265391685386,2.86884028436942));
#93308=CARTESIAN_POINT('Ctrl Pts',(-11.3177830551722,23.4262066950051,2.8633754583176));
#93309=CARTESIAN_POINT('Ctrl Pts',(-11.3163543439752,23.4260263803924,2.86042652632021));
#93310=CARTESIAN_POINT('Ctrl Pts',(-11.3122950715138,23.4255159183703,2.85211920258404));
#93311=CARTESIAN_POINT('Ctrl Pts',(-11.3096416444315,23.4251844054637,2.84677213543443));
#93312=CARTESIAN_POINT('Ctrl Pts',(-11.292997408534,23.4231188401392,2.81374047722888));
#93313=CARTESIAN_POINT('Ctrl Pts',(-11.2781629935707,23.4213379441754,2.78649210635572));
#93314=CARTESIAN_POINT('Ctrl Pts',(-11.182015491558,23.410234127612,2.62251800540867));
#93315=CARTESIAN_POINT('Ctrl Pts',(-11.079718451366,23.4003521842531,2.49931923367241));
#93316=CARTESIAN_POINT('Ctrl Pts',(-10.9391425458784,23.3897884236964,2.37724651157466));
#93317=CARTESIAN_POINT('Ctrl Pts',(-10.9182273781797,23.3882755129909,2.36007774999035));
#93318=CARTESIAN_POINT('Ctrl Pts',(-10.8899155711151,23.3863026481125,2.33812243797221));
#93319=CARTESIAN_POINT('Ctrl Pts',(-10.8829356113594,23.3858220765509,2.33280939699018));
#93320=CARTESIAN_POINT('Ctrl Pts',(-10.8715335385063,23.3850463071887,2.32429112439137));
#93321=CARTESIAN_POINT('Ctrl Pts',(-10.8671405821222,23.3847496187462,2.32104737970939));
#93322=CARTESIAN_POINT('Ctrl Pts',(-10.858672683635,23.3841818831132,2.31486764634948));
#93323=CARTESIAN_POINT('Ctrl Pts',(-10.854600588547,23.3839106938222,2.31192790277092));
#93324=CARTESIAN_POINT('Ctrl Pts',(-10.8451695547439,23.3832867745188,2.30519298897646));
#93325=CARTESIAN_POINT('Ctrl Pts',(-10.8398000221075,23.3829346179594,2.30141279222511));
#93326=CARTESIAN_POINT('Ctrl Pts',(-10.8228252374415,23.3818308130526,2.28963247055054));
#93327=CARTESIAN_POINT('Ctrl Pts',(-10.811129558823,23.3810841027067,2.28176365806137));
#93328=CARTESIAN_POINT('Ctrl Pts',(-10.7531947883521,23.3774497194202,2.24398961914468));
#93329=CARTESIAN_POINT('Ctrl Pts',(-10.7054048273343,23.3746526114417,2.21654009464506));
#93330=CARTESIAN_POINT('Ctrl Pts',(-10.5624940011442,23.3667031977485,2.14485512230858));
#93331=CARTESIAN_POINT('Ctrl Pts',(-10.4640395967639,23.3617458600027,2.10806511993116));
#93332=CARTESIAN_POINT('Ctrl Pts',(-10.3524648877767,23.3560027984606,2.07953946264981));
#93333=CARTESIAN_POINT('Ctrl Pts',(-10.342398292027,23.3554833392569,2.07707939833107));
#93334=CARTESIAN_POINT('Ctrl Pts',(-10.2966815823984,23.3531150951225,2.06642041754621));
#93335=CARTESIAN_POINT('Ctrl Pts',(-10.2607604035848,23.3512292676502,2.05945358476841));
#93336=CARTESIAN_POINT('Ctrl Pts',(-10.2187432672426,23.3489562776205,2.05292744128819));
#93337=CARTESIAN_POINT('Ctrl Pts',(-10.2128621248004,23.3486366073718,2.05205064986091));
#93338=CARTESIAN_POINT('Ctrl Pts',(-10.2034179087093,23.3481205989619,2.05070143789938));
#93339=CARTESIAN_POINT('Ctrl Pts',(-10.1998580928725,23.3479254927213,2.05020625265458));
#93340=CARTESIAN_POINT('Ctrl Pts',(-10.1935233503482,23.3475771631589,2.04934883784084));
#93341=CARTESIAN_POINT('Ctrl Pts',(-10.1907491682092,23.347424230102,2.04898144873012));
#93342=CARTESIAN_POINT('Ctrl Pts',(-10.1848174475355,23.347096381962,2.0482132073175));
#93343=CARTESIAN_POINT('Ctrl Pts',(-10.1816596997272,23.3469213439259,2.0478147041727));
#93344=CARTESIAN_POINT('Ctrl Pts',(-10.1730032350141,23.3464401601862,2.04675094726629));
#93345=CARTESIAN_POINT('Ctrl Pts',(-10.1675020604446,23.3461328828674,2.04610661108514));
#93346=CARTESIAN_POINT('Ctrl Pts',(-10.1381497675732,23.344485928735,2.042837463267));
#93347=CARTESIAN_POINT('Ctrl Pts',(-10.1142417447085,23.343118344492,2.04076845456114));
#93348=CARTESIAN_POINT('Ctrl Pts',(-10.0404221280921,23.3388373269634,2.03620523060962));
#93349=CARTESIAN_POINT('Ctrl Pts',(-9.99042675817685,23.3358568814999,2.03567871350067));
#93350=CARTESIAN_POINT('Ctrl Pts',(-9.81456210462102,23.325281853267,2.04283387757246));
#93351=CARTESIAN_POINT('Ctrl Pts',(-9.68978186000774,23.3176728032944,2.06420897701625));
#93352=CARTESIAN_POINT('Ctrl Pts',(-9.55029787953807,23.3094738924047,2.10716312457877));
#93353=CARTESIAN_POINT('Ctrl Pts',(-9.53144045429824,23.3083705902725,2.1133931468163));
#93354=CARTESIAN_POINT('Ctrl Pts',(-9.50539886178193,23.3068535474493,2.12258860052247));
#93355=CARTESIAN_POINT('Ctrl Pts',(-9.49810330949461,23.3064292703481,2.12523014120577));
#93356=CARTESIAN_POINT('Ctrl Pts',(-9.48640626101758,23.3057501092564,2.12957087898147));
#93357=CARTESIAN_POINT('Ctrl Pts',(-9.48199143939019,23.3054940237328,2.13123353477724));
#93358=CARTESIAN_POINT('Ctrl Pts',(-9.47285838992828,23.3049647464603,2.1347236276359));
#93359=CARTESIAN_POINT('Ctrl Pts',(-9.46814143973695,23.3046916646018,2.13655424648889));
#93360=CARTESIAN_POINT('Ctrl Pts',(-9.45709838241703,23.304052942589,2.14090601587066));
#93361=CARTESIAN_POINT('Ctrl Pts',(-9.45078016070777,23.303687967372,2.14344694378261));
#93362=CARTESIAN_POINT('Ctrl Pts',(-9.4302054019061,23.302500816227,2.15188857070964));
#93363=CARTESIAN_POINT('Ctrl Pts',(-9.41602414599485,23.3016847228339,2.15797073966035));
#93364=CARTESIAN_POINT('Ctrl Pts',(-9.34224590152656,23.2974465479455,2.1910043028034));
#93365=CARTESIAN_POINT('Ctrl Pts',(-9.28440630869461,23.2941546344506,2.22170538834727));
#93366=CARTESIAN_POINT('Ctrl Pts',(-9.15689389870421,23.286759799131,2.30076506349985));
#93367=CARTESIAN_POINT('Ctrl Pts',(-9.08898316446741,23.2827197268619,2.35150534435276));
#93368=CARTESIAN_POINT('Ctrl Pts',(-9.02143385367742,23.2782386133338,2.41175582593712));
#93369=CARTESIAN_POINT('Ctrl Pts',(-9.0170530810563,23.277945689634,2.41571109074918));
#93370=CARTESIAN_POINT('Ctrl Pts',(-9.00331008218715,23.2770190158152,2.42827095472169));
#93371=CARTESIAN_POINT('Ctrl Pts',(-8.99403614000006,23.2763822387354,2.43697100709232));
#93372=CARTESIAN_POINT('Ctrl Pts',(-8.95881370713339,23.2739140938223,2.47088751948754));
#93373=CARTESIAN_POINT('Ctrl Pts',(-8.93369213583686,23.2720479596064,2.49694041704338));
#93374=CARTESIAN_POINT('Ctrl Pts',(-8.90560883913313,23.2697970169586,2.52831311806146));
#93375=CARTESIAN_POINT('Ctrl Pts',(-8.90168098651855,23.2694782272225,2.53275507147281));
#93376=CARTESIAN_POINT('Ctrl Pts',(-8.89541909311083,23.268963369262,2.53992388184037));
#93377=CARTESIAN_POINT('Ctrl Pts',(-8.89306786164096,23.2687685242123,2.54263571560635));
#93378=CARTESIAN_POINT('Ctrl Pts',(-8.88890158620925,23.2684204862605,2.54747682807188));
#93379=CARTESIAN_POINT('Ctrl Pts',(-8.88708264600147,23.2682675818162,2.54960269294711));
#93380=CARTESIAN_POINT('Ctrl Pts',(-8.88320551986509,23.267939592452,2.55416043174865));
#93381=CARTESIAN_POINT('Ctrl Pts',(-8.8811492075398,23.2677643832859,2.55659377596874));
#93382=CARTESIAN_POINT('Ctrl Pts',(-8.87553076939329,23.2672822579619,2.56328657994895));
#93383=CARTESIAN_POINT('Ctrl Pts',(-8.87198495194373,23.26697420297,2.56755958302119));
#93384=CARTESIAN_POINT('Ctrl Pts',(-8.8531230885981,23.2653155977007,2.59055472882892));
#93385=CARTESIAN_POINT('Ctrl Pts',(-8.8382494979434,23.2639366810581,2.60963323191021));
#93386=CARTESIAN_POINT('Ctrl Pts',(-8.79373001966236,23.259605297363,2.66975438663009));
#93387=CARTESIAN_POINT('Ctrl Pts',(-8.76573659039813,23.2565841590063,2.71197191164284));
#93388=CARTESIAN_POINT('Ctrl Pts',(-8.67284352356797,23.245609574786,2.86919756308391));
#93389=CARTESIAN_POINT('Ctrl Pts',(-8.6213676387662,23.237654381996,2.99143144450295));
#93390=CARTESIAN_POINT('Ctrl Pts',(-8.58298529249327,23.2294356849403,3.13375227232262));
#93391=CARTESIAN_POINT('Ctrl Pts',(-8.57922013462518,23.2285868725809,3.14864166619938));
#93392=CARTESIAN_POINT('Ctrl Pts',(-8.57428361476905,23.2274103659465,3.16954203385923));
#93393=CARTESIAN_POINT('Ctrl Pts',(-8.57291464210262,23.227076399603,3.17550491318166));
#93394=CARTESIAN_POINT('Ctrl Pts',(-8.57047572243623,23.2264668752726,3.18644222720206));
#93395=CARTESIAN_POINT('Ctrl Pts',(-8.56939425365882,23.2261909546299,3.19141397233299));
#93396=CARTESIAN_POINT('Ctrl Pts',(-8.56725580517542,23.2256336173116,3.20149778708062));
#93397=CARTESIAN_POINT('Ctrl Pts',(-8.56620020494644,23.2253522479343,3.20661007584037));
#93398=CARTESIAN_POINT('Ctrl Pts',(-8.56366398540935,23.2246603502547,3.21923370296954));
#93399=CARTESIAN_POINT('Ctrl Pts',(-8.56221490003068,23.2242508232875,3.2267512677378));
#93400=CARTESIAN_POINT('Ctrl Pts',(-8.55705625614476,23.2227377885463,3.25469117004693));
#93401=CARTESIAN_POINT('Ctrl Pts',(-8.55372219686599,23.221646088447,3.27518086611885));
#93402=CARTESIAN_POINT('Ctrl Pts',(-8.53663135843362,23.2152795472986,3.39643339167672));
#93403=CARTESIAN_POINT('Ctrl Pts',(-8.53297124394648,23.2103349814459,3.49833741550094));
#93404=CARTESIAN_POINT('Ctrl Pts',(-8.54596128297862,23.2010739510337,3.68837360792246));
#93405=CARTESIAN_POINT('Ctrl Pts',(-8.56006087037098,23.196767056641,3.77619696614342));
#93406=CARTESIAN_POINT('Ctrl Pts',(-8.58480149378482,23.191492710328,3.87305660669383));
#93407=CARTESIAN_POINT('Ctrl Pts',(-8.58770194194969,23.1908950371236,3.88389090093137));
#93408=CARTESIAN_POINT('Ctrl Pts',(-8.59190119147437,23.1900558360469,3.89888465315383));
#93409=CARTESIAN_POINT('Ctrl Pts',(-8.59309454848456,23.1898200686923,3.90307353002356));
#93410=CARTESIAN_POINT('Ctrl Pts',(-8.59503870182253,23.1894401720479,3.90978399496553));
#93411=CARTESIAN_POINT('Ctrl Pts',(-8.59577763958166,23.1892967214946,3.91230902752832));
#93412=CARTESIAN_POINT('Ctrl Pts',(-8.59733713228558,23.188995900171,3.91758516673725));
#93413=CARTESIAN_POINT('Ctrl Pts',(-8.59815897544982,23.1888384525243,3.92033585781708));
#93414=CARTESIAN_POINT('Ctrl Pts',(-8.60017580564527,23.1884547064939,3.92701443933313));
#93415=CARTESIAN_POINT('Ctrl Pts',(-8.60137923454308,23.1882279250823,3.93093974067632));
#93416=CARTESIAN_POINT('Ctrl Pts',(-8.60570210166082,23.1874211077206,3.94483106178019));
#93417=CARTESIAN_POINT('Ctrl Pts',(-8.60891159981861,23.1868361562742,3.95476846080497));
#93418=CARTESIAN_POINT('Ctrl Pts',(-8.62933717053681,23.1832009346289,4.01577096110999));
#93419=CARTESIAN_POINT('Ctrl Pts',(-8.6492552212961,23.1800233902133,4.06588318245053));
#93420=CARTESIAN_POINT('Ctrl Pts',(-8.71106002443181,23.1712264548011,4.19940072776324));
#93421=CARTESIAN_POINT('Ctrl Pts',(-8.75823340650999,23.1655523979265,4.28009329937455));
#93422=CARTESIAN_POINT('Ctrl Pts',(-8.84697252406236,23.1566519456506,4.40320662572449));
#93423=CARTESIAN_POINT('Ctrl Pts',(-8.8839969289981,23.1533049202004,4.44857421088516));
#93424=CARTESIAN_POINT('Ctrl Pts',(-8.9305013832462,23.1495058338649,4.49905327290175));
#93425=CARTESIAN_POINT('Ctrl Pts',(-8.93743777428377,23.1489487338904,4.50642747232824));
#93426=CARTESIAN_POINT('Ctrl Pts',(-8.94885794735696,23.1480467616796,4.51831877465833));
#93427=CARTESIAN_POINT('Ctrl Pts',(-8.95329558090572,23.1476999322257,4.52287956402217));
#93428=CARTESIAN_POINT('Ctrl Pts',(-8.96127043618129,23.1470830801619,4.530969498547));
#93429=CARTESIAN_POINT('Ctrl Pts',(-8.96479623111008,23.1468125682619,4.53450972514551));
#93430=CARTESIAN_POINT('Ctrl Pts',(-8.97228706870468,23.1462424501754,4.54195458011746));
#93431=CARTESIAN_POINT('Ctrl Pts',(-8.97625639784298,23.1459430390391,4.54585479603831));
#93432=CARTESIAN_POINT('Ctrl Pts',(-8.98687755017851,23.1451489209597,4.55617260953813));
#93433=CARTESIAN_POINT('Ctrl Pts',(-8.99356814729659,23.1446559485351,4.56255005087068));
#93434=CARTESIAN_POINT('Ctrl Pts',(-9.02596106013155,23.1423030911922,4.59284632058364));
#93435=CARTESIAN_POINT('Ctrl Pts',(-9.05245915722957,23.1404798058875,4.61589943327915));
#93436=CARTESIAN_POINT('Ctrl Pts',(-9.13053700935324,23.1353574659586,4.67903787322278));
#93437=CARTESIAN_POINT('Ctrl Pts',(-9.1840050877526,23.1321462581884,4.7166549800129));
#93438=CARTESIAN_POINT('Ctrl Pts',(-9.33310267538688,23.1236444654527,4.8072872519166));
#93439=CARTESIAN_POINT('Ctrl Pts',(-9.43243620930461,23.1184442891638,4.85337240871525));
#93440=CARTESIAN_POINT('Ctrl Pts',(-9.54545439915662,23.1121382749076,4.89115812745899));
#93441=CARTESIAN_POINT('Ctrl Pts',(-9.5549889202999,23.1116032436673,4.89423734234839));
#93442=CARTESIAN_POINT('Ctrl Pts',(-9.56812852638618,23.1108608072702,4.89833232752536));
#93443=CARTESIAN_POINT('Ctrl Pts',(-9.57170723254709,23.1106580797545,4.89943258953251));
#93444=CARTESIAN_POINT('Ctrl Pts',(-9.57783360307508,23.1103100863705,4.90129042234548));
#93445=CARTESIAN_POINT('Ctrl Pts',(-9.58037920051778,23.110165211746,4.90205481307217));
#93446=CARTESIAN_POINT('Ctrl Pts',(-9.58565830928646,23.109864165248,4.90362435634884));
#93447=CARTESIAN_POINT('Ctrl Pts',(-9.58839209096988,23.1097079314967,4.9044284599533));
#93448=CARTESIAN_POINT('Ctrl Pts',(-9.59496125611254,23.1093317256189,4.90633986020267));
#93449=CARTESIAN_POINT('Ctrl Pts',(-9.59879884463419,23.1091113147192,4.90743945468558));
#93450=CARTESIAN_POINT('Ctrl Pts',(-9.6120102780117,23.1083504448057,4.91116653824107));
#93451=CARTESIAN_POINT('Ctrl Pts',(-9.62140560496999,23.1078057679646,4.91371613015089));
#93452=CARTESIAN_POINT('Ctrl Pts',(-9.67623851796131,23.1046089660205,4.92801024295915));
#93453=CARTESIAN_POINT('Ctrl Pts',(-9.72219109816754,23.1018590684047,4.93765649757183));
#93454=CARTESIAN_POINT('Ctrl Pts',(-9.83231283422067,23.0952210562306,4.95529611892682));
#93455=CARTESIAN_POINT('Ctrl Pts',(-9.8967085531115,23.0913037976168,4.96127911044436));
#93456=CARTESIAN_POINT('Ctrl Pts',(-9.9867199916218,23.0859089540211,4.96366085426181));
#93457=CARTESIAN_POINT('Ctrl Pts',(-10.0121651137151,23.0843923057755,4.96367056651665));
#93458=CARTESIAN_POINT('Ctrl Pts',(-10.1065936189521,23.078807917991,4.96124384243889));
#93459=CARTESIAN_POINT('Ctrl Pts',(-10.1753837173784,23.0748325462652,4.95459219188854));
#93460=CARTESIAN_POINT('Ctrl Pts',(-10.2537500861445,23.0704305712913,4.94137161724813));
#93461=CARTESIAN_POINT('Ctrl Pts',(-10.2640259993883,23.0698557578925,4.93952475658371));
#93462=CARTESIAN_POINT('Ctrl Pts',(-10.2805576373101,23.0689347397767,4.93637059509323));
#93463=CARTESIAN_POINT('Ctrl Pts',(-10.2868259714919,23.0685863825012,4.9351320281393));
#93464=CARTESIAN_POINT('Ctrl Pts',(-10.2979972780856,23.067967043965,4.93284856144747));
#93465=CARTESIAN_POINT('Ctrl Pts',(-10.3029033436998,23.0676955680726,4.93181945196736));
#93466=CARTESIAN_POINT('Ctrl Pts',(-10.3131750518944,23.0671282358291,4.92960967381251));
#93467=CARTESIAN_POINT('Ctrl Pts',(-10.3185395362618,23.0668325443672,4.92842395581855));
#93468=CARTESIAN_POINT('Ctrl Pts',(-10.3325981443541,23.0660591492435,4.92523342956317));
#93469=CARTESIAN_POINT('Ctrl Pts',(-10.3412809074715,23.0655830201735,4.92317925832111));
#93470=CARTESIAN_POINT('Ctrl Pts',(-10.380609474594,23.0634327922,4.9134942679144));
#93471=CARTESIAN_POINT('Ctrl Pts',(-10.411023289227,23.0617879117006,4.90495183681221));
#93472=CARTESIAN_POINT('Ctrl Pts',(-10.4940180318713,23.057328341729,4.87871466943892));
#93473=CARTESIAN_POINT('Ctrl Pts',(-10.5459071062503,23.054574588893,4.85900479136008));
#93474=CARTESIAN_POINT('Ctrl Pts',(-10.6684754957301,23.0479992730299,4.80429140150898));
#93475=CARTESIAN_POINT('Ctrl Pts',(-10.73768422059,23.0442290290857,4.76643464969769));
#93476=CARTESIAN_POINT('Ctrl Pts',(-10.8155808967734,23.0395938933898,4.71526486194281));
#93477=CARTESIAN_POINT('Ctrl Pts',(-10.827535045466,23.0388706446855,4.70715641724224));
#93478=CARTESIAN_POINT('Ctrl Pts',(-10.8683403438949,23.0363535603659,4.67858739199002));
#93479=CARTESIAN_POINT('Ctrl Pts',(-10.8965666937535,23.0345276683949,4.65726011568945));
#93480=CARTESIAN_POINT('Ctrl Pts',(-10.928559106889,23.0323219576975,4.63121392287582));
#93481=CARTESIAN_POINT('Ctrl Pts',(-10.9331049844457,23.0320052058447,4.62746709041018));
#93482=CARTESIAN_POINT('Ctrl Pts',(-10.9404047329227,23.0314909290128,4.62137605932743));
#93483=CARTESIAN_POINT('Ctrl Pts',(-10.9431727981696,23.0312945919339,4.6190488820226));
#93484=CARTESIAN_POINT('Ctrl Pts',(-10.9480643389099,23.0309452277237,4.61490540735256));
#93485=CARTESIAN_POINT('Ctrl Pts',(-10.9501912697296,23.0307925013838,4.61309326153195));
#93486=CARTESIAN_POINT('Ctrl Pts',(-10.9523249508494,23.0306384595706,4.6112647921337));
#93487=CARTESIAN_POINT('Ctrl Pts',(-10.9523368681591,23.0306375991705,4.61125457919919));
#93488=CARTESIAN_POINT('Ctrl Pts',(-10.9523605487933,23.030635889436,4.61123428463221));
#93489=CARTESIAN_POINT('Ctrl Pts',(-10.952372312197,23.0306350400965,4.6112242029404));
#93490=CARTESIAN_POINT('Ctrl Pts',(-10.9523956883441,23.0306333522451,4.61120416803462));
#93491=CARTESIAN_POINT('Ctrl Pts',(-10.9524073009021,23.0306325137473,4.61119421498775));
#93492=CARTESIAN_POINT('Ctrl Pts',(-10.9524303776033,23.030630847419,4.61117443547197));
#93493=CARTESIAN_POINT('Ctrl Pts',(-10.952441841901,23.030630019578,4.6111646088786));
#93494=CARTESIAN_POINT('Ctrl Pts',(-10.9524646252504,23.0306283743365,4.61114507957735));
#93495=CARTESIAN_POINT('Ctrl Pts',(-10.9524759441808,23.0306275569454,4.61113537698118));
#93496=CARTESIAN_POINT('Ctrl Pts',(-10.9524984390757,23.0306259324406,4.61111609374318));
#93497=CARTESIAN_POINT('Ctrl Pts',(-10.9525096151478,23.0306251253199,4.61110651301652));
#93498=CARTESIAN_POINT('Ctrl Pts',(-10.9525318272815,23.0306235211443,4.61108747100626));
#93499=CARTESIAN_POINT('Ctrl Pts',(-10.9525428632257,23.0306227240985,4.61107800983062));
#93500=CARTESIAN_POINT('Ctrl Pts',(-10.9525647974261,23.0306211399068,4.61105920495296));
#93501=CARTESIAN_POINT('Ctrl Pts',(-10.9525756957366,23.0306203527576,4.61104986121145));
#93502=CARTESIAN_POINT('Ctrl Pts',(-10.9525973570583,23.0306187881881,4.6110312891753));
#93503=CARTESIAN_POINT('Ctrl Pts',(-10.9526081201667,23.0306180107613,4.61102206080415));
#93504=CARTESIAN_POINT('Ctrl Pts',(-10.9526295136086,23.0306164654561,4.61100371736456));
#93505=CARTESIAN_POINT('Ctrl Pts',(-10.9526401439421,23.0306156975781,4.61099460230281));
#93506=CARTESIAN_POINT('Ctrl Pts',(-10.9526612742903,23.0306141711946,4.610976483396));
#93507=CARTESIAN_POINT('Ctrl Pts',(-10.952671774227,23.0306134126952,4.61096747962417));
#93508=CARTESIAN_POINT('Ctrl Pts',(-10.9526926462581,23.0306119048913,4.61094958119281));
#93509=CARTESIAN_POINT('Ctrl Pts',(-10.9527030182358,23.0306111555959,4.61094068663956));
#93510=CARTESIAN_POINT('Ctrl Pts',(-10.9527236360655,23.0306096660773,4.61092300519182));
#93511=CARTESIAN_POINT('Ctrl Pts',(-10.9527338821429,23.0306089258385,4.61091421811006));
#93512=CARTESIAN_POINT('Ctrl Pts',(-10.952754250693,23.0306074542526,4.6108967494616));
#93513=CARTESIAN_POINT('Ctrl Pts',(-10.9527643731362,23.030606722908,4.6108880679259));
#93514=CARTESIAN_POINT('Ctrl Pts',(-10.9527844967566,23.0306052689432,4.61087080838141));
#93515=CARTESIAN_POINT('Ctrl Pts',(-10.9527944978278,23.0306045463309,4.61086223046907));
#93516=CARTESIAN_POINT('Ctrl Pts',(-10.9528143804219,23.0306031097078,4.61084517671488));
#93517=CARTESIAN_POINT('Ctrl Pts',(-10.952824262079,23.0306023956877,4.61083670076346));
#93518=CARTESIAN_POINT('Ctrl Pts',(-10.9552872847535,23.0304244202936,4.60872399598248));
#93519=CARTESIAN_POINT('Ctrl Pts',(-10.9577334242768,23.0302465630711,4.6066116677886));
#93520=CARTESIAN_POINT('Ctrl Pts',(-10.9644624545162,23.0297543014739,4.60076188872639));
#93521=CARTESIAN_POINT('Ctrl Pts',(-10.9687305510463,23.0294386978024,4.59700760213731));
#93522=CARTESIAN_POINT('Ctrl Pts',(-10.9783589302154,23.0287192670967,4.58843831708486));
#93523=CARTESIAN_POINT('Ctrl Pts',(-10.9837057091619,23.0283144419386,4.58360843484943));
#93524=CARTESIAN_POINT('Ctrl Pts',(-11.0004316116084,23.0270318297848,4.56827368950422));
#93525=CARTESIAN_POINT('Ctrl Pts',(-11.0116794744991,23.0261453330871,4.55762786019576));
#93526=CARTESIAN_POINT('Ctrl Pts',(-11.0567928968582,23.0224983913433,4.51355090731788));
#93527=CARTESIAN_POINT('Ctrl Pts',(-11.0891857827384,23.019665579348,4.47865747361497));
#93528=CARTESIAN_POINT('Ctrl Pts',(-11.1264843322814,23.0161883078593,4.43432995192514));
#93529=CARTESIAN_POINT('Ctrl Pts',(-11.1330649195315,23.0155659108045,4.42633865088414));
#93530=CARTESIAN_POINT('Ctrl Pts',(-11.2176150503767,23.0074571491648,4.32141407137539));
#93531=CARTESIAN_POINT('Ctrl Pts',(-11.2830167386506,22.9999901814597,4.21497307682452));
#93532=CARTESIAN_POINT('Ctrl Pts',(-11.3407058238333,22.9921532613856,4.08702074242542));
#93533=CARTESIAN_POINT('Ctrl Pts',(-11.3470093254799,22.9912727084644,4.07240838853835));
#93534=CARTESIAN_POINT('Ctrl Pts',(-11.3555040026487,22.9900504448996,4.05179872324019));
#93535=CARTESIAN_POINT('Ctrl Pts',(-11.3578960139323,22.9897020197334,4.04588583908946));
#93536=CARTESIAN_POINT('Ctrl Pts',(-11.3619793355063,22.9890996957697,4.03559922205542));
#93537=CARTESIAN_POINT('Ctrl Pts',(-11.3636884089891,22.988845206278,4.03123268057793));
#93538=CARTESIAN_POINT('Ctrl Pts',(-11.3672049856253,22.9883165102487,4.02211931159909));
#93539=CARTESIAN_POINT('Ctrl Pts',(-11.3690088246199,22.9880424284064,4.017371131079));
#93540=CARTESIAN_POINT('Ctrl Pts',(-11.3732135905657,22.9873965838185,4.00612710200566));
#93541=CARTESIAN_POINT('Ctrl Pts',(-11.375593213383,22.987025530078,3.99962338039434));
#93542=CARTESIAN_POINT('Ctrl Pts',(-11.3833476881162,22.9857974041388,3.97795427986121));
#93543=CARTESIAN_POINT('Ctrl Pts',(-11.3885187179659,22.9849470236355,3.96271688612295));
#93544=CARTESIAN_POINT('Ctrl Pts',(-11.4151157823096,22.9803905222009,3.87987914613787));
#93545=CARTESIAN_POINT('Ctrl Pts',(-11.4318592815955,22.9768388640165,3.81087190089729));
#93546=CARTESIAN_POINT('Ctrl Pts',(-11.4568229829728,22.9693929687705,3.66129315498171));
#93547=CARTESIAN_POINT('Ctrl Pts',(-11.4634999999988,22.9655328877089,3.58071335569824));
#93548=CARTESIAN_POINT('Ctrl Pts',(-11.4635,22.9615280277103,3.50000000002193));
#93549=CARTESIAN_POINT('Ctrl Pts',(-11.4635,22.8886966621701,3.49999999996283));
#93550=CARTESIAN_POINT('Ctrl Pts',(-11.4635000000021,22.8937025595212,3.58372973847256));
#93551=CARTESIAN_POINT('Ctrl Pts',(-11.4563143010388,22.898792645016,3.66731143336459));
#93552=CARTESIAN_POINT('Ctrl Pts',(-11.4314010571588,22.9074124895052,3.81111579450248));
#93553=CARTESIAN_POINT('Ctrl Pts',(-11.416884068329,22.9110010896834,3.87167606728241));
#93554=CARTESIAN_POINT('Ctrl Pts',(-11.3941261690681,22.9153060509761,3.94550022529331));
#93555=CARTESIAN_POINT('Ctrl Pts',(-11.3894765407924,22.9161366426632,3.95979690332411));
#93556=CARTESIAN_POINT('Ctrl Pts',(-11.3824241860813,22.9173292740733,3.98039676483398));
#93557=CARTESIAN_POINT('Ctrl Pts',(-11.3801969786291,22.9176970188189,3.98675865091151));
#93558=CARTESIAN_POINT('Ctrl Pts',(-11.3762244309044,22.9183377417142,3.99785948400651));
#93559=CARTESIAN_POINT('Ctrl Pts',(-11.3744983783646,22.9186113488688,4.00260517187402));
#93560=CARTESIAN_POINT('Ctrl Pts',(-11.3711050989067,22.9191401297543,4.01178658799793));
#93561=CARTESIAN_POINT('Ctrl Pts',(-11.3694408252204,22.9193953969098,4.01622333427418));
#93562=CARTESIAN_POINT('Ctrl Pts',(-11.3654188835486,22.9200027142629,4.02678899305744));
#93563=CARTESIAN_POINT('Ctrl Pts',(-11.3630414448596,22.9203541049237,4.03291030414066));
#93564=CARTESIAN_POINT('Ctrl Pts',(-11.3543464020176,22.9216125518846,4.05485897650305));
#93565=CARTESIAN_POINT('Ctrl Pts',(-11.3477935325393,22.9225117750562,4.07059204865107));
#93566=CARTESIAN_POINT('Ctrl Pts',(-11.2983203266025,22.928966640721,4.18376348041435));
#93567=CARTESIAN_POINT('Ctrl Pts',(-11.2451555538814,22.9341445989993,4.27637522888001));
#93568=CARTESIAN_POINT('Ctrl Pts',(-11.1498840933806,22.9420052592637,4.4069978113952));
#93569=CARTESIAN_POINT('Ctrl Pts',(-11.1148654046305,22.9446886973284,4.44971208895779));
#93570=CARTESIAN_POINT('Ctrl Pts',(-11.0589617407059,22.9488378641672,4.51053669669999));
#93571=CARTESIAN_POINT('Ctrl Pts',(-11.0398403248026,22.9502365251758,4.53020208144455));
#93572=CARTESIAN_POINT('Ctrl Pts',(-11.0124641018614,22.9522303927913,4.55681808551152));
#93573=CARTESIAN_POINT('Ctrl Pts',(-11.0046671313447,22.9527973437842,4.56423304133091));
#93574=CARTESIAN_POINT('Ctrl Pts',(-10.9910419749323,22.9537879835973,4.57690745605331));
#93575=CARTESIAN_POINT('Ctrl Pts',(-10.9852518351393,22.9542089340998,4.58220731881851));
#93576=CARTESIAN_POINT('Ctrl Pts',(-10.9766817943306,22.9548324280526,4.58992591357902));
#93577=CARTESIAN_POINT('Ctrl Pts',(-10.9739348474169,22.9550323416452,4.59238122322338));
#93578=CARTESIAN_POINT('Ctrl Pts',(-10.9690745550257,22.9553862333389,4.59669260414874));
#93579=CARTESIAN_POINT('Ctrl Pts',(-10.9669650640809,22.9555398906743,4.59855301463682));
#93580=CARTESIAN_POINT('Ctrl Pts',(-10.9624988818325,22.9558653591276,4.60246901622453));
#93581=CARTESIAN_POINT('Ctrl Pts',(-10.960140971205,22.956037270746,4.60452312981589));
#93582=CARTESIAN_POINT('Ctrl Pts',(-10.9537808184027,22.9565011535274,4.61002807476317));
#93583=CARTESIAN_POINT('Ctrl Pts',(-10.9497664783668,22.9567941266349,4.6134647776789));
#93584=CARTESIAN_POINT('Ctrl Pts',(-10.9317473009013,22.9581096626698,4.62872277220361));
#93585=CARTESIAN_POINT('Ctrl Pts',(-10.9175403451224,22.9591481170951,4.64030161814578));
#93586=CARTESIAN_POINT('Ctrl Pts',(-10.8081182811567,22.9671313530352,4.72611304263082));
#93587=CARTESIAN_POINT('Ctrl Pts',(-10.7042644820556,22.9745793570156,4.7885730893246));
#93588=CARTESIAN_POINT('Ctrl Pts',(-10.5256988943206,22.9861673048739,4.86786127589499));
#93589=CARTESIAN_POINT('Ctrl Pts',(-10.4552545788374,22.9904783766083,4.8928925797401));
#93590=CARTESIAN_POINT('Ctrl Pts',(-10.3723341030013,22.9952342074735,4.91538909561249));
#93591=CARTESIAN_POINT('Ctrl Pts',(-10.3614357189462,22.9958533128884,4.91821127031986));
#93592=CARTESIAN_POINT('Ctrl Pts',(-10.3446777466164,22.9967963603612,4.92234508190429));
#93593=CARTESIAN_POINT('Ctrl Pts',(-10.3388410070031,22.9971231712414,4.92374683652096));
#93594=CARTESIAN_POINT('Ctrl Pts',(-10.32862703471,22.997692238648,4.92613346140754));
#93595=CARTESIAN_POINT('Ctrl Pts',(-10.3242536186214,22.9979349973668,4.92713418048937));
#93596=CARTESIAN_POINT('Ctrl Pts',(-10.3143656882362,22.9984818413064,4.9293489240532));
#93597=CARTESIAN_POINT('Ctrl Pts',(-10.3088485925227,22.9987855491592,4.93055118075345));
#93598=CARTESIAN_POINT('Ctrl Pts',(-10.2939253890208,22.99960331623,4.93371281177883));
#93599=CARTESIAN_POINT('Ctrl Pts',(-10.2845066281513,23.0001154517433,4.93561155798408));
#93600=CARTESIAN_POINT('Ctrl Pts',(-10.2409877083828,23.0024640725947,4.94393950485668));
#93601=CARTESIAN_POINT('Ctrl Pts',(-10.2066830320024,23.0042651577015,4.94924764659064));
#93602=CARTESIAN_POINT('Ctrl Pts',(-10.04503497652,23.0125666405154,4.96840298399521));
#93603=CARTESIAN_POINT('Ctrl Pts',(-9.91643235842142,23.0185796574468,4.96671403208011));
#93604=CARTESIAN_POINT('Ctrl Pts',(-9.74332276811312,23.0272642201687,4.94157714298139));
#93605=CARTESIAN_POINT('Ctrl Pts',(-9.69730572637098,23.0296385340975,4.93262112164391));
#93606=CARTESIAN_POINT('Ctrl Pts',(-9.64235249806421,23.0326362372217,4.91916001955848));
#93607=CARTESIAN_POINT('Ctrl Pts',(-9.63292677333581,23.0331562884835,4.91675126006371));
#93608=CARTESIAN_POINT('Ctrl Pts',(-9.61966856185606,23.0338969890205,4.9132219151892));
#93609=CARTESIAN_POINT('Ctrl Pts',(-9.61581536835474,23.0341133575106,4.91217929189465));
#93610=CARTESIAN_POINT('Ctrl Pts',(-9.60921826350841,23.034485768747,4.91036520396044));
#93611=CARTESIAN_POINT('Ctrl Pts',(-9.60647221986265,23.0346413701986,4.90960145441706));
#93612=CARTESIAN_POINT('Ctrl Pts',(-9.60116848789708,23.0349430600413,4.90810963589697));
#93613=CARTESIAN_POINT('Ctrl Pts',(-9.59861053932601,23.0350890828149,4.9073826140669));
#93614=CARTESIAN_POINT('Ctrl Pts',(-9.59245311847913,23.0354418142173,4.90561439581743));
#93615=CARTESIAN_POINT('Ctrl Pts',(-9.58885565505423,23.0356489111278,4.90456634494435));
#93616=CARTESIAN_POINT('Ctrl Pts',(-9.57563869390418,23.0364134089598,4.90066071293694));
#93617=CARTESIAN_POINT('Ctrl Pts',(-9.56604486210916,23.0369754242256,4.89771809669462));
#93618=CARTESIAN_POINT('Ctrl Pts',(-9.45263613124677,23.0436969931857,4.86165327913227));
#93619=CARTESIAN_POINT('Ctrl Pts',(-9.35280981319758,23.0503644264584,4.81713677057715));
#93620=CARTESIAN_POINT('Ctrl Pts',(-9.17835442233576,23.0624946045419,4.71467955693113));
#93621=CARTESIAN_POINT('Ctrl Pts',(-9.10255141115444,23.0679677192448,4.65980123022178));
#93622=CARTESIAN_POINT('Ctrl Pts',(-9.02233695720921,23.0739101339972,4.58912357607396));
#93623=CARTESIAN_POINT('Ctrl Pts',(-9.01231297860954,23.0746561527892,4.58004145950308));
#93624=CARTESIAN_POINT('Ctrl Pts',(-8.99768966560636,23.0757498810816,4.56641829068668));
#93625=CARTESIAN_POINT('Ctrl Pts',(-8.99299238323127,23.0761020547853,4.56198382228049));
#93626=CARTESIAN_POINT('Ctrl Pts',(-8.98470480512746,23.0767249750428,4.55405550668758));
#93627=CARTESIAN_POINT('Ctrl Pts',(-8.9811028212063,23.0769962459546,4.55057407345802));
#93628=CARTESIAN_POINT('Ctrl Pts',(-8.97357251969335,23.0775645278476,4.54322063832996));
#93629=CARTESIAN_POINT('Ctrl Pts',(-8.96964806754071,23.0778613652198,4.53934477868884));
#93630=CARTESIAN_POINT('Ctrl Pts',(-8.95936711718237,23.0786408478511,4.5290756673897));
#93631=CARTESIAN_POINT('Ctrl Pts',(-8.9530475644933,23.0791218730946,4.52264565158095));
#93632=CARTESIAN_POINT('Ctrl Pts',(-8.92658804141508,23.0811444863814,4.49522126822913));
#93633=CARTESIAN_POINT('Ctrl Pts',(-8.90701631609068,23.0826617805098,4.4736865113541));
#93634=CARTESIAN_POINT('Ctrl Pts',(-8.78620872849108,23.0922042776851,4.3325256048145));
#93635=CARTESIAN_POINT('Ctrl Pts',(-8.70411667639938,23.0993937177774,4.19790032297425));
#93636=CARTESIAN_POINT('Ctrl Pts',(-8.63326035128343,23.1089395912479,4.02422319550739));
#93637=CARTESIAN_POINT('Ctrl Pts',(-8.6224968793901,23.1105447258081,3.99524954553582));
#93638=CARTESIAN_POINT('Ctrl Pts',(-8.61076019305092,23.1125193610057,3.96030488296422));
#93639=CARTESIAN_POINT('Ctrl Pts',(-8.60889575873792,23.1128407114197,3.95463921298278));
#93640=CARTESIAN_POINT('Ctrl Pts',(-8.60606090231911,23.1133416489456,3.94584389348931));
#93641=CARTESIAN_POINT('Ctrl Pts',(-8.60506624805134,23.113519857383,3.94272204897525));
#93642=CARTESIAN_POINT('Ctrl Pts',(-8.60324498437891,23.1138507859955,3.93693871783368));
#93643=CARTESIAN_POINT('Ctrl Pts',(-8.60241548904494,23.1140033367239,3.93427819559775));
#93644=CARTESIAN_POINT('Ctrl Pts',(-8.60055563392569,23.1143495508551,3.92825238231057));
#93645=CARTESIAN_POINT('Ctrl Pts',(-8.59952981660688,23.1145434715495,3.92488575121337));
#93646=CARTESIAN_POINT('Ctrl Pts',(-8.59646225404224,23.115132367723,3.91468650715257));
#93647=CARTESIAN_POINT('Ctrl Pts',(-8.59445832679202,23.1155294336795,3.90784274445678));
#93648=CARTESIAN_POINT('Ctrl Pts',(-8.5780749033127,23.1188803246379,3.85033533551735));
#93649=CARTESIAN_POINT('Ctrl Pts',(-8.56639109989419,23.1219668345176,3.79894860190357));
#93650=CARTESIAN_POINT('Ctrl Pts',(-8.54476688026983,23.1296003436141,3.67268707318201));
#93651=CARTESIAN_POINT('Ctrl Pts',(-8.53780028193211,23.1341854447125,3.5974506706282));
#93652=CARTESIAN_POINT('Ctrl Pts',(-8.53543170949651,23.1435669509989,3.43998488473847));
#93653=CARTESIAN_POINT('Ctrl Pts',(-8.54109664249258,23.1483274520173,3.3579908879184));
#93654=CARTESIAN_POINT('Ctrl Pts',(-8.5553496851577,23.153504476523,3.26558894905294));
#93655=CARTESIAN_POINT('Ctrl Pts',(-8.55722583930858,23.1541336650272,3.25430546472472));
#93656=CARTESIAN_POINT('Ctrl Pts',(-8.56029467594815,23.155088782984,3.23709827487902));
#93657=CARTESIAN_POINT('Ctrl Pts',(-8.56139205137798,23.1554176963114,3.23115820848394));
#93658=CARTESIAN_POINT('Ctrl Pts',(-8.56345965032266,23.15601521438,3.2203416501542));
#93659=CARTESIAN_POINT('Ctrl Pts',(-8.564418003776,23.1562841890715,3.21546300442164));
#93660=CARTESIAN_POINT('Ctrl Pts',(-8.56654651970561,23.1568647908666,3.20491202504406));
#93661=CARTESIAN_POINT('Ctrl Pts',(-8.56772553304102,23.1571761331146,3.1992415491617));
#93662=CARTESIAN_POINT('Ctrl Pts',(-8.57103193634381,23.1580221573305,3.18379987053516));
#93663=CARTESIAN_POINT('Ctrl Pts',(-8.57322588391218,23.1585547249872,3.17404313608866));
#93664=CARTESIAN_POINT('Ctrl Pts',(-8.58482358974776,23.1612318870614,3.12482904463172));
#93665=CARTESIAN_POINT('Ctrl Pts',(-8.59576523049385,23.1633270905225,3.08575054272287));
#93666=CARTESIAN_POINT('Ctrl Pts',(-8.61254634397472,23.1660742408351,3.03417660266031));
#93667=CARTESIAN_POINT('Ctrl Pts',(-8.61695758629698,23.1667619419361,3.0212382859478));
#93668=CARTESIAN_POINT('Ctrl Pts',(-8.66562409351874,23.1740083561033,2.88478713744418));
#93669=CARTESIAN_POINT('Ctrl Pts',(-8.72610938857207,23.1801112962626,2.76771424503984));
#93670=CARTESIAN_POINT('Ctrl Pts',(-8.81814092906498,23.1882947743067,2.63634779226111));
#93671=CARTESIAN_POINT('Ctrl Pts',(-8.83561790402756,23.1898154654618,2.61292609910041));
#93672=CARTESIAN_POINT('Ctrl Pts',(-8.85743437493096,23.1916956019755,2.58544517265444));
#93673=CARTESIAN_POINT('Ctrl Pts',(-8.86111347779629,23.1920120800991,2.58086767709557));
#93674=CARTESIAN_POINT('Ctrl Pts',(-8.86687537430508,23.1925070332029,2.57378650510597));
#93675=CARTESIAN_POINT('Ctrl Pts',(-8.86893918489258,23.1926841816826,2.5712673756213));
#93676=CARTESIAN_POINT('Ctrl Pts',(-8.87278592585717,23.1930141633791,2.56660380409002));
#93677=CARTESIAN_POINT('Ctrl Pts',(-8.87456658697335,23.1931668352226,2.56445755845141));
#93678=CARTESIAN_POINT('Ctrl Pts',(-8.87862539302519,23.1935146517819,2.55959380290808));
#93679=CARTESIAN_POINT('Ctrl Pts',(-8.8809072773608,23.1937100640358,2.5568794868701));
#93680=CARTESIAN_POINT('Ctrl Pts',(-8.88789408781464,23.1943079147478,2.54862968924078));
#93681=CARTESIAN_POINT('Ctrl Pts',(-8.89263031313694,23.1947125359804,2.54312101063837));
#93682=CARTESIAN_POINT('Ctrl Pts',(-8.94549683050246,23.1992195995307,2.48255041388535));
#93683=CARTESIAN_POINT('Ctrl Pts',(-8.99764396342708,23.2035754572301,2.43114044228027));
#93684=CARTESIAN_POINT('Ctrl Pts',(-9.07353880045009,23.2095576035611,2.36677510817375));
#93685=CARTESIAN_POINT('Ctrl Pts',(-9.09412830144786,23.2111490737651,2.35024982149241));
#93686=CARTESIAN_POINT('Ctrl Pts',(-9.19263068806143,23.2185898359108,2.2754803390266));
#93687=CARTESIAN_POINT('Ctrl Pts',(-9.2757883655974,23.2243576161389,2.22453289374682));
#93688=CARTESIAN_POINT('Ctrl Pts',(-9.3818036026017,23.2309735749948,2.17331868716748));
#93689=CARTESIAN_POINT('Ctrl Pts',(-9.40039446825325,23.2321092748022,2.16481336237043));
#93690=CARTESIAN_POINT('Ctrl Pts',(-9.42614515125295,23.2336497577142,2.15367878683996));
#93691=CARTESIAN_POINT('Ctrl Pts',(-9.43315575341989,23.2340658949496,2.15071211388196));
#93692=CARTESIAN_POINT('Ctrl Pts',(-9.4450052236418,23.2347638656202,2.14580643304056));
#93693=CARTESIAN_POINT('Ctrl Pts',(-9.44983182920665,23.2350466719247,2.14383835646204));
#93694=CARTESIAN_POINT('Ctrl Pts',(-9.45939922417467,23.2356043393218,2.13999667831226));
#93695=CARTESIAN_POINT('Ctrl Pts',(-9.46413949001787,23.2358792341282,2.13812197735152));
#93696=CARTESIAN_POINT('Ctrl Pts',(-9.47462018360812,23.2364839675119,2.13404022004967));
#93697=CARTESIAN_POINT('Ctrl Pts',(-9.48036494081066,23.2368134259113,2.13184449760066));
#93698=CARTESIAN_POINT('Ctrl Pts',(-9.50068342966843,23.2379717275707,2.12422493887533));
#93699=CARTESIAN_POINT('Ctrl Pts',(-9.51532987442783,23.23879410264,2.11899712164681));
#93700=CARTESIAN_POINT('Ctrl Pts',(-9.65370638310688,23.2464532233741,2.07207850194481));
#93701=CARTESIAN_POINT('Ctrl Pts',(-9.78240355481591,23.2526822643321,2.04688860198743));
#93702=CARTESIAN_POINT('Ctrl Pts',(-9.96415333620947,23.2615825051734,2.03603284564221));
#93703=CARTESIAN_POINT('Ctrl Pts',(-10.0156877715751,23.2641269927053,2.03567831213103));
#93704=CARTESIAN_POINT('Ctrl Pts',(-10.0915514969956,23.2680315690132,2.03916179875368));
#93705=CARTESIAN_POINT('Ctrl Pts',(-10.1159398593617,23.2693112864002,2.04089488504383));
#93706=CARTESIAN_POINT('Ctrl Pts',(-10.145818416135,23.270921379738,2.04377189677918));
#93707=CARTESIAN_POINT('Ctrl Pts',(-10.1513617485163,23.2712218929209,2.04433763593095));
#93708=CARTESIAN_POINT('Ctrl Pts',(-10.1600740725861,23.2716972123874,2.04527709761038));
#93709=CARTESIAN_POINT('Ctrl Pts',(-10.1632453621957,23.2718708569266,2.04562955792767));
#93710=CARTESIAN_POINT('Ctrl Pts',(-10.1691954680698,23.272197877064,2.04631056502229));
#93711=CARTESIAN_POINT('Ctrl Pts',(-10.1719745083046,23.272351118643,2.04663671168225));
#93712=CARTESIAN_POINT('Ctrl Pts',(-10.1783113306848,23.27270168243,2.04739882720235));
#93713=CARTESIAN_POINT('Ctrl Pts',(-10.1818684540578,23.2728992853135,2.04783989769752));
#93714=CARTESIAN_POINT('Ctrl Pts',(-10.1912872534378,23.2734246112179,2.04904294457913));
#93715=CARTESIAN_POINT('Ctrl Pts',(-10.1971459335241,23.273753530381,2.04982736596946));
#93716=CARTESIAN_POINT('Ctrl Pts',(-10.2383244312395,23.2760797878145,2.05559491874596));
#93717=CARTESIAN_POINT('Ctrl Pts',(-10.2734539078621,23.2781387538969,2.06183202253101));
#93718=CARTESIAN_POINT('Ctrl Pts',(-10.4085024221498,23.2862558521334,2.09093605699013));
#93719=CARTESIAN_POINT('Ctrl Pts',(-10.5061423467224,23.2925346786565,2.12299002641057));
#93720=CARTESIAN_POINT('Ctrl Pts',(-10.660326143257,23.3025508771655,2.19224308173794));
#93721=CARTESIAN_POINT('Ctrl Pts',(-10.7190932462435,23.3064014513024,2.22361230993027));
#93722=CARTESIAN_POINT('Ctrl Pts',(-10.7887312887505,23.3109814397479,2.26712628202359));
#93723=CARTESIAN_POINT('Ctrl Pts',(-10.8018026320707,23.3118421992046,2.27558699130427));
#93724=CARTESIAN_POINT('Ctrl Pts',(-10.8204155682214,23.3130698289545,2.28806053118212));
#93725=CARTESIAN_POINT('Ctrl Pts',(-10.8260676241583,23.3134428811942,2.29190593776933));
#93726=CARTESIAN_POINT('Ctrl Pts',(-10.835860499199,23.3140897669519,2.29866943204233));
#93727=CARTESIAN_POINT('Ctrl Pts',(-10.8400134639367,23.3143642656683,2.30156965620346));
#93728=CARTESIAN_POINT('Ctrl Pts',(-10.8480012681559,23.3148925924222,2.30720986285703));
#93729=CARTESIAN_POINT('Ctrl Pts',(-10.8518380884348,23.3151465266012,2.30994691972722));
#93730=CARTESIAN_POINT('Ctrl Pts',(-10.8609089566859,23.3157472865384,2.31648411365783));
#93731=CARTESIAN_POINT('Ctrl Pts',(-10.8661311905898,23.3160934858749,2.32030052664382));
#93732=CARTESIAN_POINT('Ctrl Pts',(-10.8845340134632,23.3173148126791,2.33393739798975));
#93733=CARTESIAN_POINT('Ctrl Pts',(-10.8975745496082,23.3181827069297,2.34394534326842));
#93734=CARTESIAN_POINT('Ctrl Pts',(-11.0031424200493,23.3252363004946,2.42782666700192));
#93735=CARTESIAN_POINT('Ctrl Pts',(-11.0865593042528,23.3309396058576,2.51245668811158));
#93736=CARTESIAN_POINT('Ctrl Pts',(-11.1951585539255,23.3395999948395,2.65326607584663));
#93737=CARTESIAN_POINT('Ctrl Pts',(-11.2285427195277,23.3425110075756,2.70247624563452));
#93738=CARTESIAN_POINT('Ctrl Pts',(-11.2724213116506,23.346918352538,2.77647724425439));
#93739=CARTESIAN_POINT('Ctrl Pts',(-11.2853727386823,23.3483083789709,2.79974439065669));
#93740=CARTESIAN_POINT('Ctrl Pts',(-11.3003250413342,23.3500421914841,2.82841997754414));
#93741=CARTESIAN_POINT('Ctrl Pts',(-11.3029387490456,23.3503504234604,2.83350502346331));
#93742=CARTESIAN_POINT('Ctrl Pts',(-11.3069789939376,23.3508352397599,2.84148003410413));
#93743=CARTESIAN_POINT('Ctrl Pts',(-11.3084259237483,23.3510105838645,2.84435967350196));
#93744=CARTESIAN_POINT('Ctrl Pts',(-11.3111090656648,23.3513390057636,2.8497438436725));
#93745=CARTESIAN_POINT('Ctrl Pts',(-11.3123476259413,23.3514919361305,2.85224714653069));
#93746=CARTESIAN_POINT('Ctrl Pts',(-11.3151638807789,23.3518427170639,2.85798042204626));
#93747=CARTESIAN_POINT('Ctrl Pts',(-11.3167368412838,23.3520408538252,2.86121266291609));
#93748=CARTESIAN_POINT('Ctrl Pts',(-11.3208237956901,23.3525614423942,2.86969008969881));
#93749=CARTESIAN_POINT('Ctrl Pts',(-11.3233184303534,23.3528850273899,2.87494447296516));
#93750=CARTESIAN_POINT('Ctrl Pts',(-11.340110509812,23.3551026467678,2.91086431059281));
#93751=CARTESIAN_POINT('Ctrl Pts',(-11.3533710994117,23.3570521853978,2.94200057623519));
#93752=CARTESIAN_POINT('Ctrl Pts',(-11.398714046218,23.3644439404849,3.05961754847301));
#93753=CARTESIAN_POINT('Ctrl Pts',(-11.4236795437323,23.370076016115,3.14861095853915));
#93754=CARTESIAN_POINT('Ctrl Pts',(-11.4552606781815,23.3806568484099,3.32310607387804));
#93755=CARTESIAN_POINT('Ctrl Pts',(-11.4630854948338,23.3856051615986,3.40802267691719));
#93756=CARTESIAN_POINT('Ctrl Pts',(-11.463494655631,23.3904459116752,3.49543302098015));
#93757=CARTESIAN_POINT('Ctrl Pts',(-11.4635,23.3905722042834,3.49771651079369));
#93758=CARTESIAN_POINT('Ctrl Pts',(-11.4635,23.3906983315425,3.49999999997929));
#93759=CARTESIAN_POINT('Origin',(-10.,13.2,3.5));
#93760=CARTESIAN_POINT('',(-11.4635,23.9605564584951,3.50000000010085));
#93761=CARTESIAN_POINT('',(-11.4635,23.8891760003868,3.49999987117833));
#93762=CARTESIAN_POINT('',(-11.4635,13.2,3.5));
#93763=CARTESIAN_POINT('Ctrl Pts',(-11.4635,23.9605564584951,3.50000000010084));
#93764=CARTESIAN_POINT('Ctrl Pts',(-11.4635000000071,23.9543681829968,3.39710918915123));
#93765=CARTESIAN_POINT('Ctrl Pts',(-11.4526495736673,23.9482887247367,3.29448451306187));
#93766=CARTESIAN_POINT('Ctrl Pts',(-11.4289758303516,23.9419849953737,3.18382767216033));
#93767=CARTESIAN_POINT('Ctrl Pts',(-11.4267312326161,23.9414185100086,3.17384840647046));
#93768=CARTESIAN_POINT('Ctrl Pts',(-11.4223784615672,23.94037494965,3.15540185477534));
#93769=CARTESIAN_POINT('Ctrl Pts',(-11.4202988392615,23.9398969951479,3.14692836216495));
#93770=CARTESIAN_POINT('Ctrl Pts',(-11.4167970973129,23.9391243851414,3.13319222553145));
#93771=CARTESIAN_POINT('Ctrl Pts',(-11.4154211517208,23.9388282616594,3.12791812359778));
#93772=CARTESIAN_POINT('Ctrl Pts',(-11.4127198823064,23.9382609023692,3.11779580862157));
#93773=CARTESIAN_POINT('Ctrl Pts',(-11.4113989870901,23.9379895291454,3.11294650255681));
#93774=CARTESIAN_POINT('Ctrl Pts',(-11.4083180880955,23.9373701393845,3.10186133744637));
#93775=CARTESIAN_POINT('Ctrl Pts',(-11.4065415932648,23.9370226588313,3.09563014438016));
#93776=CARTESIAN_POINT('Ctrl Pts',(-11.4017091642415,23.9361024318987,3.07909724664258));
#93777=CARTESIAN_POINT('Ctrl Pts',(-11.3985810276646,23.9355320170316,3.06881694592079));
#93778=CARTESIAN_POINT('Ctrl Pts',(-11.3683197729957,23.9302390896538,2.97316211450145));
#93779=CARTESIAN_POINT('Ctrl Pts',(-11.3335141095995,23.9257856365212,2.89041003346788));
#93780=CARTESIAN_POINT('Ctrl Pts',(-11.268148401827,23.9190034737887,2.76783603669243));
#93781=CARTESIAN_POINT('Ctrl Pts',(-11.2427577025094,23.9166204217943,2.72552103708051));
#93782=CARTESIAN_POINT('Ctrl Pts',(-11.1879708728508,23.9118069157457,2.6438693574715));
#93783=CARTESIAN_POINT('Ctrl Pts',(-11.1586365462398,23.9093796434825,2.60456982203685));
#93784=CARTESIAN_POINT('Ctrl Pts',(-11.1120687876538,23.9056223175329,2.54831071531222));
#93785=CARTESIAN_POINT('Ctrl Pts',(-11.0962965693742,23.9043641129525,2.53018394403956));
#93786=CARTESIAN_POINT('Ctrl Pts',(-11.0763297883332,23.9027768838485,2.50834611468825));
#93787=CARTESIAN_POINT('Ctrl Pts',(-11.0725499173417,23.9024766451298,2.50425911286629));
#93788=CARTESIAN_POINT('Ctrl Pts',(-11.0665681319396,23.9020016897821,2.49786485888969));
#93789=CARTESIAN_POINT('Ctrl Pts',(-11.0643817961627,23.9018281321982,2.49554302595069));
#93790=CARTESIAN_POINT('Ctrl Pts',(-11.0602634672969,23.901501236911,2.49119800961621));
#93791=CARTESIAN_POINT('Ctrl Pts',(-11.0583332532581,23.9013480328503,2.48917320945137));
#93792=CARTESIAN_POINT('Ctrl Pts',(-11.0539165423878,23.9009975016114,2.48456658507592));
#93793=CARTESIAN_POINT('Ctrl Pts',(-11.0514263604299,23.9007998935227,2.48198835640601));
#93794=CARTESIAN_POINT('Ctrl Pts',(-11.0448030808621,23.9002744343683,2.47518111874148));
#93795=CARTESIAN_POINT('Ctrl Pts',(-11.0406538238061,23.8999453857695,2.47096801130838));
#93796=CARTESIAN_POINT('Ctrl Pts',(-11.0112631148531,23.8976163207678,2.44148458460281));
#93797=CARTESIAN_POINT('Ctrl Pts',(-10.9851313347235,23.8955545144942,2.41712243448815));
#93798=CARTESIAN_POINT('Ctrl Pts',(-10.9516079953416,23.8929486140665,2.38808764837277));
#93799=CARTESIAN_POINT('Ctrl Pts',(-10.945029156253,23.8924389852871,2.3824908302785));
#93800=CARTESIAN_POINT('Ctrl Pts',(-10.9300655200673,23.8912844629442,2.36998744393083));
#93801=CARTESIAN_POINT('Ctrl Pts',(-10.9216526079498,23.8906385863462,2.36311534771559));
#93802=CARTESIAN_POINT('Ctrl Pts',(-10.8505180829529,23.8852088966488,2.30631755868577));
#93803=CARTESIAN_POINT('Ctrl Pts',(-10.783864896324,23.8803336605694,2.26152701696299));
#93804=CARTESIAN_POINT('Ctrl Pts',(-10.6695503925618,23.8725606869711,2.19765091602785));
#93805=CARTESIAN_POINT('Ctrl Pts',(-10.6239593197965,23.869595982601,2.17520326217796));
#93806=CARTESIAN_POINT('Ctrl Pts',(-10.5591810452508,23.8655852121357,2.14739615300045));
#93807=CARTESIAN_POINT('Ctrl Pts',(-10.540916454845,23.864475482809,2.13998895244032));
#93808=CARTESIAN_POINT('Ctrl Pts',(-10.5089105420873,23.8625670785485,2.12775578471672));
#93809=CARTESIAN_POINT('Ctrl Pts',(-10.4952367888932,23.8617630256511,2.12276194117572));
#93810=CARTESIAN_POINT('Ctrl Pts',(-10.4751219633236,23.8605962847328,2.11575404988019));
#93811=CARTESIAN_POINT('Ctrl Pts',(-10.4687381433734,23.8602283391433,2.11357932591354));
#93812=CARTESIAN_POINT('Ctrl Pts',(-10.4575490668385,23.859587458352,2.10985375112556));
#93813=CARTESIAN_POINT('Ctrl Pts',(-10.4527504275493,23.8593138923398,2.10828350837317));
#93814=CARTESIAN_POINT('Ctrl Pts',(-10.4434357432137,23.8587853290166,2.10528877036745));
#93815=CARTESIAN_POINT('Ctrl Pts',(-10.4389207268927,23.8585302375357,2.103861300353));
#93816=CARTESIAN_POINT('Ctrl Pts',(-10.4281364282006,23.8579235567038,2.10050921564819));
#93817=CARTESIAN_POINT('Ctrl Pts',(-10.4218609509691,23.8575726242696,2.09860476788857));
#93818=CARTESIAN_POINT('Ctrl Pts',(-10.3992776116565,23.8563170970655,2.09191674222341));
#93819=CARTESIAN_POINT('Ctrl Pts',(-10.3828991694546,23.8554202888611,2.08737502158141));
#93820=CARTESIAN_POINT('Ctrl Pts',(-10.2620452711281,23.8488960549862,2.05611882857454));
#93821=CARTESIAN_POINT('Ctrl Pts',(-10.154981120853,23.8436574592109,2.04073850806824));
#93822=CARTESIAN_POINT('Ctrl Pts',(-9.98016220777543,23.8351526879851,2.03509859552735));
#93823=CARTESIAN_POINT('Ctrl Pts',(-9.91306939801964,23.831890922504,2.03754606693212));
#93824=CARTESIAN_POINT('Ctrl Pts',(-9.81802562915411,23.8270095240859,2.04757758899404));
#93825=CARTESIAN_POINT('Ctrl Pts',(-9.78976044708354,23.8255240700692,2.05139907207021));
#93826=CARTESIAN_POINT('Ctrl Pts',(-9.75587362331828,23.823683452169,2.05699322101328));
#93827=CARTESIAN_POINT('Ctrl Pts',(-9.75012619362705,23.8233691866638,2.05797734740935));
#93828=CARTESIAN_POINT('Ctrl Pts',(-9.74118797866969,23.8228769914377,2.05956286860933));
#93829=CARTESIAN_POINT('Ctrl Pts',(-9.73799298892843,23.8227003651004,2.06014059102847));
#93830=CARTESIAN_POINT('Ctrl Pts',(-9.73205741570793,23.8223709064475,2.061234279476));
#93831=CARTESIAN_POINT('Ctrl Pts',(-9.72931637027296,23.8222182318842,2.06174744942576));
#93832=CARTESIAN_POINT('Ctrl Pts',(-9.723082825866,23.8218698261695,2.06293292497623));
#93833=CARTESIAN_POINT('Ctrl Pts',(-9.71959131403065,23.821673823124,2.06361012683548));
#93834=CARTESIAN_POINT('Ctrl Pts',(-9.71051812246244,23.8211623185226,2.06540427456578));
#93835=CARTESIAN_POINT('Ctrl Pts',(-9.70494048355168,23.8208457450908,2.06654106007386));
#93836=CARTESIAN_POINT('Ctrl Pts',(-9.66864891163044,23.8187726569218,2.07415847573261));
#93837=CARTESIAN_POINT('Ctrl Pts',(-9.63814565524022,23.8169683362648,2.08159288504689));
#93838=CARTESIAN_POINT('Ctrl Pts',(-9.50726099412317,23.8090242467858,2.11798931742116));
#93839=CARTESIAN_POINT('Ctrl Pts',(-9.40990128364166,23.8026185679344,2.15667220869621));
#93840=CARTESIAN_POINT('Ctrl Pts',(-9.27257190836735,23.7934035067501,2.22907167012974));
#93841=CARTESIAN_POINT('Ctrl Pts',(-9.22891546086121,23.790439049915,2.25507436120165));
#93842=CARTESIAN_POINT('Ctrl Pts',(-9.16195781472005,23.7858567824691,2.2998321136181));
#93843=CARTESIAN_POINT('Ctrl Pts',(-9.13772875301896,23.784190281127,2.31711955879814));
#93844=CARTESIAN_POINT('Ctrl Pts',(-9.10708496483639,23.7820703967399,2.34042620113659));
#93845=CARTESIAN_POINT('Ctrl Pts',(-9.10017505672099,23.7815915333914,2.34578003346862));
#93846=CARTESIAN_POINT('Ctrl Pts',(-9.08903231448923,23.7808178380375,2.35457437152227));
#93847=CARTESIAN_POINT('Ctrl Pts',(-9.08477008812104,23.7805215300343,2.35797714386127));
#93848=CARTESIAN_POINT('Ctrl Pts',(-9.07661806556957,23.7799540711631,2.36456030689361));
#93849=CARTESIAN_POINT('Ctrl Pts',(-9.07272543721932,23.7796827812032,2.36773705368233));
#93850=CARTESIAN_POINT('Ctrl Pts',(-9.06385714376911,23.7790639320408,2.37505081307066));
#93851=CARTESIAN_POINT('Ctrl Pts',(-9.05889238209177,23.7787169058427,2.37920092175541));
#93852=CARTESIAN_POINT('Ctrl Pts',(-9.04577864055623,23.777798635608,2.3903114421323));
#93853=CARTESIAN_POINT('Ctrl Pts',(-9.03767822866114,23.7772297075361,2.3973287367525));
#93854=CARTESIAN_POINT('Ctrl Pts',(-8.95727051033018,23.7715627107345,2.46854601124162));
#93855=CARTESIAN_POINT('Ctrl Pts',(-8.89141478136627,23.7667828479379,2.53967508974194));
#93856=CARTESIAN_POINT('Ctrl Pts',(-8.78368632444051,23.7580870661973,2.68201208555751));
#93857=CARTESIAN_POINT('Ctrl Pts',(-8.73988020463631,23.7541597935185,2.75125469238017));
#93858=CARTESIAN_POINT('Ctrl Pts',(-8.68698178934722,23.7483486950862,2.85278702992535));
#93859=CARTESIAN_POINT('Ctrl Pts',(-8.67285054304131,23.7466538156276,2.88228205625691));
#93860=CARTESIAN_POINT('Ctrl Pts',(-8.65728845269251,23.7445788374401,2.91776757037786));
#93861=CARTESIAN_POINT('Ctrl Pts',(-8.65489147412222,23.7442527417254,2.92332682356009));
#93862=CARTESIAN_POINT('Ctrl Pts',(-8.65124327387973,23.7437460183106,2.93193450980706));
#93863=CARTESIAN_POINT('Ctrl Pts',(-8.64996771138036,23.743566821238,2.93497263194652));
#93864=CARTESIAN_POINT('Ctrl Pts',(-8.64763322828445,23.743235049758,2.94058591585531));
#93865=CARTESIAN_POINT('Ctrl Pts',(-8.64657139030461,23.7430826526084,2.94315980669144));
#93866=CARTESIAN_POINT('Ctrl Pts',(-8.64419399589271,23.7427380624659,2.94896957375032));
#93867=CARTESIAN_POINT('Ctrl Pts',(-8.64288268335588,23.7425456220755,2.95220711964457));
#93868=CARTESIAN_POINT('Ctrl Pts',(-8.63954278058361,23.742049385323,2.96053872347024));
#93869=CARTESIAN_POINT('Ctrl Pts',(-8.63753122394465,23.7417446175078,2.96563949708205));
#93870=CARTESIAN_POINT('Ctrl Pts',(-8.62553318937835,23.7398911728908,2.99657153249675));
#93871=CARTESIAN_POINT('Ctrl Pts',(-8.61625353682907,23.7383052810604,3.02266913131957));
#93872=CARTESIAN_POINT('Ctrl Pts',(-8.57491228529225,23.7304959575204,3.15029699046659));
#93873=CARTESIAN_POINT('Ctrl Pts',(-8.55325438382536,23.7239630109981,3.25485756940824));
#93874=CARTESIAN_POINT('Ctrl Pts',(-8.53641451493989,23.7134375559269,3.43115858339805));
#93875=CARTESIAN_POINT('Ctrl Pts',(-8.53479684064148,23.7093370306252,3.5018745978602));
#93876=CARTESIAN_POINT('Ctrl Pts',(-8.53908865047082,23.7044970537929,3.58847664664175));
#93877=CARTESIAN_POINT('Ctrl Pts',(-8.54014735344128,23.7036088374729,3.60450056170623));
#93878=CARTESIAN_POINT('Ctrl Pts',(-8.54203935478994,23.702349553272,3.62740050915816));
#93879=CARTESIAN_POINT('Ctrl Pts',(-8.54265803393002,23.7019718531621,3.63429269879728));
#93880=CARTESIAN_POINT('Ctrl Pts',(-8.54381547011056,23.7013196090063,3.64623492708816));
#93881=CARTESIAN_POINT('Ctrl Pts',(-8.54433166994195,23.7010443673951,3.65128698807051));
#93882=CARTESIAN_POINT('Ctrl Pts',(-8.54537520285233,23.7005164866035,3.66099984207542));
#93883=CARTESIAN_POINT('Ctrl Pts',(-8.54589866589839,23.7002637303348,3.66566098060342));
#93884=CARTESIAN_POINT('Ctrl Pts',(-8.54718742724437,23.699668626216,3.6766596357364));
#93885=CARTESIAN_POINT('Ctrl Pts',(-8.5479718029144,23.6993268770486,3.68299484986503));
#93886=CARTESIAN_POINT('Ctrl Pts',(-8.55086006751484,23.6981360610574,3.70513382226229));
#93887=CARTESIAN_POINT('Ctrl Pts',(-8.55318076382091,23.6972937561501,3.7209084720094));
#93888=CARTESIAN_POINT('Ctrl Pts',(-8.57582664036929,23.6899612385402,3.85911742053291));
#93889=CARTESIAN_POINT('Ctrl Pts',(-8.61138990099582,23.6840098804222,3.97853879557646));
#93890=CARTESIAN_POINT('Ctrl Pts',(-8.68408874516995,23.6752444652851,4.14288411813394));
#93891=CARTESIAN_POINT('Ctrl Pts',(-8.70945373911387,23.6725101409102,4.19239579737966));
#93892=CARTESIAN_POINT('Ctrl Pts',(-8.75052123281472,23.6683442640722,4.26242404274384));
#93893=CARTESIAN_POINT('Ctrl Pts',(-8.76404794001469,23.667006106158,4.28416194603441));
#93894=CARTESIAN_POINT('Ctrl Pts',(-8.78124651768241,23.6653305055343,4.31024941699723));
#93895=CARTESIAN_POINT('Ctrl Pts',(-8.78438339982547,23.6650258772773,4.31494812576634));
#93896=CARTESIAN_POINT('Ctrl Pts',(-8.78934355318423,23.664545529096,4.32228553682562));
#93897=CARTESIAN_POINT('Ctrl Pts',(-8.79114846077446,23.664371012689,4.32493665938436));
#93898=CARTESIAN_POINT('Ctrl Pts',(-8.79454213814973,23.6640433449285,4.32988637840088));
#93899=CARTESIAN_POINT('Ctrl Pts',(-8.79612878409373,23.6638903348799,4.3321863690509));
#93900=CARTESIAN_POINT('Ctrl Pts',(-8.79978354159911,23.6635383156789,4.33745195371094));
#93901=CARTESIAN_POINT('Ctrl Pts',(-8.801856057825,23.6633390120951,4.34041443052928));
#93902=CARTESIAN_POINT('Ctrl Pts',(-8.80733262769193,23.6628132534526,4.34818126518695));
#93903=CARTESIAN_POINT('Ctrl Pts',(-8.81075470029879,23.6624856288094,4.35297276295648));
#93904=CARTESIAN_POINT('Ctrl Pts',(-8.83490304813642,23.660180695975,4.38635684649629));
#93905=CARTESIAN_POINT('Ctrl Pts',(-8.85662790605432,23.6581429586635,4.41420962021629));
#93906=CARTESIAN_POINT('Ctrl Pts',(-8.88058870871303,23.655954816684,4.44273771529126));
#93907=CARTESIAN_POINT('Ctrl Pts',(-8.88184356998543,23.6558403833516,4.44422573406034));
#93908=CARTESIAN_POINT('Ctrl Pts',(-8.89662388934563,23.654494484795,4.46168150429698));
#93909=CARTESIAN_POINT('Ctrl Pts',(-8.91048702115756,23.6532512627442,4.4773594938065));
#93910=CARTESIAN_POINT('Ctrl Pts',(-8.97952175168928,23.6471708933847,4.55213714495103));
#93911=CARTESIAN_POINT('Ctrl Pts',(-9.03919348808335,23.6422564068561,4.60689665050153));
#93912=CARTESIAN_POINT('Ctrl Pts',(-9.16035108970536,23.633175437658,4.70086405303821));
#93913=CARTESIAN_POINT('Ctrl Pts',(-9.22084552465803,23.6289954454839,4.74096959099842));
#93914=CARTESIAN_POINT('Ctrl Pts',(-9.2938331427261,23.6243638265268,4.78190713672895));
#93915=CARTESIAN_POINT('Ctrl Pts',(-9.30365826919754,23.6237483001826,4.78727065578239));
#93916=CARTESIAN_POINT('Ctrl Pts',(-9.31883244167052,23.622809609249,4.79532963435776));
#93917=CARTESIAN_POINT('Ctrl Pts',(-9.32413796563381,23.622483615709,4.798105780034));
#93918=CARTESIAN_POINT('Ctrl Pts',(-9.33383482729666,23.6218917718208,4.80310415250842));
#93919=CARTESIAN_POINT('Ctrl Pts',(-9.3382206025941,23.6216255556642,4.80533692953072));
#93920=CARTESIAN_POINT('Ctrl Pts',(-9.34781294306131,23.6210464605069,4.81015957311223));
#93921=CARTESIAN_POINT('Ctrl Pts',(-9.3530238633584,23.6207338907921,4.81274062335622));
#93922=CARTESIAN_POINT('Ctrl Pts',(-9.36733380977932,23.6198809521415,4.81972265998443));
#93923=CARTESIAN_POINT('Ctrl Pts',(-9.37646335519453,23.6193427573395,4.82406059792162));
#93924=CARTESIAN_POINT('Ctrl Pts',(-9.4237508163019,23.6165847779411,4.84593184192215));
#93925=CARTESIAN_POINT('Ctrl Pts',(-9.46260729887426,23.6144181499851,4.86191231395234));
#93926=CARTESIAN_POINT('Ctrl Pts',(-9.63599083623422,23.6050934835798,4.92464131622404));
#93927=CARTESIAN_POINT('Ctrl Pts',(-9.77621417859209,23.5985130682301,4.95327833017854));
#93928=CARTESIAN_POINT('Ctrl Pts',(-9.94836092545851,23.5897275599948,4.96289750402448));
#93929=CARTESIAN_POINT('Ctrl Pts',(-9.97841410790338,23.5881647724552,4.96364937866056));
#93930=CARTESIAN_POINT('Ctrl Pts',(-10.0143847984895,23.5862375972276,4.96344126957989));
#93931=CARTESIAN_POINT('Ctrl Pts',(-10.0203022696429,23.5859187237099,4.9633711379504));
#93932=CARTESIAN_POINT('Ctrl Pts',(-10.0294842333617,23.5854208652798,4.96320661385304));
#93933=CARTESIAN_POINT('Ctrl Pts',(-10.0327491783033,23.5852432326608,4.96313717939708));
#93934=CARTESIAN_POINT('Ctrl Pts',(-10.038799784885,23.5849128816183,4.96298824087418));
#93935=CARTESIAN_POINT('Ctrl Pts',(-10.041585466855,23.5847603286252,4.96291170779709));
#93936=CARTESIAN_POINT('Ctrl Pts',(-10.0479001802112,23.5844134763294,4.96272016801026));
#93937=CARTESIAN_POINT('Ctrl Pts',(-10.0514290077657,23.5842189150392,4.96260034657077));
#93938=CARTESIAN_POINT('Ctrl Pts',(-10.0605607399908,23.5837136073046,4.9622571898706));
#93939=CARTESIAN_POINT('Ctrl Pts',(-10.06616280344,23.5834018302963,4.9620144232989));
#93940=CARTESIAN_POINT('Ctrl Pts',(-10.1015524847365,23.5814215666116,4.96027698769106));
#93941=CARTESIAN_POINT('Ctrl Pts',(-10.1312880617372,23.5797099148056,4.95790431246343));
#93942=CARTESIAN_POINT('Ctrl Pts',(-10.3059844534842,23.5694512341025,4.93857729052175));
#93943=CARTESIAN_POINT('Ctrl Pts',(-10.4478332918166,23.5604000257373,4.9009239418998));
#93944=CARTESIAN_POINT('Ctrl Pts',(-10.6178548370982,23.5497402358234,4.82726523545954));
#93945=CARTESIAN_POINT('Ctrl Pts',(-10.6532840365219,23.5475226475161,4.81019005742227));
#93946=CARTESIAN_POINT('Ctrl Pts',(-10.6964413787712,23.5448252378798,4.7872037323046));
#93947=CARTESIAN_POINT('Ctrl Pts',(-10.7048532820597,23.5442996313555,4.78261681706844));
#93948=CARTESIAN_POINT('Ctrl Pts',(-10.7181439941829,23.5434692910718,4.77519930025588));
#93949=CARTESIAN_POINT('Ctrl Pts',(-10.7230524305683,23.5431626594194,4.77242258532526));
#93950=CARTESIAN_POINT('Ctrl Pts',(-10.7322683720483,23.5425869415287,4.76713855612959));
#93951=CARTESIAN_POINT('Ctrl Pts',(-10.7365793458197,23.5423176379663,4.76463748058266));
#93952=CARTESIAN_POINT('Ctrl Pts',(-10.7462598382276,23.541712870559,4.75895490622871));
#93953=CARTESIAN_POINT('Ctrl Pts',(-10.7516219696941,23.541377859835,4.75576097183759));
#93954=CARTESIAN_POINT('Ctrl Pts',(-10.7652840618685,23.5405241338797,4.74750433698011));
#93955=CARTESIAN_POINT('Ctrl Pts',(-10.7735543771945,23.5400071845511,4.74239301259026));
#93956=CARTESIAN_POINT('Ctrl Pts',(-10.8242641229988,23.5368355315662,4.71035006230517));
#93957=CARTESIAN_POINT('Ctrl Pts',(-10.8653458494322,23.5342591811885,4.68132800874782));
#93958=CARTESIAN_POINT('Ctrl Pts',(-11.0099878620285,23.5250315900361,4.56754362834255));
#93959=CARTESIAN_POINT('Ctrl Pts',(-11.1032720823039,23.5188190513534,4.47082907660747));
#93960=CARTESIAN_POINT('Ctrl Pts',(-11.1994648900954,23.5104969730295,4.33903637219664));
#93961=CARTESIAN_POINT('Ctrl Pts',(-11.2160902273755,23.5089659483734,4.31475295792951));
#93962=CARTESIAN_POINT('Ctrl Pts',(-11.235146861266,23.5070743189959,4.28503445181814));
#93963=CARTESIAN_POINT('Ctrl Pts',(-11.2382925069395,23.506757300823,4.28006315406942));
#93964=CARTESIAN_POINT('Ctrl Pts',(-11.2431335549875,23.5062617212544,4.2723094133114));
#93965=CARTESIAN_POINT('Ctrl Pts',(-11.2448498184939,23.5060844923462,4.26953998882264));
#93966=CARTESIAN_POINT('Ctrl Pts',(-11.2480172776146,23.5057545000391,4.26439053845503));
#93967=CARTESIAN_POINT('Ctrl Pts',(-11.2494709290368,23.5056018989879,4.26201208494968));
#93968=CARTESIAN_POINT('Ctrl Pts',(-11.2527558029482,23.5052544281633,4.25660272787043));
#93969=CARTESIAN_POINT('Ctrl Pts',(-11.2545828175223,23.5050592924624,4.25356933528042));
#93970=CARTESIAN_POINT('Ctrl Pts',(-11.2601134945302,23.504462909639,4.2443108890349));
#93971=CARTESIAN_POINT('Ctrl Pts',(-11.2637819081826,23.5040594943091,4.23806503966421));
#93972=CARTESIAN_POINT('Ctrl Pts',(-11.2987298205431,23.5001415870304,4.17753815050211));
#93973=CARTESIAN_POINT('Ctrl Pts',(-11.3265368152965,23.4964401316593,4.12133369070578));
#93974=CARTESIAN_POINT('Ctrl Pts',(-11.3818491481376,23.487835051943,3.9887618787863));
#93975=CARTESIAN_POINT('Ctrl Pts',(-11.4067833023341,23.4829173331846,3.91153031144746));
#93976=CARTESIAN_POINT('Ctrl Pts',(-11.4353262932692,23.4755080236475,3.78923438261099));
#93977=CARTESIAN_POINT('Ctrl Pts',(-11.4434679743336,23.472921971183,3.74539527512577));
#93978=CARTESIAN_POINT('Ctrl Pts',(-11.4533340272061,23.4688532343965,3.67433037236646));
#93979=CARTESIAN_POINT('Ctrl Pts',(-11.4563208811755,23.4673343047547,3.6473109068342));
#93980=CARTESIAN_POINT('Ctrl Pts',(-11.459249067983,23.4653728503826,3.61178582297373));
#93981=CARTESIAN_POINT('Ctrl Pts',(-11.4598712712659,23.4649093132918,3.60334306066155));
#93982=CARTESIAN_POINT('Ctrl Pts',(-11.4607699047658,23.4641541887159,3.58951325845839));
#93983=CARTESIAN_POINT('Ctrl Pts',(-11.4610898656212,23.4638612546469,3.58412932766789));
#93984=CARTESIAN_POINT('Ctrl Pts',(-11.4616515599508,23.4632960447493,3.57370501575531));
#93985=CARTESIAN_POINT('Ctrl Pts',(-11.4618970011509,23.4630236576435,3.56866491798058));
#93986=CARTESIAN_POINT('Ctrl Pts',(-11.4624037093391,23.4623963519076,3.55702039848241));
#93987=CARTESIAN_POINT('Ctrl Pts',(-11.4626463139728,23.4620420170152,3.55041524676307));
#93988=CARTESIAN_POINT('Ctrl Pts',(-11.4632813540841,23.4609091098581,3.52921017164921));
#93989=CARTESIAN_POINT('Ctrl Pts',(-11.4635,23.4601359197492,3.51460567629416));
#93990=CARTESIAN_POINT('Ctrl Pts',(-11.4635,23.4593691294935,3.50000000000014));
#93991=CARTESIAN_POINT('Ctrl Pts',(-11.4635,23.3906983315425,3.49999999997929));
#93992=CARTESIAN_POINT('Ctrl Pts',(-11.4635000000001,23.3912074294038,3.50921703575764));
#93993=CARTESIAN_POINT('Ctrl Pts',(-11.4634129275492,23.3917138314248,3.51843406141093));
#93994=CARTESIAN_POINT('Ctrl Pts',(-11.4631244128564,23.3925483519854,3.53370234837801));
#93995=CARTESIAN_POINT('Ctrl Pts',(-11.4629724897685,23.3928779932348,3.53975413817928));
#93996=CARTESIAN_POINT('Ctrl Pts',(-11.4626273931823,23.3934762749692,3.55077483019609));
#93997=CARTESIAN_POINT('Ctrl Pts',(-11.4624464372592,23.3937452902563,3.55574400113536));
#93998=CARTESIAN_POINT('Ctrl Pts',(-11.4620003484589,23.3943253544777,3.5664879537063));
#93999=CARTESIAN_POINT('Ctrl Pts',(-11.461726318057,23.394636122758,3.5722622951167));
#94000=CARTESIAN_POINT('Ctrl Pts',(-11.4608874126257,23.3954790516295,3.58797310230369));
#94001=CARTESIAN_POINT('Ctrl Pts',(-11.4602553767715,23.3960091240089,3.59790577235364));
#94002=CARTESIAN_POINT('Ctrl Pts',(-11.4565795420355,23.3986509037902,3.64765902006547));
#94003=CARTESIAN_POINT('Ctrl Pts',(-11.4520079048078,23.4007148223623,3.68735143334495));
#94004=CARTESIAN_POINT('Ctrl Pts',(-11.4433918987835,23.4035328160469,3.74227492096282));
#94005=CARTESIAN_POINT('Ctrl Pts',(-11.440717792496,23.4043201497397,3.75770054492073));
#94006=CARTESIAN_POINT('Ctrl Pts',(-11.4192878089853,23.4100586458689,3.87053155916608));
#94007=CARTESIAN_POINT('Ctrl Pts',(-11.3909205558537,23.414773281846,3.96584434415665));
#94008=CARTESIAN_POINT('Ctrl Pts',(-11.3329290384623,23.4222857546511,4.10658431205819));
#94009=CARTESIAN_POINT('Ctrl Pts',(-11.3100781448902,23.424953532139,4.15447579479587));
#94010=CARTESIAN_POINT('Ctrl Pts',(-11.2797193890136,23.4283062234842,4.21011116313542));
#94011=CARTESIAN_POINT('Ctrl Pts',(-11.2746606830645,23.428859404488,4.21915207677826));
#94012=CARTESIAN_POINT('Ctrl Pts',(-11.2674699191754,23.4296392926779,4.23168914895539));
#94013=CARTESIAN_POINT('Ctrl Pts',(-11.2654184090124,23.4298610859948,4.2352314302484));
#94014=CARTESIAN_POINT('Ctrl Pts',(-11.2619037256965,23.4302399521439,4.24124184279518));
#94015=CARTESIAN_POINT('Ctrl Pts',(-11.2604480879947,23.4303965437505,4.24371439396251));
#94016=CARTESIAN_POINT('Ctrl Pts',(-11.2576417667,23.4306978565715,4.24844931642227));
#94017=CARTESIAN_POINT('Ctrl Pts',(-11.2562922334766,23.430842499369,4.250712339368));
#94018=CARTESIAN_POINT('Ctrl Pts',(-11.2526867675871,23.43122822969,4.25672137159404));
#94019=CARTESIAN_POINT('Ctrl Pts',(-11.2504201627304,23.4314699972862,4.2604609046783));
#94020=CARTESIAN_POINT('Ctrl Pts',(-11.2422275209524,23.4323411244157,4.27384178624076));
#94021=CARTESIAN_POINT('Ctrl Pts',(-11.236206609363,23.4329762483821,4.28342423171753));
#94022=CARTESIAN_POINT('Ctrl Pts',(-11.1849399700597,23.4383361116751,4.36295380733965));
#94023=CARTESIAN_POINT('Ctrl Pts',(-11.1339123406492,23.4433564274495,4.42898467047999));
#94024=CARTESIAN_POINT('Ctrl Pts',(-11.0003776861745,23.4552409214194,4.57428293112232));
#94025=CARTESIAN_POINT('Ctrl Pts',(-10.9136394915394,23.4620351592899,4.6489607599487));
#94026=CARTESIAN_POINT('Ctrl Pts',(-10.8061105600909,23.4692734297799,4.72158238463592));
#94027=CARTESIAN_POINT('Ctrl Pts',(-10.7929854823801,23.470139782948,4.73014300352123));
#94028=CARTESIAN_POINT('Ctrl Pts',(-10.7739253172125,23.4713738862977,4.74214283536102));
#94029=CARTESIAN_POINT('Ctrl Pts',(-10.7680999015707,23.4717479088373,4.74575349227136));
#94030=CARTESIAN_POINT('Ctrl Pts',(-10.7579227196591,23.4723959254996,4.75196289415709));
#94031=CARTESIAN_POINT('Ctrl Pts',(-10.7535824516535,23.4726705914718,4.75458017949424));
#94032=CARTESIAN_POINT('Ctrl Pts',(-10.7451839016029,23.4731988532377,4.7595853973536));
#94033=CARTESIAN_POINT('Ctrl Pts',(-10.741127525107,23.4734525574434,4.7619763914895));
#94034=CARTESIAN_POINT('Ctrl Pts',(-10.7314866795827,23.4740521761558,4.76759658418733));
#94035=CARTESIAN_POINT('Ctrl Pts',(-10.7258922338726,23.4743974699716,4.77080853367548));
#94036=CARTESIAN_POINT('Ctrl Pts',(-10.7060575681069,23.475612490521,4.78202253127321));
#94037=CARTESIAN_POINT('Ctrl Pts',(-10.6917045203374,23.4764750830559,4.78982322233451));
#94038=CARTESIAN_POINT('Ctrl Pts',(-10.5710905347894,23.4835938031456,4.85278279158265));
#94039=CARTESIAN_POINT('Ctrl Pts',(-10.4585633439973,23.4893548244639,4.8949508375397));
#94040=CARTESIAN_POINT('Ctrl Pts',(-10.2852621820657,23.4980382713809,4.93662135274832));
#94041=CARTESIAN_POINT('Ctrl Pts',(-10.2276102801366,23.5009074934132,4.94687527445646));
#94042=CARTESIAN_POINT('Ctrl Pts',(-10.1432937750199,23.5052579058688,4.95670706039194));
#94043=CARTESIAN_POINT('Ctrl Pts',(-10.1170072954747,23.5066359145043,4.95905369546237));
#94044=CARTESIAN_POINT('Ctrl Pts',(-10.084982086561,23.5083562586701,4.96104168710037));
#94045=CARTESIAN_POINT('Ctrl Pts',(-10.0792887970383,23.5086636851918,4.96136171121067));
#94046=CARTESIAN_POINT('Ctrl Pts',(-10.0703785277654,23.5091475108078,4.96181034252474));
#94047=CARTESIAN_POINT('Ctrl Pts',(-10.0671626844056,23.5093226779747,4.96196162333239));
#94048=CARTESIAN_POINT('Ctrl Pts',(-10.0611555791827,23.509650950606,4.96222434965143));
#94049=CARTESIAN_POINT('Ctrl Pts',(-10.0583644835089,23.5098039100244,4.96233841508109));
#94050=CARTESIAN_POINT('Ctrl Pts',(-10.0519759898551,23.5101549985461,4.96258117868936));
#94051=CARTESIAN_POINT('Ctrl Pts',(-10.0483784420901,23.5103534157619,4.96270459544909));
#94052=CARTESIAN_POINT('Ctrl Pts',(-10.0389500161523,23.5108752181624,4.96299322377851));
#94053=CARTESIAN_POINT('Ctrl Pts',(-10.0331186003284,23.5111997449206,4.96313684683909));
#94054=CARTESIAN_POINT('Ctrl Pts',(-9.99311175813237,23.5134377751768,4.96388289383226));
#94055=CARTESIAN_POINT('Ctrl Pts',(-9.95892760717565,23.5154079173911,4.96332268288292));
#94056=CARTESIAN_POINT('Ctrl Pts',(-9.82457592999175,23.5232996323083,4.95640981504714));
#94057=CARTESIAN_POINT('Ctrl Pts',(-9.7251514606692,23.5294445074818,4.94095875797759));
#94058=CARTESIAN_POINT('Ctrl Pts',(-9.57829745194627,23.5384629635976,4.90237282047192));
#94059=CARTESIAN_POINT('Ctrl Pts',(-9.52922797043155,23.5414705900432,4.8866712140115));
#94060=CARTESIAN_POINT('Ctrl Pts',(-9.45299685464826,23.5461107510936,4.85776366144886));
#94061=CARTESIAN_POINT('Ctrl Pts',(-9.42524264703663,23.5477935047904,4.84624989266624));
#94062=CARTESIAN_POINT('Ctrl Pts',(-9.38986601936233,23.5499308395707,4.83028031644137));
#94063=CARTESIAN_POINT('Ctrl Pts',(-9.38190355055782,23.5504114163702,4.8265994039391));
#94064=CARTESIAN_POINT('Ctrl Pts',(-9.36903755682835,23.551187257947,4.82051068822291));
#94065=CARTESIAN_POINT('Ctrl Pts',(-9.36411365287844,23.5514840129918,4.81814666751325));
#94066=CARTESIAN_POINT('Ctrl Pts',(-9.35468604669761,23.5520519190293,4.81355524985056));
#94067=CARTESIAN_POINT('Ctrl Pts',(-9.35018036182279,23.5523232119286,4.8113321209541));
#94068=CARTESIAN_POINT('Ctrl Pts',(-9.33990758163315,23.5529415065507,4.80619752853585));
#94069=CARTESIAN_POINT('Ctrl Pts',(-9.33414811394634,23.5532879795763,4.80327098180013));
#94070=CARTESIAN_POINT('Ctrl Pts',(-9.31892193142294,23.5542035884413,4.79540685039448));
#94071=CARTESIAN_POINT('Ctrl Pts',(-9.30948945320616,23.5547704310484,4.79040359435589));
#94072=CARTESIAN_POINT('Ctrl Pts',(-9.21408026041001,23.5605025744142,4.73845008775281));
#94073=CARTESIAN_POINT('Ctrl Pts',(-9.13296612948781,23.5653403437218,4.68308232362608));
#94074=CARTESIAN_POINT('Ctrl Pts',(-9.00446566970936,23.5735173533358,4.57500428320357));
#94075=CARTESIAN_POINT('Ctrl Pts',(-8.95424396841218,23.5768855711764,4.52621453271419));
#94076=CARTESIAN_POINT('Ctrl Pts',(-8.88852742325798,23.5818331800146,4.4525183704844));
#94077=CARTESIAN_POINT('Ctrl Pts',(-8.86999028792273,23.583299498442,4.43045172412937));
#94078=CARTESIAN_POINT('Ctrl Pts',(-8.84521299814401,23.5853828488466,4.39912352722885));
#94079=CARTESIAN_POINT('Ctrl Pts',(-8.83840844824702,23.5859687850385,4.39031521956254));
#94080=CARTESIAN_POINT('Ctrl Pts',(-8.82677171945817,23.5869967335051,4.37489127967897));
#94081=CARTESIAN_POINT('Ctrl Pts',(-8.82189332148713,23.5874358833291,4.36831100269691));
#94082=CARTESIAN_POINT('Ctrl Pts',(-8.81487822977822,23.5880799981029,4.35868067615856));
#94083=CARTESIAN_POINT('Ctrl Pts',(-8.81269744491141,23.5882820480314,4.35566275828639));
#94084=CARTESIAN_POINT('Ctrl Pts',(-8.80889243524333,23.5886378425583,4.35035457461003));
#94085=CARTESIAN_POINT('Ctrl Pts',(-8.80726325325438,23.588791246254,4.3480679137093));
#94086=CARTESIAN_POINT('Ctrl Pts',(-8.8038225045393,23.5891175134407,4.34320907656469));
#94087=CARTESIAN_POINT('Ctrl Pts',(-8.80201267740766,23.5892904836699,4.34063578437401));
#94088=CARTESIAN_POINT('Ctrl Pts',(-8.79713646055003,23.5897601544766,4.33365483611582));
#94089=CARTESIAN_POINT('Ctrl Pts',(-8.79408603865047,23.5900578994709,4.3292361523121));
#94090=CARTESIAN_POINT('Ctrl Pts',(-8.78027535397555,23.5914236422683,4.3089933405341));
#94091=CARTESIAN_POINT('Ctrl Pts',(-8.76980225136383,23.5925090094735,4.2929765848516));
#94092=CARTESIAN_POINT('Ctrl Pts',(-8.74942540632657,23.5947160802679,4.26043823450301));
#94093=CARTESIAN_POINT('Ctrl Pts',(-8.73952762730232,23.595837770075,4.24391697436218));
#94094=CARTESIAN_POINT('Ctrl Pts',(-8.72494000965346,23.5975637848104,4.21844018529922));
#94095=CARTESIAN_POINT('Ctrl Pts',(-8.72001186434161,23.5981604876917,4.20962288951818));
#94096=CARTESIAN_POINT('Ctrl Pts',(-8.67045171980135,23.6042983895561,4.11875510921249));
#94097=CARTESIAN_POINT('Ctrl Pts',(-8.63368012113684,23.6100006217181,4.03266095603095));
#94098=CARTESIAN_POINT('Ctrl Pts',(-8.58563102793481,23.6193833890263,3.88161488111155));
#94099=CARTESIAN_POINT('Ctrl Pts',(-8.57005707368791,23.6231466901718,3.81833077532525));
#94100=CARTESIAN_POINT('Ctrl Pts',(-8.55607393135115,23.6276353357323,3.73905377258055));
#94101=CARTESIAN_POINT('Ctrl Pts',(-8.55363938058424,23.6284861942424,3.72385303651734));
#94102=CARTESIAN_POINT('Ctrl Pts',(-8.55047502946003,23.6297023538986,3.70188094432194));
#94103=CARTESIAN_POINT('Ctrl Pts',(-8.54955200184913,23.6300736784682,3.69513882942634));
#94104=CARTESIAN_POINT('Ctrl Pts',(-8.54802464389022,23.6307185540238,3.68337235539854));
#94105=CARTESIAN_POINT('Ctrl Pts',(-8.54739929122677,23.6309927583898,3.67835088236336));
#94106=CARTESIAN_POINT('Ctrl Pts',(-8.54624086449818,23.6315212150679,3.66863841238113));
#94107=CARTESIAN_POINT('Ctrl Pts',(-8.5457044216321,23.6317755694375,3.66394788697628));
#94108=CARTESIAN_POINT('Ctrl Pts',(-8.544483445273,23.6323784057571,3.65279414041362));
#94109=CARTESIAN_POINT('Ctrl Pts',(-8.54381924697325,23.6327262508379,3.64632876269826));
#94110=CARTESIAN_POINT('Ctrl Pts',(-8.54160941330306,23.6339591422253,3.62331066987504));
#94111=CARTESIAN_POINT('Ctrl Pts',(-8.54030273999111,23.6348367716442,3.60673595195195));
#94112=CARTESIAN_POINT('Ctrl Pts',(-8.53215590185929,23.6417538883302,3.4747192922915));
#94113=CARTESIAN_POINT('Ctrl Pts',(-8.5387376484625,23.6473367116108,3.35886047152888));
#94114=CARTESIAN_POINT('Ctrl Pts',(-8.57386758289224,23.6571493904704,3.16034538405839));
#94115=CARTESIAN_POINT('Ctrl Pts',(-8.59626830586342,23.661354714722,3.07720876805326));
#94116=CARTESIAN_POINT('Ctrl Pts',(-8.6283330912345,23.6663266552157,2.98969108657156));
#94117=CARTESIAN_POINT('Ctrl Pts',(-8.63088962320762,23.6667178511021,2.98287132403634));
#94118=CARTESIAN_POINT('Ctrl Pts',(-8.6347676903831,23.6673040540762,2.97275661092185));
#94119=CARTESIAN_POINT('Ctrl Pts',(-8.63605052306429,23.6674968357774,2.96944682229547));
#94120=CARTESIAN_POINT('Ctrl Pts',(-8.63836277762046,23.6678423740748,2.96354487268786));
#94121=CARTESIAN_POINT('Ctrl Pts',(-8.6393875804885,23.6679948553176,2.96095095519485));
#94122=CARTESIAN_POINT('Ctrl Pts',(-8.64162409435158,23.6683262148944,2.95533704257536));
#94123=CARTESIAN_POINT('Ctrl Pts',(-8.64283844730232,23.6685052455081,2.95231819667746));
#94124=CARTESIAN_POINT('Ctrl Pts',(-8.64620931932002,23.6689997375778,2.94401836138178));
#94125=CARTESIAN_POINT('Ctrl Pts',(-8.64838663869101,23.6693164042342,2.93874594975514));
#94126=CARTESIAN_POINT('Ctrl Pts',(-8.65968336054095,23.6709450795215,2.91183775385509));
#94127=CARTESIAN_POINT('Ctrl Pts',(-8.66929117634481,23.6722835094616,2.89041208997631));
#94128=CARTESIAN_POINT('Ctrl Pts',(-8.6821257881266,23.6740069534355,2.86354141700963));
#94129=CARTESIAN_POINT('Ctrl Pts',(-8.68487866764491,23.6743731359694,2.85787240726105));
#94130=CARTESIAN_POINT('Ctrl Pts',(-8.73430206442872,23.6808843924724,2.75774574992416));
#94131=CARTESIAN_POINT('Ctrl Pts',(-8.79100076328839,23.6873469492549,2.66858310208491));
#94132=CARTESIAN_POINT('Ctrl Pts',(-8.88918141947249,23.6966904549748,2.54574251604854));
#94133=CARTESIAN_POINT('Ctrl Pts',(-8.92371634816917,23.6997233753054,2.50695439417005));
#94134=CARTESIAN_POINT('Ctrl Pts',(-8.98149663479204,23.704397306475,2.44862216364288));
#94135=CARTESIAN_POINT('Ctrl Pts',(-9.00341163434028,23.7060894467004,2.42782637641828));
#94136=CARTESIAN_POINT('Ctrl Pts',(-9.03251486834469,23.7082367861879,2.40187341127457));
#94137=CARTESIAN_POINT('Ctrl Pts',(-9.03912665820261,23.7087182821949,2.39608337697353));
#94138=CARTESIAN_POINT('Ctrl Pts',(-9.04993435879627,23.7094952377843,2.38678959780096));
#94139=CARTESIAN_POINT('Ctrl Pts',(-9.05409838086998,23.7097921955656,2.38324924436234));
#94140=CARTESIAN_POINT('Ctrl Pts',(-9.06212721379505,23.7103602464071,2.37650005858213));
#94141=CARTESIAN_POINT('Ctrl Pts',(-9.0659888971158,23.7106314829962,2.37328764006588));
#94142=CARTESIAN_POINT('Ctrl Pts',(-9.07484882257735,23.7112493156504,2.36599418673633));
#94143=CARTESIAN_POINT('Ctrl Pts',(-9.07985768874789,23.7115953857987,2.36192618233066));
#94144=CARTESIAN_POINT('Ctrl Pts',(-9.09320513927605,23.7125092181573,2.35123162959849));
#94145=CARTESIAN_POINT('Ctrl Pts',(-9.1015895202636,23.7130747015515,2.34466268729551));
#94146=CARTESIAN_POINT('Ctrl Pts',(-9.17207181688326,23.7177595741196,2.29067292883538));
#94147=CARTESIAN_POINT('Ctrl Pts',(-9.23780684439185,23.7216789204664,2.24820103123834));
#94148=CARTESIAN_POINT('Ctrl Pts',(-9.36512936956547,23.7287750257926,2.17970274562462));
#94149=CARTESIAN_POINT('Ctrl Pts',(-9.42570712249699,23.7319693083531,2.15224888152499));
#94150=CARTESIAN_POINT('Ctrl Pts',(-9.53032754788325,23.7374534491439,2.113173614276));
#94151=CARTESIAN_POINT('Ctrl Pts',(-9.57342439056545,23.7397050746534,2.09931717969435));
#94152=CARTESIAN_POINT('Ctrl Pts',(-9.63885413113765,23.7432019411162,2.08158032820589));
#94153=CARTESIAN_POINT('Ctrl Pts',(-9.66074984669421,23.744385086094,2.07618472889172));
#94154=CARTESIAN_POINT('Ctrl Pts',(-9.68806376261951,23.7458866348142,2.07011974340862));
#94155=CARTESIAN_POINT('Ctrl Pts',(-9.69337373615627,23.7461797374485,2.06897166456006));
#94156=CARTESIAN_POINT('Ctrl Pts',(-9.70178223699026,23.7466459331697,2.06720259572797));
#94157=CARTESIAN_POINT('Ctrl Pts',(-9.70487664872617,23.7468179377778,2.06656201982508));
#94158=CARTESIAN_POINT('Ctrl Pts',(-9.71072110873403,23.7471436760102,2.06537188168046));
#94159=CARTESIAN_POINT('Ctrl Pts',(-9.71347067547705,23.7472972888507,2.06482019923414));
#94160=CARTESIAN_POINT('Ctrl Pts',(-9.71978817208197,23.7476510628716,2.06357151328188));
#94161=CARTESIAN_POINT('Ctrl Pts',(-9.72335712560096,23.7478515238229,2.06287989874965));
#94162=CARTESIAN_POINT('Ctrl Pts',(-9.73290660553494,23.7483894406915,2.06106622998448));
#94163=CARTESIAN_POINT('Ctrl Pts',(-9.73889154979099,23.748728183542,2.05996817727254));
#94164=CARTESIAN_POINT('Ctrl Pts',(-9.78434068015442,23.7513118893759,2.05192230718739));
#94165=CARTESIAN_POINT('Ctrl Pts',(-9.8240653539505,23.7536344875168,2.04656118086459));
#94166=CARTESIAN_POINT('Ctrl Pts',(-9.95141974968251,23.7611825599238,2.03467110851035));
#94167=CARTESIAN_POINT('Ctrl Pts',(-10.0394401651108,23.7665406072006,2.03439652104904));
#94168=CARTESIAN_POINT('Ctrl Pts',(-10.2094693422858,23.7767121510989,2.04920188757023));
#94169=CARTESIAN_POINT('Ctrl Pts',(-10.2912345862112,23.7815210109707,2.06337945700882));
#94170=CARTESIAN_POINT('Ctrl Pts',(-10.3824512719545,23.7867429806841,2.08730948789723));
#94171=CARTESIAN_POINT('Ctrl Pts',(-10.3934966717795,23.7873731098237,2.09034619917073));
#94172=CARTESIAN_POINT('Ctrl Pts',(-10.4103140338702,23.7883293527013,2.09518286839099));
#94173=CARTESIAN_POINT('Ctrl Pts',(-10.4161122157039,23.7886584611566,2.09688938243383));
#94174=CARTESIAN_POINT('Ctrl Pts',(-10.4266605943626,23.7892561833274,2.10006510596323));
#94175=CARTESIAN_POINT('Ctrl Pts',(-10.4314141724557,23.7895251682968,2.10152269129109));
#94176=CARTESIAN_POINT('Ctrl Pts',(-10.4416859068248,23.7901056236096,2.10472966110867));
#94177=CARTESIAN_POINT('Ctrl Pts',(-10.447201311261,23.7904168102328,2.10648762208454));
#94178=CARTESIAN_POINT('Ctrl Pts',(-10.4622034260914,23.7912619961072,2.11136758495307));
#94179=CARTESIAN_POINT('Ctrl Pts',(-10.4716689373083,23.7917938881245,2.11455407488816));
#94180=CARTESIAN_POINT('Ctrl Pts',(-10.5192478743587,23.7944614171595,2.13111528395226));
#94181=CARTESIAN_POINT('Ctrl Pts',(-10.5568303053279,23.7965481022977,2.14596746333614));
#94182=CARTESIAN_POINT('Ctrl Pts',(-10.6071965002018,23.7993398329171,2.16832398383076));
#94183=CARTESIAN_POINT('Ctrl Pts',(-10.6205499732611,23.8000796116419,2.17449392787499));
#94184=CARTESIAN_POINT('Ctrl Pts',(-10.7236865949669,23.8057989703966,2.22404823334212));
#94185=CARTESIAN_POINT('Ctrl Pts',(-10.8089124218148,23.8105374522379,2.27630260807894));
#94186=CARTESIAN_POINT('Ctrl Pts',(-10.9302446611886,23.8180721266269,2.36894717852285));
#94187=CARTESIAN_POINT('Ctrl Pts',(-10.97054817513,23.8207360104829,2.40333650516365));
#94188=CARTESIAN_POINT('Ctrl Pts',(-11.0163951107256,23.824083981939,2.446966102421));
#94189=CARTESIAN_POINT('Ctrl Pts',(-11.0238179203126,23.8246367374346,2.45418153368306));
#94190=CARTESIAN_POINT('Ctrl Pts',(-11.0340672627171,23.825416123773,2.46435822193894));
#94191=CARTESIAN_POINT('Ctrl Pts',(-11.0369590336273,23.8256378491634,2.46725368165889));
#94192=CARTESIAN_POINT('Ctrl Pts',(-11.0418574412937,23.8260166344921,2.47219965309399));
#94193=CARTESIAN_POINT('Ctrl Pts',(-11.0438702867074,23.8261732137143,2.47424403219436));
#94194=CARTESIAN_POINT('Ctrl Pts',(-11.0477204068644,23.8264745322719,2.47817753824375));
#94195=CARTESIAN_POINT('Ctrl Pts',(-11.0495586057889,23.8266191933508,2.48006572412928));
#94196=CARTESIAN_POINT('Ctrl Pts',(-11.0544346147417,23.8270050284649,2.48510146874311));
#94197=CARTESIAN_POINT('Ctrl Pts',(-11.0574634044309,23.8272468832122,2.48825767470511));
#94198=CARTESIAN_POINT('Ctrl Pts',(-11.0682835557755,23.8281186250283,2.49963467589067));
#94199=CARTESIAN_POINT('Ctrl Pts',(-11.0759933709856,23.8287542867525,2.5079320654771));
#94200=CARTESIAN_POINT('Ctrl Pts',(-11.1353419302449,23.8337560246244,2.57330932742279));
#94201=CARTESIAN_POINT('Ctrl Pts',(-11.1824968697725,23.8383752703551,2.63428873496673));
#94202=CARTESIAN_POINT('Ctrl Pts',(-11.2599362719332,23.8468910854631,2.7526380550076));
#94203=CARTESIAN_POINT('Ctrl Pts',(-11.2916364442379,23.8507749371621,2.80886657267899));
#94204=CARTESIAN_POINT('Ctrl Pts',(-11.3444467221146,23.8579583824061,2.91895354179092));
#94205=CARTESIAN_POINT('Ctrl Pts',(-11.3662798428304,23.8612705589165,2.9723328669278));
#94206=CARTESIAN_POINT('Ctrl Pts',(-11.3895782093693,23.8652825537784,3.04052951177835));
#94207=CARTESIAN_POINT('Ctrl Pts',(-11.3940437773868,23.8660798044702,3.05426162692007));
#94208=CARTESIAN_POINT('Ctrl Pts',(-11.4002628856262,23.8672335885791,3.0743944503738));
#94209=CARTESIAN_POINT('Ctrl Pts',(-11.4021771878489,23.8675953208337,3.08074426821107));
#94210=CARTESIAN_POINT('Ctrl Pts',(-11.4054682768792,23.868229117632,3.09193566012703));
#94211=CARTESIAN_POINT('Ctrl Pts',(-11.4068633631765,23.8685017705102,3.09677170111645));
#94212=CARTESIAN_POINT('Ctrl Pts',(-11.4097128521104,23.8690671452016,3.10684423040019));
#94213=CARTESIAN_POINT('Ctrl Pts',(-11.4111630924045,23.8693597292699,3.11208182266669));
#94214=CARTESIAN_POINT('Ctrl Pts',(-11.4148452621738,23.870115452321,3.12567405501381));
#94215=CARTESIAN_POINT('Ctrl Pts',(-11.4170324021359,23.8705771505744,3.13404070525964));
#94216=CARTESIAN_POINT('Ctrl Pts',(-11.4261910350154,23.8725684127715,3.17038966971276));
#94217=CARTESIAN_POINT('Ctrl Pts',(-11.4324090284434,23.8740739152525,3.19855620594468));
#94218=CARTESIAN_POINT('Ctrl Pts',(-11.4468430287676,23.8780505865583,3.27454401483362));
#94219=CARTESIAN_POINT('Ctrl Pts',(-11.4535207052353,23.880476716683,3.32262133396581));
#94220=CARTESIAN_POINT('Ctrl Pts',(-11.461599903769,23.8849905269656,3.41388284459606));
#94221=CARTESIAN_POINT('Ctrl Pts',(-11.46349999621,23.8870825918401,3.45694326727398));
#94222=CARTESIAN_POINT('Ctrl Pts',(-11.4635,23.8891760003868,3.49999987117833));
#94223=CARTESIAN_POINT('Origin',(-10.,13.2,3.5));
#94224=CARTESIAN_POINT('',(-11.4635,24.4618423224409,3.5000000024766));
#94225=CARTESIAN_POINT('',(-11.4635,24.3883362350912,3.49999997785042));
#94226=CARTESIAN_POINT('',(-11.4635,13.2,3.5));
#94227=CARTESIAN_POINT('',(-11.4634993894688,23.9606357550012,3.50131794111532));
#94228=CARTESIAN_POINT('Ctrl Pts',(-11.4635,24.4618423224409,3.5000000024766));
#94229=CARTESIAN_POINT('Ctrl Pts',(-11.4635000000413,24.4605992464299,3.47560470021283));
#94230=CARTESIAN_POINT('Ctrl Pts',(-11.4628900255798,24.4593350241618,3.45121150056634));
#94231=CARTESIAN_POINT('Ctrl Pts',(-11.4612084486067,24.4575508424555,3.41761358387352));
#94232=CARTESIAN_POINT('Ctrl Pts',(-11.4606590987307,24.4570564898491,3.40838864519993));
#94233=CARTESIAN_POINT('Ctrl Pts',(-11.4597544135585,24.456347357988,3.3952887978131));
#94234=CARTESIAN_POINT('Ctrl Pts',(-11.4594709207471,24.4561364416346,3.39140895733704));
#94235=CARTESIAN_POINT('Ctrl Pts',(-11.4589552409549,24.4557711333003,3.38471857087606));
#94236=CARTESIAN_POINT('Ctrl Pts',(-11.4587303949448,24.4556171524389,3.38190750334044));
#94237=CARTESIAN_POINT('Ctrl Pts',(-11.4582451514157,24.4552954668714,3.3760538293116));
#94238=CARTESIAN_POINT('Ctrl Pts',(-11.4579833598935,24.4551276921148,3.3730114305314));
#94239=CARTESIAN_POINT('Ctrl Pts',(-11.457271900044,24.4546863734907,3.36503555713485));
#94240=CARTESIAN_POINT('Ctrl Pts',(-11.4568067042835,24.4544119866951,3.36010355115903));
#94241=CARTESIAN_POINT('Ctrl Pts',(-11.454786693268,24.453276046025,3.33979105976632));
#94242=CARTESIAN_POINT('Ctrl Pts',(-11.45301332472,24.4524033307197,3.32443386932067));
#94243=CARTESIAN_POINT('Ctrl Pts',(-11.4372726914926,24.4455104654705,3.20478689737983));
#94244=CARTESIAN_POINT('Ctrl Pts',(-11.4123388201589,24.4390713827039,3.1022550533107));
#94245=CARTESIAN_POINT('Ctrl Pts',(-11.3449846918308,24.4271872177322,2.91558433975732));
#94246=CARTESIAN_POINT('Ctrl Pts',(-11.3050272236307,24.4217382590728,2.83109457089067));
#94247=CARTESIAN_POINT('Ctrl Pts',(-11.2513280475935,24.4159263074224,2.74095702639467));
#94248=CARTESIAN_POINT('Ctrl Pts',(-11.2452427554995,24.4152849220257,2.73101455840975));
#94249=CARTESIAN_POINT('Ctrl Pts',(-11.2357958904314,24.4143147562223,2.71598602823573));
#94250=CARTESIAN_POINT('Ctrl Pts',(-11.2325203480046,24.413982861006,2.71084666632516));
#94251=CARTESIAN_POINT('Ctrl Pts',(-11.2265071958815,24.4133816182688,2.70154073330227));
#94252=CARTESIAN_POINT('Ctrl Pts',(-11.2237802291797,24.4131118853662,2.69736742301124));
#94253=CARTESIAN_POINT('Ctrl Pts',(-11.2178497437404,24.4125315215079,2.6883919830812));
#94254=CARTESIAN_POINT('Ctrl Pts',(-11.2146390225884,24.4122211633616,2.68359469773532));
#94255=CARTESIAN_POINT('Ctrl Pts',(-11.2058552591927,24.4113823573186,2.67063699638782));
#94256=CARTESIAN_POINT('Ctrl Pts',(-11.2002277600222,24.4108559499104,2.66251374438105));
#94257=CARTESIAN_POINT('Ctrl Pts',(-11.1720840478895,24.4082758650757,2.62275488993514));
#94258=CARTESIAN_POINT('Ctrl Pts',(-11.1483962910001,24.4062670416568,2.59196569733561));
#94259=CARTESIAN_POINT('Ctrl Pts',(-11.0276800369282,24.3967041380207,2.44735147800674));
#94260=CARTESIAN_POINT('Ctrl Pts',(-10.914837715372,24.389823106038,2.34793342793114));
#94261=CARTESIAN_POINT('Ctrl Pts',(-10.7673264346335,24.3808406815148,2.2535253424028));
#94262=CARTESIAN_POINT('Ctrl Pts',(-10.7453848254409,24.3795022017801,2.24028168447792));
#94263=CARTESIAN_POINT('Ctrl Pts',(-10.7179926271854,24.3778143135933,2.2247143617253));
#94264=CARTESIAN_POINT('Ctrl Pts',(-10.7128595999059,24.377497304607,2.22183801481982));
#94265=CARTESIAN_POINT('Ctrl Pts',(-10.7048183975702,24.3769993595737,2.21739554588596));
#94266=CARTESIAN_POINT('Ctrl Pts',(-10.7019219710476,24.3768197329366,2.21580815086366));
#94267=CARTESIAN_POINT('Ctrl Pts',(-10.6965901436601,24.3764885345314,2.21290945444745));
#94268=CARTESIAN_POINT('Ctrl Pts',(-10.6941563844152,24.3763371483724,2.21159524435182));
#94269=CARTESIAN_POINT('Ctrl Pts',(-10.6886396813893,24.3759935244096,2.20863643840028));
#94270=CARTESIAN_POINT('Ctrl Pts',(-10.6855545926824,24.3758010341536,2.20699599422859));
#94271=CARTESIAN_POINT('Ctrl Pts',(-10.6762763603838,24.3752212208592,2.20210499046995));
#94272=CARTESIAN_POINT('Ctrl Pts',(-10.6700658506369,24.3748319032563,2.1988878129801));
#94273=CARTESIAN_POINT('Ctrl Pts',(-10.6027711116291,24.3706023302133,2.16463727998377));
#94274=CARTESIAN_POINT('Ctrl Pts',(-10.5396085436835,24.3665378906929,2.13788867564553));
#94275=CARTESIAN_POINT('Ctrl Pts',(-10.3797877727207,24.3563971630509,2.08307178870065));
#94276=CARTESIAN_POINT('Ctrl Pts',(-10.2816476108466,24.3503097343258,2.06034625668137));
#94277=CARTESIAN_POINT('Ctrl Pts',(-10.13907714812,24.3420031489043,2.04248273590023));
#94278=CARTESIAN_POINT('Ctrl Pts',(-10.0959865747642,24.3395568576619,2.03901192661985));
#94279=CARTESIAN_POINT('Ctrl Pts',(-10.0426126114907,24.336605972174,2.03708497243275));
#94280=CARTESIAN_POINT('Ctrl Pts',(-10.0324193070899,24.3360459231807,2.03682358942609));
#94281=CARTESIAN_POINT('Ctrl Pts',(-10.0163877176333,24.3351704674137,2.0365801143203));
#94282=CARTESIAN_POINT('Ctrl Pts',(-10.0105509813942,24.3348528510723,2.03652639338397));
#94283=CARTESIAN_POINT('Ctrl Pts',(-10.0002405443076,24.3342937225662,2.03649318268341));
#94284=CARTESIAN_POINT('Ctrl Pts',(-9.99576699208508,24.3340517670489,2.03649928443706));
#94285=CARTESIAN_POINT('Ctrl Pts',(-9.98550691261684,24.3334982885705,2.03656032367706));
#94286=CARTESIAN_POINT('Ctrl Pts',(-9.97972052119056,24.3331871974598,2.03662906962207));
#94287=CARTESIAN_POINT('Ctrl Pts',(-9.96368942687116,24.3323281668534,2.0369146334498));
#94288=CARTESIAN_POINT('Ctrl Pts',(-9.95344625330707,24.3317825018007,2.037204729516));
#94289=CARTESIAN_POINT('Ctrl Pts',(-9.89376184005028,24.3286206928419,2.03952261434719));
#94290=CARTESIAN_POINT('Ctrl Pts',(-9.84444344419266,24.3260801876343,2.04394932739963));
#94291=CARTESIAN_POINT('Ctrl Pts',(-9.67874424122476,24.3176762772866,2.06733942607496));
#94292=CARTESIAN_POINT('Ctrl Pts',(-9.5644742715828,24.3121353977366,2.097845719034));
#94293=CARTESIAN_POINT('Ctrl Pts',(-9.44582016518994,24.3057541781828,2.14544582514436));
#94294=CARTESIAN_POINT('Ctrl Pts',(-9.43657528336014,24.3052523614222,2.14926505749606));
#94295=CARTESIAN_POINT('Ctrl Pts',(-9.39416734121248,24.3029260398728,2.16729569182307));
#94296=CARTESIAN_POINT('Ctrl Pts',(-9.36150016062898,24.3010649588785,2.18263462332949));
#94297=CARTESIAN_POINT('Ctrl Pts',(-9.32416998150307,24.298819703213,2.2018778439513));
#94298=CARTESIAN_POINT('Ctrl Pts',(-9.31892087339443,24.2985011914166,2.20462416000015));
#94299=CARTESIAN_POINT('Ctrl Pts',(-9.31052036262235,24.2979867175908,2.20908445367893));
#94300=CARTESIAN_POINT('Ctrl Pts',(-9.30735828213727,24.29779197635,2.2107783091303));
#94301=CARTESIAN_POINT('Ctrl Pts',(-9.30174228573925,24.2974441155898,2.21381329707106));
#94302=CARTESIAN_POINT('Ctrl Pts',(-9.2992859500533,24.297291284266,2.21514985682126));
#94303=CARTESIAN_POINT('Ctrl Pts',(-9.29404143577756,24.2969634923553,2.21802305388046));
#94304=CARTESIAN_POINT('Ctrl Pts',(-9.291254480004,24.2967884078324,2.21956172649082));
#94305=CARTESIAN_POINT('Ctrl Pts',(-9.28362273490776,24.2963065488991,2.22380774727159));
#94306=CARTESIAN_POINT('Ctrl Pts',(-9.27878834276833,24.2959986355492,2.22653355155644));
#94307=CARTESIAN_POINT('Ctrl Pts',(-9.25295986205717,24.2943396628485,2.24129082328629));
#94308=CARTESIAN_POINT('Ctrl Pts',(-9.23225223680887,24.2929601906867,2.2538134205982));
#94309=CARTESIAN_POINT('Ctrl Pts',(-9.16917210382241,24.2886254431122,2.29412912856841));
#94310=CARTESIAN_POINT('Ctrl Pts',(-9.1279266467284,24.285601309655,2.32361273170463));
#94311=CARTESIAN_POINT('Ctrl Pts',(-8.98507538527094,24.2746257515227,2.43737503485389));
#94312=CARTESIAN_POINT('Ctrl Pts',(-8.89342298214994,24.2666729412143,2.53317828308894));
#94313=CARTESIAN_POINT('Ctrl Pts',(-8.80682578562209,24.2584564928517,2.65241312861247));
#94314=CARTESIAN_POINT('Ctrl Pts',(-8.79799500966825,24.2576074437074,2.66498368942001));
#94315=CARTESIAN_POINT('Ctrl Pts',(-8.78592761066472,24.2564308694675,2.68274980726382));
#94316=CARTESIAN_POINT('Ctrl Pts',(-8.78252338927163,24.2560970608161,2.687829852805));
#94317=CARTESIAN_POINT('Ctrl Pts',(-8.77634754064163,24.2554879234222,2.69717202738611));
#94318=CARTESIAN_POINT('Ctrl Pts',(-8.77356610215866,24.2552122314031,2.7014275298766));
#94319=CARTESIAN_POINT('Ctrl Pts',(-8.76797705494692,24.2546554577014,2.7100766506332));
#94320=CARTESIAN_POINT('Ctrl Pts',(-8.76517063793304,24.2543744226549,2.71447095371354));
#94321=CARTESIAN_POINT('Ctrl Pts',(-8.758308304691,24.2536835381748,2.72534368765688));
#94322=CARTESIAN_POINT('Ctrl Pts',(-8.75427951576073,24.2532746870019,2.73183911411364));
#94323=CARTESIAN_POINT('Ctrl Pts',(-8.73952950569231,24.2517653731785,2.75604110506058));
#94324=CARTESIAN_POINT('Ctrl Pts',(-8.72913313845304,24.2506766612723,2.77394340370713));
#94325=CARTESIAN_POINT('Ctrl Pts',(-8.66933680169356,24.244249431691,2.88213342220499));
#94326=CARTESIAN_POINT('Ctrl Pts',(-8.62919274718192,24.2392508083272,2.9772061041372));
#94327=CARTESIAN_POINT('Ctrl Pts',(-8.57393229098751,24.2299845664,3.15963009151653));
#94328=CARTESIAN_POINT('Ctrl Pts',(-8.55610762734898,24.2257268958965,3.24565384453934));
#94329=CARTESIAN_POINT('Ctrl Pts',(-8.54480362005008,24.2205090372751,3.34391594620524));
#94330=CARTESIAN_POINT('Ctrl Pts',(-8.54364716817559,24.2199097696098,3.35510296770986));
#94331=CARTESIAN_POINT('Ctrl Pts',(-8.54222167444811,24.2190688099773,3.37064160102376));
#94332=CARTESIAN_POINT('Ctrl Pts',(-8.54184294377679,24.2188329207025,3.37498304021043));
#94333=CARTESIAN_POINT('Ctrl Pts',(-8.54126679376097,24.2184529799122,3.38194663290108));
#94334=CARTESIAN_POINT('Ctrl Pts',(-8.54105703829013,24.2183096094216,3.38456777434806));
#94335=CARTESIAN_POINT('Ctrl Pts',(-8.54063314508165,24.2180089354005,3.39005061177839));
#94336=CARTESIAN_POINT('Ctrl Pts',(-8.54042035956009,24.2178515550498,3.39291238178762));
#94337=CARTESIAN_POINT('Ctrl Pts',(-8.53992402273555,24.2174682050402,3.39986409808154));
#94338=CARTESIAN_POINT('Ctrl Pts',(-8.53964923918421,24.2172417546554,3.40395463161733));
#94339=CARTESIAN_POINT('Ctrl Pts',(-8.53873799852227,24.2164374843061,3.41842892120816));
#94340=CARTESIAN_POINT('Ctrl Pts',(-8.53819509216671,24.2158547898865,3.42881800327112));
#94341=CARTESIAN_POINT('Ctrl Pts',(-8.53554173370634,24.2122453841602,3.49264340472883));
#94342=CARTESIAN_POINT('Ctrl Pts',(-8.53625101826255,24.2090932502014,3.54615220639344));
#94343=CARTESIAN_POINT('Ctrl Pts',(-8.54639665401212,24.2001726816885,3.69503926894906));
#94344=CARTESIAN_POINT('Ctrl Pts',(-8.5622701647745,24.1943433812652,3.78972124706008));
#94345=CARTESIAN_POINT('Ctrl Pts',(-8.59350079636938,24.1873406105241,3.90516603482704));
#94346=CARTESIAN_POINT('Ctrl Pts',(-8.6002809811674,24.185959421648,3.92800265788734));
#94347=CARTESIAN_POINT('Ctrl Pts',(-8.61852655509086,24.1825629590765,3.98437463994475));
#94348=CARTESIAN_POINT('Ctrl Pts',(-8.63065850041411,24.1805682148269,4.01767927569416));
#94349=CARTESIAN_POINT('Ctrl Pts',(-8.64762824433548,24.1780790606336,4.0594787953523));
#94350=CARTESIAN_POINT('Ctrl Pts',(-8.65135713281831,24.1775481172202,4.06840857759662));
#94351=CARTESIAN_POINT('Ctrl Pts',(-8.65740781018749,24.1767112338042,4.08250366445936));
#94352=CARTESIAN_POINT('Ctrl Pts',(-8.65967143679712,24.1764033464329,4.08769350104765));
#94353=CARTESIAN_POINT('Ctrl Pts',(-8.66396471900413,24.1758289588639,4.09738291026805));
#94354=CARTESIAN_POINT('Ctrl Pts',(-8.66598712543226,24.1755622181436,4.10188559117097));
#94355=CARTESIAN_POINT('Ctrl Pts',(-8.67059721555972,24.174962684309,4.11201209850057));
#94356=CARTESIAN_POINT('Ctrl Pts',(-8.67319788899172,24.1746303391109,4.11762993112479));
#94357=CARTESIAN_POINT('Ctrl Pts',(-8.68101397159529,24.1736485552074,4.13423659392936));
#94358=CARTESIAN_POINT('Ctrl Pts',(-8.68633088673907,24.1730025977637,4.14517724147775));
#94359=CARTESIAN_POINT('Ctrl Pts',(-8.7387012037998,24.1668418201424,4.24960776469685));
#94360=CARTESIAN_POINT('Ctrl Pts',(-8.79551960920961,24.1617043001886,4.33786437117493));
#94361=CARTESIAN_POINT('Ctrl Pts',(-8.92319594397368,24.1518175200531,4.49601335112564));
#94362=CARTESIAN_POINT('Ctrl Pts',(-8.99270107425714,24.147077589766,4.566252102984));
#94363=CARTESIAN_POINT('Ctrl Pts',(-9.0771029604954,24.1412999155452,4.63587466367133));
#94364=CARTESIAN_POINT('Ctrl Pts',(-9.08555719991905,24.1407208259081,4.64269179949379));
#94365=CARTESIAN_POINT('Ctrl Pts',(-9.09746296763309,24.1399035955974,4.65207536213955));
#94366=CARTESIAN_POINT('Ctrl Pts',(-9.1008513290916,24.1396708215779,4.65472178532317));
#94367=CARTESIAN_POINT('Ctrl Pts',(-9.10632434798996,24.1392944404083,4.658957700309));
#94368=CARTESIAN_POINT('Ctrl Pts',(-9.10840172747276,24.1391514874416,4.66055660883204));
#94369=CARTESIAN_POINT('Ctrl Pts',(-9.11277197244891,24.1388505365662,4.66390162096455));
#94370=CARTESIAN_POINT('Ctrl Pts',(-9.11506570633544,24.1386924553217,4.66564653802022));
#94371=CARTESIAN_POINT('Ctrl Pts',(-9.12068308571926,24.1383050344389,4.66989372269628));
#94372=CARTESIAN_POINT('Ctrl Pts',(-9.12401226370448,24.1380751905223,4.67238860585257));
#94373=CARTESIAN_POINT('Ctrl Pts',(-9.13601693227755,24.1372456891179,4.68130521534761));
#94374=CARTESIAN_POINT('Ctrl Pts',(-9.14475255003708,24.136640752458,4.68764495468732));
#94375=CARTESIAN_POINT('Ctrl Pts',(-9.20051276717484,24.1327752834402,4.72717785975241));
#94376=CARTESIAN_POINT('Ctrl Pts',(-9.24938739575732,24.1293705979757,4.75766643117006));
#94377=CARTESIAN_POINT('Ctrl Pts',(-9.33601776407901,24.1234610978858,4.80485595855693));
#94378=CARTESIAN_POINT('Ctrl Pts',(-9.37292259939883,24.1209793509464,4.82298729827759));
#94379=CARTESIAN_POINT('Ctrl Pts',(-9.49925217401818,24.1126819079522,4.87857801169276));
#94380=CARTESIAN_POINT('Ctrl Pts',(-9.59163321917607,24.1069560473513,4.90871133357948));
#94381=CARTESIAN_POINT('Ctrl Pts',(-9.70312365076309,24.1005696421488,4.93317562455307));
#94382=CARTESIAN_POINT('Ctrl Pts',(-9.71998373812841,24.0996167690119,4.93656495365636));
#94383=CARTESIAN_POINT('Ctrl Pts',(-9.74410159331199,24.0982715838354,4.94097253549342));
#94384=CARTESIAN_POINT('Ctrl Pts',(-9.7513128824114,24.0978716311227,4.94223457276102));
#94385=CARTESIAN_POINT('Ctrl Pts',(-9.76356474583563,24.0971958781554,4.94428412825072));
#94386=CARTESIAN_POINT('Ctrl Pts',(-9.76860047041574,24.0969192065697,4.94509948832378));
#94387=CARTESIAN_POINT('Ctrl Pts',(-9.77878198775772,24.0963619507379,4.9466934453799));
#94388=CARTESIAN_POINT('Ctrl Pts',(-9.78392787724483,24.096081404227,4.94747095742117));
#94389=CARTESIAN_POINT('Ctrl Pts',(-9.79657705425232,24.0953944361364,4.9493132118683));
#94390=CARTESIAN_POINT('Ctrl Pts',(-9.80408472081647,24.0949889836757,4.95034716094596));
#94391=CARTESIAN_POINT('Ctrl Pts',(-9.83164858846582,24.0935084963069,4.95392529526432));
#94392=CARTESIAN_POINT('Ctrl Pts',(-9.85174936899462,24.0924446048277,4.9561122089326));
#94393=CARTESIAN_POINT('Ctrl Pts',(-9.95793437632452,24.0868980389183,4.96544313863447));
#94394=CARTESIAN_POINT('Ctrl Pts',(-10.044482138714,24.082644767287,4.96537246235983));
#94395=CARTESIAN_POINT('Ctrl Pts',(-10.1498797483258,24.0774922705189,4.95593471421279));
#94396=CARTESIAN_POINT('Ctrl Pts',(-10.1691973472546,24.0765483659117,4.95381638818162));
#94397=CARTESIAN_POINT('Ctrl Pts',(-10.2730308924274,24.0714564070366,4.94033260691188));
#94398=CARTESIAN_POINT('Ctrl Pts',(-10.3564637043396,24.0673058268442,4.92198246495188));
#94399=CARTESIAN_POINT('Ctrl Pts',(-10.4485863038485,24.0622131318139,4.8931008714851));
#94400=CARTESIAN_POINT('Ctrl Pts',(-10.459319336881,24.0616115879296,4.88959902180716));
#94401=CARTESIAN_POINT('Ctrl Pts',(-10.4741464832155,24.0607678031505,4.88457084922579));
#94402=CARTESIAN_POINT('Ctrl Pts',(-10.4782761622519,24.0605314060915,4.88314975172676));
#94403=CARTESIAN_POINT('Ctrl Pts',(-10.4848852624666,24.0601507638355,4.88084230279655));
#94404=CARTESIAN_POINT('Ctrl Pts',(-10.4873687931607,24.0600072025104,4.87996769606254));
#94405=CARTESIAN_POINT('Ctrl Pts',(-10.4925529236495,24.059706406538,4.87812629877421));
#94406=CARTESIAN_POINT('Ctrl Pts',(-10.4952530469698,24.0595490964187,4.87715826867005));
#94407=CARTESIAN_POINT('Ctrl Pts',(-10.5018003738325,24.0591661149236,4.87478921978362));
#94408=CARTESIAN_POINT('Ctrl Pts',(-10.5056445650871,24.0589399647994,4.87337998637585));
#94409=CARTESIAN_POINT('Ctrl Pts',(-10.5187831568519,24.0581627485124,4.86850089963037));
#94410=CARTESIAN_POINT('Ctrl Pts',(-10.5280479532947,24.0576073261653,4.86495275528486));
#94411=CARTESIAN_POINT('Ctrl Pts',(-10.5507572792709,24.0562289917525,4.85598994606123));
#94412=CARTESIAN_POINT('Ctrl Pts',(-10.5641586127851,24.0554008757033,4.85046930531036));
#94413=CARTESIAN_POINT('Ctrl Pts',(-10.6168693683716,24.0520912107425,4.82783376687953));
#94414=CARTESIAN_POINT('Ctrl Pts',(-10.655498804781,24.0495494790711,4.80919486663624));
#94415=CARTESIAN_POINT('Ctrl Pts',(-10.7688477599786,24.0418433300742,4.74822810396001));
#94416=CARTESIAN_POINT('Ctrl Pts',(-10.8407253467814,24.036628656488,4.70099239909976));
#94417=CARTESIAN_POINT('Ctrl Pts',(-10.9572354004524,24.0278862082785,4.60881301122854));
#94418=CARTESIAN_POINT('Ctrl Pts',(-11.003873602144,24.0242881469058,4.56677331728973));
#94419=CARTESIAN_POINT('Ctrl Pts',(-11.0548360313142,24.0202470080194,4.51452372073893));
#94420=CARTESIAN_POINT('Ctrl Pts',(-11.0619197808835,24.0196825001892,4.50710665741033));
#94421=CARTESIAN_POINT('Ctrl Pts',(-11.0732984658576,24.0187709948098,4.49493901820026));
#94422=CARTESIAN_POINT('Ctrl Pts',(-11.0776411337006,24.0184219705346,4.49023372772759));
#94423=CARTESIAN_POINT('Ctrl Pts',(-11.0853200322576,24.0178026971717,4.48180328051215));
#94424=CARTESIAN_POINT('Ctrl Pts',(-11.0886682933413,24.0175319439779,4.47808926074207));
#94425=CARTESIAN_POINT('Ctrl Pts',(-11.0956868590616,24.0169628157268,4.47022330680425));
#94426=CARTESIAN_POINT('Ctrl Pts',(-11.0993527553319,24.0166646262469,4.46606753319355));
#94427=CARTESIAN_POINT('Ctrl Pts',(-11.106753876334,24.0160606630876,4.45758070939539));
#94428=CARTESIAN_POINT('Ctrl Pts',(-11.1104874958876,24.015754957724,4.45324838343436));
#94429=CARTESIAN_POINT('Ctrl Pts',(-11.1265352423983,24.0144363760583,4.43440505110665));
#94430=CARTESIAN_POINT('Ctrl Pts',(-11.138591369394,24.0134339348372,4.41967613295051));
#94431=CARTESIAN_POINT('Ctrl Pts',(-11.1878677699537,24.0092799168571,4.35702058804743));
#94432=CARTESIAN_POINT('Ctrl Pts',(-11.2223776735103,24.0062326820263,4.30703651282465));
#94433=CARTESIAN_POINT('Ctrl Pts',(-11.2797235512721,24.000756266381,4.21181928121408));
#94434=CARTESIAN_POINT('Ctrl Pts',(-11.3035067690404,23.9983122670245,4.16727001302749));
#94435=CARTESIAN_POINT('Ctrl Pts',(-11.3594137157013,23.991907013445,4.04810064909302));
#94436=CARTESIAN_POINT('Ctrl Pts',(-11.3877099373611,23.9879410339104,3.97188781795715));
#94437=CARTESIAN_POINT('Ctrl Pts',(-11.4125899330435,23.9830633151568,3.88281895045071));
#94438=CARTESIAN_POINT('Ctrl Pts',(-11.4155117208977,23.9824595620678,3.87186989673844));
#94439=CARTESIAN_POINT('Ctrl Pts',(-11.4193846037964,23.9816131622765,3.85664930879598));
#94440=CARTESIAN_POINT('Ctrl Pts',(-11.4204442065977,23.9813764072504,3.8524055020941));
#94441=CARTESIAN_POINT('Ctrl Pts',(-11.4221114316054,23.98099534016,3.84559841651867));
#94442=CARTESIAN_POINT('Ctrl Pts',(-11.4227311937402,23.9808517148989,3.84303810216134));
#94443=CARTESIAN_POINT('Ctrl Pts',(-11.4240111943254,23.9805508974935,3.83768712177561));
#94444=CARTESIAN_POINT('Ctrl Pts',(-11.4246701443856,23.9803936305015,3.8348961824285));
#94445=CARTESIAN_POINT('Ctrl Pts',(-11.426248803378,23.9800109855722,3.82812089530692));
#94446=CARTESIAN_POINT('Ctrl Pts',(-11.4271600213203,23.979785131083,3.82413460751766));
#94447=CARTESIAN_POINT('Ctrl Pts',(-11.4290684616233,23.9793013466763,3.81562171441978));
#94448=CARTESIAN_POINT('Ctrl Pts',(-11.4300609069921,23.9790431640214,3.81109409470195));
#94449=CARTESIAN_POINT('Ctrl Pts',(-11.4348169732641,23.9777731107869,3.78889276379791));
#94450=CARTESIAN_POINT('Ctrl Pts',(-11.4382743937767,23.9767459190681,3.77115583004349));
#94451=CARTESIAN_POINT('Ctrl Pts',(-11.45603124916,23.970841939527,3.67013457373519));
#94452=CARTESIAN_POINT('Ctrl Pts',(-11.4634233187998,23.9657175935564,3.585805604991));
#94453=CARTESIAN_POINT('Ctrl Pts',(-11.4634994065207,23.9606357315493,3.50131799604382));
#94454=CARTESIAN_POINT('Ctrl Pts',(-11.4634994065687,23.9606357283428,3.50131794273411));
#94455=CARTESIAN_POINT('Ctrl Pts',(-11.4634998021939,23.9606093036564,3.50087862372563));
#94456=CARTESIAN_POINT('Ctrl Pts',(-11.4635,23.9605828803629,3.50043930947062));
#94457=CARTESIAN_POINT('Ctrl Pts',(-11.4635,23.9605564584951,3.50000000010085));
#94458=CARTESIAN_POINT('Ctrl Pts',(-11.4635,23.8891760003868,3.49999987117833));
#94459=CARTESIAN_POINT('Ctrl Pts',(-11.4635000043558,23.8915819689193,3.54948511583872));
#94460=CARTESIAN_POINT('Ctrl Pts',(-11.4609901519458,23.8939896094975,3.59896532125907));
#94461=CARTESIAN_POINT('Ctrl Pts',(-11.454965132913,23.8969582981221,3.65813760143904));
#94462=CARTESIAN_POINT('Ctrl Pts',(-11.4538576145332,23.8974569041636,3.66801508877796));
#94463=CARTESIAN_POINT('Ctrl Pts',(-11.4482522193293,23.8997847642009,3.7137912154954));
#94464=CARTESIAN_POINT('Ctrl Pts',(-11.442525069736,23.9016507411869,3.74952393081664));
#94465=CARTESIAN_POINT('Ctrl Pts',(-11.4343256065951,23.9039015782604,3.79082207375434));
#94466=CARTESIAN_POINT('Ctrl Pts',(-11.4331353011141,23.9042204339671,3.79663214700676));
#94467=CARTESIAN_POINT('Ctrl Pts',(-11.4311678069335,23.9047354126907,3.80594745979007));
#94468=CARTESIAN_POINT('Ctrl Pts',(-11.4304129643129,23.9049303121381,3.8094574134188));
#94469=CARTESIAN_POINT('Ctrl Pts',(-11.4290467030395,23.9052784558143,3.81569859669613));
#94470=CARTESIAN_POINT('Ctrl Pts',(-11.4284403564398,23.9054314114728,3.81843088954174));
#94471=CARTESIAN_POINT('Ctrl Pts',(-11.4271267564389,23.9057595222497,3.82427091895385));
#94472=CARTESIAN_POINT('Ctrl Pts',(-11.4264171990844,23.9059348017707,3.82737804077043));
#94473=CARTESIAN_POINT('Ctrl Pts',(-11.4244429828954,23.9064171559432,3.83589477806128));
#94474=CARTESIAN_POINT('Ctrl Pts',(-11.4231576752806,23.9067253707084,3.84129949122094));
#94475=CARTESIAN_POINT('Ctrl Pts',(-11.4161059862807,23.908385427406,3.8702192533847));
#94476=CARTESIAN_POINT('Ctrl Pts',(-11.4097878121441,23.9097656892219,3.89359451711435));
#94477=CARTESIAN_POINT('Ctrl Pts',(-11.3884550623496,23.9141027294769,3.96539756220762));
#94478=CARTESIAN_POINT('Ctrl Pts',(-11.3715023840858,23.917128355793,4.0132084843924));
#94479=CARTESIAN_POINT('Ctrl Pts',(-11.3016412266426,23.9280998971019,4.1818742059472));
#94480=CARTESIAN_POINT('Ctrl Pts',(-11.2349300001728,23.9360468914732,4.29635626870393));
#94481=CARTESIAN_POINT('Ctrl Pts',(-11.1443122588589,23.944259725814,4.41247909054203));
#94482=CARTESIAN_POINT('Ctrl Pts',(-11.1346628484518,23.9451095583647,4.42445058394195));
#94483=CARTESIAN_POINT('Ctrl Pts',(-11.1209098110972,23.9462872948732,4.44097339168951));
#94484=CARTESIAN_POINT('Ctrl Pts',(-11.1169637816443,23.9466214869798,4.44565408082026));
#94485=CARTESIAN_POINT('Ctrl Pts',(-11.1096832255637,23.9472313570204,4.45418095681914));
#94486=CARTESIAN_POINT('Ctrl Pts',(-11.1063577942191,23.9475073984856,4.45803475486801));
#94487=CARTESIAN_POINT('Ctrl Pts',(-11.0995807757439,23.9480649138154,4.46580620599107));
#94488=CARTESIAN_POINT('Ctrl Pts',(-11.0961281933649,23.9483463407409,4.46972289578022));
#94489=CARTESIAN_POINT('Ctrl Pts',(-11.0875620169128,23.9490382602046,4.47933636172204));
#94490=CARTESIAN_POINT('Ctrl Pts',(-11.0824245125678,23.9494477520653,4.48501168908409));
#94491=CARTESIAN_POINT('Ctrl Pts',(-11.0632030982987,23.9509599390239,4.50591331926932));
#94492=CARTESIAN_POINT('Ctrl Pts',(-11.048840166506,23.952050846162,4.5208804023639));
#94493=CARTESIAN_POINT('Ctrl Pts',(-10.9618375290716,23.9584439026487,4.6077675841196));
#94494=CARTESIAN_POINT('Ctrl Pts',(-10.8821434031152,23.9634118528417,4.6722225832342));
#94495=CARTESIAN_POINT('Ctrl Pts',(-10.7223357933823,23.9726730174311,4.77587277489688));
#94496=CARTESIAN_POINT('Ctrl Pts',(-10.644112044499,23.9769565313717,4.81709389213275));
#94497=CARTESIAN_POINT('Ctrl Pts',(-10.5522968611014,23.9822037846373,4.8553326346104));
#94498=CARTESIAN_POINT('Ctrl Pts',(-10.5418805347667,23.9828022238575,4.85953074404555));
#94499=CARTESIAN_POINT('Ctrl Pts',(-10.5273559775163,23.9836423778154,4.86519116680553));
#94500=CARTESIAN_POINT('Ctrl Pts',(-10.5232877110615,23.9838783160043,4.86675572777747));
#94501=CARTESIAN_POINT('Ctrl Pts',(-10.5167516378089,23.9842584492258,4.86923589020384));
#94502=CARTESIAN_POINT('Ctrl Pts',(-10.5142882119134,23.984401964313,4.87016306075622));
#94503=CARTESIAN_POINT('Ctrl Pts',(-10.5091321143925,23.984702885859,4.87208782000409));
#94504=CARTESIAN_POINT('Ctrl Pts',(-10.5064390018102,23.9848603690552,4.87308413168626));
#94505=CARTESIAN_POINT('Ctrl Pts',(-10.4998883050112,23.9852441455079,4.87548565542237));
#94506=CARTESIAN_POINT('Ctrl Pts',(-10.4960277188141,23.9854709215557,4.87688256837301));
#94507=CARTESIAN_POINT('Ctrl Pts',(-10.4823320277322,23.9862774204521,4.88177313634685));
#94508=CARTESIAN_POINT('Ctrl Pts',(-10.4724657188922,23.9868620527773,4.88517772037454));
#94509=CARTESIAN_POINT('Ctrl Pts',(-10.4115053612533,23.9904928858565,4.90548636617494));
#94510=CARTESIAN_POINT('Ctrl Pts',(-10.3595514995227,23.9936660389887,4.91966554760186));
#94511=CARTESIAN_POINT('Ctrl Pts',(-10.2157773343699,24.0024576494598,4.95050523950782));
#94512=CARTESIAN_POINT('Ctrl Pts',(-10.1229461244701,24.0081311254835,4.9613048076366));
#94513=CARTESIAN_POINT('Ctrl Pts',(-9.97114050030912,24.0170366965516,4.96438793015942));
#94514=CARTESIAN_POINT('Ctrl Pts',(-9.91254056453779,24.0203889666485,4.96205918234024));
#94515=CARTESIAN_POINT('Ctrl Pts',(-9.84415403662922,24.0241932452024,4.95521368491433));
#94516=CARTESIAN_POINT('Ctrl Pts',(-9.83408664419578,24.0247506209567,4.95410027119156));
#94517=CARTESIAN_POINT('Ctrl Pts',(-9.81771171283066,24.0256530103098,4.95211699087268));
#94518=CARTESIAN_POINT('Ctrl Pts',(-9.81139697945031,24.0259999832322,4.95131033113232));
#94519=CARTESIAN_POINT('Ctrl Pts',(-9.80013404194938,24.0266170737867,4.94979682371275));
#94520=CARTESIAN_POINT('Ctrl Pts',(-9.79518384500367,24.0268876812026,4.94910578452636));
#94521=CARTESIAN_POINT('Ctrl Pts',(-9.78472832007381,24.0274579845106,4.94759156483295));
#94522=CARTESIAN_POINT('Ctrl Pts',(-9.77922394339953,24.0277574853152,4.94676230555027));
#94523=CARTESIAN_POINT('Ctrl Pts',(-9.76459060859419,24.0285518061867,4.94447226949521));
#94524=CARTESIAN_POINT('Ctrl Pts',(-9.75547045132066,24.0290448910683,4.94295634861191));
#94525=CARTESIAN_POINT('Ctrl Pts',(-9.71178536894021,24.0313979281198,4.93526909089378));
#94526=CARTESIAN_POINT('Ctrl Pts',(-9.67743423820888,24.033221279083,4.92794139350722));
#94527=CARTESIAN_POINT('Ctrl Pts',(-9.58004944210803,24.0383435634105,4.90347335450942));
#94528=CARTESIAN_POINT('Ctrl Pts',(-9.51785385010775,24.0415546649996,4.88334083163357));
#94529=CARTESIAN_POINT('Ctrl Pts',(-9.35586305284131,24.0500539680569,4.81864658826274));
#94530=CARTESIAN_POINT('Ctrl Pts',(-9.25937683698116,24.055251907348,4.76696965515162));
#94531=CARTESIAN_POINT('Ctrl Pts',(-9.16126827220221,24.0615564492934,4.69935913982343));
#94532=CARTESIAN_POINT('Ctrl Pts',(-9.15305197798639,24.0620930970591,4.69357123558492));
#94533=CARTESIAN_POINT('Ctrl Pts',(-9.14185345554479,24.0628374597779,4.68550867367234));
#94534=CARTESIAN_POINT('Ctrl Pts',(-9.13881919998386,24.0630404663896,4.6833063576978));
#94535=CARTESIAN_POINT('Ctrl Pts',(-9.13364684044202,24.0633888478916,4.6795217369945));
#94536=CARTESIAN_POINT('Ctrl Pts',(-9.13150451014229,24.0635338299707,4.67794520627324));
#94537=CARTESIAN_POINT('Ctrl Pts',(-9.1270755372757,24.0638350122379,4.67466729581145));
#94538=CARTESIAN_POINT('Ctrl Pts',(-9.12478956608063,24.0639912738644,4.67296507592236));
#94539=CARTESIAN_POINT('Ctrl Pts',(-9.11931538344049,24.0643673918053,4.66886388262));
#94540=CARTESIAN_POINT('Ctrl Pts',(-9.11613199115101,24.0645876857661,4.66645853423958));
#94541=CARTESIAN_POINT('Ctrl Pts',(-9.10523038183066,24.06534738344,4.65815110679264));
#94542=CARTESIAN_POINT('Ctrl Pts',(-9.09756129863414,24.0658909861196,4.65218533043863));
#94543=CARTESIAN_POINT('Ctrl Pts',(-9.05334967454546,24.069075678057,4.61708093750482));
#94544=CARTESIAN_POINT('Ctrl Pts',(-9.01816315329134,24.0718137525028,4.58628371677107));
#94545=CARTESIAN_POINT('Ctrl Pts',(-8.88425962363714,24.0828799742192,4.45725581302095));
#94546=CARTESIAN_POINT('Ctrl Pts',(-8.79827916926299,24.0914052414053,4.3468149000219));
#94547=CARTESIAN_POINT('Ctrl Pts',(-8.71648020514208,24.1007454651063,4.20361005832185));
#94548=CARTESIAN_POINT('Ctrl Pts',(-8.70434521070886,24.1021782090747,4.18100584561681));
#94549=CARTESIAN_POINT('Ctrl Pts',(-8.68894412817977,24.1040634358401,4.15041422529998));
#94550=CARTESIAN_POINT('Ctrl Pts',(-8.68514585918608,24.1045343071191,4.14270114074868));
#94551=CARTESIAN_POINT('Ctrl Pts',(-8.67906257946168,24.1052983974281,4.13006824853465));
#94552=CARTESIAN_POINT('Ctrl Pts',(-8.67673660075418,24.1055930238141,4.12516849257649));
#94553=CARTESIAN_POINT('Ctrl Pts',(-8.67230296855575,24.1061594829812,4.11569328226447));
#94554=CARTESIAN_POINT('Ctrl Pts',(-8.6701915979154,24.1064314402393,4.11111966074841));
#94555=CARTESIAN_POINT('Ctrl Pts',(-8.66534427996868,24.10706101034,4.10047539121013));
#94556=CARTESIAN_POINT('Ctrl Pts',(-8.66262605257737,24.1074180159052,4.09439676413424));
#94557=CARTESIAN_POINT('Ctrl Pts',(-8.65408769492063,24.10855240534,4.07494778093965));
#94558=CARTESIAN_POINT('Ctrl Pts',(-8.64842576462139,24.1093244479378,4.06150867335387));
#94559=CARTESIAN_POINT('Ctrl Pts',(-8.62098454719638,24.1131723669102,3.9935532502429));
#94560=CARTESIAN_POINT('Ctrl Pts',(-8.60229746581209,24.1161446284507,3.93784361434993));
#94561=CARTESIAN_POINT('Ctrl Pts',(-8.57043543326116,24.1222073100312,3.81972742493916));
#94562=CARTESIAN_POINT('Ctrl Pts',(-8.55788797834093,24.1252800684441,3.75728116641249));
#94563=CARTESIAN_POINT('Ctrl Pts',(-8.53844088193275,24.1324185784115,3.61203563974093));
#94564=CARTESIAN_POINT('Ctrl Pts',(-8.53444277571061,24.1364895465003,3.52907818508724));
#94565=CARTESIAN_POINT('Ctrl Pts',(-8.53774861244331,24.141292827249,3.43914295336232));
#94566=CARTESIAN_POINT('Ctrl Pts',(-8.53806118792228,24.1416744833725,3.4320470294758));
#94567=CARTESIAN_POINT('Ctrl Pts',(-8.53860558341159,24.1422491064967,3.42144456474463));
#94568=CARTESIAN_POINT('Ctrl Pts',(-8.53879840540502,24.142439974825,3.41793602087497));
#94569=CARTESIAN_POINT('Ctrl Pts',(-8.53916678214476,24.1427834618995,3.41164659765739));
#94570=CARTESIAN_POINT('Ctrl Pts',(-8.53933764484853,24.1429358188396,3.40886549411152));
#94571=CARTESIAN_POINT('Ctrl Pts',(-8.53972696334491,24.1432685303449,3.40281116426846));
#94572=CARTESIAN_POINT('Ctrl Pts',(-8.53994847960029,24.1434490480574,3.39953822261322));
#94573=CARTESIAN_POINT('Ctrl Pts',(-8.54060515491769,24.1439605411897,3.39029701038639));
#94574=CARTESIAN_POINT('Ctrl Pts',(-8.54106591327014,24.1442928905258,3.38433069622246));
#94575=CARTESIAN_POINT('Ctrl Pts',(-8.54416354205071,24.1463743617964,3.34718852607133));
#94576=CARTESIAN_POINT('Ctrl Pts',(-8.54776282814729,24.1481711479144,3.31610315316027));
#94577=CARTESIAN_POINT('Ctrl Pts',(-8.57659269711208,24.1596470917269,3.12184091109836));
#94578=CARTESIAN_POINT('Ctrl Pts',(-8.62829057149899,24.1699090742136,2.96378307721295));
#94579=CARTESIAN_POINT('Ctrl Pts',(-8.71561776615167,24.1804657712711,2.79808543613992));
#94580=CARTESIAN_POINT('Ctrl Pts',(-8.72637634017,24.1816977525921,2.77874787629847));
#94581=CARTESIAN_POINT('Ctrl Pts',(-8.74167286457121,24.1833602264146,2.75266415780829));
#94582=CARTESIAN_POINT('Ctrl Pts',(-8.7458341961306,24.1838040745777,2.74570153062397));
#94583=CARTESIAN_POINT('Ctrl Pts',(-8.75254242356152,24.1845064618376,2.73468650437593));
#94584=CARTESIAN_POINT('Ctrl Pts',(-8.75505164279409,24.1847663593352,2.73061145040577));
#94585=CARTESIAN_POINT('Ctrl Pts',(-8.76023678109076,24.1852976901061,2.7222823990478));
#94586=CARTESIAN_POINT('Ctrl Pts',(-8.76291471622812,24.1855690449882,2.71802972733174));
#94587=CARTESIAN_POINT('Ctrl Pts',(-8.76915106414651,24.186194007994,2.7082383661729));
#94588=CARTESIAN_POINT('Ctrl Pts',(-8.77272506422185,24.1865470367011,2.70270970052696));
#94589=CARTESIAN_POINT('Ctrl Pts',(-8.78411423913461,24.1876561490568,2.68534969598379));
#94590=CARTESIAN_POINT('Ctrl Pts',(-8.79206424598193,24.1884072258325,2.67360751812575));
#94591=CARTESIAN_POINT('Ctrl Pts',(-8.83206576341668,24.1920776431233,2.61633608360049));
#94592=CARTESIAN_POINT('Ctrl Pts',(-8.86652819296479,24.1949042775574,2.57254390015054));
#94593=CARTESIAN_POINT('Ctrl Pts',(-8.96924678168534,24.2026118408871,2.45632140151088));
#94594=CARTESIAN_POINT('Ctrl Pts',(-9.04250469611667,24.2073288303338,2.38873098545572));
#94595=CARTESIAN_POINT('Ctrl Pts',(-9.13733880729182,24.2132134470591,2.31762389010589));
#94596=CARTESIAN_POINT('Ctrl Pts',(-9.15285428723863,24.2141705663057,2.30645833720846));
#94597=CARTESIAN_POINT('Ctrl Pts',(-9.19557149855446,24.216802894614,2.27696996354199));
#94598=CARTESIAN_POINT('Ctrl Pts',(-9.22317611115832,24.2185009123705,2.25925344294719));
#94599=CARTESIAN_POINT('Ctrl Pts',(-9.25630393470123,24.220563178437,2.23953117916682));
#94600=CARTESIAN_POINT('Ctrl Pts',(-9.26127488604484,24.2208732621228,2.23661142570786));
#94601=CARTESIAN_POINT('Ctrl Pts',(-9.26935953778213,24.2213788110988,2.23192682626655));
#94602=CARTESIAN_POINT('Ctrl Pts',(-9.27246273751292,24.2215731529596,2.23014387031086));
#94603=CARTESIAN_POINT('Ctrl Pts',(-9.27799772085976,24.2219203642975,2.22699067166411));
#94604=CARTESIAN_POINT('Ctrl Pts',(-9.28042691682931,24.2220729472378,2.22561598450397));
#94605=CARTESIAN_POINT('Ctrl Pts',(-9.28567806447831,24.2224032256298,2.22266415033212));
#94606=CARTESIAN_POINT('Ctrl Pts',(-9.28850127220543,24.2225810647352,2.22108942441484));
#94607=CARTESIAN_POINT('Ctrl Pts',(-9.29637271343978,24.2230775994293,2.21673303085421));
#94608=CARTESIAN_POINT('Ctrl Pts',(-9.30143214036592,24.2233975465664,2.21397184489734));
#94609=CARTESIAN_POINT('Ctrl Pts',(-9.33061411064113,24.2252469250134,2.19826877890294));
#94610=CARTESIAN_POINT('Ctrl Pts',(-9.35507824488235,24.2268127916465,2.18597664682072));
#94611=CARTESIAN_POINT('Ctrl Pts',(-9.43634063407504,24.2320298106247,2.14796189524942));
#94612=CARTESIAN_POINT('Ctrl Pts',(-9.4944377235781,24.2357815247438,2.12518186690262));
#94613=CARTESIAN_POINT('Ctrl Pts',(-9.66262407252432,24.2464168834666,2.07134173351853));
#94614=CARTESIAN_POINT('Ctrl Pts',(-9.77516549909753,24.253236527815,2.04936395433782));
#94615=CARTESIAN_POINT('Ctrl Pts',(-9.90579240787828,24.2605606953189,2.03943970870383));
#94616=CARTESIAN_POINT('Ctrl Pts',(-9.92247413307491,24.2614861236123,2.03845930354126));
#94617=CARTESIAN_POINT('Ctrl Pts',(-9.94567707607168,24.2627599950842,2.03749403698348));
#94618=CARTESIAN_POINT('Ctrl Pts',(-9.95218646548796,24.2631159162833,2.03726675714144));
#94619=CARTESIAN_POINT('Ctrl Pts',(-9.96342005339138,24.2637276920648,2.03694959746934));
#94620=CARTESIAN_POINT('Ctrl Pts',(-9.96814353255016,24.2639841818322,2.03683912741972));
#94621=CARTESIAN_POINT('Ctrl Pts',(-9.97792469824924,24.2645137863734,2.03665775873468));
#94622=CARTESIAN_POINT('Ctrl Pts',(-9.98298238882209,24.2647867939368,2.03659020236446));
#94623=CARTESIAN_POINT('Ctrl Pts',(-9.99483158797663,24.2654244666349,2.03649336823946));
#94624=CARTESIAN_POINT('Ctrl Pts',(-10.0016231836129,24.2657884742982,2.03648514148917));
#94625=CARTESIAN_POINT('Ctrl Pts',(-10.0237317577064,24.2669687468812,2.03661226101212));
#94626=CARTESIAN_POINT('Ctrl Pts',(-10.0390468783546,24.26777903056,2.03694079559391));
#94627=CARTESIAN_POINT('Ctrl Pts',(-10.1187939961307,24.2719638076596,2.03990464969452));
#94628=CARTESIAN_POINT('Ctrl Pts',(-10.1830081084489,24.2752119929112,2.04655592005852));
#94629=CARTESIAN_POINT('Ctrl Pts',(-10.3459562420196,24.283365672833,2.07440861991993));
#94630=CARTESIAN_POINT('Ctrl Pts',(-10.4433046342135,24.2881416834927,2.10161688655205));
#94631=CARTESIAN_POINT('Ctrl Pts',(-10.5737851052799,24.2951921807279,2.15309243147087));
#94632=CARTESIAN_POINT('Ctrl Pts',(-10.6098883229884,24.2972198620835,2.16905106551062));
#94633=CARTESIAN_POINT('Ctrl Pts',(-10.6507414859031,24.2996519994487,2.18912070331917));
#94634=CARTESIAN_POINT('Ctrl Pts',(-10.6561666690914,24.2999778574005,2.19182787379549));
#94635=CARTESIAN_POINT('Ctrl Pts',(-10.6648121346717,24.3005019954083,2.19620927761201));
#94636=CARTESIAN_POINT('Ctrl Pts',(-10.6680433400714,24.3006989819193,2.19786194380169));
#94637=CARTESIAN_POINT('Ctrl Pts',(-10.6737603865028,24.301049512546,2.20081292471903));
#94638=CARTESIAN_POINT('Ctrl Pts',(-10.6762486824796,24.3012027540169,2.20210638558195));
#94639=CARTESIAN_POINT('Ctrl Pts',(-10.6815383521137,24.3015299783493,2.20487539243755));
#94640=CARTESIAN_POINT('Ctrl Pts',(-10.6843386154339,24.3017040761191,2.20635285585708));
#94641=CARTESIAN_POINT('Ctrl Pts',(-10.6919498824239,24.3021796113312,2.21040030980002));
#94642=CARTESIAN_POINT('Ctrl Pts',(-10.6967512982756,24.3024821352524,2.21298810138433));
#94643=CARTESIAN_POINT('Ctrl Pts',(-10.7215497981068,24.3040573799705,2.2265330461306));
#94644=CARTESIAN_POINT('Ctrl Pts',(-10.7413022399097,24.3053552391435,2.23792905749997));
#94645=CARTESIAN_POINT('Ctrl Pts',(-10.800114713254,24.3093331385733,2.27371743768528));
#94646=CARTESIAN_POINT('Ctrl Pts',(-10.838296354194,24.3120705094797,2.29949544585657));
#94647=CARTESIAN_POINT('Ctrl Pts',(-10.9203214607578,24.3182083765269,2.36069736831385));
#94648=CARTESIAN_POINT('Ctrl Pts',(-10.963466415326,24.3216147741097,2.39694301047749));
#94649=CARTESIAN_POINT('Ctrl Pts',(-11.0676288404337,24.3301696541822,2.49523392344514));
#94650=CARTESIAN_POINT('Ctrl Pts',(-11.1254101041338,24.3352320369628,2.56040305350164));
#94651=CARTESIAN_POINT('Ctrl Pts',(-11.1834477853916,24.3406449373588,2.63895487391698));
#94652=CARTESIAN_POINT('Ctrl Pts',(-11.1897286762487,24.3412359419211,2.64765438029548));
#94653=CARTESIAN_POINT('Ctrl Pts',(-11.1996468852343,24.3421778555164,2.66171511242194));
#94654=CARTESIAN_POINT('Ctrl Pts',(-11.2033451840857,24.34253107365,2.6670326706173));
#94655=CARTESIAN_POINT('Ctrl Pts',(-11.209851741543,24.3431561397246,2.67652182862578));
#94656=CARTESIAN_POINT('Ctrl Pts',(-11.2126740130567,24.3434285128493,2.6806836543938));
#94657=CARTESIAN_POINT('Ctrl Pts',(-11.2185146019752,24.3439948312592,2.68939269638869));
#94658=CARTESIAN_POINT('Ctrl Pts',(-11.2215290496094,24.3442886293374,2.6939424226746));
#94659=CARTESIAN_POINT('Ctrl Pts',(-11.2293075815342,24.34505077525,2.7058264635067));
#94660=CARTESIAN_POINT('Ctrl Pts',(-11.2340315377667,24.3455176353648,2.71318686821153));
#94661=CARTESIAN_POINT('Ctrl Pts',(-11.2545380122506,24.3475626325797,2.74577706758983));
#94662=CARTESIAN_POINT('Ctrl Pts',(-11.2696154141204,24.3491150417504,2.77144340170441));
#94663=CARTESIAN_POINT('Ctrl Pts',(-11.3082691557988,24.3532506396542,2.84209292728556));
#94664=CARTESIAN_POINT('Ctrl Pts',(-11.330304786355,24.3557839091709,2.88787288368527));
#94665=CARTESIAN_POINT('Ctrl Pts',(-11.3742182370262,24.3613737546387,2.99273820878371));
#94666=CARTESIAN_POINT('Ctrl Pts',(-11.3947516290647,24.3644038546213,3.05227446720345));
#94667=CARTESIAN_POINT('Ctrl Pts',(-11.430270734794,24.3709744280178,3.18179504891252));
#94668=CARTESIAN_POINT('Ctrl Pts',(-11.4440861921214,24.3745205271197,3.25192454721184));
#94669=CARTESIAN_POINT('Ctrl Pts',(-11.4536091432229,24.3787155573626,3.32998385639406));
#94670=CARTESIAN_POINT('Ctrl Pts',(-11.4544351961251,24.3791057884411,3.33720170065257));
#94671=CARTESIAN_POINT('Ctrl Pts',(-11.4555844503232,24.3796908348662,3.34795153787764));
#94672=CARTESIAN_POINT('Ctrl Pts',(-11.4559486198101,24.3798834382273,3.35147915032443));
#94673=CARTESIAN_POINT('Ctrl Pts',(-11.4565761616007,24.3802287331405,3.35778218200639));
#94674=CARTESIAN_POINT('Ctrl Pts',(-11.4568444289099,24.3803811502182,3.36055706502625));
#94675=CARTESIAN_POINT('Ctrl Pts',(-11.4574085595371,24.3807124022988,3.36657165432544));
#94676=CARTESIAN_POINT('Ctrl Pts',(-11.4577015458659,24.380891389665,3.36981153816001));
#94677=CARTESIAN_POINT('Ctrl Pts',(-11.4584925903416,24.3813947887294,3.37889662065334));
#94678=CARTESIAN_POINT('Ctrl Pts',(-11.4589663027267,24.3817205102055,3.38474380843458));
#94679=CARTESIAN_POINT('Ctrl Pts',(-11.4615862143736,24.3836769998825,3.4196915918393));
#94680=CARTESIAN_POINT('Ctrl Pts',(-11.4628967067121,24.3853492480198,3.44884638998033));
#94681=CARTESIAN_POINT('Ctrl Pts',(-11.4634449961681,24.3874770446995,3.48534702905904));
#94682=CARTESIAN_POINT('Ctrl Pts',(-11.4634999998891,24.3879059175572,3.49267432048072));
#94683=CARTESIAN_POINT('Ctrl Pts',(-11.4635,24.3883362350912,3.49999997785042));
#94684=CARTESIAN_POINT('Origin',(-10.,12.3756328852638,3.5));
#94685=CARTESIAN_POINT('',(-9.8111040185181,13.5868901459558,2.33749693734598));
#94686=CARTESIAN_POINT('',(-9.81117889814932,13.4873563446704,2.33776762587097));
#94687=CARTESIAN_POINT('',(-9.81110406371068,12.3756328852638,2.3374969300026));
#94688=CARTESIAN_POINT('',(-10.6730394577908,13.3,4.4664951892051));
#94689=CARTESIAN_POINT('Ctrl Pts',(-9.81110401834328,13.5868901487969,2.33749693737438));
#94690=CARTESIAN_POINT('Ctrl Pts',(-9.75202396300196,13.5831615610686,2.34709689922293));
#94691=CARTESIAN_POINT('Ctrl Pts',(-9.69374318778665,13.5793739864102,2.36118950009534));
#94692=CARTESIAN_POINT('Ctrl Pts',(-9.6273910635311,13.5747909607468,2.38270201310816));
#94693=CARTESIAN_POINT('Ctrl Pts',(-9.61805390999522,13.574139754937,2.38585935099278));
#94694=CARTESIAN_POINT('Ctrl Pts',(-9.6028328166057,13.5730673097639,2.39122015273536));
#94695=CARTESIAN_POINT('Ctrl Pts',(-9.59692481154355,13.5726483364488,2.39335420700961));
#94696=CARTESIAN_POINT('Ctrl Pts',(-9.58634487173694,13.5718930353134,2.39727179106359));
#94697=CARTESIAN_POINT('Ctrl Pts',(-9.58166665712947,13.5715572843994,2.39903802025425));
#94698=CARTESIAN_POINT('Ctrl Pts',(-9.57172488705031,13.5708399155358,2.4028639843681));
#94699=CARTESIAN_POINT('Ctrl Pts',(-9.56646464369583,13.5704580324315,2.40493191897584));
#94700=CARTESIAN_POINT('Ctrl Pts',(-9.55229253621004,13.5694227689886,2.41062145000483));
#94701=CARTESIAN_POINT('Ctrl Pts',(-9.5434099862231,13.5687670234742,2.41431443405679));
#94702=CARTESIAN_POINT('Ctrl Pts',(-9.49659002895795,13.5652730934424,2.43445635749211));
#94703=CARTESIAN_POINT('Ctrl Pts',(-9.45949754686497,13.5623721214329,2.45278405541126));
#94704=CARTESIAN_POINT('Ctrl Pts',(-9.33134228688243,13.5518619026643,2.52473111418173));
#94705=CARTESIAN_POINT('Ctrl Pts',(-9.24662356770226,13.5439427472883,2.58858756243152));
#94706=CARTESIAN_POINT('Ctrl Pts',(-9.15592205131426,13.5348136678083,2.67834839759684));
#94707=CARTESIAN_POINT('Ctrl Pts',(-9.14072211083367,13.5332598207255,2.69425773317486));
#94708=CARTESIAN_POINT('Ctrl Pts',(-9.12226871724548,13.5313524995179,2.71468895094169));
#94709=CARTESIAN_POINT('Ctrl Pts',(-9.11859065541637,13.530971256108,2.71881934304621));
#94710=CARTESIAN_POINT('Ctrl Pts',(-9.11282308212285,13.5303719131736,2.72538881287748));
#94711=CARTESIAN_POINT('Ctrl Pts',(-9.11071427510706,13.5301524488659,2.72781072595031));
#94712=CARTESIAN_POINT('Ctrl Pts',(-9.10697432871951,13.5297626955485,2.73214160341194));
#94713=CARTESIAN_POINT('Ctrl Pts',(-9.10533938231773,13.5295921310226,2.73404716447577));
#94714=CARTESIAN_POINT('Ctrl Pts',(-9.10144108415476,13.529185003522,2.73862021641051));
#94715=CARTESIAN_POINT('Ctrl Pts',(-9.09918351282071,13.5289488631688,2.74129257461589));
#94716=CARTESIAN_POINT('Ctrl Pts',(-9.09235763756514,13.5282336215705,2.74944599491719));
#94717=CARTESIAN_POINT('Ctrl Pts',(-9.08782710005801,13.5277571608841,2.75495867259661));
#94718=CARTESIAN_POINT('Ctrl Pts',(-9.04434725895376,13.5231636827305,2.80885536108641));
#94719=CARTESIAN_POINT('Ctrl Pts',(-9.00922706805586,13.5192860417631,2.86021538210638));
#94720=CARTESIAN_POINT('Ctrl Pts',(-8.92987135235927,13.5094112713398,2.99859748077979));
#94721=CARTESIAN_POINT('Ctrl Pts',(-8.89209475876031,13.5034689921077,3.08875362681169));
#94722=CARTESIAN_POINT('Ctrl Pts',(-8.86205776357743,13.4961920378801,3.19605923742308));
#94723=CARTESIAN_POINT('Ctrl Pts',(-8.85851255205064,13.4952671613288,3.20965727312548));
#94724=CARTESIAN_POINT('Ctrl Pts',(-8.85369713570107,13.4939065842509,3.22958113313364));
#94725=CARTESIAN_POINT('Ctrl Pts',(-8.85223417215518,13.4934770652193,3.23585946565418));
#94726=CARTESIAN_POINT('Ctrl Pts',(-8.8497298533271,13.4927119753081,3.24702060252618));
#94727=CARTESIAN_POINT('Ctrl Pts',(-8.8486678561173,13.4923770737206,3.25189865173501));
#94728=CARTESIAN_POINT('Ctrl Pts',(-8.84651857882453,13.4916768023943,3.26208194592172));
#94729=CARTESIAN_POINT('Ctrl Pts',(-8.84543681485228,13.4913112652322,3.26738822203785));
#94730=CARTESIAN_POINT('Ctrl Pts',(-8.84271362612029,13.4903557495275,3.28123319761674));
#94731=CARTESIAN_POINT('Ctrl Pts',(-8.84113012233277,13.4897639466948,3.28978281584553));
#94732=CARTESIAN_POINT('Ctrl Pts',(-8.83443920364395,13.4870904902932,3.3282843064565));
#94733=CARTESIAN_POINT('Ctrl Pts',(-8.83039775859294,13.4849756468521,3.35840709179579));
#94734=CARTESIAN_POINT('Ctrl Pts',(-8.81836040085209,13.4759735540945,3.48515620388857));
#94735=CARTESIAN_POINT('Ctrl Pts',(-8.82114681937698,13.4687748718923,3.58241640124573));
#94736=CARTESIAN_POINT('Ctrl Pts',(-8.84207610111523,13.4586937655097,3.71913762794658));
#94737=CARTESIAN_POINT('Ctrl Pts',(-8.85049494617204,13.455714288772,3.75970747702375));
#94738=CARTESIAN_POINT('Ctrl Pts',(-8.86254728874883,13.4524227619116,3.80550242029854));
#94739=CARTESIAN_POINT('Ctrl Pts',(-8.86410377844083,13.4520117172482,3.81123974148636));
#94740=CARTESIAN_POINT('Ctrl Pts',(-8.8666666103228,13.4513570397813,3.82041112987392));
#94741=CARTESIAN_POINT('Ctrl Pts',(-8.86764525303397,13.4511119126466,3.82385273225124));
#94742=CARTESIAN_POINT('Ctrl Pts',(-8.86941557803412,13.4506770818707,3.82997230931403));
#94743=CARTESIAN_POINT('Ctrl Pts',(-8.87020111090193,13.4504870356863,3.83265196648745));
#94744=CARTESIAN_POINT('Ctrl Pts',(-8.87191539806998,13.4500784685929,3.8384237229732));
#94745=CARTESIAN_POINT('Ctrl Pts',(-8.87284733718414,13.449860133549,3.84151480307891));
#94746=CARTESIAN_POINT('Ctrl Pts',(-8.87547412178455,13.449254981772,3.85009950472141));
#94747=CARTESIAN_POINT('Ctrl Pts',(-8.87719652703085,13.448869712043,3.85558469935143));
#94748=CARTESIAN_POINT('Ctrl Pts',(-8.88752546273618,13.4466241379359,3.8876548524438));
#94749=CARTESIAN_POINT('Ctrl Pts',(-8.89703653688503,13.4448116294827,3.91394174865034));
#94750=CARTESIAN_POINT('Ctrl Pts',(-8.93467078143929,13.4383851192914,4.00741613913582));
#94751=CARTESIAN_POINT('Ctrl Pts',(-8.96807453249571,13.4339516560813,4.07230136291291));
#94752=CARTESIAN_POINT('Ctrl Pts',(-9.0428736911354,13.4253203500996,4.18948203404957));
#94753=CARTESIAN_POINT('Ctrl Pts',(-9.08312238771654,13.4211528557023,4.2421656847102));
#94754=CARTESIAN_POINT('Ctrl Pts',(-9.13424234251521,13.4161526702062,4.29853436830593));
#94755=CARTESIAN_POINT('Ctrl Pts',(-9.14099843210263,13.4154972282875,4.30579758960577));
#94756=CARTESIAN_POINT('Ctrl Pts',(-9.15220045267458,13.4144186063107,4.31753947740409));
#94757=CARTESIAN_POINT('Ctrl Pts',(-9.15659214938311,13.4139977259003,4.32206937935486));
#94758=CARTESIAN_POINT('Ctrl Pts',(-9.16453907753637,13.4132395327588,4.33013568334671));
#94759=CARTESIAN_POINT('Ctrl Pts',(-9.16808092334,13.4129028042966,4.33368510499508));
#94760=CARTESIAN_POINT('Ctrl Pts',(-9.17566798467224,13.4121839353929,4.34119190124458));
#94761=CARTESIAN_POINT('Ctrl Pts',(-9.17971926061898,13.4118015329181,4.34514294228123));
#94762=CARTESIAN_POINT('Ctrl Pts',(-9.19072684576405,13.4107663029892,4.35572447464828));
#94763=CARTESIAN_POINT('Ctrl Pts',(-9.19773596831187,13.410111128694,4.36229915264965));
#94764=CARTESIAN_POINT('Ctrl Pts',(-9.23507109561241,13.4066413103931,4.39647090009071));
#94765=CARTESIAN_POINT('Ctrl Pts',(-9.26673913051003,13.4037653010211,4.42255303752295));
#94766=CARTESIAN_POINT('Ctrl Pts',(-9.38313166017206,13.3934185291546,4.50863107826452));
#94767=CARTESIAN_POINT('Ctrl Pts',(-9.47434020441842,13.3856539260467,4.55902849766534));
#94768=CARTESIAN_POINT('Ctrl Pts',(-9.5925018559245,13.3765696820416,4.60524893815091));
#94769=CARTESIAN_POINT('Ctrl Pts',(-9.61428567920301,13.3749348647594,4.61303844857112));
#94770=CARTESIAN_POINT('Ctrl Pts',(-9.64166370856107,13.3729407448231,4.62192786222814));
#94771=CARTESIAN_POINT('Ctrl Pts',(-9.64705360877164,13.3725510445259,4.62363511600206));
#94772=CARTESIAN_POINT('Ctrl Pts',(-9.65557029735085,13.3719400260558,4.62626545195662));
#94773=CARTESIAN_POINT('Ctrl Pts',(-9.65868889565908,13.3717172866611,4.62721445122038));
#94774=CARTESIAN_POINT('Ctrl Pts',(-9.66449886008294,13.3713042319055,4.62895611909827));
#94775=CARTESIAN_POINT('Ctrl Pts',(-9.66718916598156,13.3711137292049,4.62975213331571));
#94776=CARTESIAN_POINT('Ctrl Pts',(-9.67340508601241,13.3706752797417,4.63156718435219));
#94777=CARTESIAN_POINT('Ctrl Pts',(-9.67693270485923,13.3704277156604,4.63257938099028));
#94778=CARTESIAN_POINT('Ctrl Pts',(-9.68439944628171,13.3699062593369,4.63468412449678));
#94779=CARTESIAN_POINT('Ctrl Pts',(-9.68833965256466,13.3696325813268,4.63577268891554));
#94780=CARTESIAN_POINT('Ctrl Pts',(-9.69890817809657,13.3689023151001,4.63863332567402));
#94781=CARTESIAN_POINT('Ctrl Pts',(-9.70554655628933,13.3684476060014,4.6403680590295));
#94782=CARTESIAN_POINT('Ctrl Pts',(-9.72623567590027,13.3670417596503,4.64558180482654));
#94783=CARTESIAN_POINT('Ctrl Pts',(-9.7403361380124,13.3660997458703,4.6488599978075));
#94784=CARTESIAN_POINT('Ctrl Pts',(-9.85441722306451,13.3585815513223,4.67317471803309));
#94785=CARTESIAN_POINT('Ctrl Pts',(-9.95669310330162,13.3524411064072,4.68138124185338));
#94786=CARTESIAN_POINT('Ctrl Pts',(-10.0986419529642,13.3434407515419,4.67429126807066));
#94787=CARTESIAN_POINT('Ctrl Pts',(-10.1384007360085,13.3408722499535,4.67027131412355));
#94788=CARTESIAN_POINT('Ctrl Pts',(-10.1876132325974,13.3375932649165,4.6627524971252));
#94789=CARTESIAN_POINT('Ctrl Pts',(-10.1973314329055,13.3369409198207,4.66114270902573));
#94790=CARTESIAN_POINT('Ctrl Pts',(-10.2127467781886,13.33589791752,4.65839009720257));
#94791=CARTESIAN_POINT('Ctrl Pts',(-10.2184577706468,13.3355097082673,4.65732666493088));
#94792=CARTESIAN_POINT('Ctrl Pts',(-10.2291318425239,13.3347806384625,4.65525724564447));
#94793=CARTESIAN_POINT('Ctrl Pts',(-10.2340967724754,13.3344401001199,4.65426141087529));
#94794=CARTESIAN_POINT('Ctrl Pts',(-10.2451888117559,13.3336760540079,4.65196212985747));
#94795=CARTESIAN_POINT('Ctrl Pts',(-10.2513122171472,13.3332520279136,4.65064176395554));
#94796=CARTESIAN_POINT('Ctrl Pts',(-10.2694048325153,13.3319923887743,4.6465892128724));
#94797=CARTESIAN_POINT('Ctrl Pts',(-10.2813418687755,13.3311524828205,4.6437187242201));
#94798=CARTESIAN_POINT('Ctrl Pts',(-10.3706449206016,13.3248000772339,4.62076147674413));
#94799=CARTESIAN_POINT('Ctrl Pts',(-10.445816601514,13.3190407780083,4.59303567102166));
#94800=CARTESIAN_POINT('Ctrl Pts',(-10.5716675881365,13.3087705362018,4.53146290535402));
#94801=CARTESIAN_POINT('Ctrl Pts',(-10.6236309027657,13.3043234952939,4.50090188616107));
#94802=CARTESIAN_POINT('Ctrl Pts',(-10.6730394577914,13.2999999999999,4.4664951892047));
#94803=CARTESIAN_POINT('',(-9.31533557546056,13.3,4.45829519891841));
#94804=CARTESIAN_POINT('Origin',(-10.,13.3,3.5));
#94805=CARTESIAN_POINT('Ctrl Pts',(-9.31533557546056,13.3,4.45829519891842));
#94806=CARTESIAN_POINT('Ctrl Pts',(-9.27955485067773,13.3029712552161,4.4327312710487));
#94807=CARTESIAN_POINT('Ctrl Pts',(-9.24520412249185,13.3058633132367,4.40510172653889));
#94808=CARTESIAN_POINT('Ctrl Pts',(-9.2125067118003,13.3087216394501,4.37560718174327));
#94809=CARTESIAN_POINT('Ctrl Pts',(-9.20890953043532,13.3090360960866,4.37236236129225));
#94810=CARTESIAN_POINT('Ctrl Pts',(-9.20533237168248,13.3093501444625,4.36909501894293));
#94811=CARTESIAN_POINT('Ctrl Pts',(-9.20177554086393,13.3096638451157,4.36580545935624));
#94812=CARTESIAN_POINT('Ctrl Pts',(-9.16642056516623,13.312782036431,4.33310716551634));
#94813=CARTESIAN_POINT('Ctrl Pts',(-9.13307223486999,13.3158666386743,4.29820842073811));
#94814=CARTESIAN_POINT('Ctrl Pts',(-9.10197737074274,13.3189690571681,4.26140275777538));
#94815=CARTESIAN_POINT('Ctrl Pts',(-9.07088946296696,13.322070781608,4.22460532874886));
#94816=CARTESIAN_POINT('Ctrl Pts',(-9.04205365923209,13.3251907834279,4.1859022640497));
#94817=CARTESIAN_POINT('Ctrl Pts',(-9.01567610080399,13.3283631623632,4.14560522160206));
#94818=CARTESIAN_POINT('Ctrl Pts',(-8.98929527243636,13.331535934568,4.10530318366201));
#94819=CARTESIAN_POINT('Ctrl Pts',(-8.96537303797927,13.3347613384183,4.06340697144733));
#94820=CARTESIAN_POINT('Ctrl Pts',(-8.94407975864983,13.3380509499895,4.02024207876584));
#94821=CARTESIAN_POINT('Ctrl Pts',(-8.92222134533198,13.3414278694515,3.9759315688413));
#94822=CARTESIAN_POINT('Ctrl Pts',(-8.90313329659415,13.3448726432002,3.93028412919885));
#94823=CARTESIAN_POINT('Ctrl Pts',(-8.88696388158558,13.3483705621843,3.88366497049273));
#94824=CARTESIAN_POINT('Ctrl Pts',(-8.87117968274283,13.351785147607,3.83815645515627));
#94825=CARTESIAN_POINT('Ctrl Pts',(-8.85817661103945,13.3552501723781,3.7917219170812));
#94826=CARTESIAN_POINT('Ctrl Pts',(-8.84805986849392,13.3587267852057,3.74471375304687));
#94827=CARTESIAN_POINT('Ctrl Pts',(-8.83757277461038,13.3623306690602,3.6959847251703));
#94828=CARTESIAN_POINT('Ctrl Pts',(-8.83018777323948,13.3659467765198,3.6466389664785));
#94829=CARTESIAN_POINT('Ctrl Pts',(-8.82598263306443,13.3695072207974,3.59708597188621));
#94830=CARTESIAN_POINT('Ctrl Pts',(-8.82228640539946,13.3726367746507,3.55352995665964));
#94831=CARTESIAN_POINT('Ctrl Pts',(-8.82104684420149,13.3757226976916,3.50981264481602));
#94832=CARTESIAN_POINT('Ctrl Pts',(-8.8222856938752,13.3787078477362,3.46622919277443));
#94833=CARTESIAN_POINT('Ctrl Pts',(-8.82245626402244,13.3791188560235,3.46022843579012));
#94834=CARTESIAN_POINT('Ctrl Pts',(-8.82267376941736,13.3795279539606,3.45423015119989));
#94835=CARTESIAN_POINT('Ctrl Pts',(-8.82293822277778,13.3799349924019,3.44823504541158));
#94836=CARTESIAN_POINT('Ctrl Pts',(-8.82293899910851,13.3799361873062,3.44821744614621));
#94837=CARTESIAN_POINT('Ctrl Pts',(-8.82293977584426,13.3799373821941,3.44819984688064));
#94838=CARTESIAN_POINT('Ctrl Pts',(-8.82294055298505,13.3799385770658,3.44818224761489));
#94839=CARTESIAN_POINT('Ctrl Pts',(-8.82478706990888,13.3827776388227,3.40636570327091));
#94840=CARTESIAN_POINT('Ctrl Pts',(-8.82892295448533,13.3855245455198,3.36454473495573));
#94841=CARTESIAN_POINT('Ctrl Pts',(-8.83532312249245,13.3882274772244,3.32299108896264));
#94842=CARTESIAN_POINT('Ctrl Pts',(-8.8363298521375,13.3886526412939,3.31645480940954));
#94843=CARTESIAN_POINT('Ctrl Pts',(-8.83739253724907,13.3890767173137,3.30992522352958));
#94844=CARTESIAN_POINT('Ctrl Pts',(-8.83851100094992,13.389499892797,3.30340347508238));
#94845=CARTESIAN_POINT('Ctrl Pts',(-8.8463451349046,13.3924639705939,3.25772273379857));
#94846=CARTESIAN_POINT('Ctrl Pts',(-8.85691924720082,13.3953845903242,3.21242140052275));
#94847=CARTESIAN_POINT('Ctrl Pts',(-8.87014669802613,13.3983178983678,3.16784756043915));
#94848=CARTESIAN_POINT('Ctrl Pts',(-8.88335905457101,13.4012478591169,3.12332458503472));
#94849=CARTESIAN_POINT('Ctrl Pts',(-8.89921819650777,13.4041909205412,3.07952744451848));
#94850=CARTESIAN_POINT('Ctrl Pts',(-8.91759907150029,13.4071860650398,3.03678282607116));
#94851=CARTESIAN_POINT('Ctrl Pts',(-8.93596749485212,13.4101791805563,2.99406716384223));
#94852=CARTESIAN_POINT('Ctrl Pts',(-8.95685393734695,13.4132245375064,2.95240257307865));
#94853=CARTESIAN_POINT('Ctrl Pts',(-8.98010084810828,13.4163391323926,2.91209515177081));
#94854=CARTESIAN_POINT('Ctrl Pts',(-9.00334278896435,13.4194530614165,2.87179634769677));
#94855=CARTESIAN_POINT('Ctrl Pts',(-9.02894404419675,13.4226362773876,2.83285413167521));
#94856=CARTESIAN_POINT('Ctrl Pts',(-9.05671770647299,13.4258815931662,2.79555469395453));
#94857=CARTESIAN_POINT('Ctrl Pts',(-9.08451798305426,13.4291300187913,2.75821951378825));
#94858=CARTESIAN_POINT('Ctrl Pts',(-9.11449484231353,13.4324406099238,2.72253030300228));
#94859=CARTESIAN_POINT('Ctrl Pts',(-9.14643234661305,13.4357817278187,2.68875403987866));
#94860=CARTESIAN_POINT('Ctrl Pts',(-9.17838774451515,13.4391247176393,2.65495885295238));
#94861=CARTESIAN_POINT('Ctrl Pts',(-9.21230617688561,13.4424980354468,2.62307888816323));
#94862=CARTESIAN_POINT('Ctrl Pts',(-9.24794135391478,13.4458476269234,2.59336032458294));
#94863=CARTESIAN_POINT('Ctrl Pts',(-9.28183228109596,13.4490332645514,2.56509640790858));
#94864=CARTESIAN_POINT('Ctrl Pts',(-9.31727655903721,13.452196989286,2.53878737947735));
#94865=CARTESIAN_POINT('Ctrl Pts',(-9.35403222356578,13.4552777283284,2.51462499684154));
#94866=CARTESIAN_POINT('Ctrl Pts',(-9.35599573057558,13.455442303035,2.51333422960097));
#94867=CARTESIAN_POINT('Ctrl Pts',(-9.35796298531366,13.4556066409209,2.51204957719333));
#94868=CARTESIAN_POINT('Ctrl Pts',(-9.35993395280853,13.4557707326757,2.51077106511618));
#94869=CARTESIAN_POINT('Ctrl Pts',(-9.37393448287944,13.4569363386806,2.50168930865456));
#94870=CARTESIAN_POINT('Ctrl Pts',(-9.38812169294092,13.458089405079,2.49291774113444));
#94871=CARTESIAN_POINT('Ctrl Pts',(-9.40248114251727,13.4592262978203,2.48446578966191));
#94872=CARTESIAN_POINT('Ctrl Pts',(-9.40249912531988,13.4592277215878,2.48445520501003));
#94873=CARTESIAN_POINT('Ctrl Pts',(-9.40251710842823,13.4592291453322,2.48444462083696));
#94874=CARTESIAN_POINT('Ctrl Pts',(-9.40253509184229,13.4592305690533,2.48443403714275));
#94875=CARTESIAN_POINT('Ctrl Pts',(-9.43872182154729,13.4620954206655,2.46313723108009));
#94876=CARTESIAN_POINT('Ctrl Pts',(-9.47615075797707,13.4648664476682,2.44377993774979));
#94877=CARTESIAN_POINT('Ctrl Pts',(-9.51457842010804,13.467589944673,2.42648542847173));
#94878=CARTESIAN_POINT('Ctrl Pts',(-9.51897800508859,13.4679017579827,2.42450537922995));
#94879=CARTESIAN_POINT('Ctrl Pts',(-9.52339062599426,13.4682129482707,2.42255235918054));
#94880=CARTESIAN_POINT('Ctrl Pts',(-9.52781587487007,13.4685235850126,2.42062654460647));
#94881=CARTESIAN_POINT('Ctrl Pts',(-9.57294223216398,13.4716912948965,2.40098810189049));
#94882=CARTESIAN_POINT('Ctrl Pts',(-9.61938825430672,13.4748024362306,2.38417988326783));
#94883=CARTESIAN_POINT('Ctrl Pts',(-9.66675063387697,13.4779224731179,2.37033497931386));
#94884=CARTESIAN_POINT('Ctrl Pts',(-9.71411295086191,13.4810425058823,2.35649009365473));
#94885=CARTESIAN_POINT('Ctrl Pts',(-9.76239127307546,13.484172041595,2.34560793136728));
#94886=CARTESIAN_POINT('Ctrl Pts',(-9.81117889814932,13.4873563446704,2.33776762587097));
#94887=CARTESIAN_POINT('Origin',(-10.,12.3756328852638,3.5));
#94888=CARTESIAN_POINT('',(-9.81110406370901,14.0854724903439,2.33749693000287));
#94889=CARTESIAN_POINT('',(-9.81110406371068,13.9872487449619,2.3374969300026));
#94890=CARTESIAN_POINT('',(-9.81110406371068,12.3756328852638,2.3374969300026));
#94891=CARTESIAN_POINT('Ctrl Pts',(-9.81110406370735,14.0854724903439,2.33749693000314));
#94892=CARTESIAN_POINT('Ctrl Pts',(-9.80837956425245,14.08528176319,2.33793963582365));
#94893=CARTESIAN_POINT('Ctrl Pts',(-9.80565658690304,14.0850915193238,2.33839192511108));
#94894=CARTESIAN_POINT('Ctrl Pts',(-9.7993878303637,14.0846544523039,2.33945583192401));
#94895=CARTESIAN_POINT('Ctrl Pts',(-9.79584319597262,14.0844079842951,2.3400741364642));
#94896=CARTESIAN_POINT('Ctrl Pts',(-9.7895438660327,14.0839712321639,2.34120272428794));
#94897=CARTESIAN_POINT('Ctrl Pts',(-9.78678809288852,14.0837805978782,2.34170660288027));
#94898=CARTESIAN_POINT('Ctrl Pts',(-9.78086154463636,14.083371565388,2.3428121090767));
#94899=CARTESIAN_POINT('Ctrl Pts',(-9.77769143347412,14.0831533484427,2.34341693795891));
#94900=CARTESIAN_POINT('Ctrl Pts',(-9.76887736037341,14.0825481236561,2.34513616246796));
#94901=CARTESIAN_POINT('Ctrl Pts',(-9.76323892260838,14.0821626686444,2.34627891006022));
#94902=CARTESIAN_POINT('Ctrl Pts',(-9.73010552204535,14.0799064780369,2.35324722404107));
#94903=CARTESIAN_POINT('Ctrl Pts',(-9.70281532783585,14.0780841629291,2.36001468202912));
#94904=CARTESIAN_POINT('Ctrl Pts',(-9.60459418311645,14.0715707251508,2.38813943943628));
#94905=CARTESIAN_POINT('Ctrl Pts',(-9.53547432530339,14.0670656701688,2.4151971921999));
#94906=CARTESIAN_POINT('Ctrl Pts',(-9.41233600380801,14.0584938892006,2.47734431687218));
#94907=CARTESIAN_POINT('Ctrl Pts',(-9.3577646487029,14.054467079317,2.51070443143162));
#94908=CARTESIAN_POINT('Ctrl Pts',(-9.29821176979242,14.049625114584,2.55412191948246));
#94909=CARTESIAN_POINT('Ctrl Pts',(-9.29032667258213,14.048974447299,2.56002349923409));
#94910=CARTESIAN_POINT('Ctrl Pts',(-9.2775435736164,14.0479032512061,2.56984350681934));
#94911=CARTESIAN_POINT('Ctrl Pts',(-9.2726011146419,14.0474849950673,2.57370347682784));
#94912=CARTESIAN_POINT('Ctrl Pts',(-9.26378310363801,14.0467312509447,2.58070427705748));
#94913=CARTESIAN_POINT('Ctrl Pts',(-9.25989620626059,14.0463963411528,2.58383062816507));
#94914=CARTESIAN_POINT('Ctrl Pts',(-9.25166194902176,14.0456810702316,2.59054029073654));
#94915=CARTESIAN_POINT('Ctrl Pts',(-9.24732021881102,14.0453004464793,2.59413028177683));
#94916=CARTESIAN_POINT('Ctrl Pts',(-9.23566804944887,14.0442693866189,2.60390656560067));
#94917=CARTESIAN_POINT('Ctrl Pts',(-9.22840716625819,14.043616603529,2.61015098848929));
#94918=CARTESIAN_POINT('Ctrl Pts',(-9.19050910362557,14.040153721968,2.64355626196296));
#94919=CARTESIAN_POINT('Ctrl Pts',(-9.16123099808947,14.0372819798163,2.67220941551946));
#94920=CARTESIAN_POINT('Ctrl Pts',(-9.06398839877253,14.0270179475793,2.77784157855102));
#94921=CARTESIAN_POINT('Ctrl Pts',(-9.00464969901487,14.0193354171032,2.8621093127799));
#94922=CARTESIAN_POINT('Ctrl Pts',(-8.94544145929536,14.0101828713199,2.97500555064854));
#94923=CARTESIAN_POINT('Ctrl Pts',(-8.93459575007949,14.0084217750301,2.99737998072639));
#94924=CARTESIAN_POINT('Ctrl Pts',(-8.92212472719435,14.0063000115036,3.02532858008758));
#94925=CARTESIAN_POINT('Ctrl Pts',(-8.91982231292956,14.0059038018646,3.03059161880807));
#94926=CARTESIAN_POINT('Ctrl Pts',(-8.91627391270032,14.0052862605735,3.03886720469023));
#94927=CARTESIAN_POINT('Ctrl Pts',(-8.91500180701086,14.0050634264173,3.04186834963261));
#94928=CARTESIAN_POINT('Ctrl Pts',(-8.91266153927544,14.0046508234429,3.04745392056078));
#94929=CARTESIAN_POINT('Ctrl Pts',(-8.9115901276884,14.0044608695345,3.05003685450816));
#94930=CARTESIAN_POINT('Ctrl Pts',(-8.90915693218752,14.0040270119564,3.05596228783824));
#94931=CARTESIAN_POINT('Ctrl Pts',(-8.90780130535554,14.0037834764147,3.05930724908921));
#94932=CARTESIAN_POINT('Ctrl Pts',(-8.90363242306076,14.0030286707225,3.06973121886648));
#94933=CARTESIAN_POINT('Ctrl Pts',(-8.90087238465933,14.0025204370554,3.07683149867637));
#94934=CARTESIAN_POINT('Ctrl Pts',(-8.89456594422872,14.0013376021882,3.09353307812985));
#94935=CARTESIAN_POINT('Ctrl Pts',(-8.89107537013762,14.0006658735758,3.10315495299672));
#94936=CARTESIAN_POINT('Ctrl Pts',(-8.87911718848562,13.9982977857457,3.13750850885843));
#94937=CARTESIAN_POINT('Ctrl Pts',(-8.87134750287598,13.9966318132238,3.16247653999496));
#94938=CARTESIAN_POINT('Ctrl Pts',(-8.8426226113462,13.9898110202216,3.26692066333203));
#94939=CARTESIAN_POINT('Ctrl Pts',(-8.82918295799498,13.9848359978717,3.3482213230498));
#94940=CARTESIAN_POINT('Ctrl Pts',(-8.8216152638385,13.976799362719,3.47580071364178));
#94941=CARTESIAN_POINT('Ctrl Pts',(-8.82156239420987,13.9738818217062,3.52145363692289));
#94942=CARTESIAN_POINT('Ctrl Pts',(-8.82473330240428,13.9702143704019,3.57711019003066));
#94943=CARTESIAN_POINT('Ctrl Pts',(-8.82544040421432,13.9695437352526,3.58722119742213));
#94944=CARTESIAN_POINT('Ctrl Pts',(-8.82675838488983,13.9684819970452,3.60311636968189));
#94945=CARTESIAN_POINT('Ctrl Pts',(-8.8272817732766,13.9680936149897,3.60890744592317));
#94946=CARTESIAN_POINT('Ctrl Pts',(-8.82832745145944,13.9673739226933,3.61959405825179));
#94947=CARTESIAN_POINT('Ctrl Pts',(-8.82883759863378,13.9670429982251,3.62449067488374));
#94948=CARTESIAN_POINT('Ctrl Pts',(-8.83003797939917,13.966306365672,3.63535131346133));
#94949=CARTESIAN_POINT('Ctrl Pts',(-8.83074314345513,13.9659001997227,3.64131351248222));
#94950=CARTESIAN_POINT('Ctrl Pts',(-8.83290815535112,13.9647247017439,3.65849169076727));
#94951=CARTESIAN_POINT('Ctrl Pts',(-8.83448399259513,13.9639517741263,3.66969210595782));
#94952=CARTESIAN_POINT('Ctrl Pts',(-8.83840359154376,13.9621961434827,3.6949124526799));
#94953=CARTESIAN_POINT('Ctrl Pts',(-8.84084031144782,13.9612106656738,3.70891593162067));
#94954=CARTESIAN_POINT('Ctrl Pts',(-8.84963073527725,13.9579649509341,3.75452907296625));
#94955=CARTESIAN_POINT('Ctrl Pts',(-8.85702853339019,13.9556742860442,3.78592027868278));
#94956=CARTESIAN_POINT('Ctrl Pts',(-8.87970554916105,13.9496086225872,3.86707228580801));
#94957=CARTESIAN_POINT('Ctrl Pts',(-8.89701095039513,13.9457899365153,3.91619251828558));
#94958=CARTESIAN_POINT('Ctrl Pts',(-8.94130221639083,13.937535480823,4.01952141313446));
#94959=CARTESIAN_POINT('Ctrl Pts',(-8.96933737147941,13.9331105791918,4.07313134795413));
#94960=CARTESIAN_POINT('Ctrl Pts',(-9.00654694123221,13.9281918136267,4.13264653299781));
#94961=CARTESIAN_POINT('Ctrl Pts',(-9.01183221356889,13.927512092796,4.14087054632215));
#94962=CARTESIAN_POINT('Ctrl Pts',(-9.01926021911617,13.926583422091,4.15211828557405));
#94963=CARTESIAN_POINT('Ctrl Pts',(-9.02131555656593,13.9263291760415,4.15519885325083));
#94964=CARTESIAN_POINT('Ctrl Pts',(-9.02486407265412,13.9258949198086,4.16046346195009));
#94965=CARTESIAN_POINT('Ctrl Pts',(-9.02635012675529,13.9257144494322,4.1626522361365));
#94966=CARTESIAN_POINT('Ctrl Pts',(-9.02946778142215,13.9253387479846,4.16721102657631));
#94967=CARTESIAN_POINT('Ctrl Pts',(-9.03110070762115,13.9251436149046,4.16958009434967));
#94968=CARTESIAN_POINT('Ctrl Pts',(-9.03510643221353,13.9246688727887,4.17534630798837));
#94969=CARTESIAN_POINT('Ctrl Pts',(-9.03748853902933,13.9243898837448,4.17873700478768));
#94970=CARTESIAN_POINT('Ctrl Pts',(-9.04611528456408,13.9233911285465,4.19087958454551));
#94971=CARTESIAN_POINT('Ctrl Pts',(-9.05246202486794,13.9226778949883,4.19955875850679));
#94972=CARTESIAN_POINT('Ctrl Pts',(-9.06860179853754,13.9209135832482,4.22100718239029));
#94973=CARTESIAN_POINT('Ctrl Pts',(-9.07853956948397,13.9198707761825,4.23366524765841));
#94974=CARTESIAN_POINT('Ctrl Pts',(-9.12316729819788,13.9153538720209,4.28817112729778));
#94975=CARTESIAN_POINT('Ctrl Pts',(-9.16047322840555,13.9119976525774,4.32779529529698));
#94976=CARTESIAN_POINT('Ctrl Pts',(-9.26033177781935,13.9035901425369,4.42013719575697));
#94977=CARTESIAN_POINT('Ctrl Pts',(-9.32587192127041,13.8985432781847,4.46918045473273));
#94978=CARTESIAN_POINT('Ctrl Pts',(-9.40885645597812,13.892238466229,4.51875920346066));
#94979=CARTESIAN_POINT('Ctrl Pts',(-9.42190615942508,13.8912499787935,4.52622048425328));
#94980=CARTESIAN_POINT('Ctrl Pts',(-9.44092897139612,13.8898114390106,4.53661895529123));
#94981=CARTESIAN_POINT('Ctrl Pts',(-9.44679012810352,13.8893685338116,4.53975867780928));
#94982=CARTESIAN_POINT('Ctrl Pts',(-9.45715150761605,13.8885859764846,4.54519668373168));
#94983=CARTESIAN_POINT('Ctrl Pts',(-9.46164056230823,13.8882470695151,4.54751597021385));
#94984=CARTESIAN_POINT('Ctrl Pts',(-9.47094694665004,13.8875446782512,4.55224852523675));
#94985=CARTESIAN_POINT('Ctrl Pts',(-9.47576618230397,13.8871810636836,4.55465776194756));
#94986=CARTESIAN_POINT('Ctrl Pts',(-9.48818861456843,13.8862439775683,4.56076181461754));
#94987=CARTESIAN_POINT('Ctrl Pts',(-9.49581525737343,13.8856688461363,4.56440793891283));
#94988=CARTESIAN_POINT('Ctrl Pts',(-9.52851084610568,13.8832035360072,4.57960872120166));
#94989=CARTESIAN_POINT('Ctrl Pts',(-9.55394076555903,13.8812865073426,4.59036138589155));
#94990=CARTESIAN_POINT('Ctrl Pts',(-9.67268587944295,13.8723299124985,4.63572164850167));
#94991=CARTESIAN_POINT('Ctrl Pts',(-9.76976591482076,13.864946989495,4.65930346886787));
#94992=CARTESIAN_POINT('Ctrl Pts',(-9.89060094924893,13.8560847530131,4.67286645625058));
#94993=CARTESIAN_POINT('Ctrl Pts',(-9.91263830147108,13.8544837874729,4.67471354138045));
#94994=CARTESIAN_POINT('Ctrl Pts',(-9.95646627226951,13.8513443683494,4.67714673175867));
#94995=CARTESIAN_POINT('Ctrl Pts',(-9.97824804066715,13.8498059105185,4.67775065866112));
#94996=CARTESIAN_POINT('Ctrl Pts',(-10.0055474180099,13.8479147422302,4.67774983269789));
#94997=CARTESIAN_POINT('Ctrl Pts',(-10.0110592698183,13.8475348008846,4.67771097379941));
#94998=CARTESIAN_POINT('Ctrl Pts',(-10.0197770360231,13.8469370744195,4.67758830389097));
#94999=CARTESIAN_POINT('Ctrl Pts',(-10.0229831434751,13.8467179359008,4.67753009318425));
#95000=CARTESIAN_POINT('Ctrl Pts',(-10.0287134496716,13.8463275403495,4.67740263979577));
#95001=CARTESIAN_POINT('Ctrl Pts',(-10.0312376496056,13.8461560171673,4.67733837438944));
#95002=CARTESIAN_POINT('Ctrl Pts',(-10.0372984416242,13.8457452268282,4.67716456266365));
#95003=CARTESIAN_POINT('Ctrl Pts',(-10.0408347677477,13.8455063941555,4.67704719697413));
#95004=CARTESIAN_POINT('Ctrl Pts',(-10.0516093611394,13.8447811659782,4.67664098642276));
#95005=CARTESIAN_POINT('Ctrl Pts',(-10.0588457060926,13.8442974712538,4.67630129068867));
#95006=CARTESIAN_POINT('Ctrl Pts',(-10.1245044307226,13.8399356067439,4.67261163949672));
#95007=CARTESIAN_POINT('Ctrl Pts',(-10.18261298426,13.8362668928653,4.66497804775069));
#95008=CARTESIAN_POINT('Ctrl Pts',(-10.3385299155154,13.826384221879,4.63253584678592));
#95009=CARTESIAN_POINT('Ctrl Pts',(-10.4340888607832,13.8202473931297,4.59945656712744));
#95010=CARTESIAN_POINT('Ctrl Pts',(-10.5364514753908,13.8127735873552,4.54857039888152));
#95011=CARTESIAN_POINT('Ctrl Pts',(-10.5485249244142,13.8118775907887,4.54230535313244));
#95012=CARTESIAN_POINT('Ctrl Pts',(-10.566169355979,13.8105452575769,4.53275799160945));
#95013=CARTESIAN_POINT('Ctrl Pts',(-10.5718264447905,13.8101145565875,4.5296365004787));
#95014=CARTESIAN_POINT('Ctrl Pts',(-10.5818245613224,13.8093469057134,4.52401188938961));
#95015=CARTESIAN_POINT('Ctrl Pts',(-10.5861758713091,13.8090106203361,4.52152729593227));
#95016=CARTESIAN_POINT('Ctrl Pts',(-10.5952936625973,13.8083012628786,4.51624360818539));
#95017=CARTESIAN_POINT('Ctrl Pts',(-10.6000565461852,13.8079279838481,4.513438580025));
#95018=CARTESIAN_POINT('Ctrl Pts',(-10.6125956175627,13.8069379148144,4.50593450120273));
#95019=CARTESIAN_POINT('Ctrl Pts',(-10.6203373498948,13.8063190909114,4.5011788929235));
#95020=CARTESIAN_POINT('Ctrl Pts',(-10.6570429591657,13.8033481314669,4.47804210995675));
#95021=CARTESIAN_POINT('Ctrl Pts',(-10.6852469258132,13.8009534835102,4.45849259394078));
#95022=CARTESIAN_POINT('Ctrl Pts',(-10.7646943656913,13.7938685266969,4.39812342878894));
#95023=CARTESIAN_POINT('Ctrl Pts',(-10.8134329889313,13.7890758541339,4.35422956894727));
#95024=CARTESIAN_POINT('Ctrl Pts',(-10.9014867757059,13.7796337438237,4.26052614088151));
#95025=CARTESIAN_POINT('Ctrl Pts',(-10.940944382723,13.7750021153455,4.211128461665));
#95026=CARTESIAN_POINT('Ctrl Pts',(-10.9817324936223,13.7698920932885,4.15068597421095));
#95027=CARTESIAN_POINT('Ctrl Pts',(-10.9871081230018,13.7692112610803,4.14250174726328));
#95028=CARTESIAN_POINT('Ctrl Pts',(-10.9943767810737,13.7682813400099,4.13112883815841));
#95029=CARTESIAN_POINT('Ctrl Pts',(-10.9963575737781,13.7680269375681,4.12799711719326));
#95030=CARTESIAN_POINT('Ctrl Pts',(-10.999727730152,13.7675924551595,4.12261266646345));
#95031=CARTESIAN_POINT('Ctrl Pts',(-11.0011243259431,13.767411914338,4.1203645309294));
#95032=CARTESIAN_POINT('Ctrl Pts',(-11.0040219849772,13.7670363292457,4.11566482703329));
#95033=CARTESIAN_POINT('Ctrl Pts',(-11.0055216641355,13.7668413820931,4.11321244991888));
#95034=CARTESIAN_POINT('Ctrl Pts',(-11.0091581734917,13.7663672209954,4.10721657208559));
#95035=CARTESIAN_POINT('Ctrl Pts',(-11.0112853641807,13.7660886252733,4.1036672080122));
#95036=CARTESIAN_POINT('Ctrl Pts',(-11.0188603161551,13.7650917955673,4.09087546535479));
#95037=CARTESIAN_POINT('Ctrl Pts',(-11.0242006403187,13.7643800722587,4.08156962429296));
#95038=CARTESIAN_POINT('Ctrl Pts',(-11.0372101068087,13.7626200112229,4.05816467537152));
#95039=CARTESIAN_POINT('Ctrl Pts',(-11.0447198199632,13.7615799072526,4.04397900864297));
#95040=CARTESIAN_POINT('Ctrl Pts',(-11.0762713540244,13.7570811504198,3.98131376014176));
#95041=CARTESIAN_POINT('Ctrl Pts',(-11.0972474827516,13.7537395921702,3.93136047198861));
#95042=CARTESIAN_POINT('Ctrl Pts',(-11.1411906507918,13.7453247149666,3.80250179563829));
#95043=CARTESIAN_POINT('Ctrl Pts',(-11.1594801565671,13.7402564862725,3.72232200786644));
#95044=CARTESIAN_POINT('Ctrl Pts',(-11.1710883507654,13.7339280573422,3.62598685320325));
#95045=CARTESIAN_POINT('Ctrl Pts',(-11.1725995971807,13.7329404554373,3.61104397218368));
#95046=CARTESIAN_POINT('Ctrl Pts',(-11.1743665611913,13.7315032277465,3.58945597590824));
#95047=CARTESIAN_POINT('Ctrl Pts',(-11.1748524371892,13.7310607441739,3.58283078809333));
#95048=CARTESIAN_POINT('Ctrl Pts',(-11.1756088354499,13.7302789488712,3.5711646646585));
#95049=CARTESIAN_POINT('Ctrl Pts',(-11.1759030463892,13.7299403817666,3.56612539313044));
#95050=CARTESIAN_POINT('Ctrl Pts',(-11.1764440058136,13.7292387159503,3.5557093636069));
#95051=CARTESIAN_POINT('Ctrl Pts',(-11.1766863088642,13.728875487204,3.55033250315407));
#95052=CARTESIAN_POINT('Ctrl Pts',(-11.1772140401526,13.7279394503562,3.53651662063033));
#95053=CARTESIAN_POINT('Ctrl Pts',(-11.1774455797892,13.7273649845954,3.5280759697063));
#95054=CARTESIAN_POINT('Ctrl Pts',(-11.1780457970171,13.7249032785167,3.49207634041549));
#95055=CARTESIAN_POINT('Ctrl Pts',(-11.1775377579458,13.7229892434101,3.46451348214993));
#95056=CARTESIAN_POINT('Ctrl Pts',(-11.1707442772212,13.7140415613419,3.33770365225719));
#95057=CARTESIAN_POINT('Ctrl Pts',(-11.1528717543418,13.7066645796645,3.2394946298067));
#95058=CARTESIAN_POINT('Ctrl Pts',(-11.1162251753926,13.6978088470079,3.12367050014724));
#95059=CARTESIAN_POINT('Ctrl Pts',(-11.1089739631477,13.6962097257088,3.1028106533509));
#95060=CARTESIAN_POINT('Ctrl Pts',(-11.0933515939303,13.6930594365367,3.06164018187035));
#95061=CARTESIAN_POINT('Ctrl Pts',(-11.084989894004,13.6915086255878,3.04133441429724));
#95062=CARTESIAN_POINT('Ctrl Pts',(-11.0738200224146,13.6896048092734,3.01622720345842));
#95063=CARTESIAN_POINT('Ctrl Pts',(-11.0715397902647,13.689224111752,3.01119734032934));
#95064=CARTESIAN_POINT('Ctrl Pts',(-11.0678795653503,13.6886256001244,3.00327212577477));
#95065=CARTESIAN_POINT('Ctrl Pts',(-11.0665230168985,13.6884064238553,3.00036613187721));
#95066=CARTESIAN_POINT('Ctrl Pts',(-11.0640785260399,13.6880161980655,2.99518487256374));
#95067=CARTESIAN_POINT('Ctrl Pts',(-11.0629951518513,13.6878448808323,2.99290757274255));
#95068=CARTESIAN_POINT('Ctrl Pts',(-11.0603782759185,13.6874349223575,2.98745202497275));
#95069=CARTESIAN_POINT('Ctrl Pts',(-11.0588377962123,13.6871967124288,2.98427717049367));
#95070=CARTESIAN_POINT('Ctrl Pts',(-11.0541083891418,13.6864746479896,2.97464061063705));
#95071=CARTESIAN_POINT('Ctrl Pts',(-11.0508743377206,13.6859934644342,2.96820105604369));
#95072=CARTESIAN_POINT('Ctrl Pts',(-11.0179835920254,13.681219034786,2.90418177205053));
#95073=CARTESIAN_POINT('Ctrl Pts',(-10.9836794412224,13.6771835961947,2.84910276219508));
#95074=CARTESIAN_POINT('Ctrl Pts',(-10.889158746204,13.6673777876629,2.72202108219114));
#95075=CARTESIAN_POINT('Ctrl Pts',(-10.8245585009238,13.661645284195,2.65385844811415));
#95076=CARTESIAN_POINT('Ctrl Pts',(-10.7414997696614,13.6545950961847,2.58486039712428));
#95077=CARTESIAN_POINT('Ctrl Pts',(-10.7302563065948,13.6536474519342,2.5758635932318));
#95078=CARTESIAN_POINT('Ctrl Pts',(-10.7136718498343,13.652257663125,2.56308468655812));
#95079=CARTESIAN_POINT('Ctrl Pts',(-10.7084595318908,13.6518219917088,2.55913714996341));
#95080=CARTESIAN_POINT('Ctrl Pts',(-10.699174229687,13.6510477069659,2.55222585544457));
#95081=CARTESIAN_POINT('Ctrl Pts',(-10.6951145612694,13.6507097873466,2.54924441736699));
#95082=CARTESIAN_POINT('Ctrl Pts',(-10.6866325091008,13.6500049453644,2.54309852633936));
#95083=CARTESIAN_POINT('Ctrl Pts',(-10.682207092241,13.6496378651427,2.53993848403971));
#95084=CARTESIAN_POINT('Ctrl Pts',(-10.6706648083156,13.6486820691636,2.53181662605135));
#95085=CARTESIAN_POINT('Ctrl Pts',(-10.6635148240792,13.6480915663578,2.52690267602969));
#95086=CARTESIAN_POINT('Ctrl Pts',(-10.6315966582526,13.64546188905,2.50548169684432));
#95087=CARTESIAN_POINT('Ctrl Pts',(-10.6062641768747,13.6433912232271,2.48983938567262));
#95088=CARTESIAN_POINT('Ctrl Pts',(-10.4949928936122,13.6343578126546,2.42682541581478));
#95089=CARTESIAN_POINT('Ctrl Pts',(-10.4039172242116,13.6270741246665,2.38933931355589));
#95090=CARTESIAN_POINT('Ctrl Pts',(-10.2698749665405,13.6169581516545,2.35286024369748));
#95091=CARTESIAN_POINT('Ctrl Pts',(-10.2299426472491,13.6140225585947,2.34419324574026));
#95092=CARTESIAN_POINT('Ctrl Pts',(-10.1837658743357,13.6107714209558,2.33665974472558));
#95093=CARTESIAN_POINT('Ctrl Pts',(-10.1778877522899,13.6103602146303,2.33574642050255));
#95094=CARTESIAN_POINT('Ctrl Pts',(-10.1684488893274,13.6097044274908,2.3343529951947));
#95095=CARTESIAN_POINT('Ctrl Pts',(-10.1648925250124,13.6094583656049,2.33384459689718));
#95096=CARTESIAN_POINT('Ctrl Pts',(-10.1585530178436,13.6090216308315,2.33296791653498));
#95097=CARTESIAN_POINT('Ctrl Pts',(-10.1557708316414,13.6088306147442,2.33259330484696));
#95098=CARTESIAN_POINT('Ctrl Pts',(-10.1497653465816,13.6084197101163,2.3318065390477));
#95099=CARTESIAN_POINT('Ctrl Pts',(-10.1465416728934,13.6082000101842,2.33139777511911));
#95100=CARTESIAN_POINT('Ctrl Pts',(-10.1375434478926,13.6075890815874,2.33029461437776));
#95101=CARTESIAN_POINT('Ctrl Pts',(-10.1317652856069,13.6071994382068,2.32962963034546));
#95102=CARTESIAN_POINT('Ctrl Pts',(-10.0971794904755,13.6048818116319,2.32590868639687));
#95103=CARTESIAN_POINT('Ctrl Pts',(-10.0682693609797,13.6030050573454,2.32387335716873));
#95104=CARTESIAN_POINT('Ctrl Pts',(-9.97995507240773,13.597376613144,2.32092395638361));
#95105=CARTESIAN_POINT('Ctrl Pts',(-9.92053037097864,13.5937299755792,2.32343396867559));
#95106=CARTESIAN_POINT('Ctrl Pts',(-9.84467507092052,13.5890005060176,2.33241367566494));
#95107=CARTESIAN_POINT('Ctrl Pts',(-9.82785742148521,13.5879474689535,2.33477466451822));
#95108=CARTESIAN_POINT('Ctrl Pts',(-9.81110401834328,13.5868901487969,2.33749693737438));
#95109=CARTESIAN_POINT('Ctrl Pts',(-9.81114449848021,13.4871956596082,2.33749036045042));
#95110=CARTESIAN_POINT('Ctrl Pts',(-9.83460130906247,13.4887031289619,2.33367968432709));
#95111=CARTESIAN_POINT('Ctrl Pts',(-9.85816692158536,13.4902261927543,2.33058002303858));
#95112=CARTESIAN_POINT('Ctrl Pts',(-9.89603391445815,13.4926982099412,2.32676067340649));
#95113=CARTESIAN_POINT('Ctrl Pts',(-9.91028309603021,13.4936339341941,2.32558511857208));
#95114=CARTESIAN_POINT('Ctrl Pts',(-9.93111828325639,13.4950118606764,2.3242476042958));
#95115=CARTESIAN_POINT('Ctrl Pts',(-9.93769019833253,13.4954478953722,2.32388101254519));
#95116=CARTESIAN_POINT('Ctrl Pts',(-9.94927241800302,13.4962189895655,2.3233322864495));
#95117=CARTESIAN_POINT('Ctrl Pts',(-9.95428150030809,13.4965533397589,2.32312701909735));
#95118=CARTESIAN_POINT('Ctrl Pts',(-9.96412617670132,13.4972122344832,2.3227865394719));
#95119=CARTESIAN_POINT('Ctrl Pts',(-9.96896159899539,13.4975367052893,2.32264912649977));
#95120=CARTESIAN_POINT('Ctrl Pts',(-9.97858607342345,13.4981842655482,2.32243495024421));
#95121=CARTESIAN_POINT('Ctrl Pts',(-9.98337502064357,13.4985073308852,2.32235760454786));
#95122=CARTESIAN_POINT('Ctrl Pts',(-9.99474056699205,13.4992761383291,2.32224338116128));
#95123=CARTESIAN_POINT('Ctrl Pts',(-10.0013172085728,13.4997226601407,2.3222323757135));
#95124=CARTESIAN_POINT('Ctrl Pts',(-10.0247357045077,13.5013187391237,2.32238933406711));
#95125=CARTESIAN_POINT('Ctrl Pts',(-10.041572779569,13.5024774958713,2.32286347872021));
#95126=CARTESIAN_POINT('Ctrl Pts',(-10.092976770881,13.5060511559269,2.32541524174278));
#95127=CARTESIAN_POINT('Ctrl Pts',(-10.1274647444889,13.5084991700587,2.32865616239873));
#95128=CARTESIAN_POINT('Ctrl Pts',(-10.2393197897243,13.5165956866793,2.34416579313634));
#95129=CARTESIAN_POINT('Ctrl Pts',(-10.3156143211647,13.5223803952931,2.36262900902497));
#95130=CARTESIAN_POINT('Ctrl Pts',(-10.4252140636606,13.5307941663748,2.40103689549037));
#95131=CARTESIAN_POINT('Ctrl Pts',(-10.4603045962512,13.5335013880817,2.41526630642648));
#95132=CARTESIAN_POINT('Ctrl Pts',(-10.5003710338081,13.5365637379917,2.43380883537797));
#95133=CARTESIAN_POINT('Ctrl Pts',(-10.5060685962099,13.5369984973955,2.43650136286607));
#95134=CARTESIAN_POINT('Ctrl Pts',(-10.5148093475971,13.5376640638446,2.44071817810893));
#95135=CARTESIAN_POINT('Ctrl Pts',(-10.5178678960987,13.5378966901573,2.44221009388881));
#95136=CARTESIAN_POINT('Ctrl Pts',(-10.5232202327771,13.5383032518542,2.44484966544022));
#95137=CARTESIAN_POINT('Ctrl Pts',(-10.5255167969995,13.5384775259928,2.44599158585664));
#95138=CARTESIAN_POINT('Ctrl Pts',(-10.5308953002472,13.5388852496528,2.44868788814847));
#95139=CARTESIAN_POINT('Ctrl Pts',(-10.533974159385,13.5391183276126,2.45024832735685));
#95140=CARTESIAN_POINT('Ctrl Pts',(-10.5428420864596,13.5397888599252,2.45479191402767));
#95141=CARTESIAN_POINT('Ctrl Pts',(-10.5486134412727,13.540224269579,2.45780962842987));
#95142=CARTESIAN_POINT('Ctrl Pts',(-10.5892555417729,13.5432855761932,2.47949166168329));
#95143=CARTESIAN_POINT('Ctrl Pts',(-10.6231956728638,13.5458168913886,2.49985639433537));
#95144=CARTESIAN_POINT('Ctrl Pts',(-10.7174158135842,13.5529562043275,2.56305307883562));
#95145=CARTESIAN_POINT('Ctrl Pts',(-10.774772921729,13.557452415181,2.60989744004744));
#95146=CARTESIAN_POINT('Ctrl Pts',(-10.8517997600858,13.5642348239417,2.6859292740451));
#95147=CARTESIAN_POINT('Ctrl Pts',(-10.8751677178338,13.5664102919784,2.71110509690412));
#95148=CARTESIAN_POINT('Ctrl Pts',(-10.9070131083949,13.5695854504994,2.748572987383));
#95149=CARTESIAN_POINT('Ctrl Pts',(-10.9164098423391,13.5705511176891,2.76006195871282));
#95150=CARTESIAN_POINT('Ctrl Pts',(-10.9327691432312,13.5722873004723,2.78085348886599));
#95151=CARTESIAN_POINT('Ctrl Pts',(-10.9398159786282,13.5730545146995,2.7900874069955));
#95152=CARTESIAN_POINT('Ctrl Pts',(-10.9503243732758,13.5742294399357,2.80428794430047));
#95153=CARTESIAN_POINT('Ctrl Pts',(-10.9538862569624,13.5746332992808,2.80917970110329));
#95154=CARTESIAN_POINT('Ctrl Pts',(-10.9574404349605,13.5750420709097,2.81414077341459));
#95155=CARTESIAN_POINT('Ctrl Pts',(-10.957470636241,13.5750455448327,2.81418293552434));
#95156=CARTESIAN_POINT('Ctrl Pts',(-10.9575330265506,13.5750527222008,2.8142700468687));
#95157=CARTESIAN_POINT('Ctrl Pts',(-10.9575652151999,13.5750564256604,2.81431499637541));
#95158=CARTESIAN_POINT('Ctrl Pts',(-10.9576317166497,13.5750640779739,2.81440787545273));
#95159=CARTESIAN_POINT('Ctrl Pts',(-10.9576660290411,13.5750680268471,2.81445580536678));
#95160=CARTESIAN_POINT('Ctrl Pts',(-10.9577369244382,13.5750761870469,2.81455485265486));
#95161=CARTESIAN_POINT('Ctrl Pts',(-10.9577735069255,13.5750803983895,2.81460597034783));
#95162=CARTESIAN_POINT('Ctrl Pts',(-10.9578490995345,13.5750891018361,2.81471161580256));
#95163=CARTESIAN_POINT('Ctrl Pts',(-10.9578881091097,13.5750935939635,2.81476614399078));
#95164=CARTESIAN_POINT('Ctrl Pts',(-10.9579687244699,13.5751028786568,2.81487884972569));
#95165=CARTESIAN_POINT('Ctrl Pts',(-10.9580103296226,13.5751076712482,2.81493702774705));
#95166=CARTESIAN_POINT('Ctrl Pts',(-10.9580963171636,13.5751175780247,2.81505729045284));
#95167=CARTESIAN_POINT('Ctrl Pts',(-10.9581406987863,13.5751226922339,2.81511937561826));
#95168=CARTESIAN_POINT('Ctrl Pts',(-10.9582324334248,13.5751332649644,2.8152477289804));
#95169=CARTESIAN_POINT('Ctrl Pts',(-10.9582797856225,13.5751387235199,2.81531399780552));
#95170=CARTESIAN_POINT('Ctrl Pts',(-10.9583776700008,13.5751500093831,2.81545101584856));
#95171=CARTESIAN_POINT('Ctrl Pts',(-10.9584282011931,13.5751558367238,2.81552176571005));
#95172=CARTESIAN_POINT('Ctrl Pts',(-10.9585326673003,13.5751678864106,2.81566806531123));
#95173=CARTESIAN_POINT('Ctrl Pts',(-10.9585866011312,13.5751741087998,2.81574361585117));
#95174=CARTESIAN_POINT('Ctrl Pts',(-10.9586981126653,13.5751869768063,2.81589986032844));
#95175=CARTESIAN_POINT('Ctrl Pts',(-10.9587556891234,13.5751936224723,2.81598055517396));
#95176=CARTESIAN_POINT('Ctrl Pts',(-10.9588747435295,13.5752073673585,2.81614745746432));
#95177=CARTESIAN_POINT('Ctrl Pts',(-10.9589362200376,13.5752144666327,2.81623366592729));
#95178=CARTESIAN_POINT('Ctrl Pts',(-10.9590633507186,13.5752291513047,2.81641199205616));
#95179=CARTESIAN_POINT('Ctrl Pts',(-10.9591290032387,13.5752367367637,2.81650411088112));
#95180=CARTESIAN_POINT('Ctrl Pts',(-10.9592399847994,13.5752495629612,2.81665987958547));
#95181=CARTESIAN_POINT('Ctrl Pts',(-10.9592853207868,13.5752548034373,2.81672352453131));
#95182=CARTESIAN_POINT('Ctrl Pts',(-10.9593926645419,13.5752672138162,2.81687425085038));
#95183=CARTESIAN_POINT('Ctrl Pts',(-10.959454666779,13.5752743839273,2.81696133614253));
#95184=CARTESIAN_POINT('Ctrl Pts',(-10.9596014023371,13.5752913571457,2.81716749309191));
#95185=CARTESIAN_POINT('Ctrl Pts',(-10.9596861253403,13.5753011606419,2.81728657206178));
#95186=CARTESIAN_POINT('Ctrl Pts',(-10.9598864906385,13.5753243534337,2.81756829834988));
#95187=CARTESIAN_POINT('Ctrl Pts',(-10.9600021137355,13.5753377434528,2.81773095926119));
#95188=CARTESIAN_POINT('Ctrl Pts',(-10.9604377907444,13.5753882220686,2.81834420850813));
#95189=CARTESIAN_POINT('Ctrl Pts',(-10.9607575684107,13.5754253210711,2.81879499216153));
#95190=CARTESIAN_POINT('Ctrl Pts',(-10.9640129001659,13.5758034862864,2.82339081468986));
#95191=CARTESIAN_POINT('Ctrl Pts',(-10.9669218883466,13.5761455489663,2.82755452133205));
#95192=CARTESIAN_POINT('Ctrl Pts',(-10.9736020181949,13.5769407942357,2.83724892913097));
#95193=CARTESIAN_POINT('Ctrl Pts',(-10.9773530906429,13.5773947141997,2.84279317960206));
#95194=CARTESIAN_POINT('Ctrl Pts',(-10.9894546955068,13.5788837245337,2.8610126317647));
#95195=CARTESIAN_POINT('Ctrl Pts',(-10.9976071953909,13.5799260369026,2.87381688174727));
#95196=CARTESIAN_POINT('Ctrl Pts',(-11.0476875402531,13.5865879756874,2.95593394741937));
#95197=CARTESIAN_POINT('Ctrl Pts',(-11.0826102054874,13.5924571720685,3.02924774727295));
#95198=CARTESIAN_POINT('Ctrl Pts',(-11.1283000118882,13.6024730078922,3.15778955476222));
#95199=CARTESIAN_POINT('Ctrl Pts',(-11.1431575516141,13.6065608364252,3.21127816082677));
#95200=CARTESIAN_POINT('Ctrl Pts',(-11.1574332193828,13.6117067526323,3.28157691914051));
#95201=CARTESIAN_POINT('Ctrl Pts',(-11.1603430830248,13.6128647311869,3.29760364190141));
#95202=CARTESIAN_POINT('Ctrl Pts',(-11.1646366415851,13.6147705898902,3.32440288491379));
#95203=CARTESIAN_POINT('Ctrl Pts',(-11.1662054179238,13.6155262969437,3.33514309808904));
#95204=CARTESIAN_POINT('Ctrl Pts',(-11.1681700458283,13.6165612030485,3.35002958950527));
#95205=CARTESIAN_POINT('Ctrl Pts',(-11.1686926650549,13.6168468914198,3.35415818169023));
#95206=CARTESIAN_POINT('Ctrl Pts',(-11.1695401059706,13.6173283651981,3.36115006002537));
#95207=CARTESIAN_POINT('Ctrl Pts',(-11.1698763178779,13.6175247716101,3.3640118878564));
#95208=CARTESIAN_POINT('Ctrl Pts',(-11.1704989192158,13.6178990636613,3.36948470765604));
#95209=CARTESIAN_POINT('Ctrl Pts',(-11.1707870830017,13.6180770494245,3.37209547292714));
#95210=CARTESIAN_POINT('Ctrl Pts',(-11.1714566053047,13.6185023549,3.3783532565542));
#95211=CARTESIAN_POINT('Ctrl Pts',(-11.1718296735018,13.6187492158504,3.38200116310408));
#95212=CARTESIAN_POINT('Ctrl Pts',(-11.1731166311541,13.6196383214344,3.39519367817268));
#95213=CARTESIAN_POINT('Ctrl Pts',(-11.1739310261744,13.6202753133151,3.40474793549087));
#95214=CARTESIAN_POINT('Ctrl Pts',(-11.1797107167689,13.6255083152135,3.48397661004278));
#95215=CARTESIAN_POINT('Ctrl Pts',(-11.1785858277258,13.6298210261132,3.55396616523511));
#95216=CARTESIAN_POINT('Ctrl Pts',(-11.1618892000277,13.6396630712478,3.71237768456328));
#95217=CARTESIAN_POINT('Ctrl Pts',(-11.1424217473845,13.6451804339534,3.79993435395114));
#95218=CARTESIAN_POINT('Ctrl Pts',(-11.1095616486035,13.6517881176117,3.89508847418353));
#95219=CARTESIAN_POINT('Ctrl Pts',(-11.1057321892027,13.6525322409155,3.90568246913281));
#95220=CARTESIAN_POINT('Ctrl Pts',(-11.0996424231589,13.6536782737071,3.92180234551705));
#95221=CARTESIAN_POINT('Ctrl Pts',(-11.0974910095438,13.6540765617867,3.92736887957926));
#95222=CARTESIAN_POINT('Ctrl Pts',(-11.0936603686493,13.6547745591338,3.937060516188));
#95223=CARTESIAN_POINT('Ctrl Pts',(-11.0919998612064,13.655073635123,3.94119292712881));
#95224=CARTESIAN_POINT('Ctrl Pts',(-11.0881965115769,13.6557509380498,3.95050508968752));
#95225=CARTESIAN_POINT('Ctrl Pts',(-11.086040060146,13.6561296187427,3.95567912998674));
#95226=CARTESIAN_POINT('Ctrl Pts',(-11.0801029187098,13.6571581023281,3.96964273243618));
#95227=CARTESIAN_POINT('Ctrl Pts',(-11.0762519879975,13.6578102749233,3.97840177673734));
#95228=CARTESIAN_POINT('Ctrl Pts',(-11.0573164384922,13.6609484607955,4.02008513285995));
#95229=CARTESIAN_POINT('Ctrl Pts',(-11.0408267525123,13.6634821863851,4.05234570360193));
#95230=CARTESIAN_POINT('Ctrl Pts',(-10.9836168486827,13.6717012577846,4.15258470600033));
#95231=CARTESIAN_POINT('Ctrl Pts',(-10.937518500822,13.6775515322287,4.21723446593321));
#95232=CARTESIAN_POINT('Ctrl Pts',(-10.8537452691142,13.6868594860221,4.31271255929083));
#95233=CARTESIAN_POINT('Ctrl Pts',(-10.8200361964558,13.6903339281926,4.34671383157753));
#95234=CARTESIAN_POINT('Ctrl Pts',(-10.7772152675003,13.6943536858202,4.38494233873553));
#95235=CARTESIAN_POINT('Ctrl Pts',(-10.7700038414104,13.6950181906,4.39122422205394));
#95236=CARTESIAN_POINT('Ctrl Pts',(-10.7597172660206,13.6959476884215,4.39996679403401));
#95237=CARTESIAN_POINT('Ctrl Pts',(-10.7567053065854,13.6962176684068,4.40250076718877));
#95238=CARTESIAN_POINT('Ctrl Pts',(-10.7515082887924,13.6966796915226,4.40682873042328));
#95239=CARTESIAN_POINT('Ctrl Pts',(-10.7493294022561,13.6968722543313,4.40863001383457));
#95240=CARTESIAN_POINT('Ctrl Pts',(-10.7450649958844,13.6972468851916,4.41212962207686));
#95241=CARTESIAN_POINT('Ctrl Pts',(-10.7429801459825,13.6974290089771,4.41382864838428));
#95242=CARTESIAN_POINT('Ctrl Pts',(-10.737266338376,13.697925389384,4.41845257509309));
#95243=CARTESIAN_POINT('Ctrl Pts',(-10.7336257597137,13.6982386425474,4.42136313845611));
#95244=CARTESIAN_POINT('Ctrl Pts',(-10.7194639059679,13.6994459938885,4.43254807300959));
#95245=CARTESIAN_POINT('Ctrl Pts',(-10.708818675215,13.7003297907966,4.44066484129783));
#95246=CARTESIAN_POINT('Ctrl Pts',(-10.6053827879264,13.7087173600827,4.5167792753322));
#95247=CARTESIAN_POINT('Ctrl Pts',(-10.5032289643628,13.7155346634489,4.57102605133776));
#95248=CARTESIAN_POINT('Ctrl Pts',(-10.3549969182846,13.725463620884,4.62376984473207));
#95249=CARTESIAN_POINT('Ctrl Pts',(-10.3144468292726,13.7281761767541,4.63578345379587));
#95250=CARTESIAN_POINT('Ctrl Pts',(-10.2639297692958,13.7315972382886,4.647836997508));
#95251=CARTESIAN_POINT('Ctrl Pts',(-10.2544904682267,13.732238153732,4.64996664662525));
#95252=CARTESIAN_POINT('Ctrl Pts',(-10.2394867963268,13.7332600160616,4.65315792950868));
#95253=CARTESIAN_POINT('Ctrl Pts',(-10.2339390256806,13.7336385351313,4.65429617792355));
#95254=CARTESIAN_POINT('Ctrl Pts',(-10.2234812036489,13.7343534278153,4.6563633442928));
#95255=CARTESIAN_POINT('Ctrl Pts',(-10.2185730136894,13.7346895136851,4.65730111413302));
#95256=CARTESIAN_POINT('Ctrl Pts',(-10.2075036684653,13.7354488211718,4.65934311936162));
#95257=CARTESIAN_POINT('Ctrl Pts',(-10.2013394190801,13.7358725933673,4.66042952243653));
#95258=CARTESIAN_POINT('Ctrl Pts',(-10.1855160225851,13.7369629227721,4.66308840474104));
#95259=CARTESIAN_POINT('Ctrl Pts',(-10.1758455653866,13.737631681646,4.66458969554645));
#95260=CARTESIAN_POINT('Ctrl Pts',(-10.1065625485152,13.7424411949564,4.67446294186497));
#95261=CARTESIAN_POINT('Ctrl Pts',(-10.0464136340409,13.7467200345899,4.67837280857284));
#95262=CARTESIAN_POINT('Ctrl Pts',(-9.9095344838565,13.7566576515529,4.67677323133549));
#95263=CARTESIAN_POINT('Ctrl Pts',(-9.83310517157141,13.7623545476245,4.66838565075373));
#95264=CARTESIAN_POINT('Ctrl Pts',(-9.73011173089593,13.7699350525143,4.64676478192213));
#95265=CARTESIAN_POINT('Ctrl Pts',(-9.70240777036819,13.7719622646432,4.63988960619347));
#95266=CARTESIAN_POINT('Ctrl Pts',(-9.66941238963437,13.7743417068642,4.6304160429034));
#95267=CARTESIAN_POINT('Ctrl Pts',(-9.66385799175535,13.7747410426571,4.62877683884532));
#95268=CARTESIAN_POINT('Ctrl Pts',(-9.65521195172755,13.775360512601,4.62615575446605));
#95269=CARTESIAN_POINT('Ctrl Pts',(-9.6521119858812,13.7755821870185,4.62520198712178));
#95270=CARTESIAN_POINT('Ctrl Pts',(-9.64633640990524,13.7759943340786,4.62339886385133));
#95271=CARTESIAN_POINT('Ctrl Pts',(-9.64365991029343,13.7761849794942,4.62255275288277));
#95272=CARTESIAN_POINT('Ctrl Pts',(-9.63755906893324,13.7766187613243,4.62060009980835));
#95273=CARTESIAN_POINT('Ctrl Pts',(-9.63413675550088,13.7768615403301,4.61948742707967));
#95274=CARTESIAN_POINT('Ctrl Pts',(-9.62504913291682,13.7775048749432,4.61648670794037));
#95275=CARTESIAN_POINT('Ctrl Pts',(-9.61939290317957,13.7779039019124,4.61457120151641));
#95276=CARTESIAN_POINT('Ctrl Pts',(-9.5745383056594,13.7810589832932,4.59899972014237));
#95277=CARTESIAN_POINT('Ctrl Pts',(-9.53606748865475,13.7837090559223,4.58332150630182));
#95278=CARTESIAN_POINT('Ctrl Pts',(-9.40892768768725,13.7925296261455,4.52348858821099));
#95279=CARTESIAN_POINT('Ctrl Pts',(-9.32502927893121,13.7984922310723,4.47021156070371));
#95280=CARTESIAN_POINT('Ctrl Pts',(-9.22688979229238,13.8066510846131,4.38893404794141));
#95281=CARTESIAN_POINT('Ctrl Pts',(-9.20566170672081,13.8084963334957,4.37001701294896));
#95282=CARTESIAN_POINT('Ctrl Pts',(-9.178974172662,13.8109372647052,4.34444335479706));
#95283=CARTESIAN_POINT('Ctrl Pts',(-9.17287298940522,13.8115039685292,4.33846818102104));
#95284=CARTESIAN_POINT('Ctrl Pts',(-9.16301582504219,13.8124341841259,4.32860231045058));
#95285=CARTESIAN_POINT('Ctrl Pts',(-9.15922063680212,13.8127959665367,4.32475108898084));
#95286=CARTESIAN_POINT('Ctrl Pts',(-9.15193534143306,13.8134976062578,4.31725568644012));
#95287=CARTESIAN_POINT('Ctrl Pts',(-9.148441863977,13.8138373067466,4.31361493455832));
#95288=CARTESIAN_POINT('Ctrl Pts',(-9.14043045396525,13.8146239446295,4.30515766636802));
#95289=CARTESIAN_POINT('Ctrl Pts',(-9.13592945747042,13.8150715887553,4.3003254129583));
#95290=CARTESIAN_POINT('Ctrl Pts',(-9.12149239871536,13.8165262068976,4.28456208646076));
#95291=CARTESIAN_POINT('Ctrl Pts',(-9.11172162932854,13.8175400017292,4.27348223941367));
#95292=CARTESIAN_POINT('Ctrl Pts',(-9.04501330910967,13.8246736787696,4.1949050630136));
#95293=CARTESIAN_POINT('Ctrl Pts',(-8.995626923395,13.8310972106859,4.1213868490978));
#95294=CARTESIAN_POINT('Ctrl Pts',(-8.92286403594545,13.8426862350412,3.98136041730383));
#95295=CARTESIAN_POINT('Ctrl Pts',(-8.89632618578527,13.8477973819049,3.91693644362181));
#95296=CARTESIAN_POINT('Ctrl Pts',(-8.87348693407732,13.8531387845478,3.84367869390256));
#95297=CARTESIAN_POINT('Ctrl Pts',(-8.87141027540495,13.8536360632117,3.83679663350687));
#95298=CARTESIAN_POINT('Ctrl Pts',(-8.86840942961839,13.8543720453029,3.82651227589115));
#95299=CARTESIAN_POINT('Ctrl Pts',(-8.8674373431335,13.8546133515125,3.82312430174083));
#95300=CARTESIAN_POINT('Ctrl Pts',(-8.8657961656235,13.855025731446,3.81730596949489));
#95301=CARTESIAN_POINT('Ctrl Pts',(-8.86511965278477,13.8551972259385,3.81487777651457));
#95302=CARTESIAN_POINT('Ctrl Pts',(-8.86359991743127,13.8555859293475,3.80935449702826));
#95303=CARTESIAN_POINT('Ctrl Pts',(-8.86276154060812,13.8558028585223,3.80625812576336));
#95304=CARTESIAN_POINT('Ctrl Pts',(-8.86051264451303,13.8563917600933,3.79781571158757));
#95305=CARTESIAN_POINT('Ctrl Pts',(-8.85912708047707,13.8567623413735,3.79246301624323));
#95306=CARTESIAN_POINT('Ctrl Pts',(-8.85240486067107,13.8586009027975,3.76571887764112));
#95307=CARTESIAN_POINT('Ctrl Pts',(-8.84763150986869,13.8600396522329,3.74418873900679));
#95308=CARTESIAN_POINT('Ctrl Pts',(-8.83929991925633,13.8628740845775,3.70088882330947));
#95309=CARTESIAN_POINT('Ctrl Pts',(-8.83574307899585,13.8642692075345,3.67912820921873));
#95310=CARTESIAN_POINT('Ctrl Pts',(-8.81951972453853,13.8718885244967,3.55873166698399));
#95311=CARTESIAN_POINT('Ctrl Pts',(-8.81877412799166,13.8778773812607,3.45890256575597));
#95312=CARTESIAN_POINT('Ctrl Pts',(-8.83384492767943,13.8860128287073,3.33286768864652));
#95313=CARTESIAN_POINT('Ctrl Pts',(-8.83806359829453,13.8877986916465,3.30569490219117));
#95314=CARTESIAN_POINT('Ctrl Pts',(-8.84481367003323,13.8901713674797,3.27041178464878));
#95315=CARTESIAN_POINT('Ctrl Pts',(-8.84648748461026,13.8907311671799,3.26214484186287));
#95316=CARTESIAN_POINT('Ctrl Pts',(-8.84937393933931,13.8916525775312,3.24863638678061));
#95317=CARTESIAN_POINT('Ctrl Pts',(-8.8505339738379,13.8920125148162,3.24338384582235));
#95318=CARTESIAN_POINT('Ctrl Pts',(-8.85285201063279,13.8927123750817,3.23321914989296));
#95319=CARTESIAN_POINT('Ctrl Pts',(-8.85400568666601,13.8930521533253,3.22830612091752));
#95320=CARTESIAN_POINT('Ctrl Pts',(-8.85675126789243,13.893841612703,3.21694251054581));
#95321=CARTESIAN_POINT('Ctrl Pts',(-8.85836624035557,13.8942920221327,3.21049773490765));
#95322=CARTESIAN_POINT('Ctrl Pts',(-8.86381274788838,13.8957672421158,3.18951722155798));
#95323=CARTESIAN_POINT('Ctrl Pts',(-8.86786791994183,13.8967991633061,3.17504162658661));
#95324=CARTESIAN_POINT('Ctrl Pts',(-8.89567888278933,13.9034819468154,3.08261473276687));
#95325=CARTESIAN_POINT('Ctrl Pts',(-8.92718991450157,13.9093869741405,3.00724294296085));
#95326=CARTESIAN_POINT('Ctrl Pts',(-8.99234167440492,13.9193681275152,2.88787836535474));
#95327=CARTESIAN_POINT('Ctrl Pts',(-9.02175873092889,13.9233853947298,2.84188694652679));
#95328=CARTESIAN_POINT('Ctrl Pts',(-9.0638617489985,13.9284507956855,2.78515741740613));
#95329=CARTESIAN_POINT('Ctrl Pts',(-9.07373064219927,13.9295960702767,2.77241503962706));
#95330=CARTESIAN_POINT('Ctrl Pts',(-9.09062058950655,13.9314827335434,2.75150822335539));
#95331=CARTESIAN_POINT('Ctrl Pts',(-9.09749743467583,13.9322317757757,2.74323055548128));
#95332=CARTESIAN_POINT('Ctrl Pts',(-9.10717724766102,13.9332587311535,2.73189860642526));
#95333=CARTESIAN_POINT('Ctrl Pts',(-9.109884075508,13.9335430220645,2.72876342139365));
#95334=CARTESIAN_POINT('Ctrl Pts',(-9.11449743501834,13.934022600436,2.72347663714609));
#95335=CARTESIAN_POINT('Ctrl Pts',(-9.11639539096728,13.9342185015318,2.72131763777697));
#95336=CARTESIAN_POINT('Ctrl Pts',(-9.12005448079591,13.9345934720572,2.7171858850478));
#95337=CARTESIAN_POINT('Ctrl Pts',(-9.1218143695892,13.9347726335102,2.71521209602311));
#95338=CARTESIAN_POINT('Ctrl Pts',(-9.12605217987942,13.9352012684823,2.7104913199606));
#95339=CARTESIAN_POINT('Ctrl Pts',(-9.1285364448156,13.9354502765422,2.70775002615424));
#95340=CARTESIAN_POINT('Ctrl Pts',(-9.13761476888779,13.9363522463308,2.69782680458505));
#95341=CARTESIAN_POINT('Ctrl Pts',(-9.14428524894664,13.9369998050882,2.69071488192203));
#95342=CARTESIAN_POINT('Ctrl Pts',(-9.19362088137094,13.9416872011651,2.63940641375144));
#95343=CARTESIAN_POINT('Ctrl Pts',(-9.23960328365098,13.9455113311542,2.59851930416609));
#95344=CARTESIAN_POINT('Ctrl Pts',(-9.34179465846534,13.9534495045036,2.52106134062607));
#95345=CARTESIAN_POINT('Ctrl Pts',(-9.39834918957576,13.9575489475891,2.48532229443791));
#95346=CARTESIAN_POINT('Ctrl Pts',(-9.48841018205785,13.9639993488808,2.43859825527454));
#95347=CARTESIAN_POINT('Ctrl Pts',(-9.51988218467226,13.966238642925,2.42399613012846));
#95348=CARTESIAN_POINT('Ctrl Pts',(-9.56037982440296,13.9691265666893,2.40733708591038));
#95349=CARTESIAN_POINT('Ctrl Pts',(-9.56884908011646,13.969730814859,2.40396760122025));
#95350=CARTESIAN_POINT('Ctrl Pts',(-9.58252058453984,13.9707071043735,2.39871138615557));
#95351=CARTESIAN_POINT('Ctrl Pts',(-9.58769861987652,13.9710770709956,2.39676238122097));
#95352=CARTESIAN_POINT('Ctrl Pts',(-9.59758876495487,13.9717841870312,2.39311909694426));
#95353=CARTESIAN_POINT('Ctrl Pts',(-9.6022983353999,13.9721211100489,2.39141823924401));
#95354=CARTESIAN_POINT('Ctrl Pts',(-9.61309449953994,13.9728940032584,2.38759686327273));
#95355=CARTESIAN_POINT('Ctrl Pts',(-9.61918789655179,13.9733306141381,2.38549618938032));
#95356=CARTESIAN_POINT('Ctrl Pts',(-9.63812054231927,13.9746885706761,2.37914262674409));
#95357=CARTESIAN_POINT('Ctrl Pts',(-9.65101564356648,13.9756154411713,2.37506094142421));
#95358=CARTESIAN_POINT('Ctrl Pts',(-9.71230321476705,13.9800316165875,2.35681675951342));
#95359=CARTESIAN_POINT('Ctrl Pts',(-9.76144827564538,13.9836081681662,2.34556553370857));
#95360=CARTESIAN_POINT('Ctrl Pts',(-9.81110406371067,13.9872487449619,2.3374969300026));
#95361=CARTESIAN_POINT('Origin',(-10.,12.3756328852638,3.5));
#95362=CARTESIAN_POINT('',(-9.81110404096668,14.5872589185639,2.33749693369829));
#95363=CARTESIAN_POINT('',(-9.81110406371066,14.4889165240206,2.3374969300026));
#95364=CARTESIAN_POINT('',(-9.81110406371068,12.3756328852638,2.3374969300026));
#95365=CARTESIAN_POINT('Ctrl Pts',(-9.81110404084991,14.5872589202102,2.33749693371726));
#95366=CARTESIAN_POINT('Ctrl Pts',(-9.73264000287283,14.5815501908489,2.35024661166853));
#95367=CARTESIAN_POINT('Ctrl Pts',(-9.65565256030276,14.5756541343893,2.37091040782615));
#95368=CARTESIAN_POINT('Ctrl Pts',(-9.54248844072707,14.566835354911,2.41394988717991));
#95369=CARTESIAN_POINT('Ctrl Pts',(-9.50445426554587,14.5638473808157,2.4307680800128));
#95370=CARTESIAN_POINT('Ctrl Pts',(-9.46175911294319,14.560523640647,2.45241630542129));
#95371=CARTESIAN_POINT('Ctrl Pts',(-9.45615611418438,14.5600881018448,2.45531407497928));
#95372=CARTESIAN_POINT('Ctrl Pts',(-9.4476170202585,14.5594256245441,2.45981765969876));
#95373=CARTESIAN_POINT('Ctrl Pts',(-9.44466414517122,14.5591967743601,2.46139114849266));
#95374=CARTESIAN_POINT('Ctrl Pts',(-9.43926218842847,14.5587786122528,2.46429929617265));
#95375=CARTESIAN_POINT('Ctrl Pts',(-9.43681114171983,14.5585890714669,2.46563007028998));
#95376=CARTESIAN_POINT('Ctrl Pts',(-9.43129738739931,14.5581631114296,2.46864912345498));
#95377=CARTESIAN_POINT('Ctrl Pts',(-9.42823745994013,14.557927007139,2.47034234295588));
#95378=CARTESIAN_POINT('Ctrl Pts',(-9.42037562274466,14.5573210099128,2.474738566366));
#95379=CARTESIAN_POINT('Ctrl Pts',(-9.41558499322758,14.5569523458842,2.47746172258458));
#95380=CARTESIAN_POINT('Ctrl Pts',(-9.38510554727746,14.5546094912099,2.49507145204672));
#95381=CARTESIAN_POINT('Ctrl Pts',(-9.35996585795815,14.5526893191643,2.51089271967742));
#95382=CARTESIAN_POINT('Ctrl Pts',(-9.26634638223819,14.5454794389545,2.57487673608849));
#95383=CARTESIAN_POINT('Ctrl Pts',(-9.20247190936922,14.5404184714153,2.62933851271936));
#95384=CARTESIAN_POINT('Ctrl Pts',(-9.12061717821991,14.532972886158,2.7157623252128));
#95385=CARTESIAN_POINT('Ctrl Pts',(-9.09749400375314,14.530738680265,2.74248728932871));
#95386=CARTESIAN_POINT('Ctrl Pts',(-9.0662397686027,14.5274852900465,2.78207558837813));
#95387=CARTESIAN_POINT('Ctrl Pts',(-9.0571013367366,14.5265024860349,2.79412061263111));
#95388=CARTESIAN_POINT('Ctrl Pts',(-9.04120268350903,14.5247321993151,2.81593580783669));
#95389=CARTESIAN_POINT('Ctrl Pts',(-9.03435356697208,14.5239481248307,2.82563877433802));
#95390=CARTESIAN_POINT('Ctrl Pts',(-9.02419888976221,14.5227515617678,2.84049661202843));
#95391=CARTESIAN_POINT('Ctrl Pts',(-9.02078472668893,14.5223431556051,2.8455766113511));
#95392=CARTESIAN_POINT('Ctrl Pts',(-9.01466695704583,14.521600025742,2.85483442564166));
#95393=CARTESIAN_POINT('Ctrl Pts',(-9.01194991969964,14.5212658114497,2.85900322825458));
#95394=CARTESIAN_POINT('Ctrl Pts',(-9.00615673021706,14.5205440661581,2.86801618272543));
#95395=CARTESIAN_POINT('Ctrl Pts',(-9.00308941099939,14.5201562209205,2.87286583117512));
#95396=CARTESIAN_POINT('Ctrl Pts',(-8.99488133353557,14.5191026229107,2.88605577197509));
#95397=CARTESIAN_POINT('Ctrl Pts',(-8.98980910245449,14.5184344028053,2.89443795593845));
#95398=CARTESIAN_POINT('Ctrl Pts',(-8.96438691808017,14.5149948828639,2.93765812262217));
#95399=CARTESIAN_POINT('Ctrl Pts',(-8.94573446475574,14.5121640843382,2.97345811443405));
#95400=CARTESIAN_POINT('Ctrl Pts',(-8.89335665811802,14.5031613765447,3.08797857263325));
#95401=CARTESIAN_POINT('Ctrl Pts',(-8.86634984066145,14.496809411726,3.16946136577115));
#95402=CARTESIAN_POINT('Ctrl Pts',(-8.84054923377066,14.4878467864521,3.2898183750055));
#95403=CARTESIAN_POINT('Ctrl Pts',(-8.83444225197902,14.4851474660677,3.32685813938582));
#95404=CARTESIAN_POINT('Ctrl Pts',(-8.82913102193451,14.481932028478,3.37258951061053));
#95405=CARTESIAN_POINT('Ctrl Pts',(-8.82824025575684,14.481341377353,3.38106006174251));
#95406=CARTESIAN_POINT('Ctrl Pts',(-8.82708727728855,14.4804957438544,3.39329917761145));
#95407=CARTESIAN_POINT('Ctrl Pts',(-8.82675120554481,14.4802369409126,3.3970602705151));
#95408=CARTESIAN_POINT('Ctrl Pts',(-8.82619613198177,14.4797869049151,3.40362848453897));
#95409=CARTESIAN_POINT('Ctrl Pts',(-8.82596909934797,14.4795952350433,3.40643486458907));
#95410=CARTESIAN_POINT('Ctrl Pts',(-8.82550866394301,14.4791896966777,3.41239209149528));
#95411=CARTESIAN_POINT('Ctrl Pts',(-8.82527787407733,14.4789759730277,3.41554307862269));
#95412=CARTESIAN_POINT('Ctrl Pts',(-8.82468395314806,14.4783958551932,3.42412584259327));
#95413=CARTESIAN_POINT('Ctrl Pts',(-8.82434579237486,14.4780308109477,3.4295593533412));
#95414=CARTESIAN_POINT('Ctrl Pts',(-8.8229250170195,14.4763136658107,3.45526154763617));
#95415=CARTESIAN_POINT('Ctrl Pts',(-8.82232873498976,14.4749861523923,3.47555502651146));
#95416=CARTESIAN_POINT('Ctrl Pts',(-8.82187983523047,14.466762875616,3.60311004156625));
#95417=CARTESIAN_POINT('Ctrl Pts',(-8.83615443400348,14.4603707737357,3.70992193752649));
#95418=CARTESIAN_POINT('Ctrl Pts',(-8.87573150267509,14.4509768423277,3.85332168356678));
#95419=CARTESIAN_POINT('Ctrl Pts',(-8.88887151538865,14.4483130949146,3.89269424801518));
#95420=CARTESIAN_POINT('Ctrl Pts',(-8.90757945971336,14.4449476375499,3.94023267430271));
#95421=CARTESIAN_POINT('Ctrl Pts',(-8.91120844680046,14.4443109870414,3.94913293022181));
#95422=CARTESIAN_POINT('Ctrl Pts',(-8.91713951200369,14.4432949032357,3.96318468038759));
#95423=CARTESIAN_POINT('Ctrl Pts',(-8.91937042827779,14.4429178632868,3.96836589483924));
#95424=CARTESIAN_POINT('Ctrl Pts',(-8.92364343451001,14.4422051398109,3.97809672030202));
#95425=CARTESIAN_POINT('Ctrl Pts',(-8.92567737296342,14.4418697387309,3.98264979204127));
#95426=CARTESIAN_POINT('Ctrl Pts',(-8.9303290908312,14.4411111536934,3.99288779552198));
#95427=CARTESIAN_POINT('Ctrl Pts',(-8.93296337693814,14.4406874139692,3.99856501613632));
#95428=CARTESIAN_POINT('Ctrl Pts',(-8.93984186190897,14.4395955920379,4.01308477468371));
#95429=CARTESIAN_POINT('Ctrl Pts',(-8.94415142862732,14.4389252845774,4.02189562937801));
#95430=CARTESIAN_POINT('Ctrl Pts',(-8.97624552973583,14.4340295424099,4.08548669269776));
#95431=CARTESIAN_POINT('Ctrl Pts',(-9.00816324131603,14.4296595554093,4.13806388105814));
#95432=CARTESIAN_POINT('Ctrl Pts',(-9.08854031040138,14.419658475103,4.2497624626265));
#95433=CARTESIAN_POINT('Ctrl Pts',(-9.13894833428935,14.4139960358093,4.30715071585918));
#95434=CARTESIAN_POINT('Ctrl Pts',(-9.21531167254281,14.4064546780836,4.37873169194922));
#95435=CARTESIAN_POINT('Ctrl Pts',(-9.23677802794976,14.4044321151721,4.39743951654077));
#95436=CARTESIAN_POINT('Ctrl Pts',(-9.2633893762249,14.4020586383702,4.41898485868214));
#95437=CARTESIAN_POINT('Ctrl Pts',(-9.26790236514378,14.4016605694306,4.42258410890734));
#95438=CARTESIAN_POINT('Ctrl Pts',(-9.27498271756564,14.4010431780308,4.42814624045627));
#95439=CARTESIAN_POINT('Ctrl Pts',(-9.27753192946841,14.4008223167546,4.43013192139706));
#95440=CARTESIAN_POINT('Ctrl Pts',(-9.28230582032924,14.4004114125545,4.43381902447509));
#95441=CARTESIAN_POINT('Ctrl Pts',(-9.28452837927286,14.4002211993335,4.43552299072252));
#95442=CARTESIAN_POINT('Ctrl Pts',(-9.28961498517904,14.3997883240167,4.43939400213159));
#95443=CARTESIAN_POINT('Ctrl Pts',(-9.29248288275444,14.3995460192511,4.44155588797786));
#95444=CARTESIAN_POINT('Ctrl Pts',(-9.30013106146574,14.3989043528509,4.44726658089956));
#95445=CARTESIAN_POINT('Ctrl Pts',(-9.30492851287194,14.3985065116086,4.45079237367361));
#95446=CARTESIAN_POINT('Ctrl Pts',(-9.34307555762783,14.3953778621256,4.47838474720255));
#95447=CARTESIAN_POINT('Ctrl Pts',(-9.37764224990899,14.3927512729352,4.50072877069635));
#95448=CARTESIAN_POINT('Ctrl Pts',(-9.49828100304296,14.3840154862437,4.57003546326752));
#95449=CARTESIAN_POINT('Ctrl Pts',(-9.58900820655437,14.3781136227497,4.60805425962421));
#95450=CARTESIAN_POINT('Ctrl Pts',(-9.71199951890322,14.3699505493562,4.64238021054537));
#95451=CARTESIAN_POINT('Ctrl Pts',(-9.74089044610851,14.3680252040898,4.64927752374096));
#95452=CARTESIAN_POINT('Ctrl Pts',(-9.7785090328746,14.3654930393325,4.6567678779022));
#95453=CARTESIAN_POINT('Ctrl Pts',(-9.78702697339062,14.3649180666082,4.65836637344915));
#95454=CARTESIAN_POINT('Ctrl Pts',(-9.8009133653959,14.3639777425019,4.66081398410473));
#95455=CARTESIAN_POINT('Ctrl Pts',(-9.80627152323963,14.3636141956293,4.6617202199232));
#95456=CARTESIAN_POINT('Ctrl Pts',(-9.81660584461781,14.3629115536109,4.66339460081994));
#95457=CARTESIAN_POINT('Ctrl Pts',(-9.82158104883559,14.3625726313256,4.66416798184521));
#95458=CARTESIAN_POINT('Ctrl Pts',(-9.83302771798309,14.3617912863312,4.66587223359262));
#95459=CARTESIAN_POINT('Ctrl Pts',(-9.83950223165438,14.3613481863132,4.66678115830852));
#95460=CARTESIAN_POINT('Ctrl Pts',(-9.85687772268891,14.3601558057525,4.66907305895338));
#95461=CARTESIAN_POINT('Ctrl Pts',(-9.8677908216153,14.3594034823178,4.67035743358119));
#95462=CARTESIAN_POINT('Ctrl Pts',(-9.96419430095064,14.3527257314768,4.68033773816634));
#95463=CARTESIAN_POINT('Ctrl Pts',(-10.050363621197,14.3465069882368,4.67980387788985));
#95464=CARTESIAN_POINT('Ctrl Pts',(-10.189721208297,14.3362107372443,4.66364062834722));
#95465=CARTESIAN_POINT('Ctrl Pts',(-10.2432553713255,14.3322039410379,4.65363817832549));
#95466=CARTESIAN_POINT('Ctrl Pts',(-10.311488669028,14.3271498289074,4.63592647942645));
#95467=CARTESIAN_POINT('Ctrl Pts',(-10.3269850636592,14.3260059201405,4.63156306955655));
#95468=CARTESIAN_POINT('Ctrl Pts',(-10.3526776703631,14.324121049715,4.62375672489656));
#95469=CARTESIAN_POINT('Ctrl Pts',(-10.3629245853431,14.3233724665536,4.62048939390675));
#95470=CARTESIAN_POINT('Ctrl Pts',(-10.3770566629269,14.3223457842745,4.61576902245199));
#95471=CARTESIAN_POINT('Ctrl Pts',(-10.3809806915762,14.3220613244956,4.61443526168062));
#95472=CARTESIAN_POINT('Ctrl Pts',(-10.3876172557555,14.3215813719677,4.61214037156372));
#95473=CARTESIAN_POINT('Ctrl Pts',(-10.3903334349332,14.3213852658928,4.61118997172978));
#95474=CARTESIAN_POINT('Ctrl Pts',(-10.3955403583679,14.3210099915795,4.60934660413308));
#95475=CARTESIAN_POINT('Ctrl Pts',(-10.3980316021944,14.3208307308099,4.60845518953512));
#95476=CARTESIAN_POINT('Ctrl Pts',(-10.4040027081984,14.3204017170422,4.60629588757482));
#95477=CARTESIAN_POINT('Ctrl Pts',(-10.4074796626152,14.3201524311404,4.60501995664189));
#95478=CARTESIAN_POINT('Ctrl Pts',(-10.4201117850419,14.3192484721804,4.6003166420171));
#95479=CARTESIAN_POINT('Ctrl Pts',(-10.4292305172535,14.3185992334928,4.59679159507934));
#95480=CARTESIAN_POINT('Ctrl Pts',(-10.4943381814432,14.3139801973661,4.57068638787015));
#95481=CARTESIAN_POINT('Ctrl Pts',(-10.5485691008014,14.3102184417342,4.54394130243486));
#95482=CARTESIAN_POINT('Ctrl Pts',(-10.6452222952771,14.3032610814468,4.48665298970563));
#95483=CARTESIAN_POINT('Ctrl Pts',(-10.6881248406501,14.300067138377,4.45722512778002));
#95484=CARTESIAN_POINT('Ctrl Pts',(-10.7543034527767,14.2947795072184,4.40507672135662));
#95485=CARTESIAN_POINT('Ctrl Pts',(-10.7788297166669,14.2927302248712,4.38405972772681));
#95486=CARTESIAN_POINT('Ctrl Pts',(-10.8179429628558,14.2892768660397,4.34765074966016));
#95487=CARTESIAN_POINT('Ctrl Pts',(-10.8330336614378,14.2878947452755,4.33282489931588));
#95488=CARTESIAN_POINT('Ctrl Pts',(-10.8530453213413,14.2859871013514,4.31207614809921));
#95489=CARTESIAN_POINT('Ctrl Pts',(-10.8583201137776,14.2854768522161,4.30649895734428));
#95490=CARTESIAN_POINT('Ctrl Pts',(-10.8670914668152,14.2846155292308,4.29704123427556));
#95491=CARTESIAN_POINT('Ctrl Pts',(-10.87061746483,14.28426571181,4.29318823074503));
#95492=CARTESIAN_POINT('Ctrl Pts',(-10.8775300331416,14.2835727227812,4.285532958229));
#95493=CARTESIAN_POINT('Ctrl Pts',(-10.880917806817,14.2832296122469,4.28173192576248));
#95494=CARTESIAN_POINT('Ctrl Pts',(-10.8883325728885,14.28247084347,4.27330326081019));
#95495=CARTESIAN_POINT('Ctrl Pts',(-10.8923482496271,14.2820547318367,4.26866591712193));
#95496=CARTESIAN_POINT('Ctrl Pts',(-10.9060170551065,14.2806202331725,4.25262957441468));
#95497=CARTESIAN_POINT('Ctrl Pts',(-10.915489109805,14.2795945958962,4.24107883153981));
#95498=CARTESIAN_POINT('Ctrl Pts',(-10.9701801319536,14.2734789660804,4.17173655161925));
#95499=CARTESIAN_POINT('Ctrl Pts',(-11.0101300409236,14.2681871430813,4.1100109374925));
#95500=CARTESIAN_POINT('Ctrl Pts',(-11.0813607104884,14.2569090456861,3.97354749953727));
#95501=CARTESIAN_POINT('Ctrl Pts',(-11.1112207757846,14.250934765998,3.89847034186178));
#95502=CARTESIAN_POINT('Ctrl Pts',(-11.135657489991,14.2446599959377,3.81218533621349));
#95503=CARTESIAN_POINT('Ctrl Pts',(-11.1380322124491,14.2440289071239,3.80341442745451));
#95504=CARTESIAN_POINT('Ctrl Pts',(-11.1412055172124,14.2431553772587,3.79113223984228));
#95505=CARTESIAN_POINT('Ctrl Pts',(-11.1420897950362,14.2429084116384,3.78764372846369));
#95506=CARTESIAN_POINT('Ctrl Pts',(-11.143589865252,14.2424832902934,3.78160990698921));
#95507=CARTESIAN_POINT('Ctrl Pts',(-11.1442131781064,14.2423047159504,3.77906652076811));
#95508=CARTESIAN_POINT('Ctrl Pts',(-11.1455098777837,14.2419291324763,3.77369803927709));
#95509=CARTESIAN_POINT('Ctrl Pts',(-11.1461813071118,14.2417322405769,3.77087249466002));
#95510=CARTESIAN_POINT('Ctrl Pts',(-11.1478159194166,14.2412467709209,3.76387872031982));
#95511=CARTESIAN_POINT('Ctrl Pts',(-11.1487668683433,14.2409588802991,3.75970761930416));
#95512=CARTESIAN_POINT('Ctrl Pts',(-11.1522262548034,14.2398904122838,3.74414303342827));
#95513=CARTESIAN_POINT('Ctrl Pts',(-11.1545881917732,14.2391176247597,3.73271720174538));
#95514=CARTESIAN_POINT('Ctrl Pts',(-11.170645175723,14.2335115634591,3.64876801158867));
#95515=CARTESIAN_POINT('Ctrl Pts',(-11.1776676828325,14.2289782333121,3.57512540585017));
#95516=CARTESIAN_POINT('Ctrl Pts',(-11.1778343182737,14.2196579903429,3.4243659146739));
#95517=CARTESIAN_POINT('Ctrl Pts',(-11.1703809414087,14.2148850839714,3.34761672360479));
#95518=CARTESIAN_POINT('Ctrl Pts',(-11.1525760591207,14.2088833636551,3.25732374774894));
#95519=CARTESIAN_POINT('Ctrl Pts',(-11.1493682062061,14.2078898815263,3.2425586900629));
#95520=CARTESIAN_POINT('Ctrl Pts',(-11.1443378381732,14.2064453880234,3.22137773996852));
#95521=CARTESIAN_POINT('Ctrl Pts',(-11.1427433951577,14.2060016082332,3.21490881912036));
#95522=CARTESIAN_POINT('Ctrl Pts',(-11.1398428676096,14.205218040621,3.20355632657173));
#95523=CARTESIAN_POINT('Ctrl Pts',(-11.13856005592,14.2048790041677,3.1986669416483));
#95524=CARTESIAN_POINT('Ctrl Pts',(-11.1358464168614,14.20417686628,3.18858877735184));
#95525=CARTESIAN_POINT('Ctrl Pts',(-11.1344114177484,14.2038136377548,3.18340125409942));
#95526=CARTESIAN_POINT('Ctrl Pts',(-11.1306382009037,14.2028786519867,3.170116144415));
#95527=CARTESIAN_POINT('Ctrl Pts',(-11.1282485588497,14.2023052489765,3.16203360738232));
#95528=CARTESIAN_POINT('Ctrl Pts',(-11.1177310394658,14.1998577387704,3.12781520676106));
#95529=CARTESIAN_POINT('Ctrl Pts',(-11.1087807353527,14.1979572603398,3.10194314153882));
#95530=CARTESIAN_POINT('Ctrl Pts',(-11.0630907116562,14.1890086969138,2.98340806077523));
#95531=CARTESIAN_POINT('Ctrl Pts',(-11.0155856838082,14.1816147802925,2.89534404959143));
#95532=CARTESIAN_POINT('Ctrl Pts',(-10.9447216564346,14.1727423995181,2.79637820105156));
#95533=CARTESIAN_POINT('Ctrl Pts',(-10.9313632835441,14.1711432197283,2.77878909356808));
#95534=CARTESIAN_POINT('Ctrl Pts',(-10.9037640573488,14.167994227367,2.74449566162142));
#95535=CARTESIAN_POINT('Ctrl Pts',(-10.8895345617414,14.1664447361073,2.72779232639233));
#95536=CARTESIAN_POINT('Ctrl Pts',(-10.8711474158172,14.1645420760754,2.70739180168754));
#95537=CARTESIAN_POINT('Ctrl Pts',(-10.8674202359574,14.1641612841618,2.70331454552107));
#95538=CARTESIAN_POINT('Ctrl Pts',(-10.8614826587253,14.1635625439229,2.69691034814909));
#95539=CARTESIAN_POINT('Ctrl Pts',(-10.8592912594282,14.1633432342188,2.69456602238922));
#95540=CARTESIAN_POINT('Ctrl Pts',(-10.8553597161028,14.1629527912163,2.69039442621587));
#95541=CARTESIAN_POINT('Ctrl Pts',(-10.8536232908956,14.1627813898922,2.68856380013272));
#95542=CARTESIAN_POINT('Ctrl Pts',(-10.8494426876443,14.1623712008741,2.68418467093694));
#95543=CARTESIAN_POINT('Ctrl Pts',(-10.8469929177981,14.1621328450294,2.68164156462753));
#95544=CARTESIAN_POINT('Ctrl Pts',(-10.8395029468061,14.1614100305416,2.67393588673134));
#95545=CARTESIAN_POINT('Ctrl Pts',(-10.8344265965686,14.1609282501319,2.66880845871165));
#95546=CARTESIAN_POINT('Ctrl Pts',(-10.7795990552481,14.1558063571191,2.61443780877662));
#95547=CARTESIAN_POINT('Ctrl Pts',(-10.7255913048443,14.1514675998386,2.56966922032444));
#95548=CARTESIAN_POINT('Ctrl Pts',(-10.5958008768419,14.1417215395552,2.48030243568998));
#95549=CARTESIAN_POINT('Ctrl Pts',(-10.5183800343025,14.1363337793593,2.43884886398708));
#95550=CARTESIAN_POINT('Ctrl Pts',(-10.4233475476614,14.1296562862507,2.40086817281709));
#95551=CARTESIAN_POINT('Ctrl Pts',(-10.4095085243001,14.1286831545855,2.39563744349147));
#95552=CARTESIAN_POINT('Ctrl Pts',(-10.3893517944854,14.1272629752923,2.38844977740205));
#95553=CARTESIAN_POINT('Ctrl Pts',(-10.3831099973379,14.1268228186416,2.38628305024445));
#95554=CARTESIAN_POINT('Ctrl Pts',(-10.3720698246499,14.1260434689013,2.38255444481612));
#95555=CARTESIAN_POINT('Ctrl Pts',(-10.3672789828027,14.1257050018039,2.38097065693091));
#95556=CARTESIAN_POINT('Ctrl Pts',(-10.3573358331121,14.1250018984862,2.37775431590113));
#95557=CARTESIAN_POINT('Ctrl Pts',(-10.3521821782253,14.1246371220853,2.37612634840046));
#95558=CARTESIAN_POINT('Ctrl Pts',(-10.3388654028385,14.1236935641894,2.37202035602145));
#95559=CARTESIAN_POINT('Ctrl Pts',(-10.3306863547233,14.1231130782288,2.36959548541245));
#95560=CARTESIAN_POINT('Ctrl Pts',(-10.2952191691576,14.1205912410778,2.35949826835654));
#95561=CARTESIAN_POINT('Ctrl Pts',(-10.2676873751124,14.1186214777836,2.35272418820644));
#95562=CARTESIAN_POINT('Ctrl Pts',(-10.1430641459899,14.1096442071177,2.32679114032415));
#95563=CARTESIAN_POINT('Ctrl Pts',(-10.0440427943208,14.1023015267758,2.31892384650854));
#95564=CARTESIAN_POINT('Ctrl Pts',(-9.9035096090453,14.0920496315411,2.32546654411423));
#95565=CARTESIAN_POINT('Ctrl Pts',(-9.86191931004656,14.0890442405331,2.32962665928955));
#95566=CARTESIAN_POINT('Ctrl Pts',(-9.81745516870227,14.0859176075736,2.33647828112878));
#95567=CARTESIAN_POINT('Ctrl Pts',(-9.81427858297399,14.0856947208985,2.33698110014891));
#95568=CARTESIAN_POINT('Ctrl Pts',(-9.81110406370735,14.0854724903439,2.33749693000314));
#95569=CARTESIAN_POINT('Ctrl Pts',(-9.81110406371067,13.9872487449619,2.3374969300026));
#95570=CARTESIAN_POINT('Ctrl Pts',(-9.86124441765218,13.9909248483166,2.32934958884876));
#95571=CARTESIAN_POINT('Ctrl Pts',(-9.9119055057115,13.9946661155459,2.32444717642581));
#95572=CARTESIAN_POINT('Ctrl Pts',(-10.0208057350382,14.0026584757658,2.32100320952519));
#95573=CARTESIAN_POINT('Ctrl Pts',(-10.0789026720657,14.0068920700218,2.32346173844195));
#95574=CARTESIAN_POINT('Ctrl Pts',(-10.1437676225063,14.0114381200553,2.33103541673644));
#95575=CARTESIAN_POINT('Ctrl Pts',(-10.1509405615333,14.0119382666453,2.33193995032179));
#95576=CARTESIAN_POINT('Ctrl Pts',(-10.161607551557,14.0126777724616,2.33338500128518));
#95577=CARTESIAN_POINT('Ctrl Pts',(-10.1651080690645,14.0129197649254,2.33387527155025));
#95578=CARTESIAN_POINT('Ctrl Pts',(-10.1711042591549,14.0133330466796,2.33474261859003));
#95579=CARTESIAN_POINT('Ctrl Pts',(-10.1736009802462,14.0135047600154,2.33511196566433));
#95580=CARTESIAN_POINT('Ctrl Pts',(-10.1792675158447,14.0138936266207,2.33596885561682));
#95581=CARTESIAN_POINT('Ctrl Pts',(-10.1824365385879,14.0141105020084,2.33646132108109));
#95582=CARTESIAN_POINT('Ctrl Pts',(-10.1910511306301,14.014698517306,2.33783608737362));
#95583=CARTESIAN_POINT('Ctrl Pts',(-10.1964926607555,14.0150682766817,2.33874372700941));
#95584=CARTESIAN_POINT('Ctrl Pts',(-10.2234585441452,14.0168932601214,2.34343657468214));
#95585=CARTESIAN_POINT('Ctrl Pts',(-10.2448825682992,14.0183198153569,2.34778241932385));
#95586=CARTESIAN_POINT('Ctrl Pts',(-10.2876817824523,14.0211450565449,2.35771207602066));
#95587=CARTESIAN_POINT('Ctrl Pts',(-10.3090452867247,14.0225427448135,2.36330583821056));
#95588=CARTESIAN_POINT('Ctrl Pts',(-10.4257321549664,14.030168792839,2.39739213910172));
#95589=CARTESIAN_POINT('Ctrl Pts',(-10.5173020255948,14.0361605532385,2.43727187470033));
#95590=CARTESIAN_POINT('Ctrl Pts',(-10.6264657589625,14.0443042109425,2.50230443900004));
#95591=CARTESIAN_POINT('Ctrl Pts',(-10.6496560097137,14.0460958192273,2.51724740777894));
#95592=CARTESIAN_POINT('Ctrl Pts',(-10.6792364247331,14.0484753759896,2.53781273600919));
#95593=CARTESIAN_POINT('Ctrl Pts',(-10.6861215265834,14.0490361501417,2.54271023391761));
#95594=CARTESIAN_POINT('Ctrl Pts',(-10.6973081030162,14.0499589929479,2.55085012838058));
#95595=CARTESIAN_POINT('Ctrl Pts',(-10.7016411638545,14.0503193828548,2.55404876189564));
#95596=CARTESIAN_POINT('Ctrl Pts',(-10.7099952497496,14.0510200049291,2.56030466526437));
#95597=CARTESIAN_POINT('Ctrl Pts',(-10.7140188516814,14.0513600914138,2.56335831031084));
#95598=CARTESIAN_POINT('Ctrl Pts',(-10.7232918405558,14.0521500982644,2.57049036341979));
#95599=CARTESIAN_POINT('Ctrl Pts',(-10.7285265471381,14.0526007462271,2.57458748761704));
#95600=CARTESIAN_POINT('Ctrl Pts',(-10.7454827106333,14.0540760397504,2.58809184890397));
#95601=CARTESIAN_POINT('Ctrl Pts',(-10.7570584194219,14.0551077843701,2.59767884813536));
#95602=CARTESIAN_POINT('Ctrl Pts',(-10.8303369987689,14.0618027892043,2.66077097309791));
#95603=CARTESIAN_POINT('Ctrl Pts',(-10.8865054160675,14.0677212011073,2.72034082963975));
#95604=CARTESIAN_POINT('Ctrl Pts',(-10.9690377057046,14.0777021233809,2.8284235714345));
#95605=CARTESIAN_POINT('Ctrl Pts',(-10.9989943956614,14.0817057328223,2.87385325523932));
#95606=CARTESIAN_POINT('Ctrl Pts',(-11.0336141511362,14.0867561715488,2.93520296624978));
#95607=CARTESIAN_POINT('Ctrl Pts',(-11.0412333895511,14.0878995107753,2.94937582160306));
#95608=CARTESIAN_POINT('Ctrl Pts',(-11.0534550830143,14.0897834850433,2.97327141525539));
#95609=CARTESIAN_POINT('Ctrl Pts',(-11.0582189230439,14.0905317359289,2.98290876493007));
#95610=CARTESIAN_POINT('Ctrl Pts',(-11.0646350366111,14.0915579678811,2.99634886824414));
#95611=CARTESIAN_POINT('Ctrl Pts',(-11.0664000217299,14.0918423051335,3.00009679070665));
#95612=CARTESIAN_POINT('Ctrl Pts',(-11.0693569240626,14.0923220497143,3.00646266130837));
#95613=CARTESIAN_POINT('Ctrl Pts',(-11.0705590827288,14.0925180699404,3.00907578305116));
#95614=CARTESIAN_POINT('Ctrl Pts',(-11.0728481225529,14.0928931663177,3.01409984371837));
#95615=CARTESIAN_POINT('Ctrl Pts',(-11.0739364681581,14.0930723350003,3.01651006354552));
#95616=CARTESIAN_POINT('Ctrl Pts',(-11.0765286456436,14.0935011159065,3.02230256587238));
#95617=CARTESIAN_POINT('Ctrl Pts',(-11.0780246806979,14.093750261528,3.02568833854362));
#95618=CARTESIAN_POINT('Ctrl Pts',(-11.0834105133549,14.0946535881988,3.03803448298171));
#95619=CARTESIAN_POINT('Ctrl Pts',(-11.0872048919799,14.0953023423085,3.04703640595085));
#95620=CARTESIAN_POINT('Ctrl Pts',(-11.1136900810083,14.0999294657895,3.11212170010008));
#95621=CARTESIAN_POINT('Ctrl Pts',(-11.1321446621535,14.1036988020779,3.1698400850009));
#95622=CARTESIAN_POINT('Ctrl Pts',(-11.1581037221486,14.1106773611151,3.2795130995613));
#95623=CARTESIAN_POINT('Ctrl Pts',(-11.166735159857,14.1138847214632,3.33103972618087));
#95624=CARTESIAN_POINT('Ctrl Pts',(-11.1751092255998,14.119174579023,3.41489498456272));
#95625=CARTESIAN_POINT('Ctrl Pts',(-11.1769913383375,14.1212115022148,3.4469367533419));
#95626=CARTESIAN_POINT('Ctrl Pts',(-11.1779381857702,14.1246459503731,3.50006529730578));
#95627=CARTESIAN_POINT('Ctrl Pts',(-11.1777487610663,14.1260218330418,3.52112204678003));
#95628=CARTESIAN_POINT('Ctrl Pts',(-11.1767208575517,14.1279220686643,3.54981742425372));
#95629=CARTESIAN_POINT('Ctrl Pts',(-11.1763719213343,14.1284312981153,3.55747043081901));
#95630=CARTESIAN_POINT('Ctrl Pts',(-11.1756598487533,14.1292912679029,3.5703292923863));
#95631=CARTESIAN_POINT('Ctrl Pts',(-11.1753367261083,14.1296407590123,3.57553719681896));
#95632=CARTESIAN_POINT('Ctrl Pts',(-11.1746299796621,14.1303333882333,3.58582186804063));
#95633=CARTESIAN_POINT('Ctrl Pts',(-11.1742480225125,14.1306764671015,3.59089863791457));
#95634=CARTESIAN_POINT('Ctrl Pts',(-11.1732398049759,14.131512748283,3.6032300523452));
#95635=CARTESIAN_POINT('Ctrl Pts',(-11.1725791642262,14.1320070096822,3.61048159650023));
#95636=CARTESIAN_POINT('Ctrl Pts',(-11.1705118774866,14.1334168620048,3.63105941542356));
#95637=CARTESIAN_POINT('Ctrl Pts',(-11.1689450178714,14.1343373821485,3.64436808903332));
#95638=CARTESIAN_POINT('Ctrl Pts',(-11.1556729142305,14.1412007155932,3.74262931842275));
#95639=CARTESIAN_POINT('Ctrl Pts',(-11.1349492511425,14.147429627284,3.82608861520466));
#95640=CARTESIAN_POINT('Ctrl Pts',(-11.0806119755649,14.1589875392999,3.97382739129924));
#95641=CARTESIAN_POINT('Ctrl Pts',(-11.0497708035041,14.1642648947757,4.03871895862753));
#95642=CARTESIAN_POINT('Ctrl Pts',(-11.0095366195933,14.1697587935403,4.10661598469172));
#95643=CARTESIAN_POINT('Ctrl Pts',(-11.0058006477705,14.170258040153,4.11279050471137));
#95644=CARTESIAN_POINT('Ctrl Pts',(-11.0001527490662,14.1709963651452,4.12193408392853));
#95645=CARTESIAN_POINT('Ctrl Pts',(-10.9982839292167,14.1712380689487,4.12492937497591));
#95646=CARTESIAN_POINT('Ctrl Pts',(-10.9950568967927,14.1716509532859,4.13005015391677));
#95647=CARTESIAN_POINT('Ctrl Pts',(-10.993705297902,14.1718225564764,4.13217972576435));
#95648=CARTESIAN_POINT('Ctrl Pts',(-10.9906194604626,14.1722113338039,4.13700740484274));
#95649=CARTESIAN_POINT('Ctrl Pts',(-10.9888810358292,14.1724282292428,4.13970278010215));
#95650=CARTESIAN_POINT('Ctrl Pts',(-10.9841213206592,14.17301643108,4.14701680658657));
#95651=CARTESIAN_POINT('Ctrl Pts',(-10.981078494559,14.1733863550082,4.15162144859135));
#95652=CARTESIAN_POINT('Ctrl Pts',(-10.9658070460457,14.1752138471674,4.17438192095784));
#95653=CARTESIAN_POINT('Ctrl Pts',(-10.9531053974664,14.1766426458147,4.19221707235233));
#95654=CARTESIAN_POINT('Ctrl Pts',(-10.9266128776836,14.179469584075,4.22730379330148));
#95655=CARTESIAN_POINT('Ctrl Pts',(-10.9128195366583,14.1808668063854,4.24454202275886));
#95656=CARTESIAN_POINT('Ctrl Pts',(-10.8342482834542,14.1884909664596,4.33726817824236));
#95657=CARTESIAN_POINT('Ctrl Pts',(-10.7605964704871,14.1944815888736,4.40469978321671));
#95658=CARTESIAN_POINT('Ctrl Pts',(-10.6568112680421,14.202624201462,4.47798514697378));
#95659=CARTESIAN_POINT('Ctrl Pts',(-10.6337273943094,14.2044160455217,4.49309888129395));
#95660=CARTESIAN_POINT('Ctrl Pts',(-10.6029080403816,14.2067958883378,4.51176497156991));
#95661=CARTESIAN_POINT('Ctrl Pts',(-10.5956337094675,14.2073567045455,4.51606443733364));
#95662=CARTESIAN_POINT('Ctrl Pts',(-10.583647911618,14.2082796093998,4.52297565363541));
#95663=CARTESIAN_POINT('Ctrl Pts',(-10.5789635900421,14.2086400190183,4.52563406360709));
#95664=CARTESIAN_POINT('Ctrl Pts',(-10.5698510433297,14.2093406745037,4.53072322540899));
#95665=CARTESIAN_POINT('Ctrl Pts',(-10.5654250828965,14.2096807746465,4.5331578065533));
#95666=CARTESIAN_POINT('Ctrl Pts',(-10.5551385670223,14.2104708065821,4.5387301983694));
#95667=CARTESIAN_POINT('Ctrl Pts',(-10.5492668807946,14.2109214659424,4.54184698689971));
#95668=CARTESIAN_POINT('Ctrl Pts',(-10.5300348161396,14.2123967732912,4.55184791868687));
#95669=CARTESIAN_POINT('Ctrl Pts',(-10.516569462522,14.2134285197689,4.55852581659148));
#95670=CARTESIAN_POINT('Ctrl Pts',(-10.4292371402673,14.220115589636,4.59977348770738));
#95671=CARTESIAN_POINT('Ctrl Pts',(-10.3520888121434,14.2260252485267,4.62684298723955));
#95672=CARTESIAN_POINT('Ctrl Pts',(-10.2198556405815,14.2360011851153,4.65832560628215));
#95673=CARTESIAN_POINT('Ctrl Pts',(-10.1661203530108,14.2400086752141,4.667244325078));
#95674=CARTESIAN_POINT('Ctrl Pts',(-10.0959347546297,14.2450634897697,4.67394663301471));
#95675=CARTESIAN_POINT('Ctrl Pts',(-10.0798801462141,14.2462074282894,4.67514824222193));
#95676=CARTESIAN_POINT('Ctrl Pts',(-10.0530670054817,14.248092303797,4.67660299268477));
#95677=CARTESIAN_POINT('Ctrl Pts',(-10.0423209096188,14.2488408627486,4.67703851706378));
#95678=CARTESIAN_POINT('Ctrl Pts',(-10.0274276409572,14.2498674756354,4.67743787843442));
#95679=CARTESIAN_POINT('Ctrl Pts',(-10.0232847556705,14.2501518895618,4.67752709290414));
#95680=CARTESIAN_POINT('Ctrl Pts',(-10.016264866399,14.2506317508259,4.6776411988785));
#95681=CARTESIAN_POINT('Ctrl Pts',(-10.0133881094558,14.2508278113248,4.67767741694235));
#95682=CARTESIAN_POINT('Ctrl Pts',(-10.0078664196317,14.2512029717302,4.67772669889318));
#95683=CARTESIAN_POINT('Ctrl Pts',(-10.0052215484168,14.2513821642553,4.67774139505611));
#95684=CARTESIAN_POINT('Ctrl Pts',(-9.99887473123479,14.2518109961491,4.67775528030774));
#95685=CARTESIAN_POINT('Ctrl Pts',(-9.99517276563141,14.2520601689187,4.67774592559472));
#95686=CARTESIAN_POINT('Ctrl Pts',(-9.98170264885298,14.2529635409298,4.67764837369698));
#95687=CARTESIAN_POINT('Ctrl Pts',(-9.97193531930477,14.2536123140564,4.67745610285185));
#95688=CARTESIAN_POINT('Ctrl Pts',(-9.90170261206705,14.2582395178387,4.67519909089871));
#95689=CARTESIAN_POINT('Ctrl Pts',(-9.8414653117913,14.2620089485544,4.66859914659879));
#95690=CARTESIAN_POINT('Ctrl Pts',(-9.73070380691363,14.268987971793,4.64773637442113));
#95691=CARTESIAN_POINT('Ctrl Pts',(-9.68011268705498,14.2721956942608,4.63467666516678));
#95692=CARTESIAN_POINT('Ctrl Pts',(-9.60009646774952,14.2774854886338,4.6082424032536));
#95693=CARTESIAN_POINT('Ctrl Pts',(-9.57006338673536,14.2795219586975,4.59694044102107));
#95694=CARTESIAN_POINT('Ctrl Pts',(-9.52114698590922,14.2829557383333,4.57621467551545));
#95695=CARTESIAN_POINT('Ctrl Pts',(-9.50198810591725,14.2843314211539,4.56748409898914));
#95696=CARTESIAN_POINT('Ctrl Pts',(-9.47619068453028,14.2862314603736,4.55488272108867));
#95697=CARTESIAN_POINT('Ctrl Pts',(-9.46934010158477,14.2867407005199,4.55145319525144));
#95698=CARTESIAN_POINT('Ctrl Pts',(-9.4578802740995,14.2876007144442,4.5455756773821));
#95699=CARTESIAN_POINT('Ctrl Pts',(-9.45325289484323,14.287950239259,4.54316340802868));
#95700=CARTESIAN_POINT('Ctrl Pts',(-9.44414228403918,14.2886429562213,4.53833674196264));
#95701=CARTESIAN_POINT('Ctrl Pts',(-9.43965837403794,14.2889860892448,4.53592386347199));
#95702=CARTESIAN_POINT('Ctrl Pts',(-9.42879922859871,14.2898225403397,4.52998921685848));
#95703=CARTESIAN_POINT('Ctrl Pts',(-9.42244081052756,14.2903169180181,4.52643727845557));
#95704=CARTESIAN_POINT('Ctrl Pts',(-9.40447443733385,14.2917272053611,4.51618111227948));
#95705=CARTESIAN_POINT('Ctrl Pts',(-9.39294774915114,14.2926480475002,4.50933754893369));
#95706=CARTESIAN_POINT('Ctrl Pts',(-9.3086497098293,14.2995045737172,4.45732223127635));
#95707=CARTESIAN_POINT('Ctrl Pts',(-9.2408957002926,14.3057255541152,4.4045366082221));
#95708=CARTESIAN_POINT('Ctrl Pts',(-9.12797791106919,14.3172825909929,4.29487457317117));
#95709=CARTESIAN_POINT('Ctrl Pts',(-9.08115606939346,14.3225671590039,4.24025412018268));
#95710=CARTESIAN_POINT('Ctrl Pts',(-9.03541931818327,14.3280676499016,4.17581895354549));
#95711=CARTESIAN_POINT('Ctrl Pts',(-9.03129594819529,14.3285669474665,4.16989522782331));
#95712=CARTESIAN_POINT('Ctrl Pts',(-9.02523676292711,14.3293053488152,4.16101751904551));
#95713=CARTESIAN_POINT('Ctrl Pts',(-9.02325945089602,14.3295470782624,4.15809226510691));
#95714=CARTESIAN_POINT('Ctrl Pts',(-9.01989213304503,14.3299599976533,4.15306201399799));
#95715=CARTESIAN_POINT('Ctrl Pts',(-9.01849570534121,14.3301316104022,4.15096140054772));
#95716=CARTESIAN_POINT('Ctrl Pts',(-9.01533907458191,14.3305203884803,4.14617970440153));
#95717=CARTESIAN_POINT('Ctrl Pts',(-9.01358306741671,14.3307372752179,4.1434959084252));
#95718=CARTESIAN_POINT('Ctrl Pts',(-9.00883527110182,14.3313254569691,4.13617450439704));
#95719=CARTESIAN_POINT('Ctrl Pts',(-9.00586503392264,14.331695369507,4.13152291490327));
#95720=CARTESIAN_POINT('Ctrl Pts',(-8.99127689375568,14.3335228418838,4.10831892481742));
#95721=CARTESIAN_POINT('Ctrl Pts',(-8.98014424647803,14.3349516307007,4.08946468071107));
#95722=CARTESIAN_POINT('Ctrl Pts',(-8.95885477731884,14.3377785585864,4.05099805787925));
#95723=CARTESIAN_POINT('Ctrl Pts',(-8.94871115641225,14.3391757799869,4.0313888399015));
#95724=CARTESIAN_POINT('Ctrl Pts',(-8.89593019320576,14.3467993358334,3.92191967356889));
#95725=CARTESIAN_POINT('Ctrl Pts',(-8.86425836478119,14.3527893819415,3.82722740622177));
#95726=CARTESIAN_POINT('Ctrl Pts',(-8.83948194661727,14.3609317004653,3.70261829754677));
#95727=CARTESIAN_POINT('Ctrl Pts',(-8.83505423995319,14.3627239268073,3.67537819574988));
#95728=CARTESIAN_POINT('Ctrl Pts',(-8.83052534360589,14.365104179563,3.63962626733462));
#95729=CARTESIAN_POINT('Ctrl Pts',(-8.8295536848012,14.3656650084218,3.63123217414234));
#95730=CARTESIAN_POINT('Ctrl Pts',(-8.82811076054309,14.3665879087885,3.61747204103559));
#95731=CARTESIAN_POINT('Ctrl Pts',(-8.82758582238143,14.3669483009046,3.61211183906176));
#95732=CARTESIAN_POINT('Ctrl Pts',(-8.8266398769313,14.3676489038822,3.6017182157676));
#95733=CARTESIAN_POINT('Ctrl Pts',(-8.82621444727896,14.3679889689138,3.59668530746457));
#95734=CARTESIAN_POINT('Ctrl Pts',(-8.82530418990082,14.3687788914421,3.58502348461544));
#95735=CARTESIAN_POINT('Ctrl Pts',(-8.82484308190171,14.3692294762038,3.57839294545722));
#95736=CARTESIAN_POINT('Ctrl Pts',(-8.82352265841797,14.3707044110595,3.55676165121913));
#95737=CARTESIAN_POINT('Ctrl Pts',(-8.82289430376089,14.3717358557591,3.54174881853642));
#95738=CARTESIAN_POINT('Ctrl Pts',(-8.82069852831664,14.3784346367233,3.44502086357339));
#95739=CARTESIAN_POINT('Ctrl Pts',(-8.82735400030145,14.3843575378299,3.36335666573198));
#95740=CARTESIAN_POINT('Ctrl Pts',(-8.85240249491681,14.3943377502013,3.22970095472508));
#95741=CARTESIAN_POINT('Ctrl Pts',(-8.86607848956628,14.3983361495799,3.17710034152597));
#95742=CARTESIAN_POINT('Ctrl Pts',(-8.88844526655302,14.4033807550033,3.11038530247083));
#95743=CARTESIAN_POINT('Ctrl Pts',(-8.89386758271315,14.4045232570814,3.09524739916394));
#95744=CARTESIAN_POINT('Ctrl Pts',(-8.90342779610554,14.4064060080679,3.07018620823077));
#95745=CARTESIAN_POINT('Ctrl Pts',(-8.90739450844109,14.4071538597087,3.06020032481886));
#95746=CARTESIAN_POINT('Ctrl Pts',(-8.91307911525705,14.4081796526779,3.04644161511211));
#95747=CARTESIAN_POINT('Ctrl Pts',(-8.91468095229681,14.4084639422263,3.04262183677734));
#95748=CARTESIAN_POINT('Ctrl Pts',(-8.91742928129862,14.4089436416149,3.03616384896349));
#95749=CARTESIAN_POINT('Ctrl Pts',(-8.91856533801684,14.4091396638902,3.03352126678986));
#95750=CARTESIAN_POINT('Ctrl Pts',(-8.92076468430593,14.409514802616,3.02845658470013));
#95751=CARTESIAN_POINT('Ctrl Pts',(-8.92182646257291,14.4096940113884,3.02603388022038));
#95752=CARTESIAN_POINT('Ctrl Pts',(-8.92439419035087,14.4101229275648,3.02022826643694));
#95753=CARTESIAN_POINT('Ctrl Pts',(-8.92590796121905,14.4103721679381,3.01684881534942));
#95754=CARTESIAN_POINT('Ctrl Pts',(-8.93147651334137,14.4112761778437,3.00457269863229));
#95755=CARTESIAN_POINT('Ctrl Pts',(-8.9356262332478,14.4119255107363,2.99571917299419));
#95756=CARTESIAN_POINT('Ctrl Pts',(-8.96616586049697,14.4165416240331,2.93261914276511));
#95757=CARTESIAN_POINT('Ctrl Pts',(-8.99658243553144,14.4203006873666,2.88041209228893));
#95758=CARTESIAN_POINT('Ctrl Pts',(-9.06035263249913,14.4272500283245,2.78806606760435));
#95759=CARTESIAN_POINT('Ctrl Pts',(-9.09262364128079,14.4304387260986,2.7473679155282));
#95760=CARTESIAN_POINT('Ctrl Pts',(-9.14921582110835,14.4357257867934,2.68494829616653));
#95761=CARTESIAN_POINT('Ctrl Pts',(-9.17193737867348,14.437780201694,2.66187408347965));
#95762=CARTESIAN_POINT('Ctrl Pts',(-9.2059889899222,14.4407929008442,2.63003178162712));
#95763=CARTESIAN_POINT('Ctrl Pts',(-9.21657426661279,14.441720786512,2.62048747683075));
#95764=CARTESIAN_POINT('Ctrl Pts',(-9.23588409826136,14.4434004412192,2.60370182259106));
#95765=CARTESIAN_POINT('Ctrl Pts',(-9.2445450514665,14.4441492933545,2.59638982952307));
#95766=CARTESIAN_POINT('Ctrl Pts',(-9.2579561617186,14.4453028176267,2.58539511215086));
#95767=CARTESIAN_POINT('Ctrl Pts',(-9.26263138094728,14.4457038473326,2.58162171400793));
#95768=CARTESIAN_POINT('Ctrl Pts',(-9.27118911851519,14.4464360423981,2.5748221841838));
#95769=CARTESIAN_POINT('Ctrl Pts',(-9.27506215064433,14.4467667314772,2.57178428953339));
#95770=CARTESIAN_POINT('Ctrl Pts',(-9.28354691567197,14.4474897629631,2.56521457998554));
#95771=CARTESIAN_POINT('Ctrl Pts',(-9.28816594199024,14.4478824727722,2.5616924410005));
#95772=CARTESIAN_POINT('Ctrl Pts',(-9.30089711404038,14.4489625415048,2.55213266983955));
#95773=CARTESIAN_POINT('Ctrl Pts',(-9.30906110376885,14.4496525812715,2.54616523899348));
#95774=CARTESIAN_POINT('Ctrl Pts',(-9.35412532739765,14.4534486071042,2.51410789136402));
#95775=CARTESIAN_POINT('Ctrl Pts',(-9.39242242888004,14.4566300549821,2.49005647991694));
#95776=CARTESIAN_POINT('Ctrl Pts',(-9.50430495861425,14.4658014963135,2.42846204853772));
#95777=CARTESIAN_POINT('Ctrl Pts',(-9.5805894708448,14.471929999649,2.39636962951048));
#95778=CARTESIAN_POINT('Ctrl Pts',(-9.68468909199254,14.4798355932033,2.3649398952871));
#95779=CARTESIAN_POINT('Ctrl Pts',(-9.71003520052362,14.4817245372623,2.35820185277116));
#95780=CARTESIAN_POINT('Ctrl Pts',(-9.74557920676294,14.4843066413364,2.35001292473762));
#95781=CARTESIAN_POINT('Ctrl Pts',(-9.75560177731054,14.4850274220478,2.34784127037439));
#95782=CARTESIAN_POINT('Ctrl Pts',(-9.77312777195125,14.4862736728282,2.34428279898195));
#95783=CARTESIAN_POINT('Ctrl Pts',(-9.78061855489875,14.4868018559942,2.34283750241962));
#95784=CARTESIAN_POINT('Ctrl Pts',(-9.79167502191317,14.4875743620624,2.34081545724837));
#95785=CARTESIAN_POINT('Ctrl Pts',(-9.79522997733308,14.4878216665144,2.34018219562515));
#95786=CARTESIAN_POINT('Ctrl Pts',(-9.80151767638914,14.4882571084843,2.33909194777495));
#95787=CARTESIAN_POINT('Ctrl Pts',(-9.80424917933254,14.4884456145673,2.33862824414529));
#95788=CARTESIAN_POINT('Ctrl Pts',(-9.80835586790926,14.4887280279149,2.33794598763162));
#95789=CARTESIAN_POINT('Ctrl Pts',(-9.80972976349543,14.4888223435607,2.33772024100504));
#95790=CARTESIAN_POINT('Ctrl Pts',(-9.81110406371064,14.4889165240206,2.33749693000261));
#95791=CARTESIAN_POINT('Origin',(-10.,12.3756328852638,3.5));
#95792=CARTESIAN_POINT('',(-9.81110406371068,15.0871826612189,2.3374969300026));
#95793=CARTESIAN_POINT('',(-9.81110406371068,14.9873061497326,2.3374969300026));
#95794=CARTESIAN_POINT('',(-9.81110406371068,12.3756328852638,2.3374969300026));
#95795=CARTESIAN_POINT('Ctrl Pts',(-9.81110406371068,15.0871826612189,2.3374969300026));
#95796=CARTESIAN_POINT('Ctrl Pts',(-9.79515642301048,15.086163901984,2.3400882732854));
#95797=CARTESIAN_POINT('Ctrl Pts',(-9.77925508557964,15.0851380650591,2.34300891814498));
#95798=CARTESIAN_POINT('Ctrl Pts',(-9.73492997612474,15.0822433730758,2.35209835980764));
#95799=CARTESIAN_POINT('Ctrl Pts',(-9.70667787143568,15.0803573243553,2.35899070974895));
#95800=CARTESIAN_POINT('Ctrl Pts',(-9.67043288027128,15.0778698994534,2.36926810425282));
#95801=CARTESIAN_POINT('Ctrl Pts',(-9.66218053588176,15.0772989562322,2.37170610672386));
#95802=CARTESIAN_POINT('Ctrl Pts',(-9.64877427818331,15.0763635739621,2.37582699727071));
#95803=CARTESIAN_POINT('Ctrl Pts',(-9.64360386412048,15.0760009032648,2.37745546173498));
#95804=CARTESIAN_POINT('Ctrl Pts',(-9.63364852141444,15.0752988008422,2.3806666912685));
#95805=CARTESIAN_POINT('Ctrl Pts',(-9.62886213944729,15.0749595342949,2.38224459339228));
#95806=CARTESIAN_POINT('Ctrl Pts',(-9.61786078480123,15.0741757290523,2.38594980670179));
#95807=CARTESIAN_POINT('Ctrl Pts',(-9.61165323633449,15.0737304990385,2.38809847509248));
#95808=CARTESIAN_POINT('Ctrl Pts',(-9.5917276463968,15.0722915898774,2.3951826897708));
#95809=CARTESIAN_POINT('Ctrl Pts',(-9.57808362769048,15.0712912911195,2.40032088986485));
#95810=CARTESIAN_POINT('Ctrl Pts',(-9.47990134218978,15.0639804426116,2.43939150843279));
#95811=CARTESIAN_POINT('Ctrl Pts',(-9.3994725387176,15.0573441213353,2.48277165602932));
#95812=CARTESIAN_POINT('Ctrl Pts',(-9.2694598080945,15.0456926755982,2.57372921502584));
#95813=CARTESIAN_POINT('Ctrl Pts',(-9.2174929237763,15.0407320728207,2.61719122026143));
#95814=CARTESIAN_POINT('Ctrl Pts',(-9.16478291082366,15.0355647769559,2.66960704415242));
#95815=CARTESIAN_POINT('Ctrl Pts',(-9.16006739343266,15.0351012581966,2.67437704193263));
#95816=CARTESIAN_POINT('Ctrl Pts',(-9.15300305419007,15.0344053202665,2.6816461685585));
#95817=CARTESIAN_POINT('Ctrl Pts',(-9.15062407321736,15.0341706885431,2.68411559923894));
#95818=CARTESIAN_POINT('Ctrl Pts',(-9.14651984857847,15.0337654900398,2.6884132751252));
#95819=CARTESIAN_POINT('Ctrl Pts',(-9.14478965157078,15.0335945477369,2.69023667582861));
#95820=CARTESIAN_POINT('Ctrl Pts',(-9.14081082490376,15.0332011546344,2.69445681434044));
#95821=CARTESIAN_POINT('Ctrl Pts',(-9.13856638147964,15.032979021896,2.69685743226108));
#95822=CARTESIAN_POINT('Ctrl Pts',(-9.13234608103675,15.032362672994,2.70356663193275));
#95823=CARTESIAN_POINT('Ctrl Pts',(-9.12839223458599,15.0319700666775,2.7078956257733));
#95824=CARTESIAN_POINT('Ctrl Pts',(-9.10666602591954,15.0298068467001,2.73204291737873));
#95825=CARTESIAN_POINT('Ctrl Pts',(-9.0895356739129,15.028079171243,2.75243151858018));
#95826=CARTESIAN_POINT('Ctrl Pts',(-9.01086387259382,15.0199379171547,2.85278745603675));
#95827=CARTESIAN_POINT('Ctrl Pts',(-8.9590757653736,15.0138973467825,2.93986233630128));
#95828=CARTESIAN_POINT('Ctrl Pts',(-8.90285572880089,15.004947601507,3.06985178960889));
#95829=CARTESIAN_POINT('Ctrl Pts',(-8.88864274116309,15.0023313389695,3.10803377493285));
#95830=CARTESIAN_POINT('Ctrl Pts',(-8.87356934886499,14.9990191740848,3.15599350390052));
#95831=CARTESIAN_POINT('Ctrl Pts',(-8.87081380929607,14.998385799955,3.16514925862222));
#95832=CARTESIAN_POINT('Ctrl Pts',(-8.86661330892795,14.9973737413982,3.17974795932868));
#95833=CARTESIAN_POINT('Ctrl Pts',(-8.86509534370761,14.9969974173279,3.18516960072175));
#95834=CARTESIAN_POINT('Ctrl Pts',(-8.86230588049519,14.9962852939782,3.19541497652682));
#95835=CARTESIAN_POINT('Ctrl Pts',(-8.86102603857296,14.995949771631,3.20023632649516));
#95836=CARTESIAN_POINT('Ctrl Pts',(-8.85820530041689,14.9951898938875,3.21114136449993));
#95837=CARTESIAN_POINT('Ctrl Pts',(-8.8566823347847,14.994764974924,3.21722949047381));
#95838=CARTESIAN_POINT('Ctrl Pts',(-8.85289074525709,14.9936680825427,3.23291811381712));
#95839=CARTESIAN_POINT('Ctrl Pts',(-8.85069399348628,14.992993848856,3.24253530471152));
#95840=CARTESIAN_POINT('Ctrl Pts',(-8.83263750569812,14.987095227857,3.3264260314709));
#95841=CARTESIAN_POINT('Ctrl Pts',(-8.8238787719305,14.9816440419769,3.40203080089322));
#95842=CARTESIAN_POINT('Ctrl Pts',(-8.82143546749479,14.9720997059448,3.53244505879391));
#95843=CARTESIAN_POINT('Ctrl Pts',(-8.8241999708502,14.9680731150544,3.58695672538426));
#95844=CARTESIAN_POINT('Ctrl Pts',(-8.833553584781,14.9624127024092,3.66447865739957));
#95845=CARTESIAN_POINT('Ctrl Pts',(-8.83707848897994,14.9607200427715,3.68778756764681));
#95846=CARTESIAN_POINT('Ctrl Pts',(-8.8430107503973,14.9583801437462,3.7203680233814));
#95847=CARTESIAN_POINT('Ctrl Pts',(-8.84483496536203,14.9577102092966,3.72973886364951));
#95848=CARTESIAN_POINT('Ctrl Pts',(-8.84823775873616,14.9565433731508,3.74615211986347));
#95849=CARTESIAN_POINT('Ctrl Pts',(-8.84976747950936,14.9560441886145,3.75320403206441));
#95850=CARTESIAN_POINT('Ctrl Pts',(-8.85214223665456,14.9553058688401,3.76368558376098));
#95851=CARTESIAN_POINT('Ctrl Pts',(-8.85293800895049,14.955064109725,3.76712604041762));
#95852=CARTESIAN_POINT('Ctrl Pts',(-8.8543289137695,14.9546511048689,3.773018664837));
#95853=CARTESIAN_POINT('Ctrl Pts',(-8.85491646419467,14.9544794364198,3.77547254971057));
#95854=CARTESIAN_POINT('Ctrl Pts',(-8.85626917212068,14.954090479467,3.78104297456336));
#95855=CARTESIAN_POINT('Ctrl Pts',(-8.85703918324864,14.9538734700838,3.78415828720341));
#95856=CARTESIAN_POINT('Ctrl Pts',(-8.85916925416681,14.9532848366537,3.79262738035619));
#95857=CARTESIAN_POINT('Ctrl Pts',(-8.86055428177709,14.9529145979175,3.79797488580829));
#95858=CARTESIAN_POINT('Ctrl Pts',(-8.86762568667007,14.951083873887,3.82450666385443));
#95859=CARTESIAN_POINT('Ctrl Pts',(-8.8738658668647,14.9496522769765,3.8455404807236));
#95860=CARTESIAN_POINT('Ctrl Pts',(-8.88755421287155,14.9468232500441,3.88735801601474));
#95861=CARTESIAN_POINT('Ctrl Pts',(-8.89500624158797,14.9454266357613,3.90813080358829));
#95862=CARTESIAN_POINT('Ctrl Pts',(-8.93930142230548,14.9377929389679,4.02147830061559));
#95863=CARTESIAN_POINT('Ctrl Pts',(-8.98719089542334,14.9317925662774,4.10929409034255));
#95864=CARTESIAN_POINT('Ctrl Pts',(-9.06162314088735,14.9236489446797,4.21224657555268));
#95865=CARTESIAN_POINT('Ctrl Pts',(-9.07845121220709,14.921868263407,4.23388960888349));
#95866=CARTESIAN_POINT('Ctrl Pts',(-9.10142305284339,14.9195010855006,4.26139716372696));
#95867=CARTESIAN_POINT('Ctrl Pts',(-9.1068974794257,14.9189413996988,4.26781120888467));
#95868=CARTESIAN_POINT('Ctrl Pts',(-9.11597880088583,14.918019813943,4.27822269455469));
#95869=CARTESIAN_POINT('Ctrl Pts',(-9.11954513056321,14.9176595828078,4.28225524226391));
#95870=CARTESIAN_POINT('Ctrl Pts',(-9.12651336288774,14.9169588856068,4.29002639585914));
#95871=CARTESIAN_POINT('Ctrl Pts',(-9.12991193966858,14.916618562821,4.29376783587075));
#95872=CARTESIAN_POINT('Ctrl Pts',(-9.13784436342581,14.915827437928,4.30238836057797));
#95873=CARTESIAN_POINT('Ctrl Pts',(-9.14239568800388,14.9153759028332,4.30725105372781));
#95874=CARTESIAN_POINT('Ctrl Pts',(-9.15739683132253,14.9138951531157,4.32300841541441));
#95875=CARTESIAN_POINT('Ctrl Pts',(-9.16801453891312,14.9128587681617,4.33374043166603));
#95876=CARTESIAN_POINT('Ctrl Pts',(-9.23063595178446,14.9068098215102,4.39464844342418));
#95877=CARTESIAN_POINT('Ctrl Pts',(-9.2869547928158,14.9016022255556,4.44014898235957));
#95878=CARTESIAN_POINT('Ctrl Pts',(-9.39845520858646,14.8917900714712,4.51442098560932));
#95879=CARTESIAN_POINT('Ctrl Pts',(-9.45244614392866,14.8872265215785,4.54455317484718));
#95880=CARTESIAN_POINT('Ctrl Pts',(-9.52420053704212,14.8815545142569,4.57750009150391));
#95881=CARTESIAN_POINT('Ctrl Pts',(-9.54000591131022,14.8803285958587,4.58434177253366));
#95882=CARTESIAN_POINT('Ctrl Pts',(-9.5664273085294,14.8783239245719,4.59509706862887));
#95883=CARTESIAN_POINT('Ctrl Pts',(-9.57695946965197,14.8775363382036,4.59920862529774));
#95884=CARTESIAN_POINT('Ctrl Pts',(-9.59150822018195,14.8764656743147,4.60464808369285));
#95885=CARTESIAN_POINT('Ctrl Pts',(-9.59547477636411,14.8761755178754,4.60610680669362));
#95886=CARTESIAN_POINT('Ctrl Pts',(-9.602170366465,14.8756887714325,4.6085283120383));
#95887=CARTESIAN_POINT('Ctrl Pts',(-9.60489522542583,14.8754915282382,4.6095024351739));
#95888=CARTESIAN_POINT('Ctrl Pts',(-9.61010207160125,14.8751162683432,4.61134224122461));
#95889=CARTESIAN_POINT('Ctrl Pts',(-9.61258339793891,14.8749381462774,4.61220966930437));
#95890=CARTESIAN_POINT('Ctrl Pts',(-9.61850538934226,14.8745146755478,4.61425767042309));
#95891=CARTESIAN_POINT('Ctrl Pts',(-9.62194868648402,14.8742697672294,4.61543063400866));
#95892=CARTESIAN_POINT('Ctrl Pts',(-9.6342298585833,14.8734007465502,4.61955082894055));
#95893=CARTESIAN_POINT('Ctrl Pts',(-9.64309748662113,14.8727815287675,4.62240922316525));
#95894=CARTESIAN_POINT('Ctrl Pts',(-9.72462454454528,14.8671558968509,4.64762473748706));
#95895=CARTESIAN_POINT('Ctrl Pts',(-9.79926601994208,14.8624854762799,4.66300621121937));
#95896=CARTESIAN_POINT('Ctrl Pts',(-9.95809474724053,14.8526108967361,4.67997584784296));
#95897=CARTESIAN_POINT('Ctrl Pts',(-10.04200932194,14.8474183703074,4.67997104891288));
#95898=CARTESIAN_POINT('Ctrl Pts',(-10.1363867317225,14.8411862355522,4.66988037047647));
#95899=CARTESIAN_POINT('Ctrl Pts',(-10.1475459805805,14.8404434683745,4.66852539173069));
#95900=CARTESIAN_POINT('Ctrl Pts',(-10.1646189485755,14.8392972973858,4.66620390213083));
#95901=CARTESIAN_POINT('Ctrl Pts',(-10.1705477420818,14.838897461752,4.66535162290304));
#95902=CARTESIAN_POINT('Ctrl Pts',(-10.181337350597,14.8381663906088,4.6637164887199));
#95903=CARTESIAN_POINT('Ctrl Pts',(-10.1862002780894,14.8378356223811,4.66294830324269));
#95904=CARTESIAN_POINT('Ctrl Pts',(-10.1968094614368,14.8371111572974,4.66120414638569));
#95905=CARTESIAN_POINT('Ctrl Pts',(-10.2025535497538,14.8367170843323,4.66021596742087));
#95906=CARTESIAN_POINT('Ctrl Pts',(-10.2183238428585,14.8356300080596,4.65738225803243));
#95907=CARTESIAN_POINT('Ctrl Pts',(-10.2283335899786,14.8349342675502,4.65544915589988));
#95908=CARTESIAN_POINT('Ctrl Pts',(-10.2841024986952,14.8310247604404,4.64392598990509));
#95909=CARTESIAN_POINT('Ctrl Pts',(-10.3292783006312,14.8277299586301,4.63174894848617));
#95910=CARTESIAN_POINT('Ctrl Pts',(-10.476822735941,14.8165426094329,4.58239586390702));
#95911=CARTESIAN_POINT('Ctrl Pts',(-10.5747448547489,14.8083573658706,4.53373434003219));
#95912=CARTESIAN_POINT('Ctrl Pts',(-10.6723249607545,14.8000100018984,4.46703774132654));
#95913=CARTESIAN_POINT('Ctrl Pts',(-10.6799969562568,14.7993527401163,4.46165846229797));
#95914=CARTESIAN_POINT('Ctrl Pts',(-10.6933774718435,14.7982058108819,4.45203640185931));
#95915=CARTESIAN_POINT('Ctrl Pts',(-10.6991131966574,14.7977139621432,4.44783246064298));
#95916=CARTESIAN_POINT('Ctrl Pts',(-10.7076231564636,14.7969843345878,4.44147589157585));
#95917=CARTESIAN_POINT('Ctrl Pts',(-10.710426284981,14.7967440190397,4.43936248615759));
#95918=CARTESIAN_POINT('Ctrl Pts',(-10.71522611727,14.7963326163181,4.43570990106464));
#95919=CARTESIAN_POINT('Ctrl Pts',(-10.7172273669088,14.7961611159705,4.43417681536315));
#95920=CARTESIAN_POINT('Ctrl Pts',(-10.721776311964,14.7957713641499,4.43066879635044));
#95921=CARTESIAN_POINT('Ctrl Pts',(-10.7243208313539,14.7955533991702,4.42868982276645));
#95922=CARTESIAN_POINT('Ctrl Pts',(-10.7312529820739,14.7949596205046,4.42325259202769));
#95923=CARTESIAN_POINT('Ctrl Pts',(-10.7356242528647,14.7945852326823,4.41977346893174));
#95924=CARTESIAN_POINT('Ctrl Pts',(-10.7576336585479,14.7926994121515,4.40199875750753));
#95925=CARTESIAN_POINT('Ctrl Pts',(-10.7748818732901,14.7912189859528,4.38722531843091));
#95926=CARTESIAN_POINT('Ctrl Pts',(-10.869264255462,14.7830326072881,4.30153124285035));
#95927=CARTESIAN_POINT('Ctrl Pts',(-10.9370953648259,14.7767771739846,4.22106110241961));
#95928=CARTESIAN_POINT('Ctrl Pts',(-11.0155227059407,14.7675554195729,4.09791834561534));
#95929=CARTESIAN_POINT('Ctrl Pts',(-11.0358150443397,14.7649090600559,4.06203143521413));
#95930=CARTESIAN_POINT('Ctrl Pts',(-11.0584617860244,14.7615631137386,4.01657113892318));
#95931=CARTESIAN_POINT('Ctrl Pts',(-11.0626342524439,14.7609276528238,4.00793260437782));
#95932=CARTESIAN_POINT('Ctrl Pts',(-11.0690901870508,14.7599130301367,3.99413865638992));
#95933=CARTESIAN_POINT('Ctrl Pts',(-11.0714430267532,14.7595362497053,3.98901603075218));
#95934=CARTESIAN_POINT('Ctrl Pts',(-11.0758079984053,14.7588237438712,3.97932983049848));
#95935=CARTESIAN_POINT('Ctrl Pts',(-11.0778281000815,14.7584882989153,3.97476996661136));
#95936=CARTESIAN_POINT('Ctrl Pts',(-11.0823202761151,14.7577292464072,3.96445358246608));
#95937=CARTESIAN_POINT('Ctrl Pts',(-11.0847754866775,14.7573050802712,3.9586899292822));
#95938=CARTESIAN_POINT('Ctrl Pts',(-11.0909641894919,14.7562114267376,3.94383420555174));
#95939=CARTESIAN_POINT('Ctrl Pts',(-11.0946299981132,14.7555397014751,3.93471464410521));
#95940=CARTESIAN_POINT('Ctrl Pts',(-11.1207624757704,14.7505686146395,3.86727683397196));
#95941=CARTESIAN_POINT('Ctrl Pts',(-11.1386659770076,14.7461193389454,3.80730810563435));
#95942=CARTESIAN_POINT('Ctrl Pts',(-11.1674612877016,14.7361024974039,3.6726093977843));
#95943=CARTESIAN_POINT('Ctrl Pts',(-11.1761037620632,14.7305115454156,3.5976709588132));
#95944=CARTESIAN_POINT('Ctrl Pts',(-11.1778974117992,14.7237241244478,3.5034695223068));
#95945=CARTESIAN_POINT('Ctrl Pts',(-11.1778007149274,14.7223711317165,3.48451098465177));
#95946=CARTESIAN_POINT('Ctrl Pts',(-11.1768917369171,14.7201829942647,3.45343800782624));
#95947=CARTESIAN_POINT('Ctrl Pts',(-11.1763497864266,14.7193369822171,3.44131960701993));
#95948=CARTESIAN_POINT('Ctrl Pts',(-11.1753596703006,14.7182009157122,3.42487632274085));
#95949=CARTESIAN_POINT('Ctrl Pts',(-11.1750746734413,14.7179026400075,3.42054287450894));
#95950=CARTESIAN_POINT('Ctrl Pts',(-11.1745581420938,14.7174061486651,3.4133008327999));
#95951=CARTESIAN_POINT('Ctrl Pts',(-11.1743397596288,14.7172072223932,3.41039138284307));
#95952=CARTESIAN_POINT('Ctrl Pts',(-11.1739057530642,14.7168316903136,3.40488352823782));
#95953=CARTESIAN_POINT('Ctrl Pts',(-11.1736923091171,14.7166549618972,3.40228498510318));
#95954=CARTESIAN_POINT('Ctrl Pts',(-11.1731675700004,14.7162384846137,3.39614653253036));
#95955=CARTESIAN_POINT('Ctrl Pts',(-11.1728488774262,14.7159991425362,3.39260725561084));
#95956=CARTESIAN_POINT('Ctrl Pts',(-11.1716834089743,14.7151686670493,3.38028848612401));
#95957=CARTESIAN_POINT('Ctrl Pts',(-11.1707540076973,14.7145818816721,3.3715168403613));
#95958=CARTESIAN_POINT('Ctrl Pts',(-11.1599944723858,14.7084873102052,3.27981357669443));
#95959=CARTESIAN_POINT('Ctrl Pts',(-11.1414669996497,14.703390024718,3.19812810115913));
#95960=CARTESIAN_POINT('Ctrl Pts',(-11.0927454466446,14.6940697106799,3.05558436386053));
#95961=CARTESIAN_POINT('Ctrl Pts',(-11.0656582272927,14.689889638275,2.99406626589762));
#95962=CARTESIAN_POINT('Ctrl Pts',(-11.0249721304659,14.6843797878794,2.91961894232744));
#95963=CARTESIAN_POINT('Ctrl Pts',(-11.0161104588839,14.6832161548251,2.90424038279996));
#95964=CARTESIAN_POINT('Ctrl Pts',(-11.003182358922,14.6815646249533,2.88293296862757));
#95965=CARTESIAN_POINT('Ctrl Pts',(-10.9994037128228,14.6810870847356,2.87683165883304));
#95966=CARTESIAN_POINT('Ctrl Pts',(-10.9928318699743,14.6802650780787,2.86643374560969));
#95967=CARTESIAN_POINT('Ctrl Pts',(-10.9900659264629,14.6799216158254,2.86212008921976));
#95968=CARTESIAN_POINT('Ctrl Pts',(-10.9847400147653,14.6792649190055,2.8539321020965));
#95969=CARTESIAN_POINT('Ctrl Pts',(-10.9821851047133,14.6789518763997,2.85005458352763));
#95970=CARTESIAN_POINT('Ctrl Pts',(-10.9755215472582,14.6781404365828,2.84007050079291));
#95971=CARTESIAN_POINT('Ctrl Pts',(-10.9713785198365,14.677640761815,2.83398723735266));
#95972=CARTESIAN_POINT('Ctrl Pts',(-10.9593677994562,14.6762055933261,2.81670221532533));
#95973=CARTESIAN_POINT('Ctrl Pts',(-10.9513616893335,14.6752649125774,2.80559857014769));
#95974=CARTESIAN_POINT('Ctrl Pts',(-10.8985606635468,14.6691591906535,2.73499653709905));
#95975=CARTESIAN_POINT('Ctrl Pts',(-10.8484085349741,14.6637843427555,2.67973117641846));
#95976=CARTESIAN_POINT('Ctrl Pts',(-10.7685465747564,14.6558647563047,2.6069374200527));
#95977=CARTESIAN_POINT('Ctrl Pts',(-10.7427501549166,14.6533911746591,2.58537066266472));
#95978=CARTESIAN_POINT('Ctrl Pts',(-10.6798507471014,14.6475952447705,2.53720261894305));
#95979=CARTESIAN_POINT('Ctrl Pts',(-10.6420500350538,14.6442894169076,2.51159296237786));
#95980=CARTESIAN_POINT('Ctrl Pts',(-10.5948015385741,14.6404403631488,2.48344007535465));
#95981=CARTESIAN_POINT('Ctrl Pts',(-10.5866906047509,14.6397892327431,2.47873749756918));
#95982=CARTESIAN_POINT('Ctrl Pts',(-10.5751055582746,14.6388736721212,2.47220427027029));
#95983=CARTESIAN_POINT('Ctrl Pts',(-10.5716773708631,14.6386045189279,2.47029351270828));
#95984=CARTESIAN_POINT('Ctrl Pts',(-10.5657538125789,14.6381425825023,2.46703061987713));
#95985=CARTESIAN_POINT('Ctrl Pts',(-10.5632630078994,14.637949291647,2.46567031302051));
#95986=CARTESIAN_POINT('Ctrl Pts',(-10.558050104394,14.6375467694765,2.46284779771027));
#95987=CARTESIAN_POINT('Ctrl Pts',(-10.5553271484494,14.6373376432458,2.46138728657768));
#95988=CARTESIAN_POINT('Ctrl Pts',(-10.5480685382285,14.6367830902484,2.45753069468107));
#95989=CARTESIAN_POINT('Ctrl Pts',(-10.5435228608847,14.6364388190237,2.45515346713946));
#95990=CARTESIAN_POINT('Ctrl Pts',(-10.5236759054407,14.6349481298397,2.44493879028469));
#95991=CARTESIAN_POINT('Ctrl Pts',(-10.508218704477,14.6338191436672,2.43740674079702));
#95992=CARTESIAN_POINT('Ctrl Pts',(-10.4228116789766,14.627724088782,2.39807957301927));
#95993=CARTESIAN_POINT('Ctrl Pts',(-10.350037250603,14.6230382503442,2.37284654546187));
#95994=CARTESIAN_POINT('Ctrl Pts',(-10.2060823929743,14.6138685967608,2.33823601714495));
#95995=CARTESIAN_POINT('Ctrl Pts',(-10.1354909893856,14.6094124103385,2.32790541231677));
#95996=CARTESIAN_POINT('Ctrl Pts',(-10.0522982170698,14.6039508728099,2.32334926303576));
#95997=CARTESIAN_POINT('Ctrl Pts',(-10.0401829621124,14.6031507042883,2.32287325576203));
#95998=CARTESIAN_POINT('Ctrl Pts',(-10.0218937506142,14.6019345536166,2.3224373452307));
#95999=CARTESIAN_POINT('Ctrl Pts',(-10.0157236667524,14.6015228630233,2.32233879826242));
#96000=CARTESIAN_POINT('Ctrl Pts',(-10.0045738873246,14.6007762391687,2.32224835506252));
#96001=CARTESIAN_POINT('Ctrl Pts',(-9.99959444424118,14.6004418383323,2.32223954395832));
#96002=CARTESIAN_POINT('Ctrl Pts',(-9.98891417538958,14.5997224587871,2.32228837617336));
#96003=CARTESIAN_POINT('Ctrl Pts',(-9.98321354402233,14.5993371839392,2.32235583586629));
#96004=CARTESIAN_POINT('Ctrl Pts',(-9.96788113268124,14.5982973292879,2.32264862453965));
#96005=CARTESIAN_POINT('Ctrl Pts',(-9.95825143043,14.5976403893599,2.32295075283073));
#96006=CARTESIAN_POINT('Ctrl Pts',(-9.91073127949011,14.5943787740444,2.32502554782517));
#96007=CARTESIAN_POINT('Ctrl Pts',(-9.87294196459308,14.5917218418744,2.3285096816482));
#96008=CARTESIAN_POINT('Ctrl Pts',(-9.82727988855788,14.5884328955156,2.33495497532425));
#96009=CARTESIAN_POINT('Ctrl Pts',(-9.81918414308965,14.5878467961096,2.33618399209425));
#96010=CARTESIAN_POINT('Ctrl Pts',(-9.81110404084991,14.5872589202102,2.33749693371726));
#96011=CARTESIAN_POINT('Ctrl Pts',(-9.81110406371064,14.4889165240206,2.33749693000261));
#96012=CARTESIAN_POINT('Ctrl Pts',(-9.81293423381957,14.4890419451336,2.33719954438254));
#96013=CARTESIAN_POINT('Ctrl Pts',(-9.8147651215191,14.4891671265006,2.33690647822745));
#96014=CARTESIAN_POINT('Ctrl Pts',(-9.82221742167204,14.489675507847,2.33573164825552));
#96015=CARTESIAN_POINT('Ctrl Pts',(-9.82784462027069,14.4900567306634,2.33488628516173));
#96016=CARTESIAN_POINT('Ctrl Pts',(-9.85733721477413,14.492041919143,2.33067400898253));
#96017=CARTESIAN_POINT('Ctrl Pts',(-9.88129756629557,14.4936108365854,2.32799920258862));
#96018=CARTESIAN_POINT('Ctrl Pts',(-10.0083675087875,14.5017797674169,2.31775135642753));
#96019=CARTESIAN_POINT('Ctrl Pts',(-10.1120613637523,14.5079580194738,2.32304295719625));
#96020=CARTESIAN_POINT('Ctrl Pts',(-10.2540911247382,14.5170821721449,2.34925395510814));
#96021=CARTESIAN_POINT('Ctrl Pts',(-10.2940218817298,14.519718000193,2.35880355559414));
#96022=CARTESIAN_POINT('Ctrl Pts',(-10.3425582451398,14.523051989106,2.37312791845606));
#96023=CARTESIAN_POINT('Ctrl Pts',(-10.3517128223254,14.5236865838296,2.37595154858003));
#96024=CARTESIAN_POINT('Ctrl Pts',(-10.3661938515876,14.5247000611114,2.38061228501019));
#96025=CARTESIAN_POINT('Ctrl Pts',(-10.3715434553918,14.5250765705145,2.38237651586326));
#96026=CARTESIAN_POINT('Ctrl Pts',(-10.3816038490228,14.5257887112024,2.38577451827883));
#96027=CARTESIAN_POINT('Ctrl Pts',(-10.3863173357958,14.5261240633218,2.38739996564203));
#96028=CARTESIAN_POINT('Ctrl Pts',(-10.39693084664,14.5268831035451,2.3911356133887));
#96029=CARTESIAN_POINT('Ctrl Pts',(-10.402824597866,14.5273073513695,2.39326305490973));
#96030=CARTESIAN_POINT('Ctrl Pts',(-10.4179259514809,14.528401605434,2.39885073114363));
#96031=CARTESIAN_POINT('Ctrl Pts',(-10.4271075329751,14.5290738547771,2.40237941060042));
#96032=CARTESIAN_POINT('Ctrl Pts',(-10.5057251545043,14.5348914096565,2.43372963229322));
#96033=CARTESIAN_POINT('Ctrl Pts',(-10.5723959245945,14.5402563171763,2.46798765006031));
#96034=CARTESIAN_POINT('Ctrl Pts',(-10.680269948406,14.5496267222032,2.53710181888544));
#96035=CARTESIAN_POINT('Ctrl Pts',(-10.723175078213,14.553565868319,2.56889420816404));
#96036=CARTESIAN_POINT('Ctrl Pts',(-10.7707674678369,14.5581061783364,2.60944012662582));
#96037=CARTESIAN_POINT('Ctrl Pts',(-10.7776874022938,14.5587707980073,2.6154765754767));
#96038=CARTESIAN_POINT('Ctrl Pts',(-10.8056081713895,14.5614686907056,2.6404136084886));
#96039=CARTESIAN_POINT('Ctrl Pts',(-10.8259981874437,14.5634772388978,2.65998774845528));
#96040=CARTESIAN_POINT('Ctrl Pts',(-10.8498136540429,14.565851061767,2.68455697518382));
#96041=CARTESIAN_POINT('Ctrl Pts',(-10.8539288001622,14.5662622943024,2.68886734665599));
#96042=CARTESIAN_POINT('Ctrl Pts',(-10.8602768545219,14.5668980546799,2.69561841436734));
#96043=CARTESIAN_POINT('Ctrl Pts',(-10.8625324246797,14.56712422851,2.69803752033576));
#96044=CARTESIAN_POINT('Ctrl Pts',(-10.86667216758,14.5675397954912,2.70251507650378));
#96045=CARTESIAN_POINT('Ctrl Pts',(-10.8685592107731,14.5677293985858,2.70457071530617));
#96046=CARTESIAN_POINT('Ctrl Pts',(-10.8728245906383,14.5681583807778,2.70925045808031));
#96047=CARTESIAN_POINT('Ctrl Pts',(-10.8751984084862,14.5683974234896,2.7118785939477));
#96048=CARTESIAN_POINT('Ctrl Pts',(-10.8824096159105,14.569124659784,2.71993513169187));
#96049=CARTESIAN_POINT('Ctrl Pts',(-10.887208734679,14.5696101262677,2.72539778162062));
#96050=CARTESIAN_POINT('Ctrl Pts',(-10.93090392215,14.5740478705638,2.77607320849554));
#96051=CARTESIAN_POINT('Ctrl Pts',(-10.9663693508976,14.5777824413029,2.82414171107008));
#96052=CARTESIAN_POINT('Ctrl Pts',(-11.0508106610127,14.5876464167405,2.95891812747188));
#96053=CARTESIAN_POINT('Ctrl Pts',(-11.0926995897543,14.5937074532342,3.04946905615169));
#96054=CARTESIAN_POINT('Ctrl Pts',(-11.126881644185,14.6011027636083,3.15733032293103));
#96055=CARTESIAN_POINT('Ctrl Pts',(-11.1308115917176,14.6020098223008,3.17053093363708));
#96056=CARTESIAN_POINT('Ctrl Pts',(-11.136232881713,14.6033506763106,3.18998205254091));
#96057=CARTESIAN_POINT('Ctrl Pts',(-11.1379061056826,14.6037786297008,3.19618100597327));
#96058=CARTESIAN_POINT('Ctrl Pts',(-11.1407961178374,14.6045438366155,3.20724678682331));
#96059=CARTESIAN_POINT('Ctrl Pts',(-11.1420326659282,14.6048804482213,3.21210832780949));
#96060=CARTESIAN_POINT('Ctrl Pts',(-11.1445565337842,14.6055873135629,3.22230321504608));
#96061=CARTESIAN_POINT('Ctrl Pts',(-11.1458377157719,14.6059577542987,3.22763794178963));
#96062=CARTESIAN_POINT('Ctrl Pts',(-11.1491017603532,14.6069329896048,3.24165990363266));
#96063=CARTESIAN_POINT('Ctrl Pts',(-11.1510233572469,14.6075397132775,3.25036089147095));
#96064=CARTESIAN_POINT('Ctrl Pts',(-11.1594578830813,14.6103619483928,3.29072207339611));
#96065=CARTESIAN_POINT('Ctrl Pts',(-11.1647638707397,14.6126149812722,3.32261734028262));
#96066=CARTESIAN_POINT('Ctrl Pts',(-11.1763434941637,14.6192644761263,3.41575273252678));
#96067=CARTESIAN_POINT('Ctrl Pts',(-11.1791375169418,14.6237526012896,3.47731205517231));
#96068=CARTESIAN_POINT('Ctrl Pts',(-11.1748179598547,14.6333779572823,3.60835592588375));
#96069=CARTESIAN_POINT('Ctrl Pts',(-11.1663645580411,14.6385053416449,3.67757754631164));
#96070=CARTESIAN_POINT('Ctrl Pts',(-11.1498404660047,14.6440551964034,3.75505772550908));
#96071=CARTESIAN_POINT('Ctrl Pts',(-11.1477194673653,14.6447237242449,3.76443823420712));
#96072=CARTESIAN_POINT('Ctrl Pts',(-11.1446277623481,14.6456399096332,3.77737322405927));
#96073=CARTESIAN_POINT('Ctrl Pts',(-11.1437549982144,14.6458926785666,3.78095039551506));
#96074=CARTESIAN_POINT('Ctrl Pts',(-11.14222778275,14.6463250475456,3.78708486930395));
#96075=CARTESIAN_POINT('Ctrl Pts',(-11.1415814905393,14.6465050993879,3.78964414490782));
#96076=CARTESIAN_POINT('Ctrl Pts',(-11.1402117380909,14.6468806452424,3.79499246887314));
#96077=CARTESIAN_POINT('Ctrl Pts',(-11.1394866398779,14.6470760377021,3.7977810641469));
#96078=CARTESIAN_POINT('Ctrl Pts',(-11.1376878728838,14.647552593278,3.80459601156371));
#96079=CARTESIAN_POINT('Ctrl Pts',(-11.1366030414523,14.6478331247181,3.80861943206589));
#96080=CARTESIAN_POINT('Ctrl Pts',(-11.1326007551473,14.6488439815732,3.82315572261975));
#96081=CARTESIAN_POINT('Ctrl Pts',(-11.1295585046124,14.649567563875,3.8336340770661));
#96082=CARTESIAN_POINT('Ctrl Pts',(-11.1215761474008,14.6513628282342,3.85976573276624));
#96083=CARTESIAN_POINT('Ctrl Pts',(-11.1164534998664,14.6524258613976,3.87536126106499));
#96084=CARTESIAN_POINT('Ctrl Pts',(-11.0922976195768,14.6570897821305,3.94402609322861));
#96085=CARTESIAN_POINT('Ctrl Pts',(-11.0697931896519,14.660564878311,3.99579914885226));
#96086=CARTESIAN_POINT('Ctrl Pts',(-11.0070677092594,14.6689323507665,4.11574906915157));
#96087=CARTESIAN_POINT('Ctrl Pts',(-10.9635290856411,14.6738241333205,4.18186651266068));
#96088=CARTESIAN_POINT('Ctrl Pts',(-10.904187954839,14.679957554904,4.25482894444066));
#96089=CARTESIAN_POINT('Ctrl Pts',(-10.8944467441091,14.6809494502705,4.26634690655712));
#96090=CARTESIAN_POINT('Ctrl Pts',(-10.8800917572543,14.6823919644239,4.28267354379114));
#96091=CARTESIAN_POINT('Ctrl Pts',(-10.8756539176771,14.6828353779541,4.28763544278683));
#96092=CARTESIAN_POINT('Ctrl Pts',(-10.867774167674,14.6836184310265,4.29629679508238));
#96093=CARTESIAN_POINT('Ctrl Pts',(-10.8643500382866,14.6839573212684,4.30001225108902));
#96094=CARTESIAN_POINT('Ctrl Pts',(-10.8572294932593,14.6846592843272,4.30763953802919));
#96095=CARTESIAN_POINT('Ctrl Pts',(-10.8535299654313,14.6850224849354,4.31154828811887));
#96096=CARTESIAN_POINT('Ctrl Pts',(-10.8439660795996,14.6859576674552,4.32151531406117));
#96097=CARTESIAN_POINT('Ctrl Pts',(-10.8380633022015,14.6865312974635,4.32753613202968));
#96098=CARTESIAN_POINT('Ctrl Pts',(-10.8126936804446,14.6889822300687,4.35286325056157));
#96099=CARTESIAN_POINT('Ctrl Pts',(-10.7926219113799,14.6908860001182,4.37154863987784));
#96100=CARTESIAN_POINT('Ctrl Pts',(-10.6966923128343,14.6998335084222,4.45479595326924));
#96101=CARTESIAN_POINT('Ctrl Pts',(-10.6134963568994,14.7072222902762,4.51026320103002));
#96102=CARTESIAN_POINT('Ctrl Pts',(-10.5045672352622,14.716089569558,4.56442211459493));
#96103=CARTESIAN_POINT('Ctrl Pts',(-10.4845237998406,14.7176885834136,4.57369423657419));
#96104=CARTESIAN_POINT('Ctrl Pts',(-10.4440561498682,14.7208385313725,4.59105044667915));
#96105=CARTESIAN_POINT('Ctrl Pts',(-10.4236420457738,14.7223891122854,4.59913807586688));
#96106=CARTESIAN_POINT('Ctrl Pts',(-10.397821672339,14.7242928332241,4.60854115614481));
#96107=CARTESIAN_POINT('Ctrl Pts',(-10.3926177189635,14.7246736360258,4.61039493317248));
#96108=CARTESIAN_POINT('Ctrl Pts',(-10.3843709103189,14.7252723469188,4.61326742507414));
#96109=CARTESIAN_POINT('Ctrl Pts',(-10.3813366865582,14.7254916167272,4.61431040941936));
#96110=CARTESIAN_POINT('Ctrl Pts',(-10.3759095565038,14.7258819586494,4.61615116798269));
#96111=CARTESIAN_POINT('Ctrl Pts',(-10.3735183617617,14.726053298851,4.61695365081446));
#96112=CARTESIAN_POINT('Ctrl Pts',(-10.3677752047501,14.7264632983501,4.61886054358723));
#96113=CARTESIAN_POINT('Ctrl Pts',(-10.3644208374066,14.7267015264306,4.61995757567266));
#96114=CARTESIAN_POINT('Ctrl Pts',(-10.354200033012,14.7274237960078,4.62324946611672));
#96115=CARTESIAN_POINT('Ctrl Pts',(-10.3473181741079,14.7279051644054,4.62539642743313));
#96116=CARTESIAN_POINT('Ctrl Pts',(-10.2756307801387,14.7328724757502,4.64704079557005));
#96117=CARTESIAN_POINT('Ctrl Pts',(-10.209268916036,14.7370768447313,4.66098415906031));
#96118=CARTESIAN_POINT('Ctrl Pts',(-10.0526088267597,14.7468413105054,4.68002055041062));
#96119=CARTESIAN_POINT('Ctrl Pts',(-9.96220888246291,14.752375586307,4.68058705396627));
#96120=CARTESIAN_POINT('Ctrl Pts',(-9.85807423215819,14.759211889364,4.66925899073041));
#96121=CARTESIAN_POINT('Ctrl Pts',(-9.84354741707947,14.7601753391968,4.66740398717299));
#96122=CARTESIAN_POINT('Ctrl Pts',(-9.822549914558,14.761583847056,4.66432375905274));
#96123=CARTESIAN_POINT('Ctrl Pts',(-9.81604858625527,14.7620221726441,4.66331432688812));
#96124=CARTESIAN_POINT('Ctrl Pts',(-9.80458246338393,14.7627993048742,4.66143551297271));
#96125=CARTESIAN_POINT('Ctrl Pts',(-9.79961411075584,14.7631373977517,4.66058862584926));
#96126=CARTESIAN_POINT('Ctrl Pts',(-9.78932077478975,14.7638407385948,4.65876599587258));
#96127=CARTESIAN_POINT('Ctrl Pts',(-9.7839967870726,14.764206132854,4.65778537710453));
#96128=CARTESIAN_POINT('Ctrl Pts',(-9.77025545296731,14.7651534797669,4.65515629832833));
#96129=CARTESIAN_POINT('Ctrl Pts',(-9.76184913977029,14.76573716417,4.65345255275223));
#96130=CARTESIAN_POINT('Ctrl Pts',(-9.72528433804273,14.7682946193264,4.64562505033576));
#96131=CARTESIAN_POINT('Ctrl Pts',(-9.69733951064603,14.7702978151118,4.63856129770724));
#96132=CARTESIAN_POINT('Ctrl Pts',(-9.57506298427151,14.7792869260106,4.6028331995487));
#96133=CARTESIAN_POINT('Ctrl Pts',(-9.48429642910721,14.7866026902786,4.56341748961802));
#96134=CARTESIAN_POINT('Ctrl Pts',(-9.36374275962097,14.7968134426532,4.49196839633069));
#96135=CARTESIAN_POINT('Ctrl Pts',(-9.32911062641871,14.7998057207872,4.46888225025379));
#96136=CARTESIAN_POINT('Ctrl Pts',(-9.29098534403438,14.8031113213706,4.44044080147653));
#96137=CARTESIAN_POINT('Ctrl Pts',(-9.28622858114858,14.8035239464685,4.4368356573072));
#96138=CARTESIAN_POINT('Ctrl Pts',(-9.27865071997443,14.8041813360847,4.43100118336367));
#96139=CARTESIAN_POINT('Ctrl Pts',(-9.27581214181668,14.8044275975322,4.42879488270785));
#96140=CARTESIAN_POINT('Ctrl Pts',(-9.27078069243108,14.8048640556388,4.42484707103445));
#96141=CARTESIAN_POINT('Ctrl Pts',(-9.26858387747804,14.8050546015021,4.42311069740831));
#96142=CARTESIAN_POINT('Ctrl Pts',(-9.26386885074058,14.8054635152451,4.4193565172298));
#96143=CARTESIAN_POINT('Ctrl Pts',(-9.26135272977089,14.8056817015405,4.4173361900079));
#96144=CARTESIAN_POINT('Ctrl Pts',(-9.25437246248923,14.8062870270788,4.41168402189543));
#96145=CARTESIAN_POINT('Ctrl Pts',(-9.24992650935375,14.8066726116267,4.40802970351166));
#96146=CARTESIAN_POINT('Ctrl Pts',(-9.22387628788555,14.8089332918791,4.38629602245145));
#96147=CARTESIAN_POINT('Ctrl Pts',(-9.20289755326056,14.8107597283598,4.36747717169165));
#96148=CARTESIAN_POINT('Ctrl Pts',(-9.12900729872061,14.8173021317855,4.29624777018278));
#96149=CARTESIAN_POINT('Ctrl Pts',(-9.08041994396663,14.8218301556969,4.23960320358204));
#96150=CARTESIAN_POINT('Ctrl Pts',(-9.00095229601274,14.8304010415379,4.1269141621821));
#96151=CARTESIAN_POINT('Ctrl Pts',(-8.96865184613659,14.8344014863188,4.07222114662977));
#96152=CARTESIAN_POINT('Ctrl Pts',(-8.93660820337859,14.8392141266783,4.00634947520666));
#96153=CARTESIAN_POINT('Ctrl Pts',(-8.93241459642619,14.8398642674036,3.99744678171769));
#96154=CARTESIAN_POINT('Ctrl Pts',(-8.92573363936063,14.8409346830287,3.98278994282049));
#96155=CARTESIAN_POINT('Ctrl Pts',(-8.92317974014707,14.841352689457,3.97706652355469));
#96156=CARTESIAN_POINT('Ctrl Pts',(-8.91867632547232,14.8421060378849,3.96675371875761));
#96157=CARTESIAN_POINT('Ctrl Pts',(-8.91671002983823,14.8424408026741,3.96217178873578));
#96158=CARTESIAN_POINT('Ctrl Pts',(-8.91258472669379,14.8431558211076,3.95238789416552));
#96159=CARTESIAN_POINT('Ctrl Pts',(-8.91043382796299,14.8435363375505,3.94718266765402));
#96160=CARTESIAN_POINT('Ctrl Pts',(-8.90472690878862,14.8445672450048,3.93308615424925));
#96161=CARTESIAN_POINT('Ctrl Pts',(-8.90124192215698,14.8452199833791,3.92416675762203));
#96162=CARTESIAN_POINT('Ctrl Pts',(-8.88342201305638,14.848684774279,3.87686512721869));
#96163=CARTESIAN_POINT('Ctrl Pts',(-8.87099005429562,14.8515585665808,3.83780107855562));
#96164=CARTESIAN_POINT('Ctrl Pts',(-8.83456994791559,14.8618427957405,3.69863216364627));
#96165=CARTESIAN_POINT('Ctrl Pts',(-8.82167971737458,14.8695451621305,3.59612227437252));
#96166=CARTESIAN_POINT('Ctrl Pts',(-8.82241038998768,14.8786952191972,3.46864150248868));
#96167=CARTESIAN_POINT('Ctrl Pts',(-8.82332268216843,14.8804383357746,3.44404161405692));
#96168=CARTESIAN_POINT('Ctrl Pts',(-8.82539670375381,14.8825415351595,3.41377387075647));
#96169=CARTESIAN_POINT('Ctrl Pts',(-8.82582980620738,14.882936454466,3.40806410785191));
#96170=CARTESIAN_POINT('Ctrl Pts',(-8.82657437265931,14.8835523750952,3.39911416248918));
#96171=CARTESIAN_POINT('Ctrl Pts',(-8.82685764804543,14.8837748672258,3.39587182028009));
#96172=CARTESIAN_POINT('Ctrl Pts',(-8.82740926856241,14.8841871066834,3.38984621164526));
#96173=CARTESIAN_POINT('Ctrl Pts',(-8.82767408249321,14.8843770369204,3.3870627433592));
#96174=CARTESIAN_POINT('Ctrl Pts',(-8.82830387567952,14.8848111726653,3.38068397723092));
#96175=CARTESIAN_POINT('Ctrl Pts',(-8.82867549102864,14.8850550076705,3.37708939592085));
#96176=CARTESIAN_POINT('Ctrl Pts',(-8.82988463869388,14.8858118444432,3.36589733248134));
#96177=CARTESIAN_POINT('Ctrl Pts',(-8.83077960961855,14.8863217861112,3.35830606743831));
#96178=CARTESIAN_POINT('Ctrl Pts',(-8.83305142829184,14.8875092764791,3.34052656990169));
#96179=CARTESIAN_POINT('Ctrl Pts',(-8.83448791102983,14.8881839215533,3.33034644009327));
#96180=CARTESIAN_POINT('Ctrl Pts',(-8.84007543750577,14.8905661542634,3.29417817271374));
#96181=CARTESIAN_POINT('Ctrl Pts',(-8.84496417718864,14.8922429639983,3.26831043742945));
#96182=CARTESIAN_POINT('Ctrl Pts',(-8.86885246286306,14.8991245716152,3.1616388672475));
#96183=CARTESIAN_POINT('Ctrl Pts',(-8.89549862713555,14.9041474763056,3.08279426334177));
#96184=CARTESIAN_POINT('Ctrl Pts',(-8.94888091858975,14.9121800298246,2.96686228332463));
#96185=CARTESIAN_POINT('Ctrl Pts',(-8.96983612135003,14.9150366982327,2.92741915022942));
#96186=CARTESIAN_POINT('Ctrl Pts',(-8.99820566270971,14.9186362252825,2.88064159187921));
#96187=CARTESIAN_POINT('Ctrl Pts',(-9.00354475615701,14.9193034491926,2.8720878496451));
#96188=CARTESIAN_POINT('Ctrl Pts',(-9.01212802464166,14.9203609145502,2.85872183356845));
#96189=CARTESIAN_POINT('Ctrl Pts',(-9.01529914929462,14.9207484712044,2.85386304933259));
#96190=CARTESIAN_POINT('Ctrl Pts',(-9.0212268379329,14.9214673082475,2.84492565947373));
#96191=CARTESIAN_POINT('Ctrl Pts',(-9.02397333398012,14.9217982084992,2.84084050461848));
#96192=CARTESIAN_POINT('Ctrl Pts',(-9.03013288883432,14.9225356287542,2.8318016488143));
#96193=CARTESIAN_POINT('Ctrl Pts',(-9.03355843457985,14.9229426123702,2.82685666597219));
#96194=CARTESIAN_POINT('Ctrl Pts',(-9.04356834698078,14.9241230915321,2.81264066214283));
#96195=CARTESIAN_POINT('Ctrl Pts',(-9.05024913575004,14.9249002304131,2.80343869882319));
#96196=CARTESIAN_POINT('Ctrl Pts',(-9.1069787832802,14.9314137302726,2.72763423188245));
#96197=CARTESIAN_POINT('Ctrl Pts',(-9.16382208758642,14.9374250002639,2.66643109383375));
#96198=CARTESIAN_POINT('Ctrl Pts',(-9.28411001039993,14.9491220011564,2.5617011230202));
#96199=CARTESIAN_POINT('Ctrl Pts',(-9.34631482058239,14.9547585212957,2.5173500529682));
#96200=CARTESIAN_POINT('Ctrl Pts',(-9.42043600508338,14.9607458557213,2.47467703485501));
#96201=CARTESIAN_POINT('Ctrl Pts',(-9.42855329944845,14.9613922503499,2.4701309359869));
#96202=CARTESIAN_POINT('Ctrl Pts',(-9.43991588032141,14.9622833492175,2.46394302682071));
#96203=CARTESIAN_POINT('Ctrl Pts',(-9.44311592341879,14.9625328128592,2.46221948422438));
#96204=CARTESIAN_POINT('Ctrl Pts',(-9.44864273048926,14.9629610247593,2.45927567240799));
#96205=CARTESIAN_POINT('Ctrl Pts',(-9.45096566917556,14.9631402059725,2.45804833672202));
#96206=CARTESIAN_POINT('Ctrl Pts',(-9.45585524913933,14.9635156622435,2.4554857958263));
#96207=CARTESIAN_POINT('Ctrl Pts',(-9.45842273393063,14.963711827104,2.45415225879698));
#96208=CARTESIAN_POINT('Ctrl Pts',(-9.46475319388827,14.964193141046,2.4508938166906));
#96209=CARTESIAN_POINT('Ctrl Pts',(-9.46852171487081,14.964477628646,2.44897965713209));
#96210=CARTESIAN_POINT('Ctrl Pts',(-9.4824158605233,14.9655193316351,2.4420161902041));
#96211=CARTESIAN_POINT('Ctrl Pts',(-9.49260418409054,14.9662692526915,2.43709238753589));
#96212=CARTESIAN_POINT('Ctrl Pts',(-9.5184918678138,14.9681437681776,2.42503850091484));
#96213=CARTESIAN_POINT('Ctrl Pts',(-9.53428016873737,14.9692587043117,2.41810471426228));
#96214=CARTESIAN_POINT('Ctrl Pts',(-9.60741140232171,14.9743196859778,2.38788526934962));
#96215=CARTESIAN_POINT('Ctrl Pts',(-9.66638524333647,14.9781173908488,2.36879384822741));
#96216=CARTESIAN_POINT('Ctrl Pts',(-9.75456087925998,14.9837249510963,2.34774932249269));
#96217=CARTESIAN_POINT('Ctrl Pts',(-9.78275116732423,14.985506817339,2.34210401195159));
#96218=CARTESIAN_POINT('Ctrl Pts',(-9.81110406371068,14.9873061497326,2.3374969300026));
#96219=CARTESIAN_POINT('Origin',(-10.,12.3756328852638,3.5));
#96220=CARTESIAN_POINT('',(-9.81110406370779,15.5854602598056,2.33749693000307));
#96221=CARTESIAN_POINT('',(-9.81110406371068,15.4869977587645,2.3374969300026));
#96222=CARTESIAN_POINT('',(-9.81110406371068,12.3756328852638,2.3374969300026));
#96223=CARTESIAN_POINT('',(-11.177749800465,15.2252691226695,3.49931443112735));
#96224=CARTESIAN_POINT('Ctrl Pts',(-9.8111040637049,15.5854602598056,2.33749693000354));
#96225=CARTESIAN_POINT('Ctrl Pts',(-9.80497997839647,15.5850478740051,2.33849203690528));
#96226=CARTESIAN_POINT('Ctrl Pts',(-9.79886362718618,15.584637878246,2.33953555748687));
#96227=CARTESIAN_POINT('Ctrl Pts',(-9.77690176011872,15.5831715139842,2.34346136555285));
#96228=CARTESIAN_POINT('Ctrl Pts',(-9.76110689590806,15.5821277871477,2.34662036760273));
#96229=CARTESIAN_POINT('Ctrl Pts',(-9.69222399029384,15.5776042086662,2.36187294157862));
#96230=CARTESIAN_POINT('Ctrl Pts',(-9.63994279147801,15.5742425680384,2.37731615278718));
#96231=CARTESIAN_POINT('Ctrl Pts',(-9.51254385567699,15.5658386917472,2.42476831621584));
#96232=CARTESIAN_POINT('Ctrl Pts',(-9.43934172860403,15.5608006364909,2.46105974364422));
#96233=CARTESIAN_POINT('Ctrl Pts',(-9.35777022547683,15.5545056865252,2.51264901278325));
#96234=CARTESIAN_POINT('Ctrl Pts',(-9.34522040918453,15.5535170920549,2.52092660682595));
#96235=CARTESIAN_POINT('Ctrl Pts',(-9.32735333313186,15.5520784311383,2.53320853446642));
#96236=CARTESIAN_POINT('Ctrl Pts',(-9.321905847371,15.551635513586,2.5370214989951));
#96237=CARTESIAN_POINT('Ctrl Pts',(-9.31237623576086,15.5508529480452,2.54381270048421));
#96238=CARTESIAN_POINT('Ctrl Pts',(-9.30828040701381,15.5505140453434,2.54677148793252));
#96239=CARTESIAN_POINT('Ctrl Pts',(-9.29985686714895,15.5498116760611,2.55293945124579));
#96240=CARTESIAN_POINT('Ctrl Pts',(-9.29553189175542,15.5494480792905,2.55615214558587));
#96241=CARTESIAN_POINT('Ctrl Pts',(-9.28447857322339,15.5485110669654,2.56448110870179));
#96242=CARTESIAN_POINT('Ctrl Pts',(-9.27778308732061,15.5479359918963,2.56964026704523));
#96243=CARTESIAN_POINT('Ctrl Pts',(-9.24946641369543,15.545471199995,2.59194935026712));
#96244=CARTESIAN_POINT('Ctrl Pts',(-9.22839764286046,15.5435546453094,2.60978304409426));
#96245=CARTESIAN_POINT('Ctrl Pts',(-9.13433484186276,15.5345995569571,2.69525203735334));
#96246=CARTESIAN_POINT('Ctrl Pts',(-9.06947770343406,15.527217691094,2.77122172524814));
#96247=CARTESIAN_POINT('Ctrl Pts',(-9.00283768800216,15.5183566656608,2.87290281522489));
#96248=CARTESIAN_POINT('Ctrl Pts',(-8.99124471207531,15.5167561491735,2.89172669079959));
#96249=CARTESIAN_POINT('Ctrl Pts',(-8.96927072961381,15.5136141533542,2.92976447832821));
#96250=CARTESIAN_POINT('Ctrl Pts',(-8.95888012308026,15.5120727559877,2.94896376721643));
#96251=CARTESIAN_POINT('Ctrl Pts',(-8.9465394495763,15.5101785552789,2.97336317809581));
#96252=CARTESIAN_POINT('Ctrl Pts',(-8.94408505144539,15.5097984136241,2.97830171756258));
#96253=CARTESIAN_POINT('Ctrl Pts',(-8.94025833212916,15.5092004645616,2.98613917829176));
#96254=CARTESIAN_POINT('Ctrl Pts',(-8.93886304627302,15.5089813016404,2.98902670053372));
#96255=CARTESIAN_POINT('Ctrl Pts',(-8.93639086798018,15.5085909785756,2.99419663366376));
#96256=CARTESIAN_POINT('Ctrl Pts',(-8.93530952245058,15.5084195515121,2.99647679466824));
#96257=CARTESIAN_POINT('Ctrl Pts',(-8.93273131592822,15.5080091188783,3.00195872682732));
#96258=CARTESIAN_POINT('Ctrl Pts',(-8.93124152936349,15.5077705466124,3.00516377856169));
#96259=CARTESIAN_POINT('Ctrl Pts',(-8.92674767615076,15.5070464290515,3.01494659886172));
#96260=CARTESIAN_POINT('Ctrl Pts',(-8.92378967162901,15.5065635760108,3.02154552129065));
#96261=CARTESIAN_POINT('Ctrl Pts',(-8.89759106263942,15.5022259430144,3.08146371763057));
#96262=CARTESIAN_POINT('Ctrl Pts',(-8.87826593986942,15.4985782748313,3.13641685949991));
#96263=CARTESIAN_POINT('Ctrl Pts',(-8.83664217166861,15.4886820186467,3.29035262503834));
#96264=CARTESIAN_POINT('Ctrl Pts',(-8.82292928160331,15.4825140124548,3.39111505943759));
#96265=CARTESIAN_POINT('Ctrl Pts',(-8.82218706975079,15.4750067508844,3.50592792649185));
#96266=CARTESIAN_POINT('Ctrl Pts',(-8.82233308625764,15.4741146523486,3.51946932382251));
#96267=CARTESIAN_POINT('Ctrl Pts',(-8.82289324673785,15.4727871272006,3.53945038335277));
#96268=CARTESIAN_POINT('Ctrl Pts',(-8.82312687570919,15.4723572819168,3.54589431180603));
#96269=CARTESIAN_POINT('Ctrl Pts',(-8.82363591445121,15.4715907159037,3.55733823977421));
#96270=CARTESIAN_POINT('Ctrl Pts',(-8.8238903210968,15.4712546547294,3.56233905174174));
#96271=CARTESIAN_POINT('Ctrl Pts',(-8.82449280984534,15.4705453200025,3.57285941340306));
#96272=CARTESIAN_POINT('Ctrl Pts',(-8.82484789534452,15.4701718367676,3.57837842396655));
#96273=CARTESIAN_POINT('Ctrl Pts',(-8.82589047010176,15.4691801793425,3.59297736720144));
#96274=CARTESIAN_POINT('Ctrl Pts',(-8.82664440411178,15.4685599572445,3.60205202836472));
#96275=CARTESIAN_POINT('Ctrl Pts',(-8.83076578604388,15.4655687024723,3.64554054904665));
#96276=CARTESIAN_POINT('Ctrl Pts',(-8.83554216272774,15.4631544213527,3.67980049146867));
#96277=CARTESIAN_POINT('Ctrl Pts',(-8.85387899485703,15.4559798897554,3.77913444296485));
#96278=CARTESIAN_POINT('Ctrl Pts',(-8.8714458742821,15.4511138615483,3.84332658666985));
#96279=CARTESIAN_POINT('Ctrl Pts',(-8.91563961387797,15.4416929990599,3.96377338156195));
#96280=CARTESIAN_POINT('Ctrl Pts',(-8.94149831566611,15.4371562621329,4.02009512604862));
#96281=CARTESIAN_POINT('Ctrl Pts',(-8.97641790205619,15.4321366740237,4.08264035539016));
#96282=CARTESIAN_POINT('Ctrl Pts',(-8.98127576595169,15.4314588385059,4.09109309367742));
#96283=CARTESIAN_POINT('Ctrl Pts',(-8.98812161176306,15.4305322371013,4.10266979416489));
#96284=CARTESIAN_POINT('Ctrl Pts',(-8.99002003479769,15.4302782071096,4.10584587495526));
#96285=CARTESIAN_POINT('Ctrl Pts',(-8.99330112077183,15.4298442090149,4.11127688060304));
#96286=CARTESIAN_POINT('Ctrl Pts',(-8.99467645463314,15.4296637820819,4.11353616656569));
#96287=CARTESIAN_POINT('Ctrl Pts',(-8.99756438642479,15.4292880508206,4.11824444058674));
#96288=CARTESIAN_POINT('Ctrl Pts',(-8.9990783659331,15.4290928451208,4.12069254093943));
#96289=CARTESIAN_POINT('Ctrl Pts',(-9.00279620870083,15.4286177161067,4.12665530444166));
#96290=CARTESIAN_POINT('Ctrl Pts',(-9.00500972416929,15.4283384149822,4.13016396617993));
#96291=CARTESIAN_POINT('Ctrl Pts',(-9.01304220243794,15.4273373728062,4.14274847085491));
#96292=CARTESIAN_POINT('Ctrl Pts',(-9.01896739133281,15.4266222028266,4.15175634410521));
#96293=CARTESIAN_POINT('Ctrl Pts',(-9.03407546891208,15.424852136019,4.17405169813914));
#96294=CARTESIAN_POINT('Ctrl Pts',(-9.04340976598194,15.4238055785717,4.18723436330639));
#96295=CARTESIAN_POINT('Ctrl Pts',(-9.08554765861703,15.419261736104,4.24422211100597));
#96296=CARTESIAN_POINT('Ctrl Pts',(-9.12111233029219,15.415883741409,4.28590524180874));
#96297=CARTESIAN_POINT('Ctrl Pts',(-9.21627615992236,15.4074855073915,4.38286675718949));
#96298=CARTESIAN_POINT('Ctrl Pts',(-9.27892561369515,15.402468800792,4.43473332766982));
#96299=CARTESIAN_POINT('Ctrl Pts',(-9.35891722482121,15.3961973419562,4.48809626133481));
#96300=CARTESIAN_POINT('Ctrl Pts',(-9.37158929024165,15.395208122119,4.49620343937413));
#96301=CARTESIAN_POINT('Ctrl Pts',(-9.39008289854408,15.3937687142639,4.50754177490907));
#96302=CARTESIAN_POINT('Ctrl Pts',(-9.39578234549652,15.3933256856728,4.5109699905384));
#96303=CARTESIAN_POINT('Ctrl Pts',(-9.40586241323323,15.3925429905768,4.51691746161065));
#96304=CARTESIAN_POINT('Ctrl Pts',(-9.41023082066017,15.3922040701362,4.51945716412018));
#96305=CARTESIAN_POINT('Ctrl Pts',(-9.41928983776777,15.3915017292105,4.52464617782961));
#96306=CARTESIAN_POINT('Ctrl Pts',(-9.42398254383709,15.391138178932,4.52729157048406));
#96307=CARTESIAN_POINT('Ctrl Pts',(-9.43608195233882,15.3902014246819,4.53400333242571));
#96308=CARTESIAN_POINT('Ctrl Pts',(-9.44351445867763,15.3896265629591,4.53802229829774));
#96309=CARTESIAN_POINT('Ctrl Pts',(-9.4753786754746,15.3871639904873,4.55481159774689));
#96310=CARTESIAN_POINT('Ctrl Pts',(-9.50020969459478,15.3852495021509,4.56680104596345));
#96311=CARTESIAN_POINT('Ctrl Pts',(-9.6165223649936,15.3762952418274,4.6180092589184));
#96312=CARTESIAN_POINT('Ctrl Pts',(-9.71231518810764,15.3689118162868,4.64639928008942));
#96313=CARTESIAN_POINT('Ctrl Pts',(-9.83232309546905,15.3600493210264,4.66596221879791));
#96314=CARTESIAN_POINT('Ctrl Pts',(-9.85423129963794,15.3584489743901,4.66890334069077));
#96315=CARTESIAN_POINT('Ctrl Pts',(-9.89792808957471,15.3553060978113,4.67352175962943));
#96316=CARTESIAN_POINT('Ctrl Pts',(-9.91970731040881,15.3537636800646,4.67521284388546));
#96317=CARTESIAN_POINT('Ctrl Pts',(-9.94703157128658,15.3518684119954,4.6765712184568));
#96318=CARTESIAN_POINT('Ctrl Pts',(-9.95254255984136,15.351488187589,4.67680639058072));
#96319=CARTESIAN_POINT('Ctrl Pts',(-9.96126026912912,15.3508901375277,4.67711706372251));
#96320=CARTESIAN_POINT('Ctrl Pts',(-9.96446590889335,15.3506709556178,4.67721819449417));
#96321=CARTESIAN_POINT('Ctrl Pts',(-9.97019458475274,15.3502806165287,4.67737550004441));
#96322=CARTESIAN_POINT('Ctrl Pts',(-9.97271737522506,15.3501091922898,4.67743666048219));
#96323=CARTESIAN_POINT('Ctrl Pts',(-9.97877353729265,15.3496987892744,4.67756400600079));
#96324=CARTESIAN_POINT('Ctrl Pts',(-9.98230703057967,15.3494602436205,4.67762239729099));
#96325=CARTESIAN_POINT('Ctrl Pts',(-9.99306942488246,15.3487362881248,4.67775179487399));
#96326=CARTESIAN_POINT('Ctrl Pts',(-10.0002989300676,15.3482535687784,4.67777215127619));
#96327=CARTESIAN_POINT('Ctrl Pts',(-10.0656196288155,15.3439207760291,4.67735460125613));
#96328=CARTESIAN_POINT('Ctrl Pts',(-10.1236124619663,15.3402773097701,4.67268566257046));
#96329=CARTESIAN_POINT('Ctrl Pts',(-10.2812022703571,15.3303794258593,4.64817136583203));
#96330=CARTESIAN_POINT('Ctrl Pts',(-10.3789309832042,15.3242062154971,4.61972383351043));
#96331=CARTESIAN_POINT('Ctrl Pts',(-10.4842049936918,15.3166935073353,4.57369625673667));
#96332=CARTESIAN_POINT('Ctrl Pts',(-10.4965072739199,15.3158021538,4.56806302715288));
#96333=CARTESIAN_POINT('Ctrl Pts',(-10.5145230441135,15.3144755276765,4.55943506183962));
#96334=CARTESIAN_POINT('Ctrl Pts',(-10.5203136554389,15.3140458253088,4.55660319437225));
#96335=CARTESIAN_POINT('Ctrl Pts',(-10.5304012041859,15.3132913254447,4.55156690012374));
#96336=CARTESIAN_POINT('Ctrl Pts',(-10.5347084114321,15.3129672548892,4.54938329336373));
#96337=CARTESIAN_POINT('Ctrl Pts',(-10.5391410849613,15.3126317331571,4.54710170349962));
#96338=CARTESIAN_POINT('Ctrl Pts',(-10.539280142287,15.3126212054605,4.54703009273848));
#96339=CARTESIAN_POINT('Ctrl Pts',(-10.5395852440368,15.3125981024381,4.54687289668485));
#96340=CARTESIAN_POINT('Ctrl Pts',(-10.5397512823491,15.3125855267004,4.54678729959723));
#96341=CARTESIAN_POINT('Ctrl Pts',(-10.5400344625771,15.3125640736426,4.54664122750279));
#96342=CARTESIAN_POINT('Ctrl Pts',(-10.5401516147559,15.3125551970149,4.5465807723038));
#96343=CARTESIAN_POINT('Ctrl Pts',(-10.5403511731348,15.3125400739787,4.54647774978475));
#96344=CARTESIAN_POINT('Ctrl Pts',(-10.5404335844838,15.312533827917,4.54643519238637));
#96345=CARTESIAN_POINT('Ctrl Pts',(-10.5406174607539,15.3125198900865,4.54634021076868));
#96346=CARTESIAN_POINT('Ctrl Pts',(-10.5407189230572,15.3125121981432,4.54628778153586));
#96347=CARTESIAN_POINT('Ctrl Pts',(-10.5457612505635,15.312129880544,4.54368129963983));
#96348=CARTESIAN_POINT('Ctrl Pts',(-10.5506838942261,15.3117540373113,4.54109233242541));
#96349=CARTESIAN_POINT('Ctrl Pts',(-10.563981795412,15.3107315611732,4.53397786277853));
#96350=CARTESIAN_POINT('Ctrl Pts',(-10.5723206695486,15.31008259189,4.52938560715));
#96351=CARTESIAN_POINT('Ctrl Pts',(-10.5906765951926,15.3086363238807,4.51898492898944));
#96352=CARTESIAN_POINT('Ctrl Pts',(-10.6006653957554,15.307837386662,4.51312891155158));
#96353=CARTESIAN_POINT('Ctrl Pts',(-10.6310474746586,15.3053699275826,4.49470991677268));
#96354=CARTESIAN_POINT('Ctrl Pts',(-10.6511441510626,15.3036850291149,4.481671987425));
#96355=CARTESIAN_POINT('Ctrl Pts',(-10.7334473066008,15.2965603845836,4.42463737969575));
#96356=CARTESIAN_POINT('Ctrl Pts',(-10.7917023962785,15.2909473658913,4.37527373097714));
#96357=CARTESIAN_POINT('Ctrl Pts',(-10.8830895676957,15.2813345391011,4.2811986764104));
#96358=CARTESIAN_POINT('Ctrl Pts',(-10.9185990278178,15.2773365879844,4.23911829785002));
#96359=CARTESIAN_POINT('Ctrl Pts',(-10.954977091309,15.2730489588954,4.18931730291256));
#96360=CARTESIAN_POINT('Ctrl Pts',(-10.9588673609428,15.2725877271738,4.18389544401191));
#96361=CARTESIAN_POINT('Ctrl Pts',(-10.9647077442405,15.2718914740571,4.17560790432105));
#96362=CARTESIAN_POINT('Ctrl Pts',(-10.9666915578758,15.2716542912104,4.17276630778495));
#96363=CARTESIAN_POINT('Ctrl Pts',(-10.9702486305052,15.271227826574,4.16762296996047));
#96364=CARTESIAN_POINT('Ctrl Pts',(-10.9718262750049,15.2710382568555,4.16532437704725));
#96365=CARTESIAN_POINT('Ctrl Pts',(-10.9752950118096,15.2706205122952,4.16023184107989));
#96366=CARTESIAN_POINT('Ctrl Pts',(-10.9771822670968,15.2703925928189,4.15743536688117));
#96367=CARTESIAN_POINT('Ctrl Pts',(-10.982637162785,15.269731837673,4.14927709389871));
#96368=CARTESIAN_POINT('Ctrl Pts',(-10.9861729434346,15.2693010500652,4.14389398865759));
#96369=CARTESIAN_POINT('Ctrl Pts',(-11.0149389975124,15.2657730747218,4.09930582152382));
#96370=CARTESIAN_POINT('Ctrl Pts',(-11.0378684037033,15.2628107266906,4.05865815634376));
#96371=CARTESIAN_POINT('Ctrl Pts',(-11.0965276287925,15.2544515883057,3.93852187180898));
#96372=CARTESIAN_POINT('Ctrl Pts',(-11.1259330724032,15.2491782937948,3.8562991985869));
#96373=CARTESIAN_POINT('Ctrl Pts',(-11.1539622040777,15.2414494534809,3.7380249982986));
#96374=CARTESIAN_POINT('Ctrl Pts',(-11.16043689709,15.2392221904702,3.70413358519621));
#96375=CARTESIAN_POINT('Ctrl Pts',(-11.1667307815935,15.2363467634431,3.66098895369808));
#96376=CARTESIAN_POINT('Ctrl Pts',(-11.1679418508406,15.235742458922,3.65195389186633));
#96377=CARTESIAN_POINT('Ctrl Pts',(-11.1697192067958,15.2347661204175,3.63741415344351));
#96378=CARTESIAN_POINT('Ctrl Pts',(-11.1703518080219,15.2343961625815,3.6319178380571));
#96379=CARTESIAN_POINT('Ctrl Pts',(-11.1714661979238,15.2336996369797,3.62159575784115));
#96380=CARTESIAN_POINT('Ctrl Pts',(-11.1719569527852,15.2333733565928,3.61677106152563));
#96381=CARTESIAN_POINT('Ctrl Pts',(-11.1728779720587,15.2327195351027,3.60712495298329));
#96382=CARTESIAN_POINT('Ctrl Pts',(-11.173308337893,15.2323920038548,3.60230364562684));
#96383=CARTESIAN_POINT('Ctrl Pts',(-11.1742220445471,15.2316428848166,3.59130213796457));
#96384=CARTESIAN_POINT('Ctrl Pts',(-11.1746863330126,15.2312207131845,3.58512054258543));
#96385=CARTESIAN_POINT('Ctrl Pts',(-11.1758162101567,15.2300684504547,3.56830025548825));
#96386=CARTESIAN_POINT('Ctrl Pts',(-11.1763861882568,15.2293354365132,3.55765594578078));
#96387=CARTESIAN_POINT('Ctrl Pts',(-11.1774464169547,15.2274976079971,3.53111256017193));
#96388=CARTESIAN_POINT('Ctrl Pts',(-11.177759058463,15.2263882685434,3.51521889493337));
#96389=CARTESIAN_POINT('Ctrl Pts',(-11.177749800465,15.2252691226695,3.49931443112713));
#96390=CARTESIAN_POINT('Ctrl Pts',(-11.177749800465,15.2252691226695,3.49931443112735));
#96391=CARTESIAN_POINT('Ctrl Pts',(-11.1776833668831,15.2172383509074,3.38518711153303));
#96392=CARTESIAN_POINT('Ctrl Pts',(-11.1610284219822,15.2087014221751,3.27169185811116));
#96393=CARTESIAN_POINT('Ctrl Pts',(-11.1196692688029,15.1982875511688,3.13346584831714));
#96394=CARTESIAN_POINT('Ctrl Pts',(-11.1099049574073,15.1961385686007,3.10488242312908));
#96395=CARTESIAN_POINT('Ctrl Pts',(-11.0969444877652,15.1936381828625,3.07123172618874));
#96396=CARTESIAN_POINT('Ctrl Pts',(-11.0947962321001,15.19323374056,3.06577580027221));
#96397=CARTESIAN_POINT('Ctrl Pts',(-11.0913936342866,15.1926086592552,3.05732001782686));
#96398=CARTESIAN_POINT('Ctrl Pts',(-11.0901675028691,15.192386420441,3.0543090219499));
#96399=CARTESIAN_POINT('Ctrl Pts',(-11.087863039499,15.1919743269229,3.04871638972749));
#96400=CARTESIAN_POINT('Ctrl Pts',(-11.0867879837102,15.1917842916463,3.04613353470317));
#96401=CARTESIAN_POINT('Ctrl Pts',(-11.0842999670474,15.1913494933342,3.04021552567359));
#96402=CARTESIAN_POINT('Ctrl Pts',(-11.0828808167649,15.1911051043933,3.03688303968229));
#96403=CARTESIAN_POINT('Ctrl Pts',(-11.0790991015843,15.1904631606693,3.02811514582162));
#96404=CARTESIAN_POINT('Ctrl Pts',(-11.0767108082343,15.1900670903676,3.02269084895906));
#96405=CARTESIAN_POINT('Ctrl Pts',(-11.0577517766247,15.186992851637,2.98049757709027));
#96406=CARTESIAN_POINT('Ctrl Pts',(-11.0393412493931,15.1844148917533,2.94457932968132));
#96407=CARTESIAN_POINT('Ctrl Pts',(-10.970505839098,15.1757855565023,2.8257440998208));
#96408=CARTESIAN_POINT('Ctrl Pts',(-10.9117102467698,15.1699440992857,2.74814376419847));
#96409=CARTESIAN_POINT('Ctrl Pts',(-10.8296294692402,15.1624334948981,2.66379523812977));
#96410=CARTESIAN_POINT('Ctrl Pts',(-10.8148068776277,15.1610998030292,2.64934546605115));
#96411=CARTESIAN_POINT('Ctrl Pts',(-10.7919360972944,15.1590685768218,2.62819636412402));
#96412=CARTESIAN_POINT('Ctrl Pts',(-10.7841663285791,15.1583829389213,2.62120109255491));
#96413=CARTESIAN_POINT('Ctrl Pts',(-10.7697377617936,15.1571168901355,2.608554491469));
#96414=CARTESIAN_POINT('Ctrl Pts',(-10.7631072063315,15.1565377883769,2.60287197042473));
#96415=CARTESIAN_POINT('Ctrl Pts',(-10.7523154979748,15.1555992184905,2.59382945952206));
#96416=CARTESIAN_POINT('Ctrl Pts',(-10.7481934929498,15.1552416351816,2.59042309152715));
#96417=CARTESIAN_POINT('Ctrl Pts',(-10.7403779595496,15.1545652683916,2.58405351627686));
#96418=CARTESIAN_POINT('Ctrl Pts',(-10.736689468107,15.1542467353907,2.58108427454734));
#96419=CARTESIAN_POINT('Ctrl Pts',(-10.7280779298954,15.153504550736,2.57423714468381));
#96420=CARTESIAN_POINT('Ctrl Pts',(-10.723141674674,15.15308024196,2.57037617715715));
#96421=CARTESIAN_POINT('Ctrl Pts',(-10.7103796434105,15.1519859748301,2.56055731330556));
#96422=CARTESIAN_POINT('Ctrl Pts',(-10.7025097546642,15.1513137743737,2.55465782187964));
#96423=CARTESIAN_POINT('Ctrl Pts',(-10.6440044194409,15.1463343595559,2.51193457949146));
#96424=CARTESIAN_POINT('Ctrl Pts',(-10.5905866073816,15.1418766655007,2.47910818689937));
#96425=CARTESIAN_POINT('Ctrl Pts',(-10.4678597453528,15.1318586558835,2.41655592939871));
#96426=CARTESIAN_POINT('Ctrl Pts',(-10.3977866085547,15.1262758118892,2.38891520076487));
#96427=CARTESIAN_POINT('Ctrl Pts',(-10.2983712036894,15.1188237831731,2.36032023452068));
#96428=CARTESIAN_POINT('Ctrl Pts',(-10.2709086493638,15.1168138484527,2.35348172774307));
#96429=CARTESIAN_POINT('Ctrl Pts',(-10.2375855139173,15.1144530957466,2.34644835608135));
#96430=CARTESIAN_POINT('Ctrl Pts',(-10.2319382004814,15.1140556933246,2.34529962926442));
#96431=CARTESIAN_POINT('Ctrl Pts',(-10.2231135140134,15.1134391061994,2.34357194343144));
#96432=CARTESIAN_POINT('Ctrl Pts',(-10.2199419015342,15.1132183890078,2.34296454214207));
#96433=CARTESIAN_POINT('Ctrl Pts',(-10.2140146625963,15.1128076066233,2.34185465845969));
#96434=CARTESIAN_POINT('Ctrl Pts',(-10.2112597624101,15.1126173722187,2.34134896497963));
#96435=CARTESIAN_POINT('Ctrl Pts',(-10.2049652466684,15.112184265859,2.34021673112485));
#96436=CARTESIAN_POINT('Ctrl Pts',(-10.2014245459301,15.1119417526786,2.33959656314632));
#96437=CARTESIAN_POINT('Ctrl Pts',(-10.1920015758282,15.1112991647921,2.33799052103239));
#96438=CARTESIAN_POINT('Ctrl Pts',(-10.1861144706314,15.1109006174054,2.33703308653611));
#96439=CARTESIAN_POINT('Ctrl Pts',(-10.1392815540829,15.1077514198969,2.32978127344454));
#96440=CARTESIAN_POINT('Ctrl Pts',(-10.0980318741861,15.1051065180071,2.32560577691198));
#96441=CARTESIAN_POINT('Ctrl Pts',(-9.974492121498,15.0973427768696,2.31965729954626));
#96442=CARTESIAN_POINT('Ctrl Pts',(-9.89219890068557,15.0923631211769,2.32431977326732));
#96443=CARTESIAN_POINT('Ctrl Pts',(-9.81110406371068,15.0871826612189,2.3374969300026));
#96444=CARTESIAN_POINT('Ctrl Pts',(-9.81110406371068,14.9873061497326,2.3374969300026));
#96445=CARTESIAN_POINT('Ctrl Pts',(-9.85382366066147,14.9900172221248,2.33055539283837));
#96446=CARTESIAN_POINT('Ctrl Pts',(-9.89691233808748,14.9927689462918,2.32597078310509));
#96447=CARTESIAN_POINT('Ctrl Pts',(-9.95524335233313,14.9965779852906,2.32300403118289));
#96448=CARTESIAN_POINT('Ctrl Pts',(-9.97032322240293,14.9975700414155,2.32252731531612));
#96449=CARTESIAN_POINT('Ctrl Pts',(-9.99206440473281,14.9990127471275,2.32225791899193));
#96450=CARTESIAN_POINT('Ctrl Pts',(-9.99872172368918,14.9994561887225,2.32223187935902));
#96451=CARTESIAN_POINT('Ctrl Pts',(-10.0104314715965,15.0002392741427,2.32228535841672));
#96452=CARTESIAN_POINT('Ctrl Pts',(-10.0154838812806,15.0005781684674,2.32234094889161));
#96453=CARTESIAN_POINT('Ctrl Pts',(-10.0259166256504,15.0012801231873,2.32252288596704));
#96454=CARTESIAN_POINT('Ctrl Pts',(-10.0312967558706,15.0016433112713,2.32265360366425));
#96455=CARTESIAN_POINT('Ctrl Pts',(-10.0451024508674,15.0025784259567,2.32308372852481));
#96456=CARTESIAN_POINT('Ctrl Pts',(-10.0535259180664,15.0031520001999,2.32343673744501));
#96457=CARTESIAN_POINT('Ctrl Pts',(-10.0893160365843,15.0056023608956,2.32532175580102));
#96458=CARTESIAN_POINT('Ctrl Pts',(-10.11662656937,15.007505599446,2.32771831074809));
#96459=CARTESIAN_POINT('Ctrl Pts',(-10.24268799486,15.0164528770807,2.3432290209597));
#96460=CARTESIAN_POINT('Ctrl Pts',(-10.3395969898255,15.0238420411843,2.3678849584096));
#96461=CARTESIAN_POINT('Ctrl Pts',(-10.4527630746817,15.0327096782441,2.41253133482747));
#96462=CARTESIAN_POINT('Ctrl Pts',(-10.4730696612519,15.0343086433027,2.42121008141764));
#96463=CARTESIAN_POINT('Ctrl Pts',(-10.5130598745858,15.0374588522303,2.43964784663435));
#96464=CARTESIAN_POINT('Ctrl Pts',(-10.5327392455676,15.0390097340415,2.44939723410744));
#96465=CARTESIAN_POINT('Ctrl Pts',(-10.5570156841951,15.0409137689563,2.46228177757084));
#96466=CARTESIAN_POINT('Ctrl Pts',(-10.561877240778,15.0412945955104,2.46490601832155));
#96467=CARTESIAN_POINT('Ctrl Pts',(-10.5695328867124,15.041893335113,2.46910832389682));
#96468=CARTESIAN_POINT('Ctrl Pts',(-10.5723392251657,15.0421126100963,2.47066372410792));
#96469=CARTESIAN_POINT('Ctrl Pts',(-10.5773402922241,15.0425029561764,2.47346231858933));
#96470=CARTESIAN_POINT('Ctrl Pts',(-10.5795373725677,15.0426742954003,2.4747010882871));
#96471=CARTESIAN_POINT('Ctrl Pts',(-10.584798991138,15.043084285936,2.47769003900725));
#96472=CARTESIAN_POINT('Ctrl Pts',(-10.5878596601965,15.0433225060838,2.47944694546925));
#96473=CARTESIAN_POINT('Ctrl Pts',(-10.5971475350763,15.0440447275684,2.48483408293118));
#96474=CARTESIAN_POINT('Ctrl Pts',(-10.6033494957051,15.0445260563251,2.48850782984524));
#96475=CARTESIAN_POINT('Ctrl Pts',(-10.6671563875382,15.0494725565345,2.52709971393274));
#96476=CARTESIAN_POINT('Ctrl Pts',(-10.7217073613132,15.053658770948,2.56684736044128));
#96477=CARTESIAN_POINT('Ctrl Pts',(-10.8408497092787,15.0634261184581,2.67039100710969));
#96478=CARTESIAN_POINT('Ctrl Pts',(-10.9020601655457,15.068980379451,2.73739620740219));
#96479=CARTESIAN_POINT('Ctrl Pts',(-10.9635536025526,15.0758382424028,2.82259813766731));
#96480=CARTESIAN_POINT('Ctrl Pts',(-10.9718882924676,15.076800183266,2.83461143368669));
#96481=CARTESIAN_POINT('Ctrl Pts',(-10.9836436743103,15.0782068850301,2.85224741145965));
#96482=CARTESIAN_POINT('Ctrl Pts',(-10.9872445049607,15.0786449381334,2.85774881981766));
#96483=CARTESIAN_POINT('Ctrl Pts',(-10.9935234281681,15.079421754592,2.86751944262066));
#96484=CARTESIAN_POINT('Ctrl Pts',(-10.996220559926,15.0797598060807,2.87177627200917));
#96485=CARTESIAN_POINT('Ctrl Pts',(-11.0017591927968,15.0804632270825,2.88064314977036));
#96486=CARTESIAN_POINT('Ctrl Pts',(-11.0045963776939,15.0808287439061,2.88525574056514));
#96487=CARTESIAN_POINT('Ctrl Pts',(-11.0118490657507,15.0817767690765,2.89723119040767));
#96488=CARTESIAN_POINT('Ctrl Pts',(-11.0162159855994,15.082361013878,2.90462294846806));
#96489=CARTESIAN_POINT('Ctrl Pts',(-11.0349269406528,15.0849245555859,2.9371000929038));
#96490=CARTESIAN_POINT('Ctrl Pts',(-11.0484247057341,15.0869334516445,2.962658896209));
#96491=CARTESIAN_POINT('Ctrl Pts',(-11.103740418389,15.0959250991095,3.07743815501205));
#96492=CARTESIAN_POINT('Ctrl Pts',(-11.1352028175276,15.103236849838,3.17119853312383));
#96493=CARTESIAN_POINT('Ctrl Pts',(-11.1628179518424,15.1134404830624,3.30849067507048));
#96494=CARTESIAN_POINT('Ctrl Pts',(-11.1688508492515,15.1164299244796,3.34963413837847));
#96495=CARTESIAN_POINT('Ctrl Pts',(-11.1732487382952,15.1197327678433,3.39695600462471));
#96496=CARTESIAN_POINT('Ctrl Pts',(-11.1737557553988,15.1201452955867,3.40290161033677));
#96497=CARTESIAN_POINT('Ctrl Pts',(-11.1744957784003,15.1208025605947,3.41243487661072));
#96498=CARTESIAN_POINT('Ctrl Pts',(-11.1747575758616,15.1210487939129,3.41602010278482));
#96499=CARTESIAN_POINT('Ctrl Pts',(-11.1751940944341,15.121485220909,3.42240010629715));
#96500=CARTESIAN_POINT('Ctrl Pts',(-11.1753752685559,15.1216757636012,3.42519437330717));
#96501=CARTESIAN_POINT('Ctrl Pts',(-11.1757437917784,15.1220846921656,3.43121037493215));
#96502=CARTESIAN_POINT('Ctrl Pts',(-11.1759278661915,15.122302896313,3.43443224443988));
#96503=CARTESIAN_POINT('Ctrl Pts',(-11.1764033998383,15.1229083221537,3.44340286621349));
#96504=CARTESIAN_POINT('Ctrl Pts',(-11.1766659664153,15.123293988316,3.44915315602665));
#96505=CARTESIAN_POINT('Ctrl Pts',(-11.1779658474826,15.1255562194959,3.48307758155231));
#96506=CARTESIAN_POINT('Ctrl Pts',(-11.178033495014,15.1273840473419,3.51128226157366));
#96507=CARTESIAN_POINT('Ctrl Pts',(-11.1745892818148,15.1339360561513,3.6140106429075));
#96508=CARTESIAN_POINT('Ctrl Pts',(-11.1650139715779,15.1384716896318,3.68815535785766));
#96509=CARTESIAN_POINT('Ctrl Pts',(-11.1344722447445,15.1470419270055,3.8226006253844));
#96510=CARTESIAN_POINT('Ctrl Pts',(-11.1155087412005,15.1510332579587,3.88306274652448));
#96511=CARTESIAN_POINT('Ctrl Pts',(-11.0880939317458,15.1558358038783,3.95082530759093));
#96512=CARTESIAN_POINT('Ctrl Pts',(-11.0842899718103,15.1564858062412,3.95989902120511));
#96513=CARTESIAN_POINT('Ctrl Pts',(-11.0778777571775,15.1575560401017,3.97467238703678));
#96514=CARTESIAN_POINT('Ctrl Pts',(-11.0753368433064,15.1579740044518,3.98040087978508));
#96515=CARTESIAN_POINT('Ctrl Pts',(-11.070692443946,15.1587273070269,3.99065019408407));
#96516=CARTESIAN_POINT('Ctrl Pts',(-11.0686057227055,15.1590620683366,3.99517848354624));
#96517=CARTESIAN_POINT('Ctrl Pts',(-11.0641005731521,15.1597771117106,4.00479377798365));
#96518=CARTESIAN_POINT('Ctrl Pts',(-11.0616742866537,15.1601576567807,4.00987694125349));
#96519=CARTESIAN_POINT('Ctrl Pts',(-11.055023989345,15.1611887226017,4.02355628111543));
#96520=CARTESIAN_POINT('Ctrl Pts',(-11.0507315026505,15.1618415919515,4.03211849947542));
#96521=CARTESIAN_POINT('Ctrl Pts',(-11.0275147145909,15.1653084914841,4.07705249852453));
#96522=CARTESIAN_POINT('Ctrl Pts',(-11.0068072664957,15.168184351883,4.11246591954439));
#96523=CARTESIAN_POINT('Ctrl Pts',(-10.9276709934895,15.1784874209678,4.23290929970419));
#96524=CARTESIAN_POINT('Ctrl Pts',(-10.8599792347659,15.186208086191,4.31127150756626));
#96525=CARTESIAN_POINT('Ctrl Pts',(-10.7647471084255,15.1953554618111,4.39601958719909));
#96526=CARTESIAN_POINT('Ctrl Pts',(-10.7460373822594,15.1970816742009,4.41165655036606));
#96527=CARTESIAN_POINT('Ctrl Pts',(-10.7223616923607,15.1991674893352,4.43022644975674));
#96528=CARTESIAN_POINT('Ctrl Pts',(-10.7178434352604,15.1995612679325,4.43371755267993));
#96529=CARTESIAN_POINT('Ctrl Pts',(-10.7107129941767,15.200175799264,4.43914464851306));
#96530=CARTESIAN_POINT('Ctrl Pts',(-10.708117952842,15.2003980321963,4.44110286177138));
#96531=CARTESIAN_POINT('Ctrl Pts',(-10.7032968348339,15.2008082306458,4.44470963647622));
#96532=CARTESIAN_POINT('Ctrl Pts',(-10.7010730639282,15.2009963879725,4.44636108035955));
#96533=CARTESIAN_POINT('Ctrl Pts',(-10.695942254151,15.2014281318097,4.45014337442574));
#96534=CARTESIAN_POINT('Ctrl Pts',(-10.6930312440266,15.2016713423006,4.45226873767299));
#96535=CARTESIAN_POINT('Ctrl Pts',(-10.6839565151991,15.2024242821144,4.45883065280589));
#96536=CARTESIAN_POINT('Ctrl Pts',(-10.6777594600841,15.2029309962893,4.46322108426798));
#96537=CARTESIAN_POINT('Ctrl Pts',(-10.6631446141224,15.2041097615554,4.47336438394347));
#96538=CARTESIAN_POINT('Ctrl Pts',(-10.6546936138136,15.2047789670157,4.47906858331985));
#96539=CARTESIAN_POINT('Ctrl Pts',(-10.6244392640184,15.2071350988749,4.49892252431281));
#96540=CARTESIAN_POINT('Ctrl Pts',(-10.6022416172956,15.2087919720935,4.51246028209265));
#96541=CARTESIAN_POINT('Ctrl Pts',(-10.5087269246475,15.2155577450496,4.56532752015965));
#96542=CARTESIAN_POINT('Ctrl Pts',(-10.4338753579854,15.2204889629681,4.59794303460385));
#96543=CARTESIAN_POINT('Ctrl Pts',(-10.3119283092016,15.2285285081471,4.63664355106482));
#96544=CARTESIAN_POINT('Ctrl Pts',(-10.2668119269487,15.2315007092127,4.64807162142226));
#96545=CARTESIAN_POINT('Ctrl Pts',(-10.2111430260604,15.2352290347448,4.65871364571938));
#96546=CARTESIAN_POINT('Ctrl Pts',(-10.2011202217855,15.2359025533648,4.66049529767797));
#96547=CARTESIAN_POINT('Ctrl Pts',(-10.1853290531485,15.2369678107395,4.66309162271102));
#96548=CARTESIAN_POINT('Ctrl Pts',(-10.1795754320136,15.2373567978227,4.66399383285021));
#96549=CARTESIAN_POINT('Ctrl Pts',(-10.1689476949566,15.2380769898298,4.66557966755463));
#96550=CARTESIAN_POINT('Ctrl Pts',(-10.1640755070351,15.238407804204,4.66627548708473));
#96551=CARTESIAN_POINT('Ctrl Pts',(-10.1532636382531,15.2391434198352,4.66775048955194));
#96552=CARTESIAN_POINT('Ctrl Pts',(-10.1473221182794,15.2395486732193,4.66851492922595));
#96553=CARTESIAN_POINT('Ctrl Pts',(-10.1302059099205,15.2407191472101,4.67058449442906));
#96554=CARTESIAN_POINT('Ctrl Pts',(-10.1190182746367,15.2414879163002,4.67177483868667));
#96555=CARTESIAN_POINT('Ctrl Pts',(-10.093755958055,15.2432327347495,4.67409719693852));
#96556=CARTESIAN_POINT('Ctrl Pts',(-10.0796747279584,15.2442115096691,4.67513672206575));
#96557=CARTESIAN_POINT('Ctrl Pts',(-10.0336997147781,15.2474281823065,4.67770065107144));
#96558=CARTESIAN_POINT('Ctrl Pts',(-10.0017642241214,15.2496959021146,4.67818125734417));
#96559=CARTESIAN_POINT('Ctrl Pts',(-9.91751246579765,15.2557605114777,4.67602380162299));
#96560=CARTESIAN_POINT('Ctrl Pts',(-9.86532477286585,15.2596029916686,4.67119514750037));
#96561=CARTESIAN_POINT('Ctrl Pts',(-9.75380805791747,15.2678955066511,4.65332380723034));
#96562=CARTESIAN_POINT('Ctrl Pts',(-9.69480362607636,15.2723346584006,4.63913254637539));
#96563=CARTESIAN_POINT('Ctrl Pts',(-9.62785761028928,15.2772658435852,4.617452673635));
#96564=CARTESIAN_POINT('Ctrl Pts',(-9.6186041099383,15.2779449110793,4.61432832981488));
#96565=CARTESIAN_POINT('Ctrl Pts',(-9.6058981758352,15.2788728206988,4.6098614849761));
#96566=CARTESIAN_POINT('Ctrl Pts',(-9.60241192341497,15.2791269479137,4.60861737580304));
#96567=CARTESIAN_POINT('Ctrl Pts',(-9.59644487348197,15.2795610299417,4.60645619750104));
#96568=CARTESIAN_POINT('Ctrl Pts',(-9.59396122058463,15.2797414443404,4.60554717994859));
#96569=CARTESIAN_POINT('Ctrl Pts',(-9.5887824610702,15.2801170532314,4.60363194677012));
#96570=CARTESIAN_POINT('Ctrl Pts',(-9.58608795269781,15.2803121496529,4.60262421322578));
#96571=CARTESIAN_POINT('Ctrl Pts',(-9.57952138450873,15.2807868497534,4.60014088472318));
#96572=CARTESIAN_POINT('Ctrl Pts',(-9.57565331811511,15.2810658333237,4.59865468969866));
#96573=CARTESIAN_POINT('Ctrl Pts',(-9.56177421135269,15.2820648312136,4.59323780082984));
#96574=CARTESIAN_POINT('Ctrl Pts',(-9.55180891105699,15.2827783082046,4.58919029514864));
#96575=CARTESIAN_POINT('Ctrl Pts',(-9.52706848874539,15.2845434299411,4.57874465719054));
#96576=CARTESIAN_POINT('Ctrl Pts',(-9.51236612842047,15.2855867933907,4.57217886147675));
#96577=CARTESIAN_POINT('Ctrl Pts',(-9.44858127803158,15.2901082329093,4.5421101431506));
#96578=CARTESIAN_POINT('Ctrl Pts',(-9.40102353283894,15.2934681983367,4.51552168333167));
#96579=CARTESIAN_POINT('Ctrl Pts',(-9.28722433921445,15.3018731321247,4.4411136783521));
#96580=CARTESIAN_POINT('Ctrl Pts',(-9.22380397606758,15.3069138439129,4.3895289294965));
#96581=CARTESIAN_POINT('Ctrl Pts',(-9.15560716399373,15.3132116203702,4.32117093782908));
#96582=CARTESIAN_POINT('Ctrl Pts',(-9.14519680747071,15.3142000342822,4.31032859953318));
#96583=CARTESIAN_POINT('Ctrl Pts',(-9.13048577262265,15.3156383903409,4.29440811939364));
#96584=CARTESIAN_POINT('Ctrl Pts',(-9.12601588323514,15.3160811859421,4.2894878164768));
#96585=CARTESIAN_POINT('Ctrl Pts',(-9.11822329559463,15.3168635173597,4.28076271659858));
#96586=CARTESIAN_POINT('Ctrl Pts',(-9.11488294540117,15.3172023082004,4.2769738569345));
#96587=CARTESIAN_POINT('Ctrl Pts',(-9.10803159084474,15.3179044264327,4.26910104956554));
#96588=CARTESIAN_POINT('Ctrl Pts',(-9.10452402639036,15.3182678838146,4.26501427855584));
#96589=CARTESIAN_POINT('Ctrl Pts',(-9.09558624507283,15.3192044935746,4.25445490460956));
#96590=CARTESIAN_POINT('Ctrl Pts',(-9.09019750214581,15.3197793037959,4.2479477599469));
#96591=CARTESIAN_POINT('Ctrl Pts',(-9.06751961445727,15.3222424866097,4.21995548941208));
#96592=CARTESIAN_POINT('Ctrl Pts',(-9.05091920904114,15.3241576581896,4.19792621982383));
#96593=CARTESIAN_POINT('Ctrl Pts',(-8.97806526624932,15.3331096812273,4.09383559929586));
#96594=CARTESIAN_POINT('Ctrl Pts',(-8.93158424697668,15.3404897974257,4.00544353385562));
#96595=CARTESIAN_POINT('Ctrl Pts',(-8.88903661479931,15.3493488933348,3.8915910043721));
#96596=CARTESIAN_POINT('Ctrl Pts',(-8.88188618651963,15.3509488256291,3.87068146944805));
#96597=CARTESIAN_POINT('Ctrl Pts',(-8.86883496738365,15.3540939664585,3.82869323054041));
#96598=CARTESIAN_POINT('Ctrl Pts',(-8.86292474037613,15.3556389861618,3.80762570546016));
#96599=CARTESIAN_POINT('Ctrl Pts',(-8.8562626290168,15.3575368922542,3.78105218930253));
#96600=CARTESIAN_POINT('Ctrl Pts',(-8.85495844701473,15.3579172458359,3.77569068143855));
#96601=CARTESIAN_POINT('Ctrl Pts',(-8.85295589799316,15.3585154082273,3.76719875557004));
#96602=CARTESIAN_POINT('Ctrl Pts',(-8.85223257515441,15.3587345747292,3.76407439484788));
#96603=CARTESIAN_POINT('Ctrl Pts',(-8.85096310927288,15.3591248290546,3.75848723262089));
#96604=CARTESIAN_POINT('Ctrl Pts',(-8.85041211922633,15.3592961842075,3.75602564371142));
#96605=CARTESIAN_POINT('Ctrl Pts',(-8.84910876155452,15.3597063430142,3.75011375363553));
#96606=CARTESIAN_POINT('Ctrl Pts',(-8.84836399836514,15.3599447144712,3.74666181918884));
#96607=CARTESIAN_POINT('Ctrl Pts',(-8.84614391539979,15.3606678565961,3.73614258505591));
#96608=CARTESIAN_POINT('Ctrl Pts',(-8.84471800840283,15.3611499447194,3.72906486154128));
#96609=CARTESIAN_POINT('Ctrl Pts',(-8.83246109930156,15.3654636652005,3.66519770173727));
#96610=CARTESIAN_POINT('Ctrl Pts',(-8.82575868397126,15.3690906547556,3.6076874457981));
#96611=CARTESIAN_POINT('Ctrl Pts',(-8.81899614360149,15.3789955432675,3.44825322757513));
#96612=CARTESIAN_POINT('Ctrl Pts',(-8.82787510282304,15.3851897204474,3.34647792598946));
#96613=CARTESIAN_POINT('Ctrl Pts',(-8.85261521884932,15.3927242297761,3.23394554978417));
#96614=CARTESIAN_POINT('Ctrl Pts',(-8.85573568233757,15.3936124154542,3.22082988437279));
#96615=CARTESIAN_POINT('Ctrl Pts',(-8.86067726530692,15.3949351315317,3.20153696575602));
#96616=CARTESIAN_POINT('Ctrl Pts',(-8.86232508386034,15.395364138175,3.19531613266589));
#96617=CARTESIAN_POINT('Ctrl Pts',(-8.86534475325112,15.3961296649969,3.18428244223013));
#96618=CARTESIAN_POINT('Ctrl Pts',(-8.86669646427889,15.3964655309349,3.17946419879257));
#96619=CARTESIAN_POINT('Ctrl Pts',(-8.86960757792984,15.3971749230406,3.16933603037875));
#96620=CARTESIAN_POINT('Ctrl Pts',(-8.87117377844989,15.3975486616852,3.16402820295518));
#96621=CARTESIAN_POINT('Ctrl Pts',(-8.87542227618869,15.398542095509,3.14999524735485));
#96622=CARTESIAN_POINT('Ctrl Pts',(-8.87816865637252,15.3991638528738,3.14129007255412));
#96623=CARTESIAN_POINT('Ctrl Pts',(-8.89189402573273,15.4021769843532,3.09948490361637));
#96624=CARTESIAN_POINT('Ctrl Pts',(-8.90423729056878,15.404612388616,3.06685471310826));
#96625=CARTESIAN_POINT('Ctrl Pts',(-8.94466030829147,15.411883809643,2.97283170958428));
#96626=CARTESIAN_POINT('Ctrl Pts',(-8.97658751685163,15.4168293435335,2.91325195648752));
#96627=CARTESIAN_POINT('Ctrl Pts',(-9.04646018834736,15.4262224733724,2.80608851643903));
#96628=CARTESIAN_POINT('Ctrl Pts',(-9.08334109605991,15.4306522382477,2.75805035471875));
#96629=CARTESIAN_POINT('Ctrl Pts',(-9.13028117129571,15.4355752078499,2.70578359192119));
#96630=CARTESIAN_POINT('Ctrl Pts',(-9.13690073450279,15.4362546647628,2.69859484819586));
#96631=CARTESIAN_POINT('Ctrl Pts',(-9.14615078526604,15.4371830060588,2.68879701225992));
#96632=CARTESIAN_POINT('Ctrl Pts',(-9.14870502622069,15.4374371820127,2.6861169387618));
#96633=CARTESIAN_POINT('Ctrl Pts',(-9.15310566781629,15.4378713255455,2.68154288553122));
#96634=CARTESIAN_POINT('Ctrl Pts',(-9.15494586878972,15.43805175299,2.67964302051611));
#96635=CARTESIAN_POINT('Ctrl Pts',(-9.15880078804323,15.4384273644047,2.67568985015263));
#96636=CARTESIAN_POINT('Ctrl Pts',(-9.16081664823704,15.4386224504282,2.67363770675323));
#96637=CARTESIAN_POINT('Ctrl Pts',(-9.16575400781213,15.4390970849753,2.66864817916817));
#96638=CARTESIAN_POINT('Ctrl Pts',(-9.16868356350469,15.4393760137984,2.66571874694888));
#96639=CARTESIAN_POINT('Ctrl Pts',(-9.1792697581953,15.4403745943019,2.65524412764747));
#96640=CARTESIAN_POINT('Ctrl Pts',(-9.18701443329813,15.4410877158351,2.64778811188352));
#96641=CARTESIAN_POINT('Ctrl Pts',(-9.20660223167084,15.4428517799165,2.62944048014546));
#96642=CARTESIAN_POINT('Ctrl Pts',(-9.21856876661526,15.4438944539055,2.61868327047147));
#96643=CARTESIAN_POINT('Ctrl Pts',(-9.27190674756109,15.4484109718669,2.57267641565309));
#96644=CARTESIAN_POINT('Ctrl Pts',(-9.31547205575955,15.4517669665735,2.54006706179593));
#96645=CARTESIAN_POINT('Ctrl Pts',(-9.42971561267296,15.4601733496869,2.46630052507641));
#96646=CARTESIAN_POINT('Ctrl Pts',(-9.50270305363433,15.465219316615,2.42927477025493));
#96647=CARTESIAN_POINT('Ctrl Pts',(-9.59296155463226,15.4715228324607,2.39472149187044));
#96648=CARTESIAN_POINT('Ctrl Pts',(-9.60709642812175,15.4725110440725,2.3896182519908));
#96649=CARTESIAN_POINT('Ctrl Pts',(-9.62761857204557,15.473949158499,2.38264986839871));
#96650=CARTESIAN_POINT('Ctrl Pts',(-9.63393044806697,15.4743919181734,2.38056606958004));
#96651=CARTESIAN_POINT('Ctrl Pts',(-9.64506912951378,15.4751742076756,2.37699303104505));
#96652=CARTESIAN_POINT('Ctrl Pts',(-9.64988855125129,15.4755129927793,2.37548119302536));
#96653=CARTESIAN_POINT('Ctrl Pts',(-9.65986666577574,15.4762151201987,2.37242145077976));
#96654=CARTESIAN_POINT('Ctrl Pts',(-9.66502654106717,15.4765785926329,2.37087784103969));
#96655=CARTESIAN_POINT('Ctrl Pts',(-9.67830840056628,15.4775152859443,2.36700354151355));
#96656=CARTESIAN_POINT('Ctrl Pts',(-9.6864450910596,15.4780901652352,2.36472480310431));
#96657=CARTESIAN_POINT('Ctrl Pts',(-9.7212486712089,15.4805540667524,2.35538050302663));
#96658=CARTESIAN_POINT('Ctrl Pts',(-9.74813292105391,15.4824699074825,2.34916601961695));
#96659=CARTESIAN_POINT('Ctrl Pts',(-9.78714530463055,15.4852701831299,2.34158046861053));
#96660=CARTESIAN_POINT('Ctrl Pts',(-9.7991118959388,15.486131784317,2.33944554572489));
#96661=CARTESIAN_POINT('Ctrl Pts',(-9.81110406371067,15.4869977587645,2.3374969300026));
#96662=CARTESIAN_POINT('Origin',(-10.,12.3756328852638,3.5));
#96663=CARTESIAN_POINT('',(-9.81110382412687,16.0869811837922,2.33749696893276));
#96664=CARTESIAN_POINT('',(-9.81110406371106,15.9888353687451,2.33749693000254));
#96665=CARTESIAN_POINT('',(-9.81110406371068,12.3756328852638,2.3374969300026));
#96666=CARTESIAN_POINT('Ctrl Pts',(-9.81110382412688,16.0869811837922,2.33749696893276));
#96667=CARTESIAN_POINT('Ctrl Pts',(-9.71998275066426,16.0802638280491,2.35230331511729));
#96668=CARTESIAN_POINT('Ctrl Pts',(-9.63092842143902,16.0733690794726,2.3777681961223));
#96669=CARTESIAN_POINT('Ctrl Pts',(-9.53775860307175,16.0662516653844,2.41671656411454));
#96670=CARTESIAN_POINT('Ctrl Pts',(-9.52980263881095,16.0656449645949,2.42014604543945));
#96671=CARTESIAN_POINT('Ctrl Pts',(-9.51753861172157,16.0647121799927,2.42559379667557));
#96672=CARTESIAN_POINT('Ctrl Pts',(-9.51320389041452,16.0643829640415,2.42755082615761));
#96673=CARTESIAN_POINT('Ctrl Pts',(-9.50509866660381,16.0637684387193,2.43126942099416));
#96674=CARTESIAN_POINT('Ctrl Pts',(-9.50132542978528,16.0634827898069,2.43302481066971));
#96675=CARTESIAN_POINT('Ctrl Pts',(-9.49495592194608,16.0630014228457,2.43602921033503));
#96676=CARTESIAN_POINT('Ctrl Pts',(-9.49235480816932,16.0628050831729,2.43726780329201));
#96677=CARTESIAN_POINT('Ctrl Pts',(-9.4873769775607,16.0624298297448,2.43966058273671));
#96678=CARTESIAN_POINT('Ctrl Pts',(-9.48499957417099,16.0622508207162,2.44081323427598));
#96679=CARTESIAN_POINT('Ctrl Pts',(-9.47931185066821,16.061823017062,2.44359452672951));
#96680=CARTESIAN_POINT('Ctrl Pts',(-9.47600523892815,16.0615746836938,2.44523075315276));
#96681=CARTESIAN_POINT('Ctrl Pts',(-9.46406477850062,16.0606790909595,2.45120931630991));
#96682=CARTESIAN_POINT('Ctrl Pts',(-9.4554764814352,16.0600371317322,2.45564248821605));
#96683=CARTESIAN_POINT('Ctrl Pts',(-9.38655498868761,16.0548953857802,2.49230029977449));
#96684=CARTESIAN_POINT('Ctrl Pts',(-9.32907057330553,16.0506647259872,2.52962389580546));
#96685=CARTESIAN_POINT('Ctrl Pts',(-9.2373201360961,16.0434671706792,2.60126885869721));
#96686=CARTESIAN_POINT('Ctrl Pts',(-9.2013364172409,16.040507731606,2.6330891264525));
#96687=CARTESIAN_POINT('Ctrl Pts',(-9.14624599267034,16.0356053192525,2.68815435488495));
#96688=CARTESIAN_POINT('Ctrl Pts',(-9.12591059438921,16.0337019704557,2.71009065824297));
#96689=CARTESIAN_POINT('Ctrl Pts',(-9.09347048028087,16.0304785568442,2.74787285724886));
#96690=CARTESIAN_POINT('Ctrl Pts',(-9.08089336842273,16.0291769838373,2.76329521961175));
#96691=CARTESIAN_POINT('Ctrl Pts',(-9.06430026014541,16.0273826882613,2.78472869942786));
#96692=CARTESIAN_POINT('Ctrl Pts',(-9.05993952838316,16.0269034756245,2.79046963248325));
#96693=CARTESIAN_POINT('Ctrl Pts',(-9.05284819493209,16.0261112245714,2.79998555528696));
#96694=CARTESIAN_POINT('Ctrl Pts',(-9.0500867545275,16.0257993846198,2.80373741328203));
#96695=CARTESIAN_POINT('Ctrl Pts',(-9.04438036225703,16.0251479316422,2.81158759536892));
#96696=CARTESIAN_POINT('Ctrl Pts',(-9.04143935380294,16.0248081765118,2.81568865486148));
#96697=CARTESIAN_POINT('Ctrl Pts',(-9.03470628789245,16.0240209447511,2.8252060849612));
#96698=CARTESIAN_POINT('Ctrl Pts',(-9.03093333321431,16.0235727572941,2.83063569662474));
#96699=CARTESIAN_POINT('Ctrl Pts',(-9.01885230257836,16.0221143246272,2.84833759634299));
#96700=CARTESIAN_POINT('Ctrl Pts',(-9.01073038195427,16.0210972056754,2.86073457747773));
#96701=CARTESIAN_POINT('Ctrl Pts',(-8.95549232020234,16.0139125633871,2.94862232384264));
#96702=CARTESIAN_POINT('Ctrl Pts',(-8.91683969518205,16.0074363066258,3.02907373728262));
#96703=CARTESIAN_POINT('Ctrl Pts',(-8.87155694883815,15.9973144032274,3.15926365353578));
#96704=CARTESIAN_POINT('Ctrl Pts',(-8.85838639747998,15.9937244479054,3.20639496989813));
#96705=CARTESIAN_POINT('Ctrl Pts',(-8.84501920029073,15.9891402766251,3.26903632565814));
#96706=CARTESIAN_POINT('Ctrl Pts',(-8.84214191792509,15.9880646452468,3.28392229407242));
#96707=CARTESIAN_POINT('Ctrl Pts',(-8.83782696231029,15.9862929198105,3.30881683654593));
#96708=CARTESIAN_POINT('Ctrl Pts',(-8.8362293526486,15.9855899503777,3.31879550490512));
#96709=CARTESIAN_POINT('Ctrl Pts',(-8.83415730792606,15.9846077453011,3.33289797487026));
#96710=CARTESIAN_POINT('Ctrl Pts',(-8.83357598155575,15.9843230255583,3.33700527623731));
#96711=CARTESIAN_POINT('Ctrl Pts',(-8.8326280595956,15.983842764384,3.34396763193602));
#96712=CARTESIAN_POINT('Ctrl Pts',(-8.8322502111005,15.9836466078098,3.34682109045668));
#96713=CARTESIAN_POINT('Ctrl Pts',(-8.83154521964688,15.9832713413337,3.35229934047037));
#96714=CARTESIAN_POINT('Ctrl Pts',(-8.83121645414841,15.98309213829,3.35492387565429));
#96715=CARTESIAN_POINT('Ctrl Pts',(-8.83044896384256,15.9826633968753,3.36122273571014));
#96716=CARTESIAN_POINT('Ctrl Pts',(-8.83001870488549,15.9824143243031,3.3648980930338));
#96717=CARTESIAN_POINT('Ctrl Pts',(-8.82851771953156,15.9815122518474,3.37826503997729));
#96718=CARTESIAN_POINT('Ctrl Pts',(-8.82754999725294,15.9808646559533,3.3879681284794));
#96719=CARTESIAN_POINT('Ctrl Pts',(-8.82138590023867,15.9761922004064,3.45865317726463));
#96720=CARTESIAN_POINT('Ctrl Pts',(-8.82082885873209,15.9723814409384,3.51995407413669));
#96721=CARTESIAN_POINT('Ctrl Pts',(-8.82964564142442,15.9644475499155,3.64780426985037));
#96722=CARTESIAN_POINT('Ctrl Pts',(-8.83993457777486,15.9603393754895,3.71406312086657));
#96723=CARTESIAN_POINT('Ctrl Pts',(-8.86402268495667,15.9538771608337,3.81281967166299));
#96724=CARTESIAN_POINT('Ctrl Pts',(-8.87373731125307,15.9516353703548,3.84616845761532));
#96725=CARTESIAN_POINT('Ctrl Pts',(-8.88784427563159,15.9487446499486,3.88766975427016));
#96726=CARTESIAN_POINT('Ctrl Pts',(-8.89087869084375,15.9481402248224,3.89626772195071));
#96727=CARTESIAN_POINT('Ctrl Pts',(-8.89591442867788,15.9471637381456,3.91002527726144));
#96728=CARTESIAN_POINT('Ctrl Pts',(-8.89785286294132,15.9467937538902,3.9152076146846));
#96729=CARTESIAN_POINT('Ctrl Pts',(-8.90161476020985,15.9460866635381,3.92505293139028));
#96730=CARTESIAN_POINT('Ctrl Pts',(-8.90343158672009,15.9457497842992,3.92971832999723));
#96731=CARTESIAN_POINT('Ctrl Pts',(-8.90765445430549,15.9449770773057,3.94036097347338));
#96732=CARTESIAN_POINT('Ctrl Pts',(-8.91007989267944,15.9445406094011,3.94633029804));
#96733=CARTESIAN_POINT('Ctrl Pts',(-8.91774450894765,15.9431834343641,3.96475885494576));
#96734=CARTESIAN_POINT('Ctrl Pts',(-8.92314910985567,15.9422572086239,3.97714764493938));
#96735=CARTESIAN_POINT('Ctrl Pts',(-8.97094580219988,15.9343142031851,4.08175993414274));
#96736=CARTESIAN_POINT('Ctrl Pts',(-9.02487578376481,15.9268798897526,4.16822256572122));
#96737=CARTESIAN_POINT('Ctrl Pts',(-9.12597641048341,15.9151813967729,4.29154465538999));
#96738=CARTESIAN_POINT('Ctrl Pts',(-9.16602278442699,15.9109515826147,4.33363288211195));
#96739=CARTESIAN_POINT('Ctrl Pts',(-9.21436700924182,15.9064093279908,4.37745546452834));
#96740=CARTESIAN_POINT('Ctrl Pts',(-9.21976607901131,15.9059093567241,4.38225978232027));
#96741=CARTESIAN_POINT('Ctrl Pts',(-9.2278703712304,15.9051701055201,4.3893387340985));
#96742=CARTESIAN_POINT('Ctrl Pts',(-9.23054203712947,15.9049281922815,4.39165127252324));
#96743=CARTESIAN_POINT('Ctrl Pts',(-9.23513951749828,15.9045150158027,4.39559470339104));
#96744=CARTESIAN_POINT('Ctrl Pts',(-9.23706020547129,15.904343328837,4.39723146445229));
#96745=CARTESIAN_POINT('Ctrl Pts',(-9.24143416611643,15.9039544539304,4.40093464035289));
#96746=CARTESIAN_POINT('Ctrl Pts',(-9.2438906285,15.903737544337,4.40299721454425));
#96747=CARTESIAN_POINT('Ctrl Pts',(-9.25059525372561,15.9031494476794,4.40858022666024));
#96748=CARTESIAN_POINT('Ctrl Pts',(-9.25485984274685,15.9027796417248,4.41208094543831));
#96749=CARTESIAN_POINT('Ctrl Pts',(-9.27613889256795,15.9009545404701,4.4292996417067));
#96750=CARTESIAN_POINT('Ctrl Pts',(-9.29350953197979,15.8995279219435,4.44257312359106));
#96751=CARTESIAN_POINT('Ctrl Pts',(-9.3291498482908,15.8967026534067,4.46826782092348));
#96752=CARTESIAN_POINT('Ctrl Pts',(-9.34741928345548,15.8953049985431,4.48067375052159));
#96753=CARTESIAN_POINT('Ctrl Pts',(-9.44988778413838,15.8876776012046,4.54612294421872));
#96754=CARTESIAN_POINT('Ctrl Pts',(-9.54019460628715,15.8816846086777,4.58884165819584));
#96755=CARTESIAN_POINT('Ctrl Pts',(-9.6610116058061,15.8735400296484,4.62824736939657));
#96756=CARTESIAN_POINT('Ctrl Pts',(-9.68751452588286,15.8717490354282,4.63587318634894));
#96757=CARTESIAN_POINT('Ctrl Pts',(-9.72245647253351,15.8693700689526,4.64461174801248));
#96758=CARTESIAN_POINT('Ctrl Pts',(-9.73067555305444,15.8688092512808,4.64657350371413));
#96759=CARTESIAN_POINT('Ctrl Pts',(-9.74416791600781,15.8678862791553,4.6496408256885));
#96760=CARTESIAN_POINT('Ctrl Pts',(-9.74942903135062,15.8675258034306,4.65079897085346));
#96761=CARTESIAN_POINT('Ctrl Pts',(-9.75964001936648,15.8668249723267,4.6529734060432));
#96762=CARTESIAN_POINT('Ctrl Pts',(-9.76458885943727,15.8664847624602,4.65399401595487));
#96763=CARTESIAN_POINT('Ctrl Pts',(-9.77606627986435,15.8656944051191,4.65628412797902));
#96764=CARTESIAN_POINT('Ctrl Pts',(-9.78259929879314,15.8652435290264,4.65753022750587));
#96765=CARTESIAN_POINT('Ctrl Pts',(-9.80394076442455,15.8637671911042,4.66141382886268));
#96766=CARTESIAN_POINT('Ctrl Pts',(-9.8187887235298,15.8627346180929,4.66382289999578));
#96767=CARTESIAN_POINT('Ctrl Pts',(-9.91405450019217,15.8560718427049,4.67741252316573));
#96768=CARTESIAN_POINT('Ctrl Pts',(-9.99538651645026,15.8501898026005,4.68053422357338));
#96769=CARTESIAN_POINT('Ctrl Pts',(-10.1309447336209,15.8402205057052,4.6717246587711));
#96770=CARTESIAN_POINT('Ctrl Pts',(-10.1852010487014,15.8361917886511,4.66438238714015));
#96771=CARTESIAN_POINT('Ctrl Pts',(-10.2545610959831,15.8311131453877,4.65002361639674));
#96772=CARTESIAN_POINT('Ctrl Pts',(-10.2703011483669,15.8299658153285,4.64642619217887));
#96773=CARTESIAN_POINT('Ctrl Pts',(-10.2964180611546,15.8280759243388,4.63988927114941));
#96774=CARTESIAN_POINT('Ctrl Pts',(-10.306837128272,15.8273256929406,4.63712893503009));
#96775=CARTESIAN_POINT('Ctrl Pts',(-10.3212119147047,15.8262971469425,4.6331086327221));
#96776=CARTESIAN_POINT('Ctrl Pts',(-10.3252006886351,15.8260124420374,4.63197030929356));
#96777=CARTESIAN_POINT('Ctrl Pts',(-10.3319469896852,15.8255321985119,4.63000643490599));
#96778=CARTESIAN_POINT('Ctrl Pts',(-10.3347076322705,15.8253360448523,4.6291918120791));
#96779=CARTESIAN_POINT('Ctrl Pts',(-10.3399994678797,15.8249607781266,4.62760916130065));
#96780=CARTESIAN_POINT('Ctrl Pts',(-10.3425310860537,15.8247815719529,4.62684271939236));
#96781=CARTESIAN_POINT('Ctrl Pts',(-10.3485982968419,15.8243528154349,4.62498354833706));
#96782=CARTESIAN_POINT('Ctrl Pts',(-10.3521313912093,15.8241037309626,4.62388266328753));
#96783=CARTESIAN_POINT('Ctrl Pts',(-10.3649558881408,15.8232015526282,4.61982023610184));
#96784=CARTESIAN_POINT('Ctrl Pts',(-10.3742159179805,15.822553864465,4.61675987725334));
#96785=CARTESIAN_POINT('Ctrl Pts',(-10.4422222015541,15.8178174470215,4.59334348108205));
#96786=CARTESIAN_POINT('Ctrl Pts',(-10.4993203726699,15.8139498119805,4.56847633383445));
#96787=CARTESIAN_POINT('Ctrl Pts',(-10.612612972518,15.8060028955478,4.50805939417687));
#96788=CARTESIAN_POINT('Ctrl Pts',(-10.6682975163286,15.8019370827577,4.47203713412819));
#96789=CARTESIAN_POINT('Ctrl Pts',(-10.7479553126756,15.7955331295536,4.41041140204768));
#96790=CARTESIAN_POINT('Ctrl Pts',(-10.7743077107265,15.7933045105246,4.38810657223371));
#96791=CARTESIAN_POINT('Ctrl Pts',(-10.8063224276096,15.7904286617853,4.35849986703975));
#96792=CARTESIAN_POINT('Ctrl Pts',(-10.8129317135178,15.7898253639941,4.35224403807633));
#96793=CARTESIAN_POINT('Ctrl Pts',(-10.8234390306121,15.7888502623246,4.34206519805909));
#96794=CARTESIAN_POINT('Ctrl Pts',(-10.8273831711333,15.7884805250204,4.33819014624981));
#96795=CARTESIAN_POINT('Ctrl Pts',(-10.8348470614639,15.787773618958,4.3307529851347));
#96796=CARTESIAN_POINT('Ctrl Pts',(-10.8383716738139,15.787436675053,4.32719591002215));
#96797=CARTESIAN_POINT('Ctrl Pts',(-10.8463843401985,15.7866634108876,4.31900562852991));
#96798=CARTESIAN_POINT('Ctrl Pts',(-10.8508571959665,15.78622644718,4.31435784523298));
#96799=CARTESIAN_POINT('Ctrl Pts',(-10.8646094431631,15.7848661739024,4.2998307807205));
#96800=CARTESIAN_POINT('Ctrl Pts',(-10.8737563565465,15.7839373093408,4.28982818997498));
#96801=CARTESIAN_POINT('Ctrl Pts',(-10.9497232832532,15.7760117740848,4.20381984382201));
#96802=CARTESIAN_POINT('Ctrl Pts',(-11.0066499632571,15.7686004130611,4.11966449275862));
#96803=CARTESIAN_POINT('Ctrl Pts',(-11.0782853583566,15.7569064498529,3.97727084799873));
#96804=CARTESIAN_POINT('Ctrl Pts',(-11.1005667522556,15.7526592161766,3.92336888561802));
#96805=CARTESIAN_POINT('Ctrl Pts',(-11.1210302576074,15.7481004956167,3.86116276698205));
#96806=CARTESIAN_POINT('Ctrl Pts',(-11.1232272998644,15.7476000664878,3.85427083163141));
#96807=CARTESIAN_POINT('Ctrl Pts',(-11.1264032819796,15.7468602732757,3.84398139925853));
#96808=CARTESIAN_POINT('Ctrl Pts',(-11.1274305969391,15.7466182703996,3.84059918761211));
#96809=CARTESIAN_POINT('Ctrl Pts',(-11.1291652475585,15.7462049940557,3.83479437701117));
#96810=CARTESIAN_POINT('Ctrl Pts',(-11.1298800391705,15.7460332962705,3.83237407946572));
#96811=CARTESIAN_POINT('Ctrl Pts',(-11.1314854149415,15.7456444688356,3.82687321807539));
#96812=CARTESIAN_POINT('Ctrl Pts',(-11.1323712012782,15.7454276170846,3.82379130324512));
#96813=CARTESIAN_POINT('Ctrl Pts',(-11.1347457233965,15.7448398315151,3.81540070284795));
#96814=CARTESIAN_POINT('Ctrl Pts',(-11.1362098102458,15.7444702763736,3.81008503702247));
#96815=CARTESIAN_POINT('Ctrl Pts',(-11.1432802550694,15.7426484233139,3.78369174819178));
#96816=CARTESIAN_POINT('Ctrl Pts',(-11.1483381055273,15.7412246803085,3.76246998298149));
#96817=CARTESIAN_POINT('Ctrl Pts',(-11.1573256594095,15.7384015791782,3.71949985782572));
#96818=CARTESIAN_POINT('Ctrl Pts',(-11.161238572333,15.7370033199704,3.69775728898744));
#96819=CARTESIAN_POINT('Ctrl Pts',(-11.1793904245861,15.7293794955202,3.57759506762583));
#96820=CARTESIAN_POINT('Ctrl Pts',(-11.181731813801,15.7233907062356,3.477792172738));
#96821=CARTESIAN_POINT('Ctrl Pts',(-11.1686603807797,15.7152455481874,3.35136177602668));
#96822=CARTESIAN_POINT('Ctrl Pts',(-11.1648468264498,15.7134486450765,3.32395430885453));
#96823=CARTESIAN_POINT('Ctrl Pts',(-11.1586119391436,15.7110629261981,3.28837532079456));
#96824=CARTESIAN_POINT('Ctrl Pts',(-11.1570619866676,15.7105014630184,3.28005868242311));
#96825=CARTESIAN_POINT('Ctrl Pts',(-11.1543782070616,15.7095777001602,3.26647256807064));
#96826=CARTESIAN_POINT('Ctrl Pts',(-11.1532975450868,15.7092170848723,3.26119280317626));
#96827=CARTESIAN_POINT('Ctrl Pts',(-11.1511336908559,15.7085161766414,3.25097828996551));
#96828=CARTESIAN_POINT('Ctrl Pts',(-11.1500549053129,15.7081760304809,3.24604272074544));
#96829=CARTESIAN_POINT('Ctrl Pts',(-11.1474836648804,15.7073861076131,3.2346314591371));
#96830=CARTESIAN_POINT('Ctrl Pts',(-11.1459681017378,15.7069356047607,3.22816120530877));
#96831=CARTESIAN_POINT('Ctrl Pts',(-11.140850990343,15.7054617614826,3.2071188026942));
#96832=CARTESIAN_POINT('Ctrl Pts',(-11.1370257272322,15.7044313432077,3.19260312740125));
#96833=CARTESIAN_POINT('Ctrl Pts',(-11.1104395647892,15.6976954120639,3.09901443710512));
#96834=CARTESIAN_POINT('Ctrl Pts',(-11.0797263081074,15.6917304883363,3.02245226779789));
#96835=CARTESIAN_POINT('Ctrl Pts',(-11.0278376228702,15.6835790157976,2.92426173141924));
#96836=CARTESIAN_POINT('Ctrl Pts',(-11.0134498946367,15.6814612223146,2.8992970143392));
#96837=CARTESIAN_POINT('Ctrl Pts',(-10.9730336524859,15.6758969763483,2.83476183624392));
#96838=CARTESIAN_POINT('Ctrl Pts',(-10.9455064599881,15.6724763196917,2.79618545131465));
#96839=CARTESIAN_POINT('Ctrl Pts',(-10.9116681131499,15.6687385378231,2.75434726659731));
#96840=CARTESIAN_POINT('Ctrl Pts',(-10.9075666651507,15.6682925856455,2.74936060561022));
#96841=CARTESIAN_POINT('Ctrl Pts',(-10.9012577450849,15.667617633815,2.7418173414062));
#96842=CARTESIAN_POINT('Ctrl Pts',(-10.8990800227074,15.6673866127442,2.73923618621772));
#96843=CARTESIAN_POINT('Ctrl Pts',(-10.895084310839,15.6669663482554,2.73454137209523));
#96844=CARTESIAN_POINT('Ctrl Pts',(-10.893269914678,15.6667768604249,2.73242479557206));
#96845=CARTESIAN_POINT('Ctrl Pts',(-10.8891856043175,15.6663533114187,2.72769435614263));
#96846=CARTESIAN_POINT('Ctrl Pts',(-10.8869116735679,15.6661195483231,2.72508404938227));
#96847=CARTESIAN_POINT('Ctrl Pts',(-10.8802323944914,15.6654387299402,2.7174846383343));
#96848=CARTESIAN_POINT('Ctrl Pts',(-10.8757961355965,15.6649938663248,2.71252270285092));
#96849=CARTESIAN_POINT('Ctrl Pts',(-10.8373922456707,15.6612022320795,2.6702941133651));
#96850=CARTESIAN_POINT('Ctrl Pts',(-10.8011010943487,15.6580124676607,2.63520174157808));
#96851=CARTESIAN_POINT('Ctrl Pts',(-10.745704017538,15.6534803693136,2.58812493431397));
#96852=CARTESIAN_POINT('Ctrl Pts',(-10.7283352447967,15.6521025758694,2.57419309748382));
#96853=CARTESIAN_POINT('Ctrl Pts',(-10.6424293103732,15.6454419608596,2.50920086500072));
#96854=CARTESIAN_POINT('Ctrl Pts',(-10.5688764255294,15.6401749527133,2.46521704315764));
#96855=CARTESIAN_POINT('Ctrl Pts',(-10.4790261717907,15.6337256763909,2.42398471392351));
#96856=CARTESIAN_POINT('Ctrl Pts',(-10.4667413170832,15.6328441892421,2.41859929334936));
#96857=CARTESIAN_POINT('Ctrl Pts',(-10.4476449681182,15.6314729880157,2.4106138697164));
#96858=CARTESIAN_POINT('Ctrl Pts',(-10.4408965612099,15.6309882437529,2.4078652204735));
#96859=CARTESIAN_POINT('Ctrl Pts',(-10.4293880254143,15.6301610652618,2.40330180380957));
#96860=CARTESIAN_POINT('Ctrl Pts',(-10.4246407761381,15.6298197099727,2.40145495324764));
#96861=CARTESIAN_POINT('Ctrl Pts',(-10.4150047303251,15.6291264535887,2.39777797833501));
#96862=CARTESIAN_POINT('Ctrl Pts',(-10.4101154527308,15.6287745087678,2.39594944628848));
#96863=CARTESIAN_POINT('Ctrl Pts',(-10.3980193011543,15.6279032386187,2.39151706532146));
#96864=CARTESIAN_POINT('Ctrl Pts',(-10.3907989475913,15.6273826831983,2.38895096494578));
#96865=CARTESIAN_POINT('Ctrl Pts',(-10.3636492034279,15.625423169241,2.37959938599999));
#96866=CARTESIAN_POINT('Ctrl Pts',(-10.3435651343849,15.6239692299577,2.37327857111096));
#96867=CARTESIAN_POINT('Ctrl Pts',(-10.2924785715365,15.6202574989402,2.3586935961774));
#96868=CARTESIAN_POINT('Ctrl Pts',(-10.2612892618296,15.617978820873,2.35115204083168));
#96869=CARTESIAN_POINT('Ctrl Pts',(-10.1786411376612,15.6119138761872,2.33470742023526));
#96870=CARTESIAN_POINT('Ctrl Pts',(-10.1268315242213,15.6080829426248,2.32793663037627));
#96871=CARTESIAN_POINT('Ctrl Pts',(-10.014371927807,15.5998090410717,2.3207848103437));
#96872=CARTESIAN_POINT('Ctrl Pts',(-9.95378383888036,15.595376948158,2.32160253464665));
#96873=CARTESIAN_POINT('Ctrl Pts',(-9.8837907050311,15.5904518679028,2.32795651354185));
#96874=CARTESIAN_POINT('Ctrl Pts',(-9.87407071524542,15.5897724439979,2.32896098903557));
#96875=CARTESIAN_POINT('Ctrl Pts',(-9.86068562549131,15.5888440813364,2.3305128134094));
#96876=CARTESIAN_POINT('Ctrl Pts',(-9.85700925496088,15.5885898520667,2.33095662086036));
#96877=CARTESIAN_POINT('Ctrl Pts',(-9.85070987419604,15.588155602528,2.33174723601867));
#96878=CARTESIAN_POINT('Ctrl Pts',(-9.8480858559742,15.5879751222836,2.33208555304258));
#96879=CARTESIAN_POINT('Ctrl Pts',(-9.84261010286847,15.5875993808907,2.33281031353234));
#96880=CARTESIAN_POINT('Ctrl Pts',(-9.83975861644863,15.5874042178622,2.33319837026518));
#96881=CARTESIAN_POINT('Ctrl Pts',(-9.83280344615905,15.5869293575943,2.33417087174944));
#96882=CARTESIAN_POINT('Ctrl Pts',(-9.82870131775477,15.5866502808701,2.33476654414031));
#96883=CARTESIAN_POINT('Ctrl Pts',(-9.82009890055875,15.5860669644847,2.33606211595207));
#96884=CARTESIAN_POINT('Ctrl Pts',(-9.81559939849938,15.5857629682338,2.3367664799111));
#96885=CARTESIAN_POINT('Ctrl Pts',(-9.8111040637049,15.5854602598056,2.33749693000354));
#96886=CARTESIAN_POINT('',(-11.1777498238975,15.6247875272409,3.49935594293548));
#96887=CARTESIAN_POINT('Ctrl Pts',(-9.81110406371067,15.4869977587645,2.3374969300026));
#96888=CARTESIAN_POINT('Ctrl Pts',(-9.89721051432613,15.4932156492593,2.32350543266437));
#96889=CARTESIAN_POINT('Ctrl Pts',(-9.98463361579959,15.4996878786372,2.31911987310096));
#96890=CARTESIAN_POINT('Ctrl Pts',(-10.0938106552571,15.5076604291426,2.32578419522931));
#96891=CARTESIAN_POINT('Ctrl Pts',(-10.115822188047,15.509260416155,2.32775066230818));
#96892=CARTESIAN_POINT('Ctrl Pts',(-10.1594864733125,15.5124052718222,2.33289356272436));
#96893=CARTESIAN_POINT('Ctrl Pts',(-10.1811328843666,15.5139499614132,2.33605653096591));
#96894=CARTESIAN_POINT('Ctrl Pts',(-10.2081151940926,15.5158475222848,2.34077026924418));
#96895=CARTESIAN_POINT('Ctrl Pts',(-10.2135435402494,15.5162278491646,2.3417579432186));
#96896=CARTESIAN_POINT('Ctrl Pts',(-10.2221158132083,15.5168259789667,2.34337996218021));
#96897=CARTESIAN_POINT('Ctrl Pts',(-10.2252643487936,15.5170451393421,2.34398904842987));
#96898=CARTESIAN_POINT('Ctrl Pts',(-10.2308850601435,15.5174353884894,2.34510021440993));
#96899=CARTESIAN_POINT('Ctrl Pts',(-10.2333580980304,15.5176067445459,2.34559737352311));
#96900=CARTESIAN_POINT('Ctrl Pts',(-10.2392894895475,15.5180169128745,2.34680961086563));
#96901=CARTESIAN_POINT('Ctrl Pts',(-10.2427462442213,15.5182552928914,2.34753230191249));
#96902=CARTESIAN_POINT('Ctrl Pts',(-10.2532604401807,15.5189784871239,2.34977987179638));
#96903=CARTESIAN_POINT('Ctrl Pts',(-10.2603073179555,15.5194606182302,2.35135414484638));
#96904=CARTESIAN_POINT('Ctrl Pts',(-10.3236652186813,15.5237758844522,2.36612133576886));
#96905=CARTESIAN_POINT('Ctrl Pts',(-10.3789558064251,15.5274042164427,2.38338261408851));
#96906=CARTESIAN_POINT('Ctrl Pts',(-10.527363584146,15.5373085702841,2.44201633451099));
#96907=CARTESIAN_POINT('Ctrl Pts',(-10.6167152720149,15.5435010747445,2.49148523909094));
#96908=CARTESIAN_POINT('Ctrl Pts',(-10.7094557296208,15.5510338374472,2.55981412659028));
#96909=CARTESIAN_POINT('Ctrl Pts',(-10.7201737257285,15.5519222690396,2.56799855727563));
#96910=CARTESIAN_POINT('Ctrl Pts',(-10.7357959124247,15.5532452819511,2.58035829740622));
#96911=CARTESIAN_POINT('Ctrl Pts',(-10.7408104349942,15.5536743358638,2.58439288855875));
#96912=CARTESIAN_POINT('Ctrl Pts',(-10.7496647316474,15.5544399156844,2.59163724412344));
#96913=CARTESIAN_POINT('Ctrl Pts',(-10.7535176198342,15.5547757870199,2.5948307885187));
#96914=CARTESIAN_POINT('Ctrl Pts',(-10.7614237631754,15.5554707354966,2.60146941511489));
#96915=CARTESIAN_POINT('Ctrl Pts',(-10.765474258161,15.5558299335185,2.60491759173413));
#96916=CARTESIAN_POINT('Ctrl Pts',(-10.7760401490486,15.5567753478283,2.61403648164033));
#96917=CARTESIAN_POINT('Ctrl Pts',(-10.7825166631317,15.557363376825,2.61975154996116));
#96918=CARTESIAN_POINT('Ctrl Pts',(-10.7965930004396,15.5586605765982,2.63245104846236));
#96919=CARTESIAN_POINT('Ctrl Pts',(-10.8041649825817,15.5593709551679,2.63946513103956));
#96920=CARTESIAN_POINT('Ctrl Pts',(-10.8263713766596,15.5614925092383,2.66058442476375));
#96921=CARTESIAN_POINT('Ctrl Pts',(-10.8407332908581,15.5629152328664,2.67496932915081));
#96922=CARTESIAN_POINT('Ctrl Pts',(-10.893434286723,15.5683322622743,2.73056026180022));
#96923=CARTESIAN_POINT('Ctrl Pts',(-10.9291719772552,15.5724206476545,2.77412089884531));
#96924=CARTESIAN_POINT('Ctrl Pts',(-11.006303335247,15.5822167179053,2.88321031515338));
#96925=CARTESIAN_POINT('Ctrl Pts',(-11.0446261002811,15.5879400390013,2.95060559192743));
#96926=CARTESIAN_POINT('Ctrl Pts',(-11.0798243951516,15.5940012599102,3.02972367831895));
#96927=CARTESIAN_POINT('Ctrl Pts',(-11.0834830188067,15.5946436053673,3.03821530520902));
#96928=CARTESIAN_POINT('Ctrl Pts',(-11.0884364190084,15.5955300407066,3.05009516109995));
#96929=CARTESIAN_POINT('Ctrl Pts',(-11.0898160055766,15.5957788275126,3.05344734111691));
#96930=CARTESIAN_POINT('Ctrl Pts',(-11.0921678045177,15.5962061901211,3.05923766233175));
#96931=CARTESIAN_POINT('Ctrl Pts',(-11.0931473735835,15.596385195041,3.06167275751346));
#96932=CARTESIAN_POINT('Ctrl Pts',(-11.0951905053741,15.5967606445765,3.06680119530579));
#96933=CARTESIAN_POINT('Ctrl Pts',(-11.0962522889287,15.5969569771928,3.0694952186432));
#96934=CARTESIAN_POINT('Ctrl Pts',(-11.0988440681521,15.5974393101586,3.07614300865987));
#96935=CARTESIAN_POINT('Ctrl Pts',(-11.1003626917843,15.5977246426164,3.08010122274846));
#96936=CARTESIAN_POINT('Ctrl Pts',(-11.1058868482925,15.5987730343144,3.09473544489942));
#96937=CARTESIAN_POINT('Ctrl Pts',(-11.1097588089668,15.5995286766528,3.10546167398037));
#96938=CARTESIAN_POINT('Ctrl Pts',(-11.1362624617959,15.6048669527807,3.18236225887081));
#96939=CARTESIAN_POINT('Ctrl Pts',(-11.1531188908204,15.6091789480721,3.25038918427057));
#96940=CARTESIAN_POINT('Ctrl Pts',(-11.1730673575496,15.6172258453243,3.37902675307541));
#96941=CARTESIAN_POINT('Ctrl Pts',(-11.1777168954739,15.6209453489766,3.43914164328542));
#96942=CARTESIAN_POINT('Ctrl Pts',(-11.1777498238975,15.624787527241,3.49935594293634));
#96943=CARTESIAN_POINT('Ctrl Pts',(-11.1777498238975,15.6247875272409,3.49935594293517));
#96944=CARTESIAN_POINT('Ctrl Pts',(-11.177761752659,15.6261794076629,3.52116937766792));
#96945=CARTESIAN_POINT('Ctrl Pts',(-11.1771680268943,15.6275849209456,3.54296784548813));
#96946=CARTESIAN_POINT('Ctrl Pts',(-11.175246262625,15.6298669495826,3.57787233849004));
#96947=CARTESIAN_POINT('Ctrl Pts',(-11.1743038763382,15.6307313594839,3.59098495780553));
#96948=CARTESIAN_POINT('Ctrl Pts',(-11.1726551053185,15.6319678083066,3.60956939399694));
#96949=CARTESIAN_POINT('Ctrl Pts',(-11.1721294427284,15.6323342813098,3.61505657691785));
#96950=CARTESIAN_POINT('Ctrl Pts',(-11.1710871171421,15.6330135732415,3.62518727707632));
#96951=CARTESIAN_POINT('Ctrl Pts',(-11.1705813034157,15.633326050214,3.62983181929543));
#96952=CARTESIAN_POINT('Ctrl Pts',(-11.169478262422,15.6339739831744,3.63942935272278));
#96953=CARTESIAN_POINT('Ctrl Pts',(-11.1688771732535,15.6343095534268,3.64438179665939));
#96954=CARTESIAN_POINT('Ctrl Pts',(-11.1674463569776,15.6350708687104,3.65557540231151));
#96955=CARTESIAN_POINT('Ctrl Pts',(-11.1665980168341,15.6354971871617,3.66181398786713));
#96956=CARTESIAN_POINT('Ctrl Pts',(-11.1639388808185,15.6367638231177,3.68025992376714));
#96957=CARTESIAN_POINT('Ctrl Pts',(-11.1619862387588,15.6376085455769,3.69244562648848));
#96958=CARTESIAN_POINT('Ctrl Pts',(-11.1539363650213,15.6408029794404,3.738079434383));
#96959=CARTESIAN_POINT('Ctrl Pts',(-11.1465837651145,15.6431911029996,3.77128624116019));
#96960=CARTESIAN_POINT('Ctrl Pts',(-11.1114071437773,15.6529131263646,3.90289019330814));
#96961=CARTESIAN_POINT('Ctrl Pts',(-11.0722666418055,15.6605583058709,3.9977815892684));
#96962=CARTESIAN_POINT('Ctrl Pts',(-11.0077369069689,15.6698853218501,4.11017331970739));
#96963=CARTESIAN_POINT('Ctrl Pts',(-10.9932744057967,15.6718294850041,4.13344406667698));
#96964=CARTESIAN_POINT('Ctrl Pts',(-10.974830726469,15.6741237219133,4.16093322318884));
#96965=CARTESIAN_POINT('Ctrl Pts',(-10.9716146310392,15.6745174626311,4.16565207342345));
#96966=CARTESIAN_POINT('Ctrl Pts',(-10.966533153882,15.6751295816648,4.1729926260965));
#96967=CARTESIAN_POINT('Ctrl Pts',(-10.9646911891974,15.6753494582162,4.17563031492671));
#96968=CARTESIAN_POINT('Ctrl Pts',(-10.9612248437051,15.6757594532525,4.18055103605163));
#96969=CARTESIAN_POINT('Ctrl Pts',(-10.9596031373696,15.675949735098,4.18283580149064));
#96970=CARTESIAN_POINT('Ctrl Pts',(-10.9558732693428,15.6763839195652,4.18805115166247));
#96971=CARTESIAN_POINT('Ctrl Pts',(-10.9537597742006,15.6766274559703,4.19097784938161));
#96972=CARTESIAN_POINT('Ctrl Pts',(-10.948086408654,15.6772747294821,4.19875851095811));
#96973=CARTESIAN_POINT('Ctrl Pts',(-10.9445026705007,15.6776769031198,4.20359505689349));
#96974=CARTESIAN_POINT('Ctrl Pts',(-10.9141763203613,15.6810266707566,4.24387364491772));
#96975=CARTESIAN_POINT('Ctrl Pts',(-10.885482896287,15.6838526043509,4.27780933790015));
#96976=CARTESIAN_POINT('Ctrl Pts',(-10.8090440451889,15.6908111577061,4.35848425102891));
#96977=CARTESIAN_POINT('Ctrl Pts',(-10.7591165231001,15.6948791396483,4.40293407589315));
#96978=CARTESIAN_POINT('Ctrl Pts',(-10.6767515444984,15.7013088343361,4.4645771830992));
#96979=CARTESIAN_POINT('Ctrl Pts',(-10.6468306971383,15.7035930851849,4.48489163386621));
#96980=CARTESIAN_POINT('Ctrl Pts',(-10.6029398222404,15.7069131051099,4.51182722503868));
#96981=CARTESIAN_POINT('Ctrl Pts',(-10.589699579295,15.7079107273866,4.51960047837317));
#96982=CARTESIAN_POINT('Ctrl Pts',(-10.5689143399039,15.7094733442095,4.53126305266973));
#96983=CARTESIAN_POINT('Ctrl Pts',(-10.5614725888179,15.7100321213202,4.53533353847116));
#96984=CARTESIAN_POINT('Ctrl Pts',(-10.5474543211416,15.7110838483694,4.54280565828641));
#96985=CARTESIAN_POINT('Ctrl Pts',(-10.5408884052169,15.7115761111437,4.54622636346372));
#96986=CARTESIAN_POINT('Ctrl Pts',(-10.5297340212421,15.7124120145146,4.55190449857282));
#96987=CARTESIAN_POINT('Ctrl Pts',(-10.5251622491513,15.7127545168353,4.55419439290754));
#96988=CARTESIAN_POINT('Ctrl Pts',(-10.516007276883,15.7134402450845,4.55870557359808));
#96989=CARTESIAN_POINT('Ctrl Pts',(-10.5114242911437,15.7137834554678,4.5609270447985));
#96990=CARTESIAN_POINT('Ctrl Pts',(-10.5002475324582,15.7146203790946,4.56625540960634));
#96991=CARTESIAN_POINT('Ctrl Pts',(-10.4936391170729,15.7151151548021,4.56933091706173));
#96992=CARTESIAN_POINT('Ctrl Pts',(-10.4747780588764,15.7165273266611,4.57789661922381));
#96993=CARTESIAN_POINT('Ctrl Pts',(-10.4624598308059,15.717449674415,4.5832387575681));
#96994=CARTESIAN_POINT('Ctrl Pts',(-10.3709071359389,15.7243076460911,4.62109687655362));
#96995=CARTESIAN_POINT('Ctrl Pts',(-10.2884415160426,15.7305284726804,4.64508800541817));
#96996=CARTESIAN_POINT('Ctrl Pts',(-10.133459201567,15.7420824978954,4.67236152475451));
#96997=CARTESIAN_POINT('Ctrl Pts',(-10.0618003882636,15.7473642515622,4.67831482822884));
#96998=CARTESIAN_POINT('Ctrl Pts',(-9.98282219017373,15.7528622073854,4.67764683668524));
#96999=CARTESIAN_POINT('Ctrl Pts',(-9.97560582810824,15.7533615015853,4.67751946056978));
#97000=CARTESIAN_POINT('Ctrl Pts',(-9.96486133799105,15.7540999018741,4.67723098986928));
#97001=CARTESIAN_POINT('Ctrl Pts',(-9.9613321913639,15.7543416335015,4.6771203551359));
#97002=CARTESIAN_POINT('Ctrl Pts',(-9.95528271212342,15.7547545581452,4.67690347496911));
#97003=CARTESIAN_POINT('Ctrl Pts',(-9.95276217138632,15.7549261739566,4.67680500220719));
#97004=CARTESIAN_POINT('Ctrl Pts',(-9.94703749135996,15.755314961416,4.67656292722283));
#97005=CARTESIAN_POINT('Ctrl Pts',(-9.94383361040631,15.7555318544521,4.67641433446639));
#97006=CARTESIAN_POINT('Ctrl Pts',(-9.93511827008212,15.75612005951,4.67597444011749));
#97007=CARTESIAN_POINT('Ctrl Pts',(-9.92960810135573,15.7564899889378,4.67565747829089));
#97008=CARTESIAN_POINT('Ctrl Pts',(-9.9022537832048,15.7583176303144,4.67389096482123));
#97009=CARTESIAN_POINT('Ctrl Pts',(-9.88044920179295,15.7597465657476,4.67187118545924));
#97010=CARTESIAN_POINT('Ctrl Pts',(-9.83679984521038,15.7625736047331,4.66659672743324));
#97011=CARTESIAN_POINT('Ctrl Pts',(-9.81496534681935,15.763970795932,4.66333335266161));
#97012=CARTESIAN_POINT('Ctrl Pts',(-9.69531446341559,15.7715949375259,4.64199607309003));
#97013=CARTESIAN_POINT('Ctrl Pts',(-9.60000441121922,15.7775855796425,4.61220156614234));
#97014=CARTESIAN_POINT('Ctrl Pts',(-9.48449557989681,15.7857279704919,4.55929738146958));
#97015=CARTESIAN_POINT('Ctrl Pts',(-9.45983291139068,15.7875195351527,4.54693604140466));
#97016=CARTESIAN_POINT('Ctrl Pts',(-9.42821244978103,15.7898990369194,4.52967249480587));
#97017=CARTESIAN_POINT('Ctrl Pts',(-9.4208405843612,15.7904597991368,4.52554415518738));
#97018=CARTESIAN_POINT('Ctrl Pts',(-9.4088434932997,15.79138262182,4.51865502148231));
#97019=CARTESIAN_POINT('Ctrl Pts',(-9.40419157339058,15.7917430035306,4.51594113281503));
#97020=CARTESIAN_POINT('Ctrl Pts',(-9.39521316460938,15.7924436092373,4.51062033399013));
#97021=CARTESIAN_POINT('Ctrl Pts',(-9.39088450379328,15.7927836875505,4.50801730473551));
#97022=CARTESIAN_POINT('Ctrl Pts',(-9.38089830387563,15.7935736749092,4.50192431802121));
#97023=CARTESIAN_POINT('Ctrl Pts',(-9.37525334595228,15.7940243115255,4.49841417472535));
#97024=CARTESIAN_POINT('Ctrl Pts',(-9.35694323219308,15.7954995678635,4.48681251080593));
#97025=CARTESIAN_POINT('Ctrl Pts',(-9.34440363509876,15.7965312862809,4.47852660059326));
#97026=CARTESIAN_POINT('Ctrl Pts',(-9.26482807917204,15.8032207955286,4.4237284779901));
#97027=CARTESIAN_POINT('Ctrl Pts',(-9.20263221955389,15.8091331884359,4.37060442993804));
#97028=CARTESIAN_POINT('Ctrl Pts',(-9.10896140987051,15.8191106589038,4.27207713806588));
#97029=CARTESIAN_POINT('Ctrl Pts',(-9.0742619757164,15.8231169123413,4.23011133406531));
#97030=CARTESIAN_POINT('Ctrl Pts',(-9.03321296510913,15.8281703167998,4.17281268673037));
#97031=CARTESIAN_POINT('Ctrl Pts',(-9.02410877069685,15.8293140522766,4.1595380545915));
#97032=CARTESIAN_POINT('Ctrl Pts',(-9.00938064686383,15.8311986162026,4.13709023893374));
#97033=CARTESIAN_POINT('Ctrl Pts',(-9.00360533997464,15.8319470648426,4.12801940845524));
#97034=CARTESIAN_POINT('Ctrl Pts',(-8.99577767109306,15.8329735357652,4.11534522278951));
#97035=CARTESIAN_POINT('Ctrl Pts',(-8.99361909551352,15.833257916871,4.11180855296335));
#97036=CARTESIAN_POINT('Ctrl Pts',(-8.98999351512012,15.8337377268542,4.10579719222085));
#97037=CARTESIAN_POINT('Ctrl Pts',(-8.98851684418025,15.833933768788,4.10332840457926));
#97038=CARTESIAN_POINT('Ctrl Pts',(-8.98569988824821,15.8343089075533,4.09857943574135));
#97039=CARTESIAN_POINT('Ctrl Pts',(-8.984358224542,15.8344880969254,4.09630012736003));
#97040=CARTESIAN_POINT('Ctrl Pts',(-8.9811571554265,15.8349169218492,4.09081978991472));
#97041=CARTESIAN_POINT('Ctrl Pts',(-8.97930512685464,15.8351660908035,4.08761445093899));
#97042=CARTESIAN_POINT('Ctrl Pts',(-8.9726210488151,15.8360694659802,4.07591924587095));
#97043=CARTESIAN_POINT('Ctrl Pts',(-8.96787939606275,15.8367182457984,4.06737779419613));
#97044=CARTESIAN_POINT('Ctrl Pts',(-8.93454089350355,15.8413454093333,4.00552160051157));
#97045=CARTESIAN_POINT('Ctrl Pts',(-8.9099796488634,15.8451147933833,3.95012527521383));
#97046=CARTESIAN_POINT('Ctrl Pts',(-8.87236327705549,15.8520936324839,3.84388142084387));
#97047=CARTESIAN_POINT('Ctrl Pts',(-8.85823416080146,15.8553012199524,3.79358062218364));
#97048=CARTESIAN_POINT('Ctrl Pts',(-8.84088206119212,15.8605910562537,3.7111157614684));
#97049=CARTESIAN_POINT('Ctrl Pts',(-8.83556215866905,15.8626277161817,3.67946737174046));
#97050=CARTESIAN_POINT('Ctrl Pts',(-8.82890168419637,15.866061789561,3.62675581642737));
#97051=CARTESIAN_POINT('Ctrl Pts',(-8.82682312079678,15.8674375711779,3.6058027584884));
#97052=CARTESIAN_POINT('Ctrl Pts',(-8.82475562427758,15.8693377264903,3.57716485642819));
#97053=CARTESIAN_POINT('Ctrl Pts',(-8.82427854369114,15.869846981453,3.56951841680842));
#97054=CARTESIAN_POINT('Ctrl Pts',(-8.8236019772305,15.8707070140562,3.55665674705193));
#97055=CARTESIAN_POINT('Ctrl Pts',(-8.82336248989264,15.8710565426199,3.5514437875224));
#97056=CARTESIAN_POINT('Ctrl Pts',(-8.82295778895651,15.8717492620643,3.54114150411683));
#97057=CARTESIAN_POINT('Ctrl Pts',(-8.82279092081317,15.87209239379,3.5360523565532));
#97058=CARTESIAN_POINT('Ctrl Pts',(-8.82246559326226,15.8729288330372,3.52368178288959));
#97059=CARTESIAN_POINT('Ctrl Pts',(-8.82234166654363,15.8734232000805,3.51639973738332));
#97060=CARTESIAN_POINT('Ctrl Pts',(-8.82218152583615,15.8748334349755,3.49571344286522));
#97061=CARTESIAN_POINT('Ctrl Pts',(-8.82230659714929,15.8757542347223,3.4823094447475));
#97062=CARTESIAN_POINT('Ctrl Pts',(-8.82492145912527,15.8826110869499,3.38328479435956));
#97063=CARTESIAN_POINT('Ctrl Pts',(-8.83651643837456,15.8888324734114,3.29817643161657));
#97064=CARTESIAN_POINT('Ctrl Pts',(-8.87459256600722,15.9003891345095,3.14545130232369));
#97065=CARTESIAN_POINT('Ctrl Pts',(-8.89828716821528,15.9056729141352,3.07753375536569));
#97066=CARTESIAN_POINT('Ctrl Pts',(-8.93101100335317,15.9111727028667,3.00562193106713));
#97067=CARTESIAN_POINT('Ctrl Pts',(-8.93406067510026,15.9116720013875,2.99908033362235));
#97068=CARTESIAN_POINT('Ctrl Pts',(-8.93869163338618,15.912410406792,2.98938068963488));
#97069=CARTESIAN_POINT('Ctrl Pts',(-8.94022722977,15.912652139266,2.98620120137853));
#97070=CARTESIAN_POINT('Ctrl Pts',(-8.94288435041313,15.9130650648525,2.98076216563614));
#97071=CARTESIAN_POINT('Ctrl Pts',(-8.94399885758412,15.9132366807656,2.97849926855728));
#97072=CARTESIAN_POINT('Ctrl Pts',(-8.9465469661601,15.9136254677741,2.97336724895143));
#97073=CARTESIAN_POINT('Ctrl Pts',(-8.94798502215157,15.9138423602619,2.97050039094686));
#97074=CARTESIAN_POINT('Ctrl Pts',(-8.95192948105874,15.9144305623703,2.96271636018252));
#97075=CARTESIAN_POINT('Ctrl Pts',(-8.95445880375256,15.9148004894201,2.95781079666966));
#97076=CARTESIAN_POINT('Ctrl Pts',(-8.96719141551378,15.9166280998969,2.93353664802352));
#97077=CARTESIAN_POINT('Ctrl Pts',(-8.97789959592997,15.9180570079712,2.91443598660133));
#97078=CARTESIAN_POINT('Ctrl Pts',(-9.00046079605369,15.920884026304,2.87669943184795));
#97079=CARTESIAN_POINT('Ctrl Pts',(-9.01231760843708,15.922281223223,2.85807647714523));
#97080=CARTESIAN_POINT('Ctrl Pts',(-9.08044728321178,15.9299053305923,2.75742948122007));
#97081=CARTESIAN_POINT('Ctrl Pts',(-9.14640992292165,15.935895932523,2.68245939409084));
#97082=CARTESIAN_POINT('Ctrl Pts',(-9.24169781415504,15.944038328813,2.59842715571879));
#97083=CARTESIAN_POINT('Ctrl Pts',(-9.26301731027366,15.9458299498601,2.58091778251157));
#97084=CARTESIAN_POINT('Ctrl Pts',(-9.2916440442888,15.9482095160661,2.55904394855642));
#97085=CARTESIAN_POINT('Ctrl Pts',(-9.29841250159619,15.9487702844499,2.55398656106795));
#97086=CARTESIAN_POINT('Ctrl Pts',(-9.30958344558528,15.9496931146866,2.54582546155538));
#97087=CARTESIAN_POINT('Ctrl Pts',(-9.3139539260595,15.9500534977304,2.54267829272718));
#97088=CARTESIAN_POINT('Ctrl Pts',(-9.32246484202575,15.9507541041723,2.53663782233348));
#97089=CARTESIAN_POINT('Ctrl Pts',(-9.32660261429722,15.9510941818756,2.53374095853776));
#97090=CARTESIAN_POINT('Ctrl Pts',(-9.33622863092652,15.9518841650775,2.52709362315991));
#97091=CARTESIAN_POINT('Ctrl Pts',(-9.34173020396016,15.9523347981234,2.52336285091671));
#97092=CARTESIAN_POINT('Ctrl Pts',(-9.35977250766573,15.9538100305901,2.51134956264405));
#97093=CARTESIAN_POINT('Ctrl Pts',(-9.37243980266421,15.9548417283877,2.50326077052136));
#97094=CARTESIAN_POINT('Ctrl Pts',(-9.45486104241834,15.961531955599,2.45282412212095));
#97095=CARTESIAN_POINT('Ctrl Pts',(-9.52868969252329,15.9674451611739,2.41758797531464));
#97096=CARTESIAN_POINT('Ctrl Pts',(-9.65678882607535,15.9774228400901,2.3720558129096));
#97097=CARTESIAN_POINT('Ctrl Pts',(-9.70922826639941,15.9814284824155,2.35741329801038));
#97098=CARTESIAN_POINT('Ctrl Pts',(-9.77825614559363,15.9864812027241,2.343201096522));
#97099=CARTESIAN_POINT('Ctrl Pts',(-9.79408401900635,15.9876248425736,2.34027904069928));
#97100=CARTESIAN_POINT('Ctrl Pts',(-9.81034639637981,15.9887815099625,2.33762023398126));
#97101=CARTESIAN_POINT('Ctrl Pts',(-9.81072521498865,15.9888084433933,2.33755848939621));
#97102=CARTESIAN_POINT('Ctrl Pts',(-9.81110406371144,15.9888353687451,2.33749693000248));
#97103=CARTESIAN_POINT('Origin',(-10.,12.3756328852638,3.5));
#97104=CARTESIAN_POINT('',(-9.81110406371068,16.5874147438851,2.3374969300026));
#97105=CARTESIAN_POINT('',(-9.81110406371068,16.4876146309988,2.3374969300026));
#97106=CARTESIAN_POINT('',(-9.81110406371068,12.3756328852638,2.3374969300026));
#97107=CARTESIAN_POINT('Ctrl Pts',(-9.81110406371068,16.5874147438851,2.3374969300026));
#97108=CARTESIAN_POINT('Ctrl Pts',(-9.79408468926281,16.5863079989926,2.34026242005107));
#97109=CARTESIAN_POINT('Ctrl Pts',(-9.77711811835858,16.5851910491628,2.34340294741657));
#97110=CARTESIAN_POINT('Ctrl Pts',(-9.74696993641862,16.5831775822287,2.34967225854604));
#97111=CARTESIAN_POINT('Ctrl Pts',(-9.73377215044021,16.5822862330308,2.35265487610149));
#97112=CARTESIAN_POINT('Ctrl Pts',(-9.71436711100458,16.5809596121411,2.35739312721334));
#97113=CARTESIAN_POINT('Ctrl Pts',(-9.70811788197619,16.5805299106053,2.35897351502779));
#97114=CARTESIAN_POINT('Ctrl Pts',(-9.69703807990843,16.5797635059656,2.36187249933278));
#97115=CARTESIAN_POINT('Ctrl Pts',(-9.69220231246993,16.5794274614067,2.36317076259259));
#97116=CARTESIAN_POINT('Ctrl Pts',(-9.68204187876341,16.5787180639963,2.36596812472266));
#97117=CARTESIAN_POINT('Ctrl Pts',(-9.67671921482961,16.578344500852,2.36747397683905));
#97118=CARTESIAN_POINT('Ctrl Pts',(-9.66265810669044,16.5773524023741,2.3715592518712));
#97119=CARTESIAN_POINT('Ctrl Pts',(-9.65393879282778,16.5767318158725,2.37420263467108));
#97120=CARTESIAN_POINT('Ctrl Pts',(-9.61221804355026,16.5737357786153,2.38738133802136));
#97121=CARTESIAN_POINT('Ctrl Pts',(-9.57966459656168,16.5713169106818,2.3992671295671));
#97122=CARTESIAN_POINT('Ctrl Pts',(-9.48613439787508,16.564121547153,2.43817085903942));
#97123=CARTESIAN_POINT('Ctrl Pts',(-9.4268749206994,16.5592384804651,2.46894967299835));
#97124=CARTESIAN_POINT('Ctrl Pts',(-9.31850085655684,16.5498232420847,2.53747964696441));
#97125=CARTESIAN_POINT('Ctrl Pts',(-9.26911361717667,16.5453091615741,2.57442279852042));
#97126=CARTESIAN_POINT('Ctrl Pts',(-9.21551297330088,16.5403103584506,2.62149546971246));
#97127=CARTESIAN_POINT('Ctrl Pts',(-9.20826765431734,16.5396324873437,2.62801948813788));
#97128=CARTESIAN_POINT('Ctrl Pts',(-9.19838513695731,16.5387058464639,2.63714290568825));
#97129=CARTESIAN_POINT('Ctrl Pts',(-9.19567817661452,16.5384518119952,2.63966567009587));
#97130=CARTESIAN_POINT('Ctrl Pts',(-9.19105668636879,16.5380178082519,2.64401356691796));
#97131=CARTESIAN_POINT('Ctrl Pts',(-9.18913635396772,16.5378373801215,2.64583244841163));
#97132=CARTESIAN_POINT('Ctrl Pts',(-9.18513904347096,16.5374616486359,2.64964421027428));
#97133=CARTESIAN_POINT('Ctrl Pts',(-9.18306322311956,16.5372664438976,2.65163825497827));
#97134=CARTESIAN_POINT('Ctrl Pts',(-9.17801360693692,16.5367913209343,2.65652466488151));
#97135=CARTESIAN_POINT('Ctrl Pts',(-9.17504770412508,16.5365120248615,2.65942520727319));
#97136=CARTESIAN_POINT('Ctrl Pts',(-9.16442970244067,16.5355110212583,2.66991954732166));
#97137=CARTESIAN_POINT('Ctrl Pts',(-9.15686634441118,16.5347958841342,2.6776029308858));
#97138=CARTESIAN_POINT('Ctrl Pts',(-9.1382393716952,16.533025915166,2.69705263048693));
#97139=CARTESIAN_POINT('Ctrl Pts',(-9.12730999438134,16.5319794215196,2.70894496576112));
#97140=CARTESIAN_POINT('Ctrl Pts',(-9.08043974925024,16.5274360366953,2.76209899527789));
#97141=CARTESIAN_POINT('Ctrl Pts',(-9.04715240375305,16.5240584114185,2.80561440427617));
#97142=CARTESIAN_POINT('Ctrl Pts',(-8.97231947764012,16.5156600511642,2.91900872634387));
#97143=CARTESIAN_POINT('Ctrl Pts',(-8.93475204657371,16.5106428630481,2.99115541704199));
#97144=CARTESIAN_POINT('Ctrl Pts',(-8.8993629247579,16.5043708741205,3.0805725705774));
#97145=CARTESIAN_POINT('Ctrl Pts',(-8.8940959378516,16.5033816679124,3.09466370537582));
#97146=CARTESIAN_POINT('Ctrl Pts',(-8.88689155917966,16.5019422763355,3.1151248289143));
#97147=CARTESIAN_POINT('Ctrl Pts',(-8.8847358802319,16.5014992501638,3.12141680115294));
#97148=CARTESIAN_POINT('Ctrl Pts',(-8.88103643866512,16.5007165578909,3.13252055284595));
#97149=CARTESIAN_POINT('Ctrl Pts',(-8.87947012161172,16.500377637837,3.13732468246038));
#97150=CARTESIAN_POINT('Ctrl Pts',(-8.87629793577131,16.4996752962943,3.14727099174285));
#97151=CARTESIAN_POINT('Ctrl Pts',(-8.87469633850272,16.4993117450035,3.15241439878776));
#97152=CARTESIAN_POINT('Ctrl Pts',(-8.8706734003786,16.4983749851343,3.16565304178214));
#97153=CARTESIAN_POINT('Ctrl Pts',(-8.86830382397239,16.4978001187663,3.17376355849627));
#97154=CARTESIAN_POINT('Ctrl Pts',(-8.85857577489246,16.4953374979942,3.20844243424092));
#97155=CARTESIAN_POINT('Ctrl Pts',(-8.85206464246632,16.4934229646919,3.23523733102931));
#97156=CARTESIAN_POINT('Ctrl Pts',(-8.82640825252528,16.484468686366,3.35970703827271));
#97157=CARTESIAN_POINT('Ctrl Pts',(-8.81875521127112,16.4770852947845,3.45932427098685));
#97158=CARTESIAN_POINT('Ctrl Pts',(-8.82481469572238,16.4682228315322,3.58076473921803));
#97159=CARTESIAN_POINT('Ctrl Pts',(-8.82653708329256,16.4666224812038,3.60280233222635));
#97160=CARTESIAN_POINT('Ctrl Pts',(-8.83119239825596,16.463479623788,3.64649495526358));
#97161=CARTESIAN_POINT('Ctrl Pts',(-8.83410985987507,16.4619372282388,3.66814372477024));
#97162=CARTESIAN_POINT('Ctrl Pts',(-8.83851636563263,16.4600419833879,3.6951441860628));
#97163=CARTESIAN_POINT('Ctrl Pts',(-8.83944304568615,16.4596617607809,3.70058176648894));
#97164=CARTESIAN_POINT('Ctrl Pts',(-8.84096891532767,16.4590637129155,3.70917048831032));
#97165=CARTESIAN_POINT('Ctrl Pts',(-8.84154281942247,16.4588445314184,3.71232595180354));
#97166=CARTESIAN_POINT('Ctrl Pts',(-8.84259132210304,16.4584541926773,3.71796004958876));
#97167=CARTESIAN_POINT('Ctrl Pts',(-8.84306099457255,16.4582827683767,3.720439490082));
#97168=CARTESIAN_POINT('Ctrl Pts',(-8.84420752393593,16.4578723647165,3.72638750690595));
#97169=CARTESIAN_POINT('Ctrl Pts',(-8.84489202664998,16.4576338184834,3.72985456648329));
#97170=CARTESIAN_POINT('Ctrl Pts',(-8.84702427888503,16.4569098594624,3.74040447241923));
#97171=CARTESIAN_POINT('Ctrl Pts',(-8.8485216777548,16.4564271372083,3.74747727919922));
#97172=CARTESIAN_POINT('Ctrl Pts',(-8.86263946094417,16.4520942392961,3.8112570915323));
#97173=CARTESIAN_POINT('Ctrl Pts',(-8.8793762232298,16.4484506817385,3.86697988372485));
#97174=CARTESIAN_POINT('Ctrl Pts',(-8.93641930215884,16.4385528055183,4.01591470650515));
#97175=CARTESIAN_POINT('Ctrl Pts',(-8.98474350453736,16.4323796812434,4.10549490890791));
#97176=CARTESIAN_POINT('Ctrl Pts',(-9.0518394195919,16.4248670774143,4.19876293572158));
#97177=CARTESIAN_POINT('Ctrl Pts',(-9.05992910494375,16.4239757264364,4.20960891639439));
#97178=CARTESIAN_POINT('Ctrl Pts',(-9.07214594089555,16.4226491033988,4.22541261230133));
#97179=CARTESIAN_POINT('Ctrl Pts',(-9.07613003742487,16.4222194015214,4.23047991248821));
#97180=CARTESIAN_POINT('Ctrl Pts',(-9.08328239131766,16.4214529964984,4.23942474853006));
#97181=CARTESIAN_POINT('Ctrl Pts',(-9.08643418231023,16.4211169519,4.24331529530101));
#97182=CARTESIAN_POINT('Ctrl Pts',(-9.09311998300004,16.4204075546388,4.25146143995624));
#97183=CARTESIAN_POINT('Ctrl Pts',(-9.09665934894785,16.4200339916846,4.25571246339029));
#97184=CARTESIAN_POINT('Ctrl Pts',(-9.1061073833304,16.4190418942558,4.26689899247183));
#97185=CARTESIAN_POINT('Ctrl Pts',(-9.11206671329609,16.418421308621,4.2737910215464));
#97186=CARTESIAN_POINT('Ctrl Pts',(-9.1410659093832,16.4154252827519,4.30655275719454));
#97187=CARTESIAN_POINT('Ctrl Pts',(-9.16515754406224,16.4130064257417,4.33146423052054));
#97188=CARTESIAN_POINT('Ctrl Pts',(-9.23871953175109,16.4058111118984,4.40110540981117));
#97189=CARTESIAN_POINT('Ctrl Pts',(-9.29092797697519,16.4009280858699,4.44273746547733));
#97190=CARTESIAN_POINT('Ctrl Pts',(-9.39759254244523,16.3915128341171,4.51389933169584));
#97191=CARTESIAN_POINT('Ctrl Pts',(-9.45142135247845,16.3869986996223,4.54400652067674));
#97192=CARTESIAN_POINT('Ctrl Pts',(-9.51621781116061,16.3819998469364,4.57384584486822));
#97193=CARTESIAN_POINT('Ctrl Pts',(-9.5251235969447,16.3813219758873,4.57781376966188));
#97194=CARTESIAN_POINT('Ctrl Pts',(-9.53747630924262,16.3803953350716,4.58313461275248));
#97195=CARTESIAN_POINT('Ctrl Pts',(-9.54088157399948,16.3801413006102,4.58458241996252));
#97196=CARTESIAN_POINT('Ctrl Pts',(-9.54673260082257,16.3797072968761,4.58703759048707));
#97197=CARTESIAN_POINT('Ctrl Pts',(-9.54917501022853,16.3795268687476,4.58805279616416));
#97198=CARTESIAN_POINT('Ctrl Pts',(-9.55428247776101,16.3791511372624,4.5901556026388));
#97199=CARTESIAN_POINT('Ctrl Pts',(-9.55694812910274,16.3789559325226,4.59124167237633));
#97200=CARTESIAN_POINT('Ctrl Pts',(-9.56346519749256,16.3784808095495,4.59386911353));
#97201=CARTESIAN_POINT('Ctrl Pts',(-9.56732087741935,16.3782015134684,4.59539994957133));
#97202=CARTESIAN_POINT('Ctrl Pts',(-9.58122510704826,16.3772005098025,4.60083553228126));
#97203=CARTESIAN_POINT('Ctrl Pts',(-9.59131943710219,16.3764853726251,4.60462278538938));
#97204=CARTESIAN_POINT('Ctrl Pts',(-9.61666128407167,16.374715403498,4.61373573509516));
#97205=CARTESIAN_POINT('Ctrl Pts',(-9.63196937591183,16.3736689097479,4.61888756043132));
#97206=CARTESIAN_POINT('Ctrl Pts',(-9.69958577349557,16.3691255241802,4.64010536406049));
#97207=CARTESIAN_POINT('Ctrl Pts',(-9.75287462376389,16.3657478983034,4.65283084047908));
#97208=CARTESIAN_POINT('Ctrl Pts',(-9.88689639807948,16.3573495382542,4.67511092631538));
#97209=CARTESIAN_POINT('Ctrl Pts',(-9.96808428688454,16.3523323509203,4.6801090614651));
#97210=CARTESIAN_POINT('Ctrl Pts',(-10.0641661153907,16.3460603628537,4.67609695586526));
#97211=CARTESIAN_POINT('Ctrl Pts',(-10.0791815476522,16.3450711566235,4.67518151318752));
#97212=CARTESIAN_POINT('Ctrl Pts',(-10.1008044976608,16.3436317650201,4.67344695303873));
#97213=CARTESIAN_POINT('Ctrl Pts',(-10.1074294628925,16.3431887388445,4.67285898802661));
#97214=CARTESIAN_POINT('Ctrl Pts',(-10.1190782688419,16.342406046567,4.67172563408231));
#97215=CARTESIAN_POINT('Ctrl Pts',(-10.1241042879964,16.3420671265125,4.67120396174805));
#97216=CARTESIAN_POINT('Ctrl Pts',(-10.1344812665587,16.3413647849708,4.670059345231));
#97217=CARTESIAN_POINT('Ctrl Pts',(-10.1398316111107,16.3410012336816,4.66943199942673));
#97218=CARTESIAN_POINT('Ctrl Pts',(-10.1535624792038,16.3400644738216,4.66772643288611));
#97219=CARTESIAN_POINT('Ctrl Pts',(-10.1619359232643,16.3394896074611,4.66659470569483));
#97220=CARTESIAN_POINT('Ctrl Pts',(-10.1975749006267,16.3370269867675,4.6613867720959));
#97221=CARTESIAN_POINT('Ctrl Pts',(-10.2247029905823,16.3351124535383,4.65644430126276));
#97222=CARTESIAN_POINT('Ctrl Pts',(-10.3488549121657,16.3261581752415,4.62929179367547));
#97223=CARTESIAN_POINT('Ctrl Pts',(-10.4429821669369,16.3187747836049,4.5957922092073));
#97224=CARTESIAN_POINT('Ctrl Pts',(-10.5514746902357,16.3099123203006,4.54089341842305));
#97225=CARTESIAN_POINT('Ctrl Pts',(-10.570909496116,16.3083119699782,4.53036201581735));
#97226=CARTESIAN_POINT('Ctrl Pts',(-10.6089375213839,16.3051691125312,4.50834868814557));
#97227=CARTESIAN_POINT('Ctrl Pts',(-10.6275313071981,16.303626716946,4.49688343828562));
#97228=CARTESIAN_POINT('Ctrl Pts',(-10.6504094721501,16.3017314720575,4.48188237828943));
#97229=CARTESIAN_POINT('Ctrl Pts',(-10.6550009112291,16.3013512494475,4.47882546735543));
#97230=CARTESIAN_POINT('Ctrl Pts',(-10.662227873313,16.3007532015785,4.4739402405816));
#97231=CARTESIAN_POINT('Ctrl Pts',(-10.6648776231661,16.3005340200808,4.4721332703153));
#97232=CARTESIAN_POINT('Ctrl Pts',(-10.6695990948661,16.3001436813391,4.46888517536519));
#97233=CARTESIAN_POINT('Ctrl Pts',(-10.6716735556494,16.2999722570386,4.46744822378684));
#97234=CARTESIAN_POINT('Ctrl Pts',(-10.6766419978878,16.2995618533794,4.46398296546346));
#97235=CARTESIAN_POINT('Ctrl Pts',(-10.6795314857109,16.2993233071472,4.46194828954442));
#97236=CARTESIAN_POINT('Ctrl Pts',(-10.6883038280757,16.2985993481319,4.45571186248531));
#97237=CARTESIAN_POINT('Ctrl Pts',(-10.694157328634,16.2981166258825,4.45146882945426));
#97238=CARTESIAN_POINT('Ctrl Pts',(-10.7466920010841,16.2937837281405,4.41264507233434));
#97239=CARTESIAN_POINT('Ctrl Pts',(-10.7908007315756,16.2901401707307,4.37470342789388));
#97240=CARTESIAN_POINT('Ctrl Pts',(-10.9036902665696,16.2802422944522,4.26204710351733));
#97241=CARTESIAN_POINT('Ctrl Pts',(-10.965893739435,16.2740691699931,4.18148303065883));
#97242=CARTESIAN_POINT('Ctrl Pts',(-11.0238364116459,16.2665565659719,4.08226894881557));
#97243=CARTESIAN_POINT('Ctrl Pts',(-11.0304577206909,16.265665215021,4.07046909453154));
#97244=CARTESIAN_POINT('Ctrl Pts',(-11.0399311240431,16.2643385920159,4.0528832339002));
#97245=CARTESIAN_POINT('Ctrl Pts',(-11.0429414898042,16.2639088901437,4.04718338712117));
#97246=CARTESIAN_POINT('Ctrl Pts',(-11.0482067967452,16.2631424851265,4.03701270382011));
#97247=CARTESIAN_POINT('Ctrl Pts',(-11.0504803186663,16.2628064405287,4.03255162338894));
#97248=CARTESIAN_POINT('Ctrl Pts',(-11.0552055336801,16.2620970432652,4.02313185973158));
#97249=CARTESIAN_POINT('Ctrl Pts',(-11.0576508700904,16.2617234803081,4.01817014210034));
#97250=CARTESIAN_POINT('Ctrl Pts',(-11.0640311911888,16.2607313828635,4.00499079097704));
#97251=CARTESIAN_POINT('Ctrl Pts',(-11.0679058603511,16.2601107972156,3.99674454208771));
#97252=CARTESIAN_POINT('Ctrl Pts',(-11.0860515789608,16.257114771174,3.9569322599231));
#97253=CARTESIAN_POINT('Ctrl Pts',(-11.0990196096179,16.2546959139986,3.92479476304034));
#97254=CARTESIAN_POINT('Ctrl Pts',(-11.1327470344868,16.2475005994033,3.82927658261698));
#97255=CARTESIAN_POINT('Ctrl Pts',(-11.1495632569813,16.2426175727593,3.76465332402885));
#97256=CARTESIAN_POINT('Ctrl Pts',(-11.1712247110378,16.233202321209,3.63827246531873));
#97257=CARTESIAN_POINT('Ctrl Pts',(-11.1768524600664,16.2286881875312,3.57685332554508));
#97258=CARTESIAN_POINT('Ctrl Pts',(-11.1777774019412,16.2236893355954,3.50552234152789));
#97259=CARTESIAN_POINT('Ctrl Pts',(-11.177782768323,16.2230114645455,3.49577260209303));
#97260=CARTESIAN_POINT('Ctrl Pts',(-11.1776231566506,16.2220848237288,3.48232360968427));
#97261=CARTESIAN_POINT('Ctrl Pts',(-11.1775618094444,16.2218307892673,3.47862385154178));
#97262=CARTESIAN_POINT('Ctrl Pts',(-11.1774267116539,16.221396785533,3.47228002573966));
#97263=CARTESIAN_POINT('Ctrl Pts',(-11.17736148911,16.2212163574045,3.46963583355809));
#97264=CARTESIAN_POINT('Ctrl Pts',(-11.1772066876413,16.2208406259193,3.46411459672561));
#97265=CARTESIAN_POINT('Ctrl Pts',(-11.1771154687181,16.2206454211796,3.46123763241353));
#97266=CARTESIAN_POINT('Ctrl Pts',(-11.1768670390667,16.2201702982065,3.45421524605915));
#97267=CARTESIAN_POINT('Ctrl Pts',(-11.1766984698143,16.2198910021255,3.45007021155055));
#97268=CARTESIAN_POINT('Ctrl Pts',(-11.1760130389459,16.2188899984606,3.43515701789258));
#97269=CARTESIAN_POINT('Ctrl Pts',(-11.1753702193692,16.2181748612839,3.42439478912335));
#97270=CARTESIAN_POINT('Ctrl Pts',(-11.1733955579491,16.2164048921591,3.39753672198264));
#97271=CARTESIAN_POINT('Ctrl Pts',(-11.17188023436,16.2153583984105,3.38145621285716));
#97272=CARTESIAN_POINT('Ctrl Pts',(-11.1637817864671,16.2108150128535,3.31105317648322));
#97273=CARTESIAN_POINT('Ctrl Pts',(-11.1537480058582,16.2074373869853,3.25719259216043));
#97274=CARTESIAN_POINT('Ctrl Pts',(-11.1196418042736,16.1990424188514,3.12573880379287));
#97275=CARTESIAN_POINT('Ctrl Pts',(-11.0912322294689,16.1940286445765,3.04957871392895));
#97276=CARTESIAN_POINT('Ctrl Pts',(-11.0485315156706,16.1877581862416,2.96343302109303));
#97277=CARTESIAN_POINT('Ctrl Pts',(-11.0415757573983,16.1867665725221,2.95005239337552));
#97278=CARTESIAN_POINT('Ctrl Pts',(-11.0311816900047,16.1853243057663,2.93096247280851));
#97279=CARTESIAN_POINT('Ctrl Pts',(-11.0279486510086,16.1848808525471,2.92514266728035));
#97280=CARTESIAN_POINT('Ctrl Pts',(-11.022174739153,16.1840976618363,2.91495349821784));
#97281=CARTESIAN_POINT('Ctrl Pts',(-11.0196547342581,16.1837586733844,2.91057245725058));
#97282=CARTESIAN_POINT('Ctrl Pts',(-11.0147577968373,16.1831052577301,2.90218449286436));
#97283=CARTESIAN_POINT('Ctrl Pts',(-11.0123851295821,16.1827909886554,2.89817517902933));
#97284=CARTESIAN_POINT('Ctrl Pts',(-11.0061964560348,16.1819771542547,2.88785777160712));
#97285=CARTESIAN_POINT('Ctrl Pts',(-11.0023449418329,16.1814763097253,2.8815713224651));
#97286=CARTESIAN_POINT('Ctrl Pts',(-10.9876822974165,16.1795901425581,2.8581357549737));
#97287=CARTESIAN_POINT('Ctrl Pts',(-10.9764885523315,16.1781909210222,2.84123141525989));
#97288=CARTESIAN_POINT('Ctrl Pts',(-10.9473006139978,16.174638326209,2.79953247481193));
#97289=CARTESIAN_POINT('Ctrl Pts',(-10.9287657176189,16.172466070771,2.77513644367566));
#97290=CARTESIAN_POINT('Ctrl Pts',(-10.8621339944376,16.1649341722304,2.69419088002059));
#97291=CARTESIAN_POINT('Ctrl Pts',(-10.8096567822685,16.159442653724,2.64147936607834));
#97292=CARTESIAN_POINT('Ctrl Pts',(-10.7173604083933,16.1506797736799,2.56480750142563));
#97293=CARTESIAN_POINT('Ctrl Pts',(-10.6804649503172,16.1473746905649,2.53762823785868));
#97294=CARTESIAN_POINT('Ctrl Pts',(-10.6370360887088,16.1437739843242,2.50938593056304));
#97295=CARTESIAN_POINT('Ctrl Pts',(-10.6319704890512,16.1433582589938,2.50614663171684));
#97296=CARTESIAN_POINT('Ctrl Pts',(-10.6238252127735,16.142696856501,2.50102543151368));
#97297=CARTESIAN_POINT('Ctrl Pts',(-10.6207613892584,16.1424496547698,2.49911869681951));
#97298=CARTESIAN_POINT('Ctrl Pts',(-10.6153026851348,16.1420120954631,2.4957562437264));
#97299=CARTESIAN_POINT('Ctrl Pts',(-10.6129113148018,16.1418213827023,2.49429495518447));
#97300=CARTESIAN_POINT('Ctrl Pts',(-10.6077610925512,16.1414127559472,2.49117301524958));
#97301=CARTESIAN_POINT('Ctrl Pts',(-10.6050006367243,16.1411950194844,2.48951513570398));
#97302=CARTESIAN_POINT('Ctrl Pts',(-10.5973173725961,16.1405924381029,2.48494347834722));
#97303=CARTESIAN_POINT('Ctrl Pts',(-10.5923800008438,16.140209124375,2.482054164676));
#97304=CARTESIAN_POINT('Ctrl Pts',(-10.563786695884,16.138010577551,2.46560006922446));
#97305=CARTESIAN_POINT('Ctrl Pts',(-10.5396843002631,16.1362408546049,2.45282294520855));
#97306=CARTESIAN_POINT('Ctrl Pts',(-10.4758661271673,16.1317115594384,2.42178128547248));
#97307=CARTESIAN_POINT('Ctrl Pts',(-10.4355386100046,16.1290004131391,2.40486951348911));
#97308=CARTESIAN_POINT('Ctrl Pts',(-10.3496063399594,16.123358642311,2.37433286219889));
#97309=CARTESIAN_POINT('Ctrl Pts',(-10.303930128911,16.1204339985987,2.36115084987585));
#97310=CARTESIAN_POINT('Ctrl Pts',(-10.2102449955396,16.1144105367713,2.34015273091622));
#97311=CARTESIAN_POINT('Ctrl Pts',(-10.1623007627449,16.1113148567481,2.33247859112658));
#97312=CARTESIAN_POINT('Ctrl Pts',(-10.1046987783066,16.1075085993253,2.32687553621102));
#97313=CARTESIAN_POINT('Ctrl Pts',(-10.0953634708839,16.1068891345141,2.32607979750357));
#97314=CARTESIAN_POINT('Ctrl Pts',(-10.0799113289411,16.1058590051262,2.3249481898576));
#97315=CARTESIAN_POINT('Ctrl Pts',(-10.0737994812606,16.1054503235702,2.32454850751636));
#97316=CARTESIAN_POINT('Ctrl Pts',(-10.0627167799741,16.1047069027666,2.32391053404979));
#97317=CARTESIAN_POINT('Ctrl Pts',(-10.0577469736507,16.1043726748621,2.32365604003823));
#97318=CARTESIAN_POINT('Ctrl Pts',(-10.0480886605663,16.1037214111156,2.32322280936124));
#97319=CARTESIAN_POINT('Ctrl Pts',(-10.0434003979779,16.10340449037,2.32304057842494));
#97320=CARTESIAN_POINT('Ctrl Pts',(-10.0330862992218,16.1027054818534,2.32270138309461));
#97321=CARTESIAN_POINT('Ctrl Pts',(-10.0274602017258,16.1023230194205,2.32255672239816));
#97322=CARTESIAN_POINT('Ctrl Pts',(-10.0135673260802,16.1013756067731,2.32229912919589));
#97323=CARTESIAN_POINT('Ctrl Pts',(-10.0053000890746,16.1008092290808,2.32223291079363));
#97324=CARTESIAN_POINT('Ctrl Pts',(-9.93473820482176,16.0959522031599,2.32241067037843));
#97325=CARTESIAN_POINT('Ctrl Pts',(-9.87257431215225,16.0915127275951,2.32750857337014));
#97326=CARTESIAN_POINT('Ctrl Pts',(-9.81110382412688,16.0869811837922,2.33749696893276));
#97327=CARTESIAN_POINT('Ctrl Pts',(-9.81110406371144,15.9888353687451,2.33749693000248));
#97328=CARTESIAN_POINT('Ctrl Pts',(-9.82133771573714,15.9895626898729,2.33583405673277));
#97329=CARTESIAN_POINT('Ctrl Pts',(-9.83159334100925,15.990284118573,2.33430631312731));
#97330=CARTESIAN_POINT('Ctrl Pts',(-9.84597389410354,15.9912840874479,2.33235785149294));
#97331=CARTESIAN_POINT('Ctrl Pts',(-9.85008252380784,15.9915684616825,2.33182322403291));
#97332=CARTESIAN_POINT('Ctrl Pts',(-9.85704846604702,15.9920482634948,2.33095415126994));
#97333=CARTESIAN_POINT('Ctrl Pts',(-9.8599043141404,15.992244304081,2.33060847575621));
#97334=CARTESIAN_POINT('Ctrl Pts',(-9.86538829123958,15.9926194429707,2.32996506651554));
#97335=CARTESIAN_POINT('Ctrl Pts',(-9.8680161832272,15.9927986337989,2.32966571862036));
#97336=CARTESIAN_POINT('Ctrl Pts',(-9.87432461832978,15.9932274657452,2.32896863186599));
#97337=CARTESIAN_POINT('Ctrl Pts',(-9.87800610081821,15.9934766402319,2.32857938544761));
#97338=CARTESIAN_POINT('Ctrl Pts',(-9.89140921393852,15.9943800648311,2.3272261338329));
#97339=CARTESIAN_POINT('Ctrl Pts',(-9.90114123387,15.9950288877394,2.32636570446306));
#97340=CARTESIAN_POINT('Ctrl Pts',(-9.97119418477143,15.9996551213019,2.32104976953188));
#97341=CARTESIAN_POINT('Ctrl Pts',(-10.0317764879289,16.0034236396761,2.32112527908273));
#97342=CARTESIAN_POINT('Ctrl Pts',(-10.1440973668961,16.0103999893853,2.32993493739083));
#97343=CARTESIAN_POINT('Ctrl Pts',(-10.1957731744748,16.0136059774717,2.33746442224576));
#97344=CARTESIAN_POINT('Ctrl Pts',(-10.2781717815971,16.0188955734774,2.35512171145559));
#97345=CARTESIAN_POINT('Ctrl Pts',(-10.3092744674143,16.0209337320896,2.36312933802495));
#97346=CARTESIAN_POINT('Ctrl Pts',(-10.3601775249149,16.0243700859389,2.37847829188075));
#97347=CARTESIAN_POINT('Ctrl Pts',(-10.3801776063132,16.0257466106985,2.38509924653422));
#97348=CARTESIAN_POINT('Ctrl Pts',(-10.4071958585967,16.0276476315504,2.39485507065346));
#97349=CARTESIAN_POINT('Ctrl Pts',(-10.4143775518253,16.0281569906098,2.39752776813885));
#97350=CARTESIAN_POINT('Ctrl Pts',(-10.4264055923121,16.0290171492364,2.40213818300635));
#97351=CARTESIAN_POINT('Ctrl Pts',(-10.4312661338857,16.0293666989009,2.40403840458048));
#97352=CARTESIAN_POINT('Ctrl Pts',(-10.4408435141628,16.0300594211834,2.40785624422752));
#97353=CARTESIAN_POINT('Ctrl Pts',(-10.4455608671857,16.030402534406,2.40977227173452));
#97354=CARTESIAN_POINT('Ctrl Pts',(-10.4569941187558,16.0312388596365,2.41450266651829));
#97355=CARTESIAN_POINT('Ctrl Pts',(-10.4636965554463,16.0317331304739,2.41734881614791));
#97356=CARTESIAN_POINT('Ctrl Pts',(-10.4826559440417,16.0331429095534,2.42560815684214));
#97357=CARTESIAN_POINT('Ctrl Pts',(-10.4948471717376,16.0340633450591,2.43116846798682));
#97358=CARTESIAN_POINT('Ctrl Pts',(-10.5843742428374,16.0409288710067,2.47386097513836));
#97359=CARTESIAN_POINT('Ctrl Pts',(-10.6575276511688,16.0471602678752,2.51912964463413));
#97360=CARTESIAN_POINT('Ctrl Pts',(-10.7815667375091,16.0587176951414,2.61604153736333));
#97361=CARTESIAN_POINT('Ctrl Pts',(-10.8338917785618,16.0639920374312,2.6652210792401));
#97362=CARTESIAN_POINT('Ctrl Pts',(-10.8862120951529,16.0694832877704,2.72425824640106));
#97363=CARTESIAN_POINT('Ctrl Pts',(-10.8909490987023,16.0699825662486,2.72970339743013));
#97364=CARTESIAN_POINT('Ctrl Pts',(-10.8979287029348,16.0707209479235,2.7378769304044));
#97365=CARTESIAN_POINT('Ctrl Pts',(-10.9002094624161,16.0709626764705,2.74057228562283));
#97366=CARTESIAN_POINT('Ctrl Pts',(-10.9040988093348,16.0713755976844,2.7452107789829));
#97367=CARTESIAN_POINT('Ctrl Pts',(-10.9057133090767,16.071547213126,2.74714886769814));
#97368=CARTESIAN_POINT('Ctrl Pts',(-10.9093665185266,16.0719360022265,2.75156303925267));
#97369=CARTESIAN_POINT('Ctrl Pts',(-10.9114013482751,16.0721528972581,2.75404227183201));
#97370=CARTESIAN_POINT('Ctrl Pts',(-10.9169101267477,16.0727411130499,2.76081034666278));
#97371=CARTESIAN_POINT('Ctrl Pts',(-10.9203641506507,16.073111051132,2.76511541225862));
#97372=CARTESIAN_POINT('Ctrl Pts',(-10.9373683627061,16.0749388049652,2.78661725459034));
#97373=CARTESIAN_POINT('Ctrl Pts',(-10.9504684471702,16.0763678399686,2.80416649384458));
#97374=CARTESIAN_POINT('Ctrl Pts',(-10.9757770783032,16.0791949541197,2.84012024148955));
#97375=CARTESIAN_POINT('Ctrl Pts',(-10.9879723691913,16.0805921245025,2.85852287862174));
#97376=CARTESIAN_POINT('Ctrl Pts',(-11.0522376619671,16.0882163907024,2.96168346345309));
#97377=CARTESIAN_POINT('Ctrl Pts',(-11.0939233510033,16.094207179116,3.05242768150119));
#97378=CARTESIAN_POINT('Ctrl Pts',(-11.1319664499123,16.1023495501806,3.17364509011271));
#97379=CARTESIAN_POINT('Ctrl Pts',(-11.1392969674781,16.1041409095899,3.20023709407712));
#97380=CARTESIAN_POINT('Ctrl Pts',(-11.1476450808248,16.1065201767902,3.23527899252488));
#97381=CARTESIAN_POINT('Ctrl Pts',(-11.1495145066207,16.1070809165594,3.24351835109228));
#97382=CARTESIAN_POINT('Ctrl Pts',(-11.1524301602058,16.1080037117448,3.25704158123248));
#97383=CARTESIAN_POINT('Ctrl Pts',(-11.1535290946224,16.1083640886026,3.26231387583481));
#97384=CARTESIAN_POINT('Ctrl Pts',(-11.1555885514673,16.1090646916328,3.27254522258486));
#97385=CARTESIAN_POINT('Ctrl Pts',(-11.1565534093225,16.1094047721667,3.27750328976581));
#97386=CARTESIAN_POINT('Ctrl Pts',(-11.1587141358635,16.1101947746593,3.28900046672267));
#97387=CARTESIAN_POINT('Ctrl Pts',(-11.1598865847367,16.1106454242749,3.29554374773423));
#97388=CARTESIAN_POINT('Ctrl Pts',(-11.1635291675291,16.1121207675244,3.31691300770058));
#97389=CARTESIAN_POINT('Ctrl Pts',(-11.165770810196,16.1131525610158,3.33177588709594));
#97390=CARTESIAN_POINT('Ctrl Pts',(-11.1783439126348,16.1198394444715,3.42753423208055));
#97391=CARTESIAN_POINT('Ctrl Pts',(-11.1805317880148,16.1257488657217,3.50926088729189));
#97392=CARTESIAN_POINT('Ctrl Pts',(-11.1700811702948,16.1357255743591,3.64479689409002));
#97393=CARTESIAN_POINT('Ctrl Pts',(-11.1621426596776,16.1397340630886,3.69869850937178));
#97394=CARTESIAN_POINT('Ctrl Pts',(-11.1470621793525,16.1447899698767,3.7675866089842));
#97395=CARTESIAN_POINT('Ctrl Pts',(-11.143297178715,16.145934055025,3.78324168552712));
#97396=CARTESIAN_POINT('Ctrl Pts',(-11.1364835253495,16.1478191321952,3.80921824525672));
#97397=CARTESIAN_POINT('Ctrl Pts',(-11.133612380222,16.1485677494038,3.81958366444777));
#97398=CARTESIAN_POINT('Ctrl Pts',(-11.1294388211204,16.1495944109884,3.83388647983951));
#97399=CARTESIAN_POINT('Ctrl Pts',(-11.1282571136758,16.1498788172146,3.83785813416692));
#97400=CARTESIAN_POINT('Ctrl Pts',(-11.1262195250046,16.1503586570704,3.8445764349187));
#97401=CARTESIAN_POINT('Ctrl Pts',(-11.1253745036843,16.1505547039314,3.84732630930728));
#97402=CARTESIAN_POINT('Ctrl Pts',(-11.1237332759864,16.150929842244,3.85259832898702));
#97403=CARTESIAN_POINT('Ctrl Pts',(-11.1229386420303,16.1511090262942,3.8551209142694));
#97404=CARTESIAN_POINT('Ctrl Pts',(-11.121011483844,16.1515378255512,3.86116757457415));
#97405=CARTESIAN_POINT('Ctrl Pts',(-11.1198708213881,16.151786974285,3.86468905681593));
#97406=CARTESIAN_POINT('Ctrl Pts',(-11.1156603241457,16.1526901688692,3.87748176270571));
#97407=CARTESIAN_POINT('Ctrl Pts',(-11.1124917019643,16.1533387912383,3.8867204008253));
#97408=CARTESIAN_POINT('Ctrl Pts',(-11.0888520214821,16.1579694826666,3.95294944607229));
#97409=CARTESIAN_POINT('Ctrl Pts',(-11.0641247160084,16.1617421454723,4.0083330126374));
#97410=CARTESIAN_POINT('Ctrl Pts',(-11.0103106359171,16.1687304137825,4.10753740695604));
#97411=CARTESIAN_POINT('Ctrl Pts',(-10.9823448350934,16.1719441137074,4.15178808421861));
#97412=CARTESIAN_POINT('Ctrl Pts',(-10.9326821906513,16.1772348495155,4.2198765342117));
#97413=CARTESIAN_POINT('Ctrl Pts',(-10.9127882786581,16.1792658194929,4.24494000853302));
#97414=CARTESIAN_POINT('Ctrl Pts',(-10.878179474341,16.1826912328201,4.28507149849349));
#97415=CARTESIAN_POINT('Ctrl Pts',(-10.8640363677881,16.1840641907022,4.30061071307899));
#97416=CARTESIAN_POINT('Ctrl Pts',(-10.8441835819076,16.1859610568706,4.32128420480624));
#97417=CARTESIAN_POINT('Ctrl Pts',(-10.8388276255506,16.1864699158548,4.32675381766051));
#97418=CARTESIAN_POINT('Ctrl Pts',(-10.8297324574212,16.1873294691158,4.33586262694271));
#97419=CARTESIAN_POINT('Ctrl Pts',(-10.8260216427965,16.1876789174567,4.3395299435722));
#97420=CARTESIAN_POINT('Ctrl Pts',(-10.8186405311911,16.1883716263678,4.34672822138231));
#97421=CARTESIAN_POINT('Ctrl Pts',(-10.8149714523703,16.1887148286992,4.35026027227464));
#97422=CARTESIAN_POINT('Ctrl Pts',(-10.805996154168,16.1895517027643,4.35878890472202));
#97423=CARTESIAN_POINT('Ctrl Pts',(-10.8006662949916,16.1900464366609,4.36376018854541));
#97424=CARTESIAN_POINT('Ctrl Pts',(-10.7853895098545,16.1914584102911,4.37774630951553));
#97425=CARTESIAN_POINT('Ctrl Pts',(-10.7753343968011,16.1923805996083,4.38664074646383));
#97426=CARTESIAN_POINT('Ctrl Pts',(-10.7004023843767,16.1992034854541,4.45067381455465));
#97427=CARTESIAN_POINT('Ctrl Pts',(-10.6298796753538,16.2053857323667,4.49879458241126));
#97428=CARTESIAN_POINT('Ctrl Pts',(-10.5157505747271,16.214885050189,4.55974358664123));
#97429=CARTESIAN_POINT('Ctrl Pts',(-10.4755515643365,16.2181406035232,4.57838125565397));
#97430=CARTESIAN_POINT('Ctrl Pts',(-10.4063321908636,16.2235156770109,4.60584849291678));
#97431=CARTESIAN_POINT('Ctrl Pts',(-10.3778462985437,16.22566487498,4.61590289523009));
#97432=CARTESIAN_POINT('Ctrl Pts',(-10.3434039232958,16.2281653776134,4.6265891767042));
#97433=CARTESIAN_POINT('Ctrl Pts',(-10.3377920052598,16.2285697349649,4.62828453519778));
#97434=CARTESIAN_POINT('Ctrl Pts',(-10.3290493868186,16.2291946674267,4.63085460006933));
#97435=CARTESIAN_POINT('Ctrl Pts',(-10.3259274266984,16.2294168418209,4.63175833932777));
#97436=CARTESIAN_POINT('Ctrl Pts',(-10.320112123416,16.2298288029068,4.63341568386164));
#97437=CARTESIAN_POINT('Ctrl Pts',(-10.3174198541804,16.2300187701505,4.63417261490602));
#97438=CARTESIAN_POINT('Ctrl Pts',(-10.311236126593,16.2304533901902,4.63588742531048));
#97439=CARTESIAN_POINT('Ctrl Pts',(-10.3077429278617,16.2306976693299,4.63683880154835));
#97440=CARTESIAN_POINT('Ctrl Pts',(-10.2985232293794,16.231339277372,4.63930418581432));
#97441=CARTESIAN_POINT('Ctrl Pts',(-10.2927895116566,16.2317351236611,4.64079115167677));
#97442=CARTESIAN_POINT('Ctrl Pts',(-10.2479922378394,16.2348049499646,4.65204874816163));
#97443=CARTESIAN_POINT('Ctrl Pts',(-10.2084574287688,16.2373790340174,4.65985461624273));
#97444=CARTESIAN_POINT('Ctrl Pts',(-10.0727546103486,16.2459952586544,4.67948276372478));
#97445=CARTESIAN_POINT('Ctrl Pts',(-9.97557150159121,16.2518276129777,4.68147232377816));
#97446=CARTESIAN_POINT('Ctrl Pts',(-9.84797169967027,16.2600117410299,4.66831951699021));
#97447=CARTESIAN_POINT('Ctrl Pts',(-9.81684836518294,16.2620468129897,4.66384633915313));
#97448=CARTESIAN_POINT('Ctrl Pts',(-9.77726026334366,16.2647035082044,4.65652930816957));
#97449=CARTESIAN_POINT('Ctrl Pts',(-9.76859588091271,16.2652891528382,4.65482689506701));
#97450=CARTESIAN_POINT('Ctrl Pts',(-9.75459766416253,16.266242492794,4.65191261113007));
#97451=CARTESIAN_POINT('Ctrl Pts',(-9.74925158365039,16.2666082859979,4.65076070496727));
#97452=CARTESIAN_POINT('Ctrl Pts',(-9.73901245936488,16.2673122324694,4.6484797696836));
#97453=CARTESIAN_POINT('Ctrl Pts',(-9.73411822306649,16.2676501926585,4.64735659543492));
#97454=CARTESIAN_POINT('Ctrl Pts',(-9.72294748559648,16.2684250184578,4.64471771967401));
#97455=CARTESIAN_POINT('Ctrl Pts',(-9.71667601261238,16.2688625252691,4.6431816429413));
#97456=CARTESIAN_POINT('Ctrl Pts',(-9.69687841022296,16.2702517525231,4.63815968520796));
#97457=CARTESIAN_POINT('Ctrl Pts',(-9.68340192795734,16.2712094699663,4.63448481645923));
#97458=CARTESIAN_POINT('Ctrl Pts',(-9.57622341298217,16.2789261701173,4.60320018852827));
#97459=CARTESIAN_POINT('Ctrl Pts',(-9.48623922667448,16.2860672923297,4.56427416158616));
#97460=CARTESIAN_POINT('Ctrl Pts',(-9.34955970974919,16.2977113381803,4.48373932751434));
#97461=CARTESIAN_POINT('Ctrl Pts',(-9.2994859919604,16.3021688878292,4.44873468758854));
#97462=CARTESIAN_POINT('Ctrl Pts',(-9.24669884863713,16.3069257639448,4.40536503090052));
#97463=CARTESIAN_POINT('Ctrl Pts',(-9.24109563625759,16.3074314118141,4.4006734354316));
#97464=CARTESIAN_POINT('Ctrl Pts',(-9.23283679958694,16.3081773297637,4.39362647629217));
#97465=CARTESIAN_POINT('Ctrl Pts',(-9.23014769754052,16.3084203019459,4.3913108820338));
#97466=CARTESIAN_POINT('Ctrl Pts',(-9.22536242867823,16.3088527859221,4.38715245862571));
#97467=CARTESIAN_POINT('Ctrl Pts',(-9.22326231131236,16.3090426262816,4.38531430309483));
#97468=CARTESIAN_POINT('Ctrl Pts',(-9.21869183028347,16.3094558476884,4.38128514615377));
#97469=CARTESIAN_POINT('Ctrl Pts',(-9.21622413908398,16.3096790086034,4.37909121564128));
#97470=CARTESIAN_POINT('Ctrl Pts',(-9.2093472967844,16.3103011656198,4.37292530132507));
#97471=CARTESIAN_POINT('Ctrl Pts',(-9.20495881471525,16.3106985022221,4.36893025966334));
#97472=CARTESIAN_POINT('Ctrl Pts',(-9.18016407865495,16.3129464759562,4.34601333449227));
#97473=CARTESIAN_POINT('Ctrl Pts',(-9.16040152362958,16.3147500995326,4.32640437104746));
#97474=CARTESIAN_POINT('Ctrl Pts',(-9.07308786107419,16.3228810530056,4.23340012776656));
#97475=CARTESIAN_POINT('Ctrl Pts',(-9.01433434755161,16.3288572348687,4.15230967285393));
#97476=CARTESIAN_POINT('Ctrl Pts',(-8.94705074494222,16.3377250535337,4.02918625624462));
#97477=CARTESIAN_POINT('Ctrl Pts',(-8.92945381013598,16.3403315303219,3.99261600887378));
#97478=CARTESIAN_POINT('Ctrl Pts',(-8.91008861238699,16.343632572551,3.94640722097116));
#97479=CARTESIAN_POINT('Ctrl Pts',(-8.90650526802961,16.3442651225191,3.93755628446393));
#97480=CARTESIAN_POINT('Ctrl Pts',(-8.90098227911052,16.345276087643,3.92342267952988));
#97481=CARTESIAN_POINT('Ctrl Pts',(-8.89897213910695,16.3456521501793,3.91816786586369));
#97482=CARTESIAN_POINT('Ctrl Pts',(-8.89525142569963,16.3463639176573,3.90822851383324));
#97483=CARTESIAN_POINT('Ctrl Pts',(-8.89353280024487,16.3466993468808,3.90354710564479));
#97484=CARTESIAN_POINT('Ctrl Pts',(-8.88971831324223,16.3474592008359,3.89294915177128));
#97485=CARTESIAN_POINT('Ctrl Pts',(-8.88763992847873,16.3478841901918,3.88702652165376));
#97486=CARTESIAN_POINT('Ctrl Pts',(-8.88241478252164,16.3489816342205,3.87174695175587));
#97487=CARTESIAN_POINT('Ctrl Pts',(-8.87933819909121,16.3496563540756,3.86236670944295));
#97488=CARTESIAN_POINT('Ctrl Pts',(-8.85643098424019,16.3549107463391,3.7894411739625));
#97489=CARTESIAN_POINT('Ctrl Pts',(-8.84190555417357,16.3596617099307,3.72436748884922));
#97490=CARTESIAN_POINT('Ctrl Pts',(-8.83208570707783,16.3649821538915,3.65202938328167));
#97491=CARTESIAN_POINT('Ctrl Pts',(-8.8312700210513,16.365453344705,3.64562611035618));
#97492=CARTESIAN_POINT('Ctrl Pts',(-8.82273383045644,16.3707317182036,3.57391755127616));
#97493=CARTESIAN_POINT('Ctrl Pts',(-8.82044311593317,16.3756014686227,3.50808180334307));
#97494=CARTESIAN_POINT('Ctrl Pts',(-8.82499438793023,16.3822979207438,3.41513618323579));
#97495=CARTESIAN_POINT('Ctrl Pts',(-8.8272767507511,16.3842352875929,3.38792631427647));
#97496=CARTESIAN_POINT('Ctrl Pts',(-8.83117710238743,16.3865226469574,3.35515303568866));
#97497=CARTESIAN_POINT('Ctrl Pts',(-8.8318924622395,16.3869160095783,3.34949288192472));
#97498=CARTESIAN_POINT('Ctrl Pts',(-8.83307535350468,16.3875276718815,3.34065046547315));
#97499=CARTESIAN_POINT('Ctrl Pts',(-8.83351482633561,16.3877474662511,3.33746463460998));
#97500=CARTESIAN_POINT('Ctrl Pts',(-8.83436162215641,16.3881573925859,3.33150642121161));
#97501=CARTESIAN_POINT('Ctrl Pts',(-8.83476578594771,16.3883476872922,3.3287337143047));
#97502=CARTESIAN_POINT('Ctrl Pts',(-8.83571357511416,16.3887820073147,3.32239023550879));
#97503=CARTESIAN_POINT('Ctrl Pts',(-8.83626373388499,16.3890256655683,3.31882049945662));
#97504=CARTESIAN_POINT('Ctrl Pts',(-8.83777552325451,16.3896734803508,3.30930223752508));
#97505=CARTESIAN_POINT('Ctrl Pts',(-8.8387664126618,16.3900760692815,3.303358370721));
#97506=CARTESIAN_POINT('Ctrl Pts',(-8.8478453478716,16.3935828563476,3.25136177888419));
#97507=CARTESIAN_POINT('Ctrl Pts',(-8.85862469037331,16.3965518524802,3.20581496961919));
#97508=CARTESIAN_POINT('Ctrl Pts',(-8.89191910443324,16.4037818806706,3.09503036160322));
#97509=CARTESIAN_POINT('Ctrl Pts',(-8.91750609203828,16.407980916882,3.030904204702));
#97510=CARTESIAN_POINT('Ctrl Pts',(-8.96354710870661,16.4143869389582,2.9396715097105));
#97511=CARTESIAN_POINT('Ctrl Pts',(-8.97979241931128,16.4164967461762,2.91061146398605));
#97512=CARTESIAN_POINT('Ctrl Pts',(-9.0048620471992,16.4195837411277,2.86991555773456));
#97513=CARTESIAN_POINT('Ctrl Pts',(-9.01270644770618,16.4205287454575,2.85769371584797));
#97514=CARTESIAN_POINT('Ctrl Pts',(-9.02716639027976,16.4222366843771,2.83605559575335));
#97515=CARTESIAN_POINT('Ctrl Pts',(-9.03369781929854,16.4229965531211,2.82658520628969));
#97516=CARTESIAN_POINT('Ctrl Pts',(-9.04387015332391,16.4241635237356,2.81228836156548));
#97517=CARTESIAN_POINT('Ctrl Pts',(-9.04741135321145,16.4245668478608,2.80739156152264));
#97518=CARTESIAN_POINT('Ctrl Pts',(-9.05364826772389,16.4252722753384,2.79890542047901));
#97519=CARTESIAN_POINT('Ctrl Pts',(-9.05632713247397,16.4255737260021,2.7953038039316));
#97520=CARTESIAN_POINT('Ctrl Pts',(-9.0624078464814,16.4262545891716,2.78722540036863));
#97521=CARTESIAN_POINT('Ctrl Pts',(-9.06582127797874,16.426634447486,2.78275750987397));
#97522=CARTESIAN_POINT('Ctrl Pts',(-9.07510762337179,16.4276617083086,2.77078122636609));
#97523=CARTESIAN_POINT('Ctrl Pts',(-9.08103981209053,16.4283114297584,2.76331954560225));
#97524=CARTESIAN_POINT('Ctrl Pts',(-9.10929080948203,16.4313763221343,2.72865688474996));
#97525=CARTESIAN_POINT('Ctrl Pts',(-9.13272863742849,16.4338360162314,2.70239546192801));
#97526=CARTESIAN_POINT('Ctrl Pts',(-9.21289066595661,16.4419967215126,2.62029265697193));
#97527=CARTESIAN_POINT('Ctrl Pts',(-9.27409832693256,16.4478674125842,2.5691454845482));
#97528=CARTESIAN_POINT('Ctrl Pts',(-9.37961365346763,16.4571966177346,2.49774981730174));
#97529=CARTESIAN_POINT('Ctrl Pts',(-9.42084540212068,16.4606707835839,2.47337174494598));
#97530=CARTESIAN_POINT('Ctrl Pts',(-9.47198862096057,16.4646933608285,2.4471984774303));
#97531=CARTESIAN_POINT('Ctrl Pts',(-9.48058051179468,16.4653597867481,2.44293308044216));
#97532=CARTESIAN_POINT('Ctrl Pts',(-9.49279198696394,16.466292855256,2.43705561077228));
#97533=CARTESIAN_POINT('Ctrl Pts',(-9.49636878467829,16.4665644634172,2.43535623649025));
#97534=CARTESIAN_POINT('Ctrl Pts',(-9.50252832256023,16.4670292099546,2.4324677633927));
#97535=CARTESIAN_POINT('Ctrl Pts',(-9.505106902609,16.4672228730952,2.43126992700627));
#97536=CARTESIAN_POINT('Ctrl Pts',(-9.51048228042158,16.4676246990225,2.42879651173683));
#97537=CARTESIAN_POINT('Ctrl Pts',(-9.51327975695162,16.4678327657488,2.42752253328754));
#97538=CARTESIAN_POINT('Ctrl Pts',(-9.52069575729485,16.4683816437886,2.42418025984194));
#97539=CARTESIAN_POINT('Ctrl Pts',(-9.52532274187637,16.4687213404432,2.42213072530875));
#97540=CARTESIAN_POINT('Ctrl Pts',(-9.54516890525096,16.4701672103479,2.41349239913891));
#97541=CARTESIAN_POINT('Ctrl Pts',(-9.56051397076029,16.4712572096055,2.40719526437053));
#97542=CARTESIAN_POINT('Ctrl Pts',(-9.65201486779166,16.4776221027912,2.37188552873384));
#97543=CARTESIAN_POINT('Ctrl Pts',(-9.73081204459537,16.4825706016215,2.35054363630281));
#97544=CARTESIAN_POINT('Ctrl Pts',(-9.81110406371068,16.4876146309988,2.3374969300026));
#97545=CARTESIAN_POINT('Origin',(-10.,12.3756328852638,3.5));
#97546=CARTESIAN_POINT('',(-9.81110406370895,17.0855891663962,2.33749693000288));
#97547=CARTESIAN_POINT('',(-9.81110406885758,16.9868193101849,2.33749692916628));
#97548=CARTESIAN_POINT('',(-9.81110406371068,12.3756328852638,2.3374969300026));
#97549=CARTESIAN_POINT('Ctrl Pts',(-9.81110406370722,17.0855891663962,2.33749693000316));
#97550=CARTESIAN_POINT('Ctrl Pts',(-9.81046679021848,17.0855476087213,2.33760048101772));
#97551=CARTESIAN_POINT('Ctrl Pts',(-9.80982959701639,17.0855060696787,2.3377045568435));
#97552=CARTESIAN_POINT('Ctrl Pts',(-9.76283177728797,17.0824432182907,2.34542061936591));
#97553=CARTESIAN_POINT('Ctrl Pts',(-9.71696418175036,17.0795222872894,2.35579995459459));
#97554=CARTESIAN_POINT('Ctrl Pts',(-9.58354864230442,17.0709238242386,2.39450729211066));
#97555=CARTESIAN_POINT('Ctrl Pts',(-9.49857442148061,17.0652861251475,2.43036640670373));
#97556=CARTESIAN_POINT('Ctrl Pts',(-9.40726731086784,17.0584326538379,2.48219159926921));
#97557=CARTESIAN_POINT('Ctrl Pts',(-9.39600613613032,17.0575730746573,2.4888336577192));
#97558=CARTESIAN_POINT('Ctrl Pts',(-9.37933497045112,17.056277664753,2.49904448959465));
#97559=CARTESIAN_POINT('Ctrl Pts',(-9.37383982298063,17.0558468810358,2.50247283614688));
#97560=CARTESIAN_POINT('Ctrl Pts',(-9.36439534825505,17.0550997654432,2.50847390233251));
#97561=CARTESIAN_POINT('Ctrl Pts',(-9.36043263155815,17.0547842168966,2.51102535128617));
#97562=CARTESIAN_POINT('Ctrl Pts',(-9.35224138241517,17.0541275732871,2.51636921902322));
#97563=CARTESIAN_POINT('Ctrl Pts',(-9.34801535146255,17.0537863481409,2.51916527558025));
#97564=CARTESIAN_POINT('Ctrl Pts',(-9.33811450053976,17.0529810539607,2.52580820714844));
#97565=CARTESIAN_POINT('Ctrl Pts',(-9.33245501695078,17.0525161531781,2.52967749907337));
#97566=CARTESIAN_POINT('Ctrl Pts',(-9.31386648797026,17.0509737389932,2.54262575233408));
#97567=CARTESIAN_POINT('Ctrl Pts',(-9.30108681563627,17.0498883142975,2.55191510667831));
#97568=CARTESIAN_POINT('Ctrl Pts',(-9.27111397333765,17.0472809548921,2.57463730049556));
#97569=CARTESIAN_POINT('Ctrl Pts',(-9.25410012807943,17.0457507143835,2.58829596837442));
#97570=CARTESIAN_POINT('Ctrl Pts',(-9.18893916043329,17.0396886509674,2.64365225908095));
#97571=CARTESIAN_POINT('Ctrl Pts',(-9.14383180479926,17.035036225825,2.68875068801303));
#97572=CARTESIAN_POINT('Ctrl Pts',(-9.05948926780255,17.0254733597546,2.78798524486116));
#97573=CARTESIAN_POINT('Ctrl Pts',(-9.02075587557147,17.0205783027184,2.84227048072301));
#97574=CARTESIAN_POINT('Ctrl Pts',(-8.98186453342811,17.0152333760837,2.90789402753671));
#97575=CARTESIAN_POINT('Ctrl Pts',(-8.97701822646156,17.0145583836961,2.91630691522565));
#97576=CARTESIAN_POINT('Ctrl Pts',(-8.97047167186255,17.0136349384507,2.92800337698872));
#97577=CARTESIAN_POINT('Ctrl Pts',(-8.9686821850994,17.0133812685793,2.93123618190912));
#97578=CARTESIAN_POINT('Ctrl Pts',(-8.96563854419849,17.0129477247704,2.93679628045461));
#97579=CARTESIAN_POINT('Ctrl Pts',(-8.96437697117387,17.0127673940706,2.93911944812095));
#97580=CARTESIAN_POINT('Ctrl Pts',(-8.96175755669441,17.0123916803676,2.94398202955287));
#97581=CARTESIAN_POINT('Ctrl Pts',(-8.96040119252868,17.0121963969138,2.94652220072547));
#97582=CARTESIAN_POINT('Ctrl Pts',(-8.95711069943527,17.0117207792727,2.95273934015649));
#97583=CARTESIAN_POINT('Ctrl Pts',(-8.95518665920033,17.0114410703212,2.95642166411791));
#97584=CARTESIAN_POINT('Ctrl Pts',(-8.94832139200565,17.0104369100489,2.96973188175211));
#97585=CARTESIAN_POINT('Ctrl Pts',(-8.94349324999972,17.0097190837273,2.97941794156666));
#97586=CARTESIAN_POINT('Ctrl Pts',(-8.93175853462316,17.0079411016092,3.00379568119295));
#97587=CARTESIAN_POINT('Ctrl Pts',(-8.92502073140274,17.0068893812309,3.01856653462524));
#97588=CARTESIAN_POINT('Ctrl Pts',(-8.89671119883383,17.002308366018,3.08418800896803));
#97589=CARTESIAN_POINT('Ctrl Pts',(-8.87842523642352,16.9989003530262,3.13638370946908));
#97590=CARTESIAN_POINT('Ctrl Pts',(-8.84267024961867,16.990512187509,3.26728570992747));
#97591=CARTESIAN_POINT('Ctrl Pts',(-8.82948182836423,16.9855344942284,3.34685557577684));
#97592=CARTESIAN_POINT('Ctrl Pts',(-8.82357408891377,16.9793060239926,3.44217351806597));
#97593=CARTESIAN_POINT('Ctrl Pts',(-8.82293092809327,16.9783157737234,3.45721924953858));
#97594=CARTESIAN_POINT('Ctrl Pts',(-8.82241978420988,16.9768751352034,3.47892462630338));
#97595=CARTESIAN_POINT('Ctrl Pts',(-8.82231951261462,16.9764319237513,3.48557770572016));
#97596=CARTESIAN_POINT('Ctrl Pts',(-8.82224228858446,16.975649015259,3.49728455976286));
#97597=CARTESIAN_POINT('Ctrl Pts',(-8.82224147951256,16.9753100655643,3.50233804850006));
#97598=CARTESIAN_POINT('Ctrl Pts',(-8.82230699423253,16.9746077711272,3.51277711070213));
#97599=CARTESIAN_POINT('Ctrl Pts',(-8.82237773827805,16.9742442972441,3.51816252793057));
#97600=CARTESIAN_POINT('Ctrl Pts',(-8.8226542492298,16.9733079671012,3.53198989425409));
#97601=CARTESIAN_POINT('Ctrl Pts',(-8.82291387249395,16.9727334559864,3.54043033705297));
#97602=CARTESIAN_POINT('Ctrl Pts',(-8.82440608436641,16.9702745261167,3.57636330928275));
#97603=CARTESIAN_POINT('Ctrl Pts',(-8.82651122632238,16.9683634285255,3.60380890524678));
#97604=CARTESIAN_POINT('Ctrl Pts',(-8.84066218104489,16.9594105224648,3.73009297141684));
#97605=CARTESIAN_POINT('Ctrl Pts',(-8.86424927016994,16.9520245324512,3.82721748329565));
#97606=CARTESIAN_POINT('Ctrl Pts',(-8.90764195769683,16.9431596191998,3.94083688415836));
#97607=CARTESIAN_POINT('Ctrl Pts',(-8.91610465512185,16.9415595501064,3.96125288742253));
#97608=CARTESIAN_POINT('Ctrl Pts',(-8.93407343246574,16.9384152309937,4.00137167607303));
#97609=CARTESIAN_POINT('Ctrl Pts',(-8.94356427729184,16.9368711426358,4.02107266131937));
#97610=CARTESIAN_POINT('Ctrl Pts',(-8.95613105673537,16.9349741272279,4.04540181260195));
#97611=CARTESIAN_POINT('Ctrl Pts',(-8.9586977686307,16.9345937674811,4.05028644708646));
#97612=CARTESIAN_POINT('Ctrl Pts',(-8.96281074384057,16.9339955522381,4.05798189775149));
#97613=CARTESIAN_POINT('Ctrl Pts',(-8.9643342839033,16.9337763392741,4.06080466870141));
#97614=CARTESIAN_POINT('Ctrl Pts',(-8.9670769961956,16.933385973965,4.065836989529));
#97615=CARTESIAN_POINT('Ctrl Pts',(-8.96829173085685,16.9332145543318,4.06804883422881));
#97616=CARTESIAN_POINT('Ctrl Pts',(-8.97122436935443,16.9328041996942,4.07334827819133));
#97617=CARTESIAN_POINT('Ctrl Pts',(-8.97294906800792,16.9325656975155,4.07643206905023));
#97618=CARTESIAN_POINT('Ctrl Pts',(-8.97824309549261,16.9318420067423,4.08579868835872));
#97619=CARTESIAN_POINT('Ctrl Pts',(-8.98185647123968,16.9313595057719,4.09205661596405));
#97620=CARTESIAN_POINT('Ctrl Pts',(-9.01497844139211,16.9270346022845,4.1482197382639));
#97621=CARTESIAN_POINT('Ctrl Pts',(-9.04808122037493,16.9233979857228,4.19592301216969));
#97622=CARTESIAN_POINT('Ctrl Pts',(-9.14844621490731,16.9134973582773,4.31991415718598));
#97623=CARTESIAN_POINT('Ctrl Pts',(-9.22225185970603,16.9073155831472,4.39022966756044));
#97624=CARTESIAN_POINT('Ctrl Pts',(-9.31505716518735,16.8997939520322,4.4581914785933));
#97625=CARTESIAN_POINT('Ctrl Pts',(-9.32609361793744,16.8989038707488,4.46598538307242));
#97626=CARTESIAN_POINT('Ctrl Pts',(-9.3425868326372,16.89757878004,4.47721261375785));
#97627=CARTESIAN_POINT('Ctrl Pts',(-9.34794188568081,16.8971493218907,4.48079395281557));
#97628=CARTESIAN_POINT('Ctrl Pts',(-9.35751031529124,16.8963831903709,4.48708010479039));
#97629=CARTESIAN_POINT('Ctrl Pts',(-9.36171209775898,16.8960471738355,4.48980234428691));
#97630=CARTESIAN_POINT('Ctrl Pts',(-9.37059421653031,16.8953376697608,4.49547679151794));
#97631=CARTESIAN_POINT('Ctrl Pts',(-9.37527824601759,16.8949639708928,4.49842296197901));
#97632=CARTESIAN_POINT('Ctrl Pts',(-9.38773678053448,16.893971123284,4.50613716177724));
#97633=CARTESIAN_POINT('Ctrl Pts',(-9.39554607610083,16.8933499178334,4.5108480023971));
#97634=CARTESIAN_POINT('Ctrl Pts',(-9.43337190242116,16.8903457345872,4.53307081324012));
#97635=CARTESIAN_POINT('Ctrl Pts',(-9.46409612573927,16.8879190513826,4.54933755790757));
#97636=CARTESIAN_POINT('Ctrl Pts',(-9.55607265190508,16.8806880468126,4.59294025328928));
#97637=CARTESIAN_POINT('Ctrl Pts',(-9.61898898289087,16.8757757876425,4.61643119935718));
#97638=CARTESIAN_POINT('Ctrl Pts',(-9.74237087960147,16.8663704471067,4.6508479250894));
#97639=CARTESIAN_POINT('Ctrl Pts',(-9.80238121211423,16.8618953815804,4.66265732388629));
#97640=CARTESIAN_POINT('Ctrl Pts',(-9.87272857348907,16.8569321642153,4.67089374502967));
#97641=CARTESIAN_POINT('Ctrl Pts',(-9.88242924558254,16.856254027694,4.67190755239104));
#97642=CARTESIAN_POINT('Ctrl Pts',(-9.89582688899466,16.8553270924379,4.67313968492315));
#97643=CARTESIAN_POINT('Ctrl Pts',(-9.89951363945905,16.8550730245991,4.67346122631912));
#97644=CARTESIAN_POINT('Ctrl Pts',(-9.90583803991798,16.8546389787524,4.6739827870265));
#97645=CARTESIAN_POINT('Ctrl Pts',(-9.90847493173633,16.8544585416969,4.67419130519454));
#97646=CARTESIAN_POINT('Ctrl Pts',(-9.91398260215263,16.8540828085334,4.67460817051098));
#97647=CARTESIAN_POINT('Ctrl Pts',(-9.91685347022546,16.8538876109572,4.6748148797961));
#97648=CARTESIAN_POINT('Ctrl Pts',(-9.92386323218239,16.853412533073,4.67529377570485));
#97649=CARTESIAN_POINT('Ctrl Pts',(-9.92800291460935,16.8531332746362,4.67555462979052));
#97650=CARTESIAN_POINT('Ctrl Pts',(-9.94290273489976,16.8521325583753,4.67641451088555));
#97651=CARTESIAN_POINT('Ctrl Pts',(-9.95366999172257,16.8514176659999,4.67688773883022));
#97652=CARTESIAN_POINT('Ctrl Pts',(-9.98057695314446,16.8496484258148,4.67770045409712));
#97653=CARTESIAN_POINT('Ctrl Pts',(-9.99672037902721,16.848602407392,4.67785606622607));
#97654=CARTESIAN_POINT('Ctrl Pts',(-10.0675290814311,16.8440624300346,4.67708268764603));
#97655=CARTESIAN_POINT('Ctrl Pts',(-10.1220919961041,16.8406875552156,4.67267997470266));
#97656=CARTESIAN_POINT('Ctrl Pts',(-10.2564397305442,16.8322882533554,4.65235707231739));
#97657=CARTESIAN_POINT('Ctrl Pts',(-10.3352428314476,16.827267479155,4.63194447556328));
#97658=CARTESIAN_POINT('Ctrl Pts',(-10.4254097040959,16.8209915427536,4.59833868912679));
#97659=CARTESIAN_POINT('Ctrl Pts',(-10.4394011017941,16.8200024387464,4.59281651277357));
#97660=CARTESIAN_POINT('Ctrl Pts',(-10.4594208336997,16.8185631692356,4.58446843763205));
#97661=CARTESIAN_POINT('Ctrl Pts',(-10.4655373551823,16.8181201612076,4.58185685861638));
#97662=CARTESIAN_POINT('Ctrl Pts',(-10.4762614723831,16.817337490105,4.57717018392443));
#97663=CARTESIAN_POINT('Ctrl Pts',(-10.4808784859632,16.8169985729508,4.57511695902701));
#97664=CARTESIAN_POINT('Ctrl Pts',(-10.4903902274359,16.8162962267809,4.57081347975867));
#97665=CARTESIAN_POINT('Ctrl Pts',(-10.4952830060794,16.8159326678984,4.56855922897039));
#97666=CARTESIAN_POINT('Ctrl Pts',(-10.5078102857342,16.8149958658868,4.56268300979571));
#97667=CARTESIAN_POINT('Ctrl Pts',(-10.5154214733629,16.8144209646802,4.5590123530534));
#97668=CARTESIAN_POINT('Ctrl Pts',(-10.5476977342848,16.8119579816261,4.543016073541));
#97669=CARTESIAN_POINT('Ctrl Pts',(-10.571963578543,16.8100431110478,4.52990911378482));
#97670=CARTESIAN_POINT('Ctrl Pts',(-10.6815932910367,16.8010886977025,4.46562393297571));
#97671=CARTESIAN_POINT('Ctrl Pts',(-10.7607057414638,16.7937055608505,4.40461032025047));
#97672=CARTESIAN_POINT('Ctrl Pts',(-10.8468470943442,16.7848433376907,4.31880001230056));
#97673=CARTESIAN_POINT('Ctrl Pts',(-10.8620627146949,16.783242959674,4.30276486669209));
#97674=CARTESIAN_POINT('Ctrl Pts',(-10.8913974160486,16.780100245936,4.27005358770503));
#97675=CARTESIAN_POINT('Ctrl Pts',(-10.9055223159447,16.778558016823,4.25339323448425));
#97676=CARTESIAN_POINT('Ctrl Pts',(-10.9226252177633,16.7766629460656,4.23204384545968));
#97677=CARTESIAN_POINT('Ctrl Pts',(-10.9260434525632,16.7762827369521,4.22771492432781));
#97678=CARTESIAN_POINT('Ctrl Pts',(-10.9314010143762,16.7756847055555,4.22083111652511));
#97679=CARTESIAN_POINT('Ctrl Pts',(-10.9333604799095,16.7754655271546,4.21829211557647));
#97680=CARTESIAN_POINT('Ctrl Pts',(-10.936843211606,16.7750751910268,4.21374100890536));
#97681=CARTESIAN_POINT('Ctrl Pts',(-10.9383703745719,16.7749037662661,4.21173202206325));
#97682=CARTESIAN_POINT('Ctrl Pts',(-10.9420207048064,16.7744933577783,4.20689783079863));
#97683=CARTESIAN_POINT('Ctrl Pts',(-10.9441376257478,16.7742548072074,4.20406796258569));
#97684=CARTESIAN_POINT('Ctrl Pts',(-10.950546251639,16.7735308217706,4.19542012634587));
#97685=CARTESIAN_POINT('Ctrl Pts',(-10.9547972520781,16.7730480777251,4.18957199953112));
#97686=CARTESIAN_POINT('Ctrl Pts',(-10.9927246122265,16.7687143913825,4.13637187801061));
#97687=CARTESIAN_POINT('Ctrl Pts',(-11.0229123635074,16.7650701493455,4.08662043234762));
#97688=CARTESIAN_POINT('Ctrl Pts',(-11.0953357600117,16.7551725433633,3.94453164957282));
#97689=CARTESIAN_POINT('Ctrl Pts',(-11.1295103673736,16.7490002715889,3.84867333589759));
#97690=CARTESIAN_POINT('Ctrl Pts',(-11.1538597316411,16.741488557525,3.73640198469781));
#97691=CARTESIAN_POINT('Ctrl Pts',(-11.156499641678,16.7405970818425,3.72312940828241));
#97692=CARTESIAN_POINT('Ctrl Pts',(-11.1600586039224,16.7392703083143,3.70347150478398));
#97693=CARTESIAN_POINT('Ctrl Pts',(-11.1611548935878,16.7388405825096,3.69711907088149));
#97694=CARTESIAN_POINT('Ctrl Pts',(-11.1630099469832,16.7380741506288,3.68581710490591));
#97695=CARTESIAN_POINT('Ctrl Pts',(-11.1637894052295,16.7377381032681,3.68087109278601));
#97696=CARTESIAN_POINT('Ctrl Pts',(-11.1653635145414,16.7370287164568,3.67045098363258));
#97697=CARTESIAN_POINT('Ctrl Pts',(-11.1661511848225,16.7366551668167,3.66497597150673));
#97698=CARTESIAN_POINT('Ctrl Pts',(-11.1681339912614,16.735663142874,3.65046938974396));
#97699=CARTESIAN_POINT('Ctrl Pts',(-11.1692629314907,16.7350426179546,3.64142930285573));
#97700=CARTESIAN_POINT('Ctrl Pts',(-11.1741793485423,16.7320473896077,3.59796550185208));
#97701=CARTESIAN_POINT('Ctrl Pts',(-11.176551787351,16.7296292975671,3.56340224659274));
#97702=CARTESIAN_POINT('Ctrl Pts',(-11.1790266296173,16.7224374623504,3.46218243014048));
#97703=CARTESIAN_POINT('Ctrl Pts',(-11.1750002751843,16.7175572827372,3.39556595837009));
#97704=CARTESIAN_POINT('Ctrl Pts',(-11.1564527214182,16.7081410951167,3.26867812348355));
#97705=CARTESIAN_POINT('Ctrl Pts',(-11.1427664593981,16.7036231812674,3.20848829075931));
#97706=CARTESIAN_POINT('Ctrl Pts',(-11.121530290797,16.6986208585573,3.1403336121244));
#97707=CARTESIAN_POINT('Ctrl Pts',(-11.1185145966299,16.6979429912583,3.13106204269438));
#97708=CARTESIAN_POINT('Ctrl Pts',(-11.1141958876418,16.6970163546021,3.11832438148826));
#97709=CARTESIAN_POINT('Ctrl Pts',(-11.1129912463117,16.6967623206123,3.11482570131375));
#97710=CARTESIAN_POINT('Ctrl Pts',(-11.1108972591547,16.6963283174734,3.10883591948904));
#97711=CARTESIAN_POINT('Ctrl Pts',(-11.1100159830757,16.6961478894711,3.10634205717396));
#97712=CARTESIAN_POINT('Ctrl Pts',(-11.1081581261211,16.6957721580096,3.10114048197866));
#97713=CARTESIAN_POINT('Ctrl Pts',(-11.1071800108205,16.6955769531685,3.09843335362022));
#97714=CARTESIAN_POINT('Ctrl Pts',(-11.1047680207984,16.6951018295579,3.09183350012173));
#97715=CARTESIAN_POINT('Ctrl Pts',(-11.1033234665046,16.6948225329446,3.08794466273947));
#97716=CARTESIAN_POINT('Ctrl Pts',(-11.0980511117898,16.693821525215,3.07397765652204));
#97717=CARTESIAN_POINT('Ctrl Pts',(-11.0941053879199,16.6931063845762,3.06394415293198));
#97718=CARTESIAN_POINT('Ctrl Pts',(-11.0839062608045,16.6913364051416,3.03901943641439));
#97719=CARTESIAN_POINT('Ctrl Pts',(-11.077483151736,16.6902899046701,3.02419964865728));
#97720=CARTESIAN_POINT('Ctrl Pts',(-11.0479695418317,16.6857464708914,2.95976962277652));
#97721=CARTESIAN_POINT('Ctrl Pts',(-11.0217412384253,16.6823688060979,2.9116677703047));
#97722=CARTESIAN_POINT('Ctrl Pts',(-10.9485547014756,16.6739704593492,2.79720419022072));
#97723=CARTESIAN_POINT('Ctrl Pts',(-10.8979077056219,16.6689533227418,2.73355520751759));
#97724=CARTESIAN_POINT('Ctrl Pts',(-10.8305960363268,16.6626813905185,2.66487631750318));
#97725=CARTESIAN_POINT('Ctrl Pts',(-10.8198623820013,16.6616921828514,2.65433636611574));
#97726=CARTESIAN_POINT('Ctrl Pts',(-10.8040962078388,16.6602527895318,2.63943705231074));
#97727=CARTESIAN_POINT('Ctrl Pts',(-10.7992236974778,16.6598097631011,2.63490996033136));
#97728=CARTESIAN_POINT('Ctrl Pts',(-10.7905823466195,16.6590270705259,2.62701652427092));
#97729=CARTESIAN_POINT('Ctrl Pts',(-10.7868296633359,16.6586881504307,2.62363268248148));
#97730=CARTESIAN_POINT('Ctrl Pts',(-10.7790315116823,16.657985808954,2.61669145469603));
#97731=CARTESIAN_POINT('Ctrl Pts',(-10.7749831856604,16.6576222577716,2.6131374725043));
#97732=CARTESIAN_POINT('Ctrl Pts',(-10.7645227688135,16.6566854985039,2.60408069954595));
#97733=CARTESIAN_POINT('Ctrl Pts',(-10.7580756756847,16.6561106326332,2.59861899264845));
#97734=CARTESIAN_POINT('Ctrl Pts',(-10.7303451661364,16.6536480170318,2.57563480681284));
#97735=CARTESIAN_POINT('Ctrl Pts',(-10.7085103513033,16.6517334885434,2.55879442505093));
#97736=CARTESIAN_POINT('Ctrl Pts',(-10.6052158020769,16.6427792121441,2.48475936452987));
#97737=CARTESIAN_POINT('Ctrl Pts',(-10.5173100439291,16.6353958169266,2.4372751558358));
#97738=CARTESIAN_POINT('Ctrl Pts',(-10.4038914296623,16.626533350247,2.39344898207655));
#97739=CARTESIAN_POINT('Ctrl Pts',(-10.3830564164077,16.6249330003137,2.38606493996355));
#97740=CARTESIAN_POINT('Ctrl Pts',(-10.3412438324976,16.6217901408474,2.37255836956875));
#97741=CARTESIAN_POINT('Ctrl Pts',(-10.3202782676314,16.6202477429231,2.36642425760843));
#97742=CARTESIAN_POINT('Ctrl Pts',(-10.293817803174,16.6183524955878,2.35947530284271));
#97743=CARTESIAN_POINT('Ctrl Pts',(-10.2884730176084,16.6179722727882,2.35811173602826));
#97744=CARTESIAN_POINT('Ctrl Pts',(-10.2800055976925,16.6173742246878,2.35601476684285));
#97745=CARTESIAN_POINT('Ctrl Pts',(-10.2768892923251,16.6171550431465,2.35525650522019));
#97746=CARTESIAN_POINT('Ctrl Pts',(-10.2713154406445,16.6167647043681,2.35392436438285));
#97747=CARTESIAN_POINT('Ctrl Pts',(-10.268859160078,16.6165932800741,2.35334565665642));
#97748=CARTESIAN_POINT('Ctrl Pts',(-10.2629586486451,16.6161828764827,2.35197547930999));
#97749=CARTESIAN_POINT('Ctrl Pts',(-10.2595126957486,16.6159443303115,2.35119161190009));
#97750=CARTESIAN_POINT('Ctrl Pts',(-10.2490069459777,16.6152203716675,2.34885150192244));
#97751=CARTESIAN_POINT('Ctrl Pts',(-10.2419361407016,16.6147376497243,2.34734470283849));
#97752=CARTESIAN_POINT('Ctrl Pts',(-10.1779245920784,16.6104047630613,2.33431874292132));
#97753=CARTESIAN_POINT('Ctrl Pts',(-10.120209888092,16.6067612152698,2.32696059416005));
#97754=CARTESIAN_POINT('Ctrl Pts',(-9.9781878657002,16.5979348116902,2.31945190491373));
#97755=CARTESIAN_POINT('Ctrl Pts',(-9.89401868714965,16.5928065599172,2.32402407489297));
#97756=CARTESIAN_POINT('Ctrl Pts',(-9.81110406371068,16.5874147438851,2.3374969300026));
#97757=CARTESIAN_POINT('Ctrl Pts',(-9.81110406371068,16.4876146309988,2.3374969300026));
#97758=CARTESIAN_POINT('Ctrl Pts',(-9.84043589666133,16.4894572877002,2.33273077996714));
#97759=CARTESIAN_POINT('Ctrl Pts',(-9.86996731794527,16.4913110864639,2.32907162145681));
#97760=CARTESIAN_POINT('Ctrl Pts',(-9.94136912962896,16.495834756206,2.32296481369049));
#97761=CARTESIAN_POINT('Ctrl Pts',(-9.98325815175191,16.4985234875482,2.32162462695854));
#97762=CARTESIAN_POINT('Ctrl Pts',(-10.0347595407365,16.5019168373448,2.32272361916799));
#97763=CARTESIAN_POINT('Ctrl Pts',(-10.0443895711777,16.5025550401039,2.32304738438359));
#97764=CARTESIAN_POINT('Ctrl Pts',(-10.0596534743491,16.5035729508274,2.32374815934164));
#97765=CARTESIAN_POINT('Ctrl Pts',(-10.0652906150367,16.503950249227,2.32404759307271));
#97766=CARTESIAN_POINT('Ctrl Pts',(-10.0759004530038,16.5046630559957,2.32468769003998));
#97767=CARTESIAN_POINT('Ctrl Pts',(-10.0808735804975,16.5049982791467,2.32501941829976));
#97768=CARTESIAN_POINT('Ctrl Pts',(-10.0920751269581,16.5057559155183,2.32583805931086));
#97769=CARTESIAN_POINT('Ctrl Pts',(-10.0983020379568,16.5061788799648,2.32634298081222));
#97770=CARTESIAN_POINT('Ctrl Pts',(-10.114260630331,16.5072676169004,2.32776490627188));
#97771=CARTESIAN_POINT('Ctrl Pts',(-10.1239852845258,16.5079355945176,2.32875355035896));
#97772=CARTESIAN_POINT('Ctrl Pts',(-10.1934017033005,16.512737310385,2.33668485764861));
#97773=CARTESIAN_POINT('Ctrl Pts',(-10.2524877164907,16.5170091118756,2.34806501320835));
#97774=CARTESIAN_POINT('Ctrl Pts',(-10.3850973391729,16.5269918437485,2.38430065558665));
#97775=CARTESIAN_POINT('Ctrl Pts',(-10.4575594063496,16.5327444414498,2.4120091898609));
#97776=CARTESIAN_POINT('Ctrl Pts',(-10.5524051297034,16.5403865383794,2.45944025397595));
#97777=CARTESIAN_POINT('Ctrl Pts',(-10.5775579129523,16.5424229763872,2.47318785467457));
#97778=CARTESIAN_POINT('Ctrl Pts',(-10.6071548185714,16.5448103288036,2.49079659506886));
#97779=CARTESIAN_POINT('Ctrl Pts',(-10.6121015918612,16.5452090315615,2.49378922142488));
#97780=CARTESIAN_POINT('Ctrl Pts',(-10.6197796703402,16.5458271421038,2.49851177135092));
#97781=CARTESIAN_POINT('Ctrl Pts',(-10.6225261454795,16.5460480950102,2.50021666811123));
#97782=CARTESIAN_POINT('Ctrl Pts',(-10.6276378098159,16.546459000378,2.50341900574549));
#97783=CARTESIAN_POINT('Ctrl Pts',(-10.6300046629453,16.5466491242837,2.50491355987514));
#97784=CARTESIAN_POINT('Ctrl Pts',(-10.6353918610386,16.5470815793592,2.50834224253688));
#97785=CARTESIAN_POINT('Ctrl Pts',(-10.638408717639,16.5473235551547,2.51028173952976));
#97786=CARTESIAN_POINT('Ctrl Pts',(-10.6463974175029,16.5479639096544,2.51546929501592));
#97787=CARTESIAN_POINT('Ctrl Pts',(-10.6513537111808,16.5483607772141,2.51874127929687));
#97788=CARTESIAN_POINT('Ctrl Pts',(-10.6901105517581,16.5514626688213,2.54475033682414));
#97789=CARTESIAN_POINT('Ctrl Pts',(-10.7227396030225,16.5540654437644,2.56919242355692));
#97790=CARTESIAN_POINT('Ctrl Pts',(-10.8288601498307,16.5627426212095,2.65763861017187));
#97791=CARTESIAN_POINT('Ctrl Pts',(-10.8956547703164,16.5686088564547,2.72903625055273));
#97792=CARTESIAN_POINT('Ctrl Pts',(-10.9708474196005,16.5767801744582,2.83255476962529));
#97793=CARTESIAN_POINT('Ctrl Pts',(-10.9878271183314,16.578759020161,2.85795235554662));
#97794=CARTESIAN_POINT('Ctrl Pts',(-11.008374516686,16.5813518900519,2.89143414602323));
#97795=CARTESIAN_POINT('Ctrl Pts',(-11.0128660937018,16.5819320860766,2.89893940911814));
#97796=CARTESIAN_POINT('Ctrl Pts',(-11.0200202612042,16.5828787381954,2.91120170045053));
#97797=CARTESIAN_POINT('Ctrl Pts',(-11.0227342062049,16.5832433419926,2.91592850388133));
#97798=CARTESIAN_POINT('Ctrl Pts',(-11.0278880273074,16.5839464981197,2.92505083860827));
#97799=CARTESIAN_POINT('Ctrl Pts',(-11.0303327667285,16.5842848675001,2.92944349681924));
#97800=CARTESIAN_POINT('Ctrl Pts',(-11.0358717370442,16.5850627566659,2.93954750440325));
#97801=CARTESIAN_POINT('Ctrl Pts',(-11.0389469671856,16.5855029351368,2.94526902748707));
#97802=CARTESIAN_POINT('Ctrl Pts',(-11.0485843432739,16.5869093908239,2.96356080704401));
#97803=CARTESIAN_POINT('Ctrl Pts',(-11.0549666618798,16.5878818779922,2.97622386036367));
#97804=CARTESIAN_POINT('Ctrl Pts',(-11.1026279777996,16.5954767609312,3.07519483415787));
#97805=CARTESIAN_POINT('Ctrl Pts',(-11.1334722827278,16.6024634375274,3.16611186597216));
#97806=CARTESIAN_POINT('Ctrl Pts',(-11.1657561928442,16.6140811373697,3.32103470004886));
#97807=CARTESIAN_POINT('Ctrl Pts',(-11.1736228978305,16.618662645728,3.38326441783167));
#97808=CARTESIAN_POINT('Ctrl Pts',(-11.176841670879,16.6235359481354,3.4531730027869));
#97809=CARTESIAN_POINT('Ctrl Pts',(-11.1771110000903,16.6240445759606,3.46051853164459));
#97810=CARTESIAN_POINT('Ctrl Pts',(-11.1774085988683,16.624794016462,3.47142193889978));
#97811=CARTESIAN_POINT('Ctrl Pts',(-11.1774895396561,16.6250375674893,3.4749780275111));
#97812=CARTESIAN_POINT('Ctrl Pts',(-11.1776052472068,16.625470670861,3.48132550831094));
#97813=CARTESIAN_POINT('Ctrl Pts',(-11.1776462017009,16.6256605557712,3.48411670505494));
#97814=CARTESIAN_POINT('Ctrl Pts',(-11.177713866033,16.6260733972704,3.49020343362058));
#97815=CARTESIAN_POINT('Ctrl Pts',(-11.1777366683032,16.6262961369331,3.49349894125733));
#97816=CARTESIAN_POINT('Ctrl Pts',(-11.1777617125409,16.6269159951946,3.50270069460164));
#97817=CARTESIAN_POINT('Ctrl Pts',(-11.1777333603021,16.6273114737592,3.50860702746551));
#97818=CARTESIAN_POINT('Ctrl Pts',(-11.1773231640359,16.629527998126,3.54189238095982));
#97819=CARTESIAN_POINT('Ctrl Pts',(-11.1760310104486,16.6313035554873,3.56925417175664));
#97820=CARTESIAN_POINT('Ctrl Pts',(-11.1655746513147,16.6394385320587,3.69637722184154));
#97821=CARTESIAN_POINT('Ctrl Pts',(-11.1446618696418,16.6454387494863,3.79475483951794));
#97822=CARTESIAN_POINT('Ctrl Pts',(-11.0981205948617,16.6543371382356,3.92764021201669));
#97823=CARTESIAN_POINT('Ctrl Pts',(-11.0827210179461,16.6569472637629,3.96525222866824));
#97824=CARTESIAN_POINT('Ctrl Pts',(-11.0613392000724,16.6602524023186,4.01063236985401));
#97825=CARTESIAN_POINT('Ctrl Pts',(-11.0571627239435,16.6608852082787,4.01922372921883));
#97826=CARTESIAN_POINT('Ctrl Pts',(-11.0503607636862,16.6618964879533,4.03279357365334));
#97827=CARTESIAN_POINT('Ctrl Pts',(-11.0478032444792,16.6622726064819,4.03780580603991));
#97828=CARTESIAN_POINT('Ctrl Pts',(-11.0429116364252,16.6629844206594,4.04722504442373));
#97829=CARTESIAN_POINT('Ctrl Pts',(-11.0405852762432,16.6633198401581,4.05163594170854));
#97830=CARTESIAN_POINT('Ctrl Pts',(-11.0352683129236,16.6640795917644,4.06156385487913));
#97831=CARTESIAN_POINT('Ctrl Pts',(-11.032261506308,16.6645044878793,4.06707197320762));
#97832=CARTESIAN_POINT('Ctrl Pts',(-11.0244139495824,16.665601530537,4.08117853193341));
#97833=CARTESIAN_POINT('Ctrl Pts',(-11.0195089819841,16.6662759394777,4.08974049497201));
#97834=CARTESIAN_POINT('Ctrl Pts',(-10.9762627575724,16.6721283014211,4.16307761837722));
#97835=CARTESIAN_POINT('Ctrl Pts',(-10.9319080591171,16.6775287561384,4.22408864052207));
#97836=CARTESIAN_POINT('Ctrl Pts',(-10.8460774338943,16.6870041076273,4.3210933614824));
#97837=CARTESIAN_POINT('Ctrl Pts',(-10.80734150892,16.691013295666,4.35920959846473));
#97838=CARTESIAN_POINT('Ctrl Pts',(-10.7389020235556,16.6975499478174,4.41782491283068));
#97839=CARTESIAN_POINT('Ctrl Pts',(-10.7106370145213,16.7001135197421,4.43987997120893));
#97840=CARTESIAN_POINT('Ctrl Pts',(-10.6764222394302,16.703024428143,4.46415007816418));
#97841=CARTESIAN_POINT('Ctrl Pts',(-10.6714094803625,16.7034462667085,4.46764752515646));
#97842=CARTESIAN_POINT('Ctrl Pts',(-10.6636455257224,16.7040922475084,4.47297512468929));
#97843=CARTESIAN_POINT('Ctrl Pts',(-10.6609135686236,16.7043181614104,4.47483292546186));
#97844=CARTESIAN_POINT('Ctrl Pts',(-10.6558594501519,16.7047334882933,4.47823884235012));
#97845=CARTESIAN_POINT('Ctrl Pts',(-10.6535396106521,16.7049231093215,4.47979019623933));
#97846=CARTESIAN_POINT('Ctrl Pts',(-10.6482593822422,16.7053524317024,4.483294163309));
#97847=CARTESIAN_POINT('Ctrl Pts',(-10.645295675408,16.7055917943887,4.48524166090922));
#97848=CARTESIAN_POINT('Ctrl Pts',(-10.6375664434981,16.7062119973061,4.49027082072084));
#97849=CARTESIAN_POINT('Ctrl Pts',(-10.6327872930025,16.7065915097063,4.49333152231843));
#97850=CARTESIAN_POINT('Ctrl Pts',(-10.6000213200897,16.7091678252716,4.51398331888461));
#97851=CARTESIAN_POINT('Ctrl Pts',(-10.5713239094828,16.7112975434286,4.53042573704475));
#97852=CARTESIAN_POINT('Ctrl Pts',(-10.4705912570159,16.7184815584326,4.58263686128327));
#97853=CARTESIAN_POINT('Ctrl Pts',(-10.3956095828412,16.7233510383896,4.6122288929363));
#97854=CARTESIAN_POINT('Ctrl Pts',(-10.2844127420646,16.7305767854396,4.6434314677864));
#97855=CARTESIAN_POINT('Ctrl Pts',(-10.250226579719,16.732796547896,4.65139588980909));
#97856=CARTESIAN_POINT('Ctrl Pts',(-10.2009435606005,16.7360305897609,4.66057882813239));
#97857=CARTESIAN_POINT('Ctrl Pts',(-10.1860983931109,16.7370089878418,4.66305154120646));
#97858=CARTESIAN_POINT('Ctrl Pts',(-10.1595035660592,16.738771975091,4.66695916129907));
#97859=CARTESIAN_POINT('Ctrl Pts',(-10.1477718169157,16.7395531963628,4.66850269371443));
#97860=CARTESIAN_POINT('Ctrl Pts',(-10.1299495373803,16.7407462003292,4.67057486661874));
#97861=CARTESIAN_POINT('Ctrl Pts',(-10.1238746310674,16.7411539365664,4.67123331323167));
#97862=CARTESIAN_POINT('Ctrl Pts',(-10.1128460466836,16.7418962504058,4.6723419175228));
#97863=CARTESIAN_POINT('Ctrl Pts',(-10.1078940866256,16.7422303226669,4.67280802632025));
#97864=CARTESIAN_POINT('Ctrl Pts',(-10.097218894109,16.7429522155613,4.67374465923538));
#97865=CARTESIAN_POINT('Ctrl Pts',(-10.0914948964841,16.7433403532105,4.6742047182445));
#97866=CARTESIAN_POINT('Ctrl Pts',(-10.0759729611386,16.7443958690103,4.67533808881992));
#97867=CARTESIAN_POINT('Ctrl Pts',(-10.0661697774648,16.745065730814,4.67593072254415));
#97868=CARTESIAN_POINT('Ctrl Pts',(-10.0156773620735,16.7485334004444,4.67834978092408));
#97869=CARTESIAN_POINT('Ctrl Pts',(-9.97492515181614,16.7513919045274,4.67818697706407));
#97870=CARTESIAN_POINT('Ctrl Pts',(-9.84875696090734,16.7604290230137,4.67113425632181));
#97871=CARTESIAN_POINT('Ctrl Pts',(-9.76402742689186,16.7667860483353,4.65704114812612));
#97872=CARTESIAN_POINT('Ctrl Pts',(-9.64586402103088,16.7757199871113,4.62385924378747));
#97873=CARTESIAN_POINT('Ctrl Pts',(-9.61063041148041,16.778388869124,4.61214377377987));
#97874=CARTESIAN_POINT('Ctrl Pts',(-9.56810436611026,16.7815720572614,4.5957339777677));
#97875=CARTESIAN_POINT('Ctrl Pts',(-9.56023591467436,16.7821593590126,4.59259981156679));
#97876=CARTESIAN_POINT('Ctrl Pts',(-9.54891760312958,16.7830010439651,4.58794941139286));
#97877=CARTESIAN_POINT('Ctrl Pts',(-9.54544035437241,16.7832592007512,4.58650116432355));
#97878=CARTESIAN_POINT('Ctrl Pts',(-9.53937807924722,16.7837084498256,4.58394207600493));
#97879=CARTESIAN_POINT('Ctrl Pts',(-9.53679000317385,16.7838999748353,4.58283862026243));
#97880=CARTESIAN_POINT('Ctrl Pts',(-9.53130125111625,16.7843055707512,4.58047514832467));
#97881=CARTESIAN_POINT('Ctrl Pts',(-9.5284016819795,16.784519494624,4.57921271785944));
#97882=CARTESIAN_POINT('Ctrl Pts',(-9.52050928780687,16.7851009371588,4.57573860136166));
#97883=CARTESIAN_POINT('Ctrl Pts',(-9.51552662597563,16.7854670948301,4.57350381195629));
#97884=CARTESIAN_POINT('Ctrl Pts',(-9.49192025988727,16.7871982897797,4.56271820790776));
#97885=CARTESIAN_POINT('Ctrl Pts',(-9.47350500626852,16.78853824797,4.55371635511099));
#97886=CARTESIAN_POINT('Ctrl Pts',(-9.37652852392038,16.7955871822333,4.50313409174675));
#97887=CARTESIAN_POINT('Ctrl Pts',(-9.30262321056359,16.8009512096102,4.45323843364391));
#97888=CARTESIAN_POINT('Ctrl Pts',(-9.19130394942888,16.8100801831732,4.35814506163547));
#97889=CARTESIAN_POINT('Ctrl Pts',(-9.15037786375663,16.8137242253025,4.31764488987397));
#97890=CARTESIAN_POINT('Ctrl Pts',(-9.10620050862984,16.8181402424008,4.26701471366485));
#97891=CARTESIAN_POINT('Ctrl Pts',(-9.09991553251678,16.8187810595857,4.25962954389171));
#97892=CARTESIAN_POINT('Ctrl Pts',(-9.08974772249118,16.8198392185778,4.2473784790997));
#97893=CARTESIAN_POINT('Ctrl Pts',(-9.08581091788151,16.8202543802878,4.24255782223009));
#97894=CARTESIAN_POINT('Ctrl Pts',(-9.07879191149343,16.8210046359522,4.23382255476919));
#97895=CARTESIAN_POINT('Ctrl Pts',(-9.07569596949907,16.8213391725862,4.2299191339516));
#97896=CARTESIAN_POINT('Ctrl Pts',(-9.06913554421656,16.8220559200752,4.22153895985334));
#97897=CARTESIAN_POINT('Ctrl Pts',(-9.06567839471781,16.8224384079548,4.21705665159116));
#97898=CARTESIAN_POINT('Ctrl Pts',(-9.05638107553406,16.8234802515922,4.20482097635192));
#97899=CARTESIAN_POINT('Ctrl Pts',(-9.05060433743039,16.8241420408211,4.19702019295044));
#97900=CARTESIAN_POINT('Ctrl Pts',(-9.01975020190054,16.8277574395485,4.15426018797108));
#97901=CARTESIAN_POINT('Ctrl Pts',(-8.99650928176368,16.8307794356234,4.11802235711924));
#97902=CARTESIAN_POINT('Ctrl Pts',(-8.94750430064617,16.8378998179387,4.03153369143788));
#97903=CARTESIAN_POINT('Ctrl Pts',(-8.92326595028848,16.8420336963367,3.98053936019234));
#97904=CARTESIAN_POINT('Ctrl Pts',(-8.88012923748968,16.8507498031537,3.86995620610662));
#97905=CARTESIAN_POINT('Ctrl Pts',(-8.86212419171976,16.8553203228154,3.81019081123515));
#97906=CARTESIAN_POINT('Ctrl Pts',(-8.84686642946797,16.8603719294707,3.73973592385056));
#97907=CARTESIAN_POINT('Ctrl Pts',(-8.84491901362492,16.8610506668538,3.73017010039572));
#97908=CARTESIAN_POINT('Ctrl Pts',(-8.8423975347273,16.8619782105034,3.71694536558011));
#97909=CARTESIAN_POINT('Ctrl Pts',(-8.84172151860359,16.8622322963681,3.71330663308328));
#97910=CARTESIAN_POINT('Ctrl Pts',(-8.84059186301836,16.862666326221,3.7070623775473));
#97911=CARTESIAN_POINT('Ctrl Pts',(-8.84012983193483,16.8628467295573,3.70445843069239));
#97912=CARTESIAN_POINT('Ctrl Pts',(-8.8391835026173,16.8632223363297,3.69901858817384));
#97913=CARTESIAN_POINT('Ctrl Pts',(-8.83870081937706,16.8634174415895,3.69618244661031));
#97914=CARTESIAN_POINT('Ctrl Pts',(-8.83754817426291,16.8638921973797,3.68925641595282));
#97915=CARTESIAN_POINT('Ctrl Pts',(-8.83688939002838,16.8641712274547,3.68516465215995));
#97916=CARTESIAN_POINT('Ctrl Pts',(-8.83459801107458,16.8651705799912,3.67043777438382));
#97917=CARTESIAN_POINT('Ctrl Pts',(-8.83308951231817,16.8658843590189,3.65978349334769));
#97918=CARTESIAN_POINT('Ctrl Pts',(-8.8296877337726,16.8676503795956,3.63313057419807));
#97919=CARTESIAN_POINT('Ctrl Pts',(-8.82797622954559,16.8686943290159,3.61711057081211));
#97920=CARTESIAN_POINT('Ctrl Pts',(-8.82191962565787,16.8732199551265,3.54678721659312));
#97921=CARTESIAN_POINT('Ctrl Pts',(-8.82101598256565,16.8765832986265,3.49225140884443));
#97922=CARTESIAN_POINT('Ctrl Pts',(-8.82819048612073,16.8849870554861,3.35649342437771));
#97923=CARTESIAN_POINT('Ctrl Pts',(-8.84091768949865,16.8900233507699,3.27581757618939));
#97924=CARTESIAN_POINT('Ctrl Pts',(-8.86573174455414,16.8963162697899,3.18257826540587));
#97925=CARTESIAN_POINT('Ctrl Pts',(-8.8698753834095,16.8973048175612,3.16812750880261));
#97926=CARTESIAN_POINT('Ctrl Pts',(-8.8762486775669,16.8987433335029,3.14740643521586));
#97927=CARTESIAN_POINT('Ctrl Pts',(-8.87825677158056,16.8991861528746,3.14106911104731));
#97928=CARTESIAN_POINT('Ctrl Pts',(-8.88188486925952,16.8999685120267,3.12994712394239));
#97929=CARTESIAN_POINT('Ctrl Pts',(-8.88348221883078,16.900307306665,3.12515520593022));
#97930=CARTESIAN_POINT('Ctrl Pts',(-8.88684623235489,16.9010094188268,3.11527574107535));
#97931=CARTESIAN_POINT('Ctrl Pts',(-8.8886170632032,16.9013728662555,3.11018974877852));
#97932=CARTESIAN_POINT('Ctrl Pts',(-8.89325520646379,16.9023094207647,3.09715711003194));
#97933=CARTESIAN_POINT('Ctrl Pts',(-8.89617321163529,16.9028841853108,3.08922896057814));
#97934=CARTESIAN_POINT('Ctrl Pts',(-8.90897720176546,16.9053468929679,3.05556273085136));
#97935=CARTESIAN_POINT('Ctrl Pts',(-8.91967933335675,16.9072616221675,3.03014654436327));
#97936=CARTESIAN_POINT('Ctrl Pts',(-8.97306417933406,16.916213468084,2.91485465846848));
#97937=CARTESIAN_POINT('Ctrl Pts',(-9.02613241568994,16.923593918325,2.83024762396939));
#97938=CARTESIAN_POINT('Ctrl Pts',(-9.10319044162635,16.9324533292332,2.73624889568174));
#97939=CARTESIAN_POINT('Ctrl Pts',(-9.11767511191638,16.9340532253582,2.71956036817943));
#97940=CARTESIAN_POINT('Ctrl Pts',(-9.14742101542142,16.9371985547891,2.68717604736834));
#97941=CARTESIAN_POINT('Ctrl Pts',(-9.16266798842002,16.9387437928039,2.67147784866777));
#97942=CARTESIAN_POINT('Ctrl Pts',(-9.18229786246077,16.940641927194,2.65236285832559));
#97943=CARTESIAN_POINT('Ctrl Pts',(-9.18627820868674,16.94102229843,2.6485410409044));
#97944=CARTESIAN_POINT('Ctrl Pts',(-9.19261420330395,16.9416204823678,2.64254240770005));
#97945=CARTESIAN_POINT('Ctrl Pts',(-9.1949520726629,16.9418396529201,2.64034705688068));
#97946=CARTESIAN_POINT('Ctrl Pts',(-9.19914481614963,16.9422299106679,2.63644201113584));
#97947=CARTESIAN_POINT('Ctrl Pts',(-9.2009962059884,16.9424012652229,2.63472873446189));
#97948=CARTESIAN_POINT('Ctrl Pts',(-9.20545256970721,16.9428114177326,2.63063131359555));
#97949=CARTESIAN_POINT('Ctrl Pts',(-9.20806277631253,16.9430497835293,2.62825292289423));
#97950=CARTESIAN_POINT('Ctrl Pts',(-9.21604163929868,16.9437728912032,2.62104808613208));
#97951=CARTESIAN_POINT('Ctrl Pts',(-9.22144413222486,16.9442549509091,2.61625911862514));
#97952=CARTESIAN_POINT('Ctrl Pts',(-9.27049228186356,16.948567649966,2.57357994692236));
#97953=CARTESIAN_POINT('Ctrl Pts',(-9.31683428954731,16.9521937524185,2.5388953618999));
#97954=CARTESIAN_POINT('Ctrl Pts',(-9.45128160918327,16.9620989975324,2.45292790371797));
#97955=CARTESIAN_POINT('Ctrl Pts',(-9.54375421683804,16.968294283096,2.40945444944903));
#97956=CARTESIAN_POINT('Ctrl Pts',(-9.65349650000306,16.9758299482593,2.37429485988698));
#97957=CARTESIAN_POINT('Ctrl Pts',(-9.66640171398731,16.9767179693012,2.37040321476699));
#97958=CARTESIAN_POINT('Ctrl Pts',(-9.68556230143841,16.9780404866469,2.36498220097633));
#97959=CARTESIAN_POINT('Ctrl Pts',(-9.69176829564313,16.9784694616381,2.36328117635206));
#97960=CARTESIAN_POINT('Ctrl Pts',(-9.70282470168288,16.9792349529721,2.36034788345764));
#97961=CARTESIAN_POINT('Ctrl Pts',(-9.70766965228018,16.9795708152968,2.35909550305639));
#97962=CARTESIAN_POINT('Ctrl Pts',(-9.71788932268201,16.9802802214282,2.35652317152172));
#97963=CARTESIAN_POINT('Ctrl Pts',(-9.7232656458224,16.9806539778474,2.35521015599783));
#97964=CARTESIAN_POINT('Ctrl Pts',(-9.73753456166153,16.9816475097869,2.35183176369908));
#97965=CARTESIAN_POINT('Ctrl Pts',(-9.74644210851361,16.9822693482201,2.34983184157236));
#97966=CARTESIAN_POINT('Ctrl Pts',(-9.77386598258773,16.9841891891545,2.34400868280322));
#97967=CARTESIAN_POINT('Ctrl Pts',(-9.7924487921988,16.9854976396007,2.34052823793873));
#97968=CARTESIAN_POINT('Ctrl Pts',(-9.81110407400449,16.9868193101849,2.33749692832995));
#97969=CARTESIAN_POINT('Origin',(-10.,12.3756328852638,3.5));
#97970=CARTESIAN_POINT('',(-9.81110406371068,17.5866589100326,2.3374969300026));
#97971=CARTESIAN_POINT('',(-9.81110408996512,17.4886290554142,2.3374969257365));
#97972=CARTESIAN_POINT('',(-9.81110406371068,12.3756328852638,2.3374969300026));
#97973=CARTESIAN_POINT('Ctrl Pts',(-9.81110406371068,17.5866589100326,2.3374969300026));
#97974=CARTESIAN_POINT('Ctrl Pts',(-9.78887392557191,17.585007544161,2.34110912068488));
#97975=CARTESIAN_POINT('Ctrl Pts',(-9.76673711519424,17.5833509725145,2.34536062552661));
#97976=CARTESIAN_POINT('Ctrl Pts',(-9.68809404061539,17.5774412249151,2.36282171791141));
#97977=CARTESIAN_POINT('Ctrl Pts',(-9.63246607121775,17.5732116756579,2.3795625026358));
#97978=CARTESIAN_POINT('Ctrl Pts',(-9.57154547594279,17.5686696714859,2.40292479392918));
#97979=CARTESIAN_POINT('Ctrl Pts',(-9.56482171302421,17.5681697072018,2.40557451049974));
#97980=CARTESIAN_POINT('Ctrl Pts',(-9.55484727225082,17.5674304642641,2.40961172216935));
#97981=CARTESIAN_POINT('Ctrl Pts',(-9.5515779144827,17.5671885523928,2.41095216748817));
#97982=CARTESIAN_POINT('Ctrl Pts',(-9.54598406958716,17.5667753774371,2.41327511974972));
#97983=CARTESIAN_POINT('Ctrl Pts',(-9.54365665916232,17.5666036906361,2.41425040357337));
#97984=CARTESIAN_POINT('Ctrl Pts',(-9.53837805569299,17.5662148150041,2.4164823346419));
#97985=CARTESIAN_POINT('Ctrl Pts',(-9.53542885044088,17.5659979045272,2.41774356170651));
#97986=CARTESIAN_POINT('Ctrl Pts',(-9.52742084186209,17.565409803118,2.42120695128754));
#97987=CARTESIAN_POINT('Ctrl Pts',(-9.52237222236276,17.5650399933324,2.42343267203003));
#97988=CARTESIAN_POINT('Ctrl Pts',(-9.49740275064387,17.563214842405,2.43465087312125));
#97989=CARTESIAN_POINT('Ctrl Pts',(-9.47771782335303,17.5617881799024,2.44416183391481));
#97990=CARTESIAN_POINT('Ctrl Pts',(-9.43870353075812,17.5589628781992,2.46437035237047));
#97991=CARTESIAN_POINT('Ctrl Pts',(-9.41938789454087,17.557565232559,2.47507455202477));
#97992=CARTESIAN_POINT('Ctrl Pts',(-9.31473773265837,17.5499377802119,2.53697741297212));
#97993=CARTESIAN_POINT('Ctrl Pts',(-9.23586022919132,17.5439447230707,2.59828619785502));
#97994=CARTESIAN_POINT('Ctrl Pts',(-9.1461710617582,17.5358001527505,2.68831574899577));
#97995=CARTESIAN_POINT('Ctrl Pts',(-9.12740613111295,17.5340092491634,2.70852357699786));
#97996=CARTESIAN_POINT('Ctrl Pts',(-9.10383967271742,17.5316303862701,2.73575977038211));
#97997=CARTESIAN_POINT('Ctrl Pts',(-9.09837984840599,17.5310695785164,2.74220876435746));
#97998=CARTESIAN_POINT('Ctrl Pts',(-9.08955360993892,17.5301466185398,2.7528645010714));
#97999=CARTESIAN_POINT('Ctrl Pts',(-9.08614576919978,17.529786144959,2.75703665895224));
#98000=CARTESIAN_POINT('Ctrl Pts',(-9.07959711032305,17.5290853150358,2.7651672869647));
#98001=CARTESIAN_POINT('Ctrl Pts',(-9.07645290375853,17.5287451041865,2.76912288644115));
#98002=CARTESIAN_POINT('Ctrl Pts',(-9.06922939932403,17.5279547401514,2.77833152649115));
#98003=CARTESIAN_POINT('Ctrl Pts',(-9.06516898303976,17.5275038583093,2.78359909037378));
#98004=CARTESIAN_POINT('Ctrl Pts',(-9.05207152951936,17.5260274819366,2.80089132826344));
#98005=CARTESIAN_POINT('Ctrl Pts',(-9.04322051832201,17.5249948757097,2.81305436384805));
#98006=CARTESIAN_POINT('Ctrl Pts',(-8.9881101163067,17.5183333498422,2.89191881920148));
#98007=CARTESIAN_POINT('Ctrl Pts',(-8.94862636918629,17.5124527201826,2.96307094596309));
#98008=CARTESIAN_POINT('Ctrl Pts',(-8.89530570297037,17.5024837820357,3.08800819492469));
#98009=CARTESIAN_POINT('Ctrl Pts',(-8.87736550802768,17.49845399928,3.13975132557812));
#98010=CARTESIAN_POINT('Ctrl Pts',(-8.85887135079861,17.4933741638347,3.20814190214777));
#98011=CARTESIAN_POINT('Ctrl Pts',(-8.85497735761024,17.4922266678515,3.22381356512481));
#98012=CARTESIAN_POINT('Ctrl Pts',(-8.84902314943137,17.490336533415,3.25007294813138));
#98013=CARTESIAN_POINT('Ctrl Pts',(-8.84678394812961,17.4895862221165,3.26061746048637));
#98014=CARTESIAN_POINT('Ctrl Pts',(-8.84388385806192,17.488557585768,3.27526073893597));
#98015=CARTESIAN_POINT('Ctrl Pts',(-8.84309947269726,17.4882728689747,3.27933409789126));
#98016=CARTESIAN_POINT('Ctrl Pts',(-8.84180729118898,17.4877926113087,3.28624079824013));
#98017=CARTESIAN_POINT('Ctrl Pts',(-8.84128833555495,17.4875964553139,3.28907198755132));
#98018=CARTESIAN_POINT('Ctrl Pts',(-8.84031240942297,17.4872211887882,3.29450851388123));
#98019=CARTESIAN_POINT('Ctrl Pts',(-8.83985383122251,17.4870419851224,3.29711351442347));
#98020=CARTESIAN_POINT('Ctrl Pts',(-8.83877476143978,17.4866132407057,3.303366582556));
#98021=CARTESIAN_POINT('Ctrl Pts',(-8.8381626743251,17.4863641657683,3.3070161014059));
#98022=CARTESIAN_POINT('Ctrl Pts',(-8.83600028880896,17.4854620722707,3.32029242709073));
#98023=CARTESIAN_POINT('Ctrl Pts',(-8.83455230370117,17.4848144580397,3.32993583022431));
#98024=CARTESIAN_POINT('Ctrl Pts',(-8.82489256659193,17.4801438139359,3.40020079690838));
#98025=CARTESIAN_POINT('Ctrl Pts',(-8.82129430365647,17.4763346840672,3.46137061038701));
#98026=CARTESIAN_POINT('Ctrl Pts',(-8.82374788231328,17.4684011814472,3.58949377070016));
#98027=CARTESIAN_POINT('Ctrl Pts',(-8.83073596767701,17.4642918125875,3.65620236613935));
#98028=CARTESIAN_POINT('Ctrl Pts',(-8.84989785458853,17.4578279569619,3.7560587256701));
#98029=CARTESIAN_POINT('Ctrl Pts',(-8.8579469485252,17.455585797464,3.78985424123171));
#98030=CARTESIAN_POINT('Ctrl Pts',(-8.86997909914695,17.4526946604607,3.83201049087118));
#98031=CARTESIAN_POINT('Ctrl Pts',(-8.87258331145889,17.4520902038654,3.84074888858841));
#98032=CARTESIAN_POINT('Ctrl Pts',(-8.87693042473741,17.4511136785261,3.8547399147036));
#98033=CARTESIAN_POINT('Ctrl Pts',(-8.87860937676447,17.450743687377,3.86001214744429));
#98034=CARTESIAN_POINT('Ctrl Pts',(-8.88187818201808,17.4500365918664,3.87003206533961));
#98035=CARTESIAN_POINT('Ctrl Pts',(-8.88346128517356,17.4496997144187,3.87478183812311));
#98036=CARTESIAN_POINT('Ctrl Pts',(-8.8871508347497,17.4489270229105,3.88562068277207));
#98037=CARTESIAN_POINT('Ctrl Pts',(-8.88927704474634,17.4484905687919,3.89170280747755));
#98038=CARTESIAN_POINT('Ctrl Pts',(-8.89601743838281,17.4471334798399,3.91048777856399));
#98039=CARTESIAN_POINT('Ctrl Pts',(-8.90080030547283,17.4462073274082,3.92312848849395));
#98040=CARTESIAN_POINT('Ctrl Pts',(-8.9433501107718,17.4382638215607,4.02999047314875));
#98041=CARTESIAN_POINT('Ctrl Pts',(-8.99292861335939,17.4308288532457,4.11902954823949));
#98042=CARTESIAN_POINT('Ctrl Pts',(-9.08778949001508,17.4191302342665,4.24721576570229));
#98043=CARTESIAN_POINT('Ctrl Pts',(-9.12569443611389,17.4149009197151,4.29123371856727));
#98044=CARTESIAN_POINT('Ctrl Pts',(-9.1718001265536,17.410359137448,4.33739611613007));
#98045=CARTESIAN_POINT('Ctrl Pts',(-9.17695404947359,17.409859179351,4.34246225765363));
#98046=CARTESIAN_POINT('Ctrl Pts',(-9.1846969787712,17.4091199437378,4.349934427415));
#98047=CARTESIAN_POINT('Ctrl Pts',(-9.1872505914906,17.4088780330782,4.35237664627971));
#98048=CARTESIAN_POINT('Ctrl Pts',(-9.19164672718939,17.4084648594721,4.35654329531557));
#98049=CARTESIAN_POINT('Ctrl Pts',(-9.19348383902302,17.4082931728171,4.35827333230182));
#98050=CARTESIAN_POINT('Ctrl Pts',(-9.19766869567849,17.4079042965421,4.36218897510374));
#98051=CARTESIAN_POINT('Ctrl Pts',(-9.20001981699484,17.4076873852823,4.36437090308806));
#98052=CARTESIAN_POINT('Ctrl Pts',(-9.2064392841798,17.4070992796627,4.37027977888195));
#98053=CARTESIAN_POINT('Ctrl Pts',(-9.2105250152603,17.4067294664824,4.3739878458312));
#98054=CARTESIAN_POINT('Ctrl Pts',(-9.23092461690728,17.4049042715374,4.39224202946819));
#98055=CARTESIAN_POINT('Ctrl Pts',(-9.24761632788545,17.4034775700653,4.40636181615246));
#98056=CARTESIAN_POINT('Ctrl Pts',(-9.28193884524745,17.4006522389711,4.43379369587739));
#98057=CARTESIAN_POINT('Ctrl Pts',(-9.29957011397894,17.3992546015039,4.44709057680385));
#98058=CARTESIAN_POINT('Ctrl Pts',(-9.39866683575855,17.3916271004004,4.51754385318835));
#98059=CARTESIAN_POINT('Ctrl Pts',(-9.48674502806125,17.385633985992,4.56469098493683));
#98060=CARTESIAN_POINT('Ctrl Pts',(-9.60545786822042,17.3774894233854,4.61004126747157));
#98061=CARTESIAN_POINT('Ctrl Pts',(-9.6315472832876,17.3756986001208,4.61897163229955));
#98062=CARTESIAN_POINT('Ctrl Pts',(-9.66600979393032,17.3733198290264,4.6294321585371));
#98063=CARTESIAN_POINT('Ctrl Pts',(-9.67412114728714,17.3727590300628,4.63179919847052));
#98064=CARTESIAN_POINT('Ctrl Pts',(-9.68744437545077,17.3718360808536,4.63553206215525));
#98065=CARTESIAN_POINT('Ctrl Pts',(-9.69264149093973,17.3714756091729,4.63694979127751));
#98066=CARTESIAN_POINT('Ctrl Pts',(-9.70273198541095,17.370774780296,4.63962815123988));
#98067=CARTESIAN_POINT('Ctrl Pts',(-9.70762411903777,17.3704345685756,4.64089304426637));
#98068=CARTESIAN_POINT('Ctrl Pts',(-9.71897395989665,17.3696441986072,4.64374982513937));
#98069=CARTESIAN_POINT('Ctrl Pts',(-9.7254372618932,17.3691933116691,4.64531855717552));
#98070=CARTESIAN_POINT('Ctrl Pts',(-9.74656079153286,17.3677169012153,4.65025644981767));
#98071=CARTESIAN_POINT('Ctrl Pts',(-9.76127182316552,17.3666842655474,4.65339939043725));
#98072=CARTESIAN_POINT('Ctrl Pts',(-9.85571246984516,17.3600238510747,4.67169205978603));
#98073=CARTESIAN_POINT('Ctrl Pts',(-9.9367538682482,17.3541444757962,4.67884543735176));
#98074=CARTESIAN_POINT('Ctrl Pts',(-10.072573854551,17.3441758565844,4.67678423744503));
#98075=CARTESIAN_POINT('Ctrl Pts',(-10.1271544461293,17.3401451258496,4.67214351736855));
#98076=CARTESIAN_POINT('Ctrl Pts',(-10.197172178646,17.335064229951,4.66124025964057));
#98077=CARTESIAN_POINT('Ctrl Pts',(-10.2130756020305,17.3339165864049,4.6584276635007));
#98078=CARTESIAN_POINT('Ctrl Pts',(-10.2394910266992,17.3320262354655,4.65319352737478));
#98079=CARTESIAN_POINT('Ctrl Pts',(-10.2500363135098,17.3312758531124,4.650953138097));
#98080=CARTESIAN_POINT('Ctrl Pts',(-10.2645952650024,17.3302471364168,4.64765047645644));
#98081=CARTESIAN_POINT('Ctrl Pts',(-10.2686359198,17.3299624090523,4.64671139101308));
#98082=CARTESIAN_POINT('Ctrl Pts',(-10.2754717259502,17.3294821388121,4.64508457130949));
#98083=CARTESIAN_POINT('Ctrl Pts',(-10.2782694473831,17.3292859807406,4.64440790917339));
#98084=CARTESIAN_POINT('Ctrl Pts',(-10.2836332805925,17.3289107143922,4.64308976925107));
#98085=CARTESIAN_POINT('Ctrl Pts',(-10.2861997385486,17.3287315129559,4.64244989755956));
#98086=CARTESIAN_POINT('Ctrl Pts',(-10.292351388053,17.328302779298,4.64089413202167));
#98087=CARTESIAN_POINT('Ctrl Pts',(-10.2959344896023,17.3280537128375,4.63996997037849));
#98088=CARTESIAN_POINT('Ctrl Pts',(-10.3089424265636,17.3271516947453,4.63654946961392));
#98089=CARTESIAN_POINT('Ctrl Pts',(-10.318340843798,17.3265041462254,4.63395292768797));
#98090=CARTESIAN_POINT('Ctrl Pts',(-10.3865819802538,17.3218255247025,4.6141843080896));
#98091=CARTESIAN_POINT('Ctrl Pts',(-10.4440445506291,17.3180092313213,4.59255605531946));
#98092=CARTESIAN_POINT('Ctrl Pts',(-10.560120283288,17.3100740337127,4.53818655485231));
#98093=CARTESIAN_POINT('Ctrl Pts',(-10.6181435769748,17.305969929319,4.50472083093807));
#98094=CARTESIAN_POINT('Ctrl Pts',(-10.7014896163509,17.2995133069973,4.44668449474595));
#98095=CARTESIAN_POINT('Ctrl Pts',(-10.7290739835956,17.2972727749235,4.42560789716553));
#98096=CARTESIAN_POINT('Ctrl Pts',(-10.7626779642778,17.2943834751922,4.39749678909456));
#98097=CARTESIAN_POINT('Ctrl Pts',(-10.76960169914,17.2937791574269,4.39156681217848));
#98098=CARTESIAN_POINT('Ctrl Pts',(-10.7806157794854,17.2928028026519,4.38190967656783));
#98099=CARTESIAN_POINT('Ctrl Pts',(-10.7847500024759,17.2924328419155,4.37823294440812));
#98100=CARTESIAN_POINT('Ctrl Pts',(-10.7925758421223,17.2917257691566,4.37117372825135));
#98101=CARTESIAN_POINT('Ctrl Pts',(-10.7962721045915,17.2913888838012,4.36779655704949));
#98102=CARTESIAN_POINT('Ctrl Pts',(-10.8046761327539,17.2906161239496,4.36001913253735));
#98103=CARTESIAN_POINT('Ctrl Pts',(-10.8093695086785,17.2901796089906,4.35560363633394));
#98104=CARTESIAN_POINT('Ctrl Pts',(-10.8237967333067,17.2888221400999,4.34180566671745));
#98105=CARTESIAN_POINT('Ctrl Pts',(-10.8334051423428,17.2878956641149,4.33229422714102));
#98106=CARTESIAN_POINT('Ctrl Pts',(-10.9137217752634,17.2799542891264,4.25000267635647));
#98107=CARTESIAN_POINT('Ctrl Pts',(-10.9749011388234,17.2725221230667,4.16854374949347));
#98108=CARTESIAN_POINT('Ctrl Pts',(-11.0534675886108,17.2608240591044,4.02978173965813));
#98109=CARTESIAN_POINT('Ctrl Pts',(-11.0782917205095,17.2565926211596,3.97723287836739));
#98110=CARTESIAN_POINT('Ctrl Pts',(-11.1017382619598,17.2520488313538,3.9163173060824));
#98111=CARTESIAN_POINT('Ctrl Pts',(-11.1042723586862,17.2515488172985,3.90954836297565));
#98112=CARTESIAN_POINT('Ctrl Pts',(-11.1079524306741,17.25080951544,3.89943580185742));
#98113=CARTESIAN_POINT('Ctrl Pts',(-11.1091458709735,17.2505675938226,3.89610981579618));
#98114=CARTESIAN_POINT('Ctrl Pts',(-11.1111659252887,17.2501544080104,3.89039943260829));
#98115=CARTESIAN_POINT('Ctrl Pts',(-11.1119998627632,17.2499827200348,3.88801770083609));
#98116=CARTESIAN_POINT('Ctrl Pts',(-11.1138763737146,17.2495938495733,3.88260263208626));
#98117=CARTESIAN_POINT('Ctrl Pts',(-11.1149142153731,17.2493769453927,3.87956770539574));
#98118=CARTESIAN_POINT('Ctrl Pts',(-11.1177034058787,17.2487888778477,3.87130121812602));
#98119=CARTESIAN_POINT('Ctrl Pts',(-11.1194304427223,17.2484190953651,3.86606144971446));
#98120=CARTESIAN_POINT('Ctrl Pts',(-11.1278148916153,17.2465942984114,3.84000898774695));
#98121=CARTESIAN_POINT('Ctrl Pts',(-11.1339294885263,17.2451679492855,3.81902445715034));
#98122=CARTESIAN_POINT('Ctrl Pts',(-11.1450412726649,17.2423428839156,3.77651947057751));
#98123=CARTESIAN_POINT('Ctrl Pts',(-11.1500240192672,17.2409451725356,3.75500467903139));
#98124=CARTESIAN_POINT('Ctrl Pts',(-11.174114333255,17.2333181119477,3.63583404759753));
#98125=CARTESIAN_POINT('Ctrl Pts',(-11.1813911463629,17.227325515038,3.53620508583269));
#98126=CARTESIAN_POINT('Ctrl Pts',(-11.1745765736589,17.2191808825607,3.40930483203998));
#98127=CARTESIAN_POINT('Ctrl Pts',(-11.1721307823067,17.2173893332852,3.38182648803447));
#98128=CARTESIAN_POINT('Ctrl Pts',(-11.1676786935231,17.2150097324581,3.34607486324095));
#98129=CARTESIAN_POINT('Ctrl Pts',(-11.1665441857005,17.2144488540573,3.33770047549173));
#98130=CARTESIAN_POINT('Ctrl Pts',(-11.164539037471,17.2135258075428,3.32400876252105));
#98131=CARTESIAN_POINT('Ctrl Pts',(-11.1637218426613,17.2131653186904,3.31868382109233));
#98132=CARTESIAN_POINT('Ctrl Pts',(-11.1620674307859,17.2124644803542,3.30837567799001));
#98133=CARTESIAN_POINT('Ctrl Pts',(-11.1612346191042,17.2121242765026,3.30339188088765));
#98134=CARTESIAN_POINT('Ctrl Pts',(-11.1592314952053,17.2113339601377,3.29186151397659));
#98135=CARTESIAN_POINT('Ctrl Pts',(-11.1580377619944,17.2108831192393,3.28531924287277));
#98136=CARTESIAN_POINT('Ctrl Pts',(-11.1539640865752,17.2094070166724,3.26401672729102));
#98137=CARTESIAN_POINT('Ctrl Pts',(-11.1508569370317,17.2083746469701,3.24930199012066));
#98138=CARTESIAN_POINT('Ctrl Pts',(-11.1291514781064,17.2017043210926,3.15543928573489));
#98139=CARTESIAN_POINT('Ctrl Pts',(-11.102684356821,17.1958137543111,3.07835109768309));
#98140=CARTESIAN_POINT('Ctrl Pts',(-11.0455341864625,17.1858422856597,2.9550833263934));
#98141=CARTESIAN_POINT('Ctrl Pts',(-11.0191520311363,17.1818200062232,2.90720524077042));
#98142=CARTESIAN_POINT('Ctrl Pts',(-10.9807953895367,17.1767485654876,2.84777639580538));
#98143=CARTESIAN_POINT('Ctrl Pts',(-10.9717706708856,17.1756022385524,2.83440474449362));
#98144=CARTESIAN_POINT('Ctrl Pts',(-10.9562661309363,17.1737138194675,2.81242007217052));
#98145=CARTESIAN_POINT('Ctrl Pts',(-10.9499378772116,17.1729640712155,2.80370328132348));
#98146=CARTESIAN_POINT('Ctrl Pts',(-10.9410085958841,17.1719360715791,2.79175210441003));
#98147=CARTESIAN_POINT('Ctrl Pts',(-10.938508961301,17.1716514385816,2.78844312243826));
#98148=CARTESIAN_POINT('Ctrl Pts',(-10.9342449720051,17.1711712805833,2.7828600708201));
#98149=CARTESIAN_POINT('Ctrl Pts',(-10.9324896788673,17.1709751410445,2.78057915986265));
#98150=CARTESIAN_POINT('Ctrl Pts',(-10.9291050400307,17.1705998730916,2.77621419976628));
#98151=CARTESIAN_POINT('Ctrl Pts',(-10.9274770179667,17.1704206517358,2.77412918399537));
#98152=CARTESIAN_POINT('Ctrl Pts',(-10.9235541674355,17.1699918219666,2.76913991568097));
#98153=CARTESIAN_POINT('Ctrl Pts',(-10.9212526276833,17.1697426797804,2.76624093876215));
#98154=CARTESIAN_POINT('Ctrl Pts',(-10.9128336325921,17.1688399874606,2.75573858464276));
#98155=CARTESIAN_POINT('Ctrl Pts',(-10.9066351989577,17.16819185133,2.74820020852376));
#98156=CARTESIAN_POINT('Ctrl Pts',(-10.8600677683204,17.1634351193504,2.69297979029275));
#98157=CARTESIAN_POINT('Ctrl Pts',(-10.8160499546143,17.1595497864289,2.64849383555287));
#98158=CARTESIAN_POINT('Ctrl Pts',(-10.7187214327034,17.1515991480519,2.56464602410488));
#98159=CARTESIAN_POINT('Ctrl Pts',(-10.665211674425,17.1475469045515,2.52586430782066));
#98160=CARTESIAN_POINT('Ctrl Pts',(-10.579252481404,17.1411616396978,2.47396493294573));
#98161=CARTESIAN_POINT('Ctrl Pts',(-10.5490025881403,17.1389372743217,2.45746597179674));
#98162=CARTESIAN_POINT('Ctrl Pts',(-10.5099077916215,17.1360662291564,2.43831651559632));
#98163=CARTESIAN_POINT('Ctrl Pts',(-10.5016943451274,17.1354632971443,2.43441070134914));
#98164=CARTESIAN_POINT('Ctrl Pts',(-10.4884172343356,17.1344886448504,2.42828444700081));
#98165=CARTESIAN_POINT('Ctrl Pts',(-10.4833816245031,17.1341189876688,2.4260038060321));
#98166=CARTESIAN_POINT('Ctrl Pts',(-10.4737539700971,17.1334121411884,2.42172484166972));
#98167=CARTESIAN_POINT('Ctrl Pts',(-10.469164858707,17.1330751760915,2.41972018658361));
#98168=CARTESIAN_POINT('Ctrl Pts',(-10.4586335687912,17.1323017301232,2.41519958022651));
#98169=CARTESIAN_POINT('Ctrl Pts',(-10.4526832621156,17.131864604729,2.41270309368438));
#98170=CARTESIAN_POINT('Ctrl Pts',(-10.4341604171754,17.1305033201419,2.40511012669013));
#98171=CARTESIAN_POINT('Ctrl Pts',(-10.4215205037104,17.1295735940546,2.40018204202376));
#98172=CARTESIAN_POINT('Ctrl Pts',(-10.3139818400233,17.1216538194914,2.36038066837943));
#98173=CARTESIAN_POINT('Ctrl Pts',(-10.2150582414701,17.1142500139131,2.33764964899599));
#98174=CARTESIAN_POINT('Ctrl Pts',(-10.0564379585503,17.1025575313189,2.32215861232979));
#98175=CARTESIAN_POINT('Ctrl Pts',(-9.99805208773803,17.0983045479692,2.32080815804299));
#98176=CARTESIAN_POINT('Ctrl Pts',(-9.93257457511583,17.0937403939624,2.32415935355092));
#98177=CARTESIAN_POINT('Ctrl Pts',(-9.92535194780163,17.0932398142679,2.3245957764874));
#98178=CARTESIAN_POINT('Ctrl Pts',(-9.91460699311278,17.0924998428301,2.32534447855696));
#98179=CARTESIAN_POINT('Ctrl Pts',(-9.91108147427308,17.092257810487,2.32560608981017));
#98180=CARTESIAN_POINT('Ctrl Pts',(-9.90504124398679,17.0918445013059,2.32608166124239));
#98181=CARTESIAN_POINT('Ctrl Pts',(-9.9025259898384,17.0916727999562,2.32628783375014));
#98182=CARTESIAN_POINT('Ctrl Pts',(-9.89681658379889,17.0912839880879,2.32677430743151));
#98183=CARTESIAN_POINT('Ctrl Pts',(-9.8936229018936,17.0910671553208,2.32705956813609));
#98184=CARTESIAN_POINT('Ctrl Pts',(-9.88494212510772,17.0904794718429,2.32787068469085));
#98185=CARTESIAN_POINT('Ctrl Pts',(-9.87945740769035,17.0901099990113,2.32842203299157));
#98186=CARTESIAN_POINT('Ctrl Pts',(-9.85294818461416,17.0883322527072,2.33127499243877));
#98187=CARTESIAN_POINT('Ctrl Pts',(-9.83198303316909,17.0869507190748,2.33410429166349));
#98188=CARTESIAN_POINT('Ctrl Pts',(-9.81110406370722,17.0855891663962,2.33749693000316));
#98189=CARTESIAN_POINT('Ctrl Pts',(-9.81110407400449,16.9868193101849,2.33749692832995));
#98190=CARTESIAN_POINT('Ctrl Pts',(-9.82687262829458,16.9879364648105,2.33493468506641));
#98191=CARTESIAN_POINT('Ctrl Pts',(-9.84269296230412,16.9890630504714,2.3326933323682));
#98192=CARTESIAN_POINT('Ctrl Pts',(-9.92559485983192,16.9949961523911,2.32266444726947));
#98193=CARTESIAN_POINT('Ctrl Pts',(-9.99320091986613,16.9999455831111,2.32033606303029));
#98194=CARTESIAN_POINT('Ctrl Pts',(-10.1209404481883,17.0093371042531,2.32692028691367));
#98195=CARTESIAN_POINT('Ctrl Pts',(-10.1809331922842,17.0137613931877,2.334664303754));
#98196=CARTESIAN_POINT('Ctrl Pts',(-10.2496419380673,17.0186795918734,2.34897023702307));
#98197=CARTESIAN_POINT('Ctrl Pts',(-10.2591868925245,17.0193592965465,2.35108190769054));
#98198=CARTESIAN_POINT('Ctrl Pts',(-10.2723098244549,17.0202879124601,2.35415702139561));
#98199=CARTESIAN_POINT('Ctrl Pts',(-10.275910877022,17.0205421193972,2.35501879448393));
#98200=CARTESIAN_POINT('Ctrl Pts',(-10.2820773387284,17.020976302027,2.35652528068629));
#98201=CARTESIAN_POINT('Ctrl Pts',(-10.2846447217656,17.0211567377636,2.3571616730881));
#98202=CARTESIAN_POINT('Ctrl Pts',(-10.2899996293392,17.0215323507873,2.35850819024454));
#98203=CARTESIAN_POINT('Ctrl Pts',(-10.2927867233921,17.0217274302065,2.35921988464087));
#98204=CARTESIAN_POINT('Ctrl Pts',(-10.2995809381463,17.0222020231084,2.36098135105936));
#98205=CARTESIAN_POINT('Ctrl Pts',(-10.3035852330447,17.0224809171499,2.36204207955225));
#98206=CARTESIAN_POINT('Ctrl Pts',(-10.3179569914633,17.0234792325595,2.36593038538513));
#98207=CARTESIAN_POINT('Ctrl Pts',(-10.3282916189902,17.0241921283395,2.36887879857151));
#98208=CARTESIAN_POINT('Ctrl Pts',(-10.3539873645198,17.0259555207915,2.37659151778332));
#98209=CARTESIAN_POINT('Ctrl Pts',(-10.3692943477133,17.0269977569866,2.38152987938963));
#98210=CARTESIAN_POINT('Ctrl Pts',(-10.4358262820918,17.0315111523539,2.40450941921656));
#98211=CARTESIAN_POINT('Ctrl Pts',(-10.4858729279928,17.0348646279584,2.42576883531757));
#98212=CARTESIAN_POINT('Ctrl Pts',(-10.6070761156188,17.0432718359703,2.48746525232517));
#98213=CARTESIAN_POINT('Ctrl Pts',(-10.6758133256797,17.0483210403588,2.53199056999242));
#98214=CARTESIAN_POINT('Ctrl Pts',(-10.7510835267188,17.0546281546339,2.59269939687553));
#98215=CARTESIAN_POINT('Ctrl Pts',(-10.7625975038567,17.055616306033,2.60235538088719));
#98216=CARTESIAN_POINT('Ctrl Pts',(-10.7789334426548,17.0570543485397,2.61659639223207));
#98217=CARTESIAN_POINT('Ctrl Pts',(-10.7839065453081,17.0574970975203,2.62100638939758));
#98218=CARTESIAN_POINT('Ctrl Pts',(-10.7925925869622,17.058279374547,2.62884125099657));
#98219=CARTESIAN_POINT('Ctrl Pts',(-10.7963213524118,17.0586181579439,2.63224837816067));
#98220=CARTESIAN_POINT('Ctrl Pts',(-10.803980610741,17.059320288101,2.63933790140317));
#98221=CARTESIAN_POINT('Ctrl Pts',(-10.8079079840038,17.0596837650181,2.6430234786624));
#98222=CARTESIAN_POINT('Ctrl Pts',(-10.8179318016278,17.0606204832105,2.65256030715612));
#98223=CARTESIAN_POINT('Ctrl Pts',(-10.8239907152286,17.0611953830694,2.65845038182173));
#98224=CARTESIAN_POINT('Ctrl Pts',(-10.8495600067438,17.0636594986468,2.68384802517512));
#98225=CARTESIAN_POINT('Ctrl Pts',(-10.8684436345414,17.0655755386833,2.70397130432733));
#98226=CARTESIAN_POINT('Ctrl Pts',(-10.9520794205608,17.0745279096467,2.79961848381354));
#98227=CARTESIAN_POINT('Ctrl Pts',(-11.0077996568005,17.0819073703161,2.8824861017343));
#98228=CARTESIAN_POINT('Ctrl Pts',(-11.0623527246101,17.0907658481259,2.99108950213175));
#98229=CARTESIAN_POINT('Ctrl Pts',(-11.0717129643809,17.0923658514626,3.01110878299789));
#98230=CARTESIAN_POINT('Ctrl Pts',(-11.089206372254,17.0955106220769,3.05144365997242));
#98231=CARTESIAN_POINT('Ctrl Pts',(-11.0973480784597,17.0970552132044,3.07174697196738));
#98232=CARTESIAN_POINT('Ctrl Pts',(-11.1068302271722,17.0989526711052,3.09744273743843));
#98233=CARTESIAN_POINT('Ctrl Pts',(-11.108703899626,17.0993329900199,3.10263220138506));
#98234=CARTESIAN_POINT('Ctrl Pts',(-11.1116088825349,17.0999311101014,3.11085858808792));
#98235=CARTESIAN_POINT('Ctrl Pts',(-11.1126643459147,17.1001502686497,3.11388680396861));
#98236=CARTESIAN_POINT('Ctrl Pts',(-11.1145279413001,17.1005405162536,3.1193047231226));
#98237=CARTESIAN_POINT('Ctrl Pts',(-11.1153407605827,17.1007118725803,3.12169269933319));
#98238=CARTESIAN_POINT('Ctrl Pts',(-11.1172731026307,17.1011220437513,3.12743007661678));
#98239=CARTESIAN_POINT('Ctrl Pts',(-11.1183852396983,17.101360426323,3.13078192065424));
#98240=CARTESIAN_POINT('Ctrl Pts',(-11.1217252777694,17.1020836361068,3.14100195276905));
#98241=CARTESIAN_POINT('Ctrl Pts',(-11.1239051620776,17.1025657800411,3.14788582843654));
#98242=CARTESIAN_POINT('Ctrl Pts',(-11.1429758088692,17.1068815077113,3.21009124580378));
#98243=CARTESIAN_POINT('Ctrl Pts',(-11.1558354034119,17.1105102404496,3.26657507215084));
#98244=CARTESIAN_POINT('Ctrl Pts',(-11.1797104012322,17.1204144291953,3.42434729725979));
#98245=CARTESIAN_POINT('Ctrl Pts',(-11.1818368910928,17.1266064289127,3.52644783762702));
#98246=CARTESIAN_POINT('Ctrl Pts',(-11.1693623135265,17.1341386674072,3.6409564495467));
#98247=CARTESIAN_POINT('Ctrl Pts',(-11.1676716426524,17.1350271761402,3.65433681195003));
#98248=CARTESIAN_POINT('Ctrl Pts',(-11.1648352529803,17.1363502821643,3.67405551476322));
#98249=CARTESIAN_POINT('Ctrl Pts',(-11.1638666741784,17.1367793509037,3.68041854330826));
#98250=CARTESIAN_POINT('Ctrl Pts',(-11.1620523849599,17.1375449473497,3.69171426922652));
#98251=CARTESIAN_POINT('Ctrl Pts',(-11.1612272910909,17.1378808203797,3.69665015513936));
#98252=CARTESIAN_POINT('Ctrl Pts',(-11.1594236613267,17.138590184991,3.70703250145479));
#98253=CARTESIAN_POINT('Ctrl Pts',(-11.1584381496537,17.1389638887839,3.71247760992541));
#98254=CARTESIAN_POINT('Ctrl Pts',(-11.1557258072524,17.1399571302396,3.72688367120089));
#98255=CARTESIAN_POINT('Ctrl Pts',(-11.1539331631769,17.1405787286631,3.73583169541007));
#98256=CARTESIAN_POINT('Ctrl Pts',(-11.1447953667268,17.1435897567271,3.77884188236983));
#98257=CARTESIAN_POINT('Ctrl Pts',(-11.136045670349,17.146023141685,3.81258442900027));
#98258=CARTESIAN_POINT('Ctrl Pts',(-11.1060262281172,17.1532852806912,3.91029361819776));
#98259=CARTESIAN_POINT('Ctrl Pts',(-11.0807498226625,17.1582231912283,3.97287715392995));
#98260=CARTESIAN_POINT('Ctrl Pts',(-11.0228408885473,17.1676194054333,4.08699643514581));
#98261=CARTESIAN_POINT('Ctrl Pts',(-10.9912813124837,17.1720598246634,4.13885144328646));
#98262=CARTESIAN_POINT('Ctrl Pts',(-10.9501619013483,17.1769921232222,4.19597613735019));
#98263=CARTESIAN_POINT('Ctrl Pts',(-10.9443583831479,17.1776711419506,4.20383071988942));
#98264=CARTESIAN_POINT('Ctrl Pts',(-10.936221161021,17.1785989975121,4.21456189420631));
#98265=CARTESIAN_POINT('Ctrl Pts',(-10.9339707844318,17.1788531186232,4.21750075801676));
#98266=CARTESIAN_POINT('Ctrl Pts',(-10.9300887829504,17.1792871929513,4.22252121964311));
#98267=CARTESIAN_POINT('Ctrl Pts',(-10.9284639505356,17.1794676057186,4.22460799741275));
#98268=CARTESIAN_POINT('Ctrl Pts',(-10.9250570652339,17.1798432143,4.22895319769596));
#98269=CARTESIAN_POINT('Ctrl Pts',(-10.92327374978,17.1800383120275,4.23121058634027));
#98270=CARTESIAN_POINT('Ctrl Pts',(-10.9189015815921,17.180513020354,4.23670354725031));
#98271=CARTESIAN_POINT('Ctrl Pts',(-10.9163038566028,17.1807920107929,4.2399320758402));
#98272=CARTESIAN_POINT('Ctrl Pts',(-10.9069024269054,17.1817910610512,4.25149100712855));
#98273=CARTESIAN_POINT('Ctrl Pts',(-10.9000014750169,17.1825045826406,4.25974213450892));
#98274=CARTESIAN_POINT('Ctrl Pts',(-10.8824904511935,17.1842698370897,4.28010569646978));
#98275=CARTESIAN_POINT('Ctrl Pts',(-10.8717429627807,17.1853132870545,4.29209756654184));
#98276=CARTESIAN_POINT('Ctrl Pts',(-10.823605359562,17.1898353444747,4.34364168445352));
#98277=CARTESIAN_POINT('Ctrl Pts',(-10.7837428566908,17.1931958084554,4.38079802170576));
#98278=CARTESIAN_POINT('Ctrl Pts',(-10.6781045261366,17.2016005682292,4.46639356104486));
#98279=CARTESIAN_POINT('Ctrl Pts',(-10.6096085871802,17.2066406280104,4.51099827877615));
#98280=CARTESIAN_POINT('Ctrl Pts',(-10.5236831149352,17.2129376874234,4.55502463241893));
#98281=CARTESIAN_POINT('Ctrl Pts',(-10.5101768129957,17.2139261212104,4.56162166797046));
#98282=CARTESIAN_POINT('Ctrl Pts',(-10.4905205877644,17.2153645010086,4.5707608535365));
#98283=CARTESIAN_POINT('Ctrl Pts',(-10.4844692149484,17.2158073001399,4.5735123796243));
#98284=CARTESIAN_POINT('Ctrl Pts',(-10.4737793434038,17.2165896356766,4.5782642115532));
#98285=CARTESIAN_POINT('Ctrl Pts',(-10.4691506221937,17.2169284270817,4.58028619748973));
#98286=CARTESIAN_POINT('Ctrl Pts',(-10.45956007375,17.217630544414,4.58440241873539));
#98287=CARTESIAN_POINT('Ctrl Pts',(-10.4545966102907,17.2179940003187,4.58649251603001));
#98288=CARTESIAN_POINT('Ctrl Pts',(-10.4418103342571,17.2189306018767,4.59177381818562));
#98289=CARTESIAN_POINT('Ctrl Pts',(-10.4339673150089,17.2195054053169,4.59491497594865));
#98290=CARTESIAN_POINT('Ctrl Pts',(-10.4003828475264,17.221968517575,4.60794814884276));
#98291=CARTESIAN_POINT('Ctrl Pts',(-10.3743339102746,17.2238836234645,4.61701809684796));
#98292=CARTESIAN_POINT('Ctrl Pts',(-10.252953543995,17.2328356201768,4.65455877366912));
#98293=CARTESIAN_POINT('Ctrl Pts',(-10.1545823256587,17.2402157859513,4.6717891575727));
#98294=CARTESIAN_POINT('Ctrl Pts',(-10.0331724901668,17.2490749286032,4.67749001702489));
#98295=CARTESIAN_POINT('Ctrl Pts',(-10.0110781180791,17.2506748555152,4.67790514190264));
#98296=CARTESIAN_POINT('Ctrl Pts',(-9.96710983856224,17.2538200244126,4.67749387588873));
#98297=CARTESIAN_POINT('Ctrl Pts',(-9.94524369011949,17.255365076605,4.67667985743916));
#98298=CARTESIAN_POINT('Ctrl Pts',(-9.91790528943456,17.2572630166728,4.67489827891918));
#98299=CARTESIAN_POINT('Ctrl Pts',(-9.9124017398964,17.257643372882,4.67450076846999));
#98300=CARTESIAN_POINT('Ctrl Pts',(-9.90370414561147,17.25824153848,4.67381108165236));
#98301=CARTESIAN_POINT('Ctrl Pts',(-9.90050823801416,17.2584607055848,4.67354451850083));
#98302=CARTESIAN_POINT('Ctrl Pts',(-9.89480048423873,17.258850960419,4.67304496399591));
#98303=CARTESIAN_POINT('Ctrl Pts',(-9.89228831064863,17.2590223154826,4.67281695836535));
#98304=CARTESIAN_POINT('Ctrl Pts',(-9.88626103793831,17.2594324733508,4.67225039172847));
#98305=CARTESIAN_POINT('Ctrl Pts',(-9.88274670873525,17.2596708439645,4.67190409117164));
#98306=CARTESIAN_POINT('Ctrl Pts',(-9.87205249856307,17.2603939809586,4.67080169985893));
#98307=CARTESIAN_POINT('Ctrl Pts',(-9.86487780036977,17.26087606485,4.66999537654611));
#98308=CARTESIAN_POINT('Ctrl Pts',(-9.80032379330966,17.265189633235,4.66213876912325));
#98309=CARTESIAN_POINT('Ctrl Pts',(-9.74352041525188,17.2688164906964,4.65093753852879));
#98310=CARTESIAN_POINT('Ctrl Pts',(-9.58965229426639,17.2787214322882,4.60863122574422));
#98311=CARTESIAN_POINT('Ctrl Pts',(-9.49546241337616,17.2849157745005,4.56905950376768));
#98312=CARTESIAN_POINT('Ctrl Pts',(-9.39588069493815,17.2924504559308,4.51109676171421));
#98313=CARTESIAN_POINT('Ctrl Pts',(-9.38434746939944,17.2933386171025,4.50411589644992));
#98314=CARTESIAN_POINT('Ctrl Pts',(-9.36748964129111,17.2946613035976,4.49351251718253));
#98315=CARTESIAN_POINT('Ctrl Pts',(-9.36207056644262,17.2950903055287,4.49004167119475));
#98316=CARTESIAN_POINT('Ctrl Pts',(-9.35248854127248,17.2958558270662,4.48379317744511));
#98317=CARTESIAN_POINT('Ctrl Pts',(-9.34831430576273,17.2961916924651,4.4810330574309));
#98318=CARTESIAN_POINT('Ctrl Pts',(-9.33956115870797,17.2969010866548,4.47516471737606));
#98319=CARTESIAN_POINT('Ctrl Pts',(-9.33498632304281,17.2972748279428,4.47205066573273));
#98320=CARTESIAN_POINT('Ctrl Pts',(-9.32292411781731,17.2982682763617,4.46371501841445));
#98321=CARTESIAN_POINT('Ctrl Pts',(-9.31547534105932,17.2988900457865,4.45843850615423));
#98322=CARTESIAN_POINT('Ctrl Pts',(-9.27986661192313,17.3019033369657,4.43258739286108));
#98323=CARTESIAN_POINT('Ctrl Pts',(-9.25257119611444,17.304338894553,4.41085733640836));
#98324=CARTESIAN_POINT('Ctrl Pts',(-9.17540268079448,17.3116110208776,4.34361635342126));
#98325=CARTESIAN_POINT('Ctrl Pts',(-9.12843293248147,17.3165571341783,4.29499575024614));
#98326=CARTESIAN_POINT('Ctrl Pts',(-9.04776862293908,17.3259500261124,4.19570498750087));
#98327=CARTESIAN_POINT('Ctrl Pts',(-9.0133135572525,17.330378977973,4.14591128741427));
#98328=CARTESIAN_POINT('Ctrl Pts',(-8.97790621627555,17.3353012383064,4.08524768353308));
#98329=CARTESIAN_POINT('Ctrl Pts',(-8.97308532936232,17.3359807311223,4.07674676298711));
#98330=CARTESIAN_POINT('Ctrl Pts',(-8.96658451774456,17.3369091122139,4.06494354614598));
#98331=CARTESIAN_POINT('Ctrl Pts',(-8.96481368844185,17.3371632926581,4.06169214930605));
#98332=CARTESIAN_POINT('Ctrl Pts',(-8.96180408813488,17.3375974418566,4.05610368348576));
#98333=CARTESIAN_POINT('Ctrl Pts',(-8.96055781773783,17.3377778705023,4.05377071815689));
#98334=CARTESIAN_POINT('Ctrl Pts',(-8.95797255652792,17.3381534821491,4.04889174188054));
#98335=CARTESIAN_POINT('Ctrl Pts',(-8.95663502096059,17.3383485672149,4.04634499906722));
#98336=CARTESIAN_POINT('Ctrl Pts',(-8.95339401928569,17.3388231957234,4.04011864065652));
#98337=CARTESIAN_POINT('Ctrl Pts',(-8.95150058689536,17.3391021195032,4.03643378609914));
#98338=CARTESIAN_POINT('Ctrl Pts',(-8.94476445295105,17.3401006615646,4.0231525046579));
#98339=CARTESIAN_POINT('Ctrl Pts',(-8.94003355744219,17.3408137503602,4.01349952654305));
#98340=CARTESIAN_POINT('Ctrl Pts',(-8.92855393456318,17.3425777170407,3.98924144625323));
#98341=CARTESIAN_POINT('Ctrl Pts',(-8.92197088422407,17.3436203275388,3.97455994696074));
#98342=CARTESIAN_POINT('Ctrl Pts',(-8.89447730638538,17.3481363925261,3.90971662513464));
#98343=CARTESIAN_POINT('Ctrl Pts',(-8.87675062626698,17.351492021793,3.85827352843769));
#98344=CARTESIAN_POINT('Ctrl Pts',(-8.84144259686948,17.3598984731633,3.72694673421329));
#98345=CARTESIAN_POINT('Ctrl Pts',(-8.82850314153887,17.3649448581125,3.64612689902622));
#98346=CARTESIAN_POINT('Ctrl Pts',(-8.82319971781619,17.3712488727301,3.5496183964485));
#98347=CARTESIAN_POINT('Ctrl Pts',(-8.82266244504893,17.3722371120225,3.53459967744389));
#98348=CARTESIAN_POINT('Ctrl Pts',(-8.82230221160309,17.3736752595121,3.51292921800282));
#98349=CARTESIAN_POINT('Ctrl Pts',(-8.82224799989554,17.3741180241031,3.50628241005698));
#98350=CARTESIAN_POINT('Ctrl Pts',(-8.8222516191197,17.3749003193418,3.49458459559518));
#98351=CARTESIAN_POINT('Ctrl Pts',(-8.82228567526641,17.375239105231,3.4895337099509));
#98352=CARTESIAN_POINT('Ctrl Pts',(-8.8224231775298,17.3759412313941,3.47909792897358));
#98353=CARTESIAN_POINT('Ctrl Pts',(-8.82253107346238,17.3763047017689,3.47371322075556));
#98354=CARTESIAN_POINT('Ctrl Pts',(-8.82290311180482,17.3772413836474,3.45988300138625));
#98355=CARTESIAN_POINT('Ctrl Pts',(-8.82322121166186,17.3778162534867,3.45143937178742));
#98356=CARTESIAN_POINT('Ctrl Pts',(-8.82496519553064,17.3802800566355,3.41544686134525));
#98357=CARTESIAN_POINT('Ctrl Pts',(-8.82726777203367,17.3821958057772,3.38795123295226));
#98358=CARTESIAN_POINT('Ctrl Pts',(-8.84231012943649,17.3911480601531,3.26178944834142));
#98359=CARTESIAN_POINT('Ctrl Pts',(-8.86655299930821,17.3985277403416,3.16491483118665));
#98360=CARTESIAN_POINT('Ctrl Pts',(-8.91069341185114,17.4073864251229,3.05167606897221));
#98361=CARTESIAN_POINT('Ctrl Pts',(-8.91929548709607,17.4089864046491,3.03131989624863));
#98362=CARTESIAN_POINT('Ctrl Pts',(-8.93754226602037,17.4121312993167,2.99131840811716));
#98363=CARTESIAN_POINT('Ctrl Pts',(-8.94717224803877,17.4136760340582,2.97167503094053));
#98364=CARTESIAN_POINT('Ctrl Pts',(-8.95991020370921,17.415573642148,2.94742537254336));
#98365=CARTESIAN_POINT('Ctrl Pts',(-8.96251028017742,17.4159539726808,2.9425588932285));
#98366=CARTESIAN_POINT('Ctrl Pts',(-8.96667556257935,17.4165521069417,2.93489297166834));
#98367=CARTESIAN_POINT('Ctrl Pts',(-8.96821812784317,17.4167712681556,2.9320814183766));
#98368=CARTESIAN_POINT('Ctrl Pts',(-8.97099457766154,17.4171615180117,2.92706957966829));
#98369=CARTESIAN_POINT('Ctrl Pts',(-8.97222404071616,17.4173328739448,2.92486696891829));
#98370=CARTESIAN_POINT('Ctrl Pts',(-8.97519169550874,17.4177430409711,2.91959025480199));
#98371=CARTESIAN_POINT('Ctrl Pts',(-8.97693664652385,17.4179814198171,2.91652000131271));
#98372=CARTESIAN_POINT('Ctrl Pts',(-8.98229116824021,17.418704606922,2.90719655335674));
#98373=CARTESIAN_POINT('Ctrl Pts',(-8.98594453688608,17.4191867321488,2.90096851770535));
#98374=CARTESIAN_POINT('Ctrl Pts',(-9.01937410399039,17.4235017868848,2.84516224096491));
#98375=CARTESIAN_POINT('Ctrl Pts',(-9.05271147142192,17.4271299352077,2.79779919344989));
#98376=CARTESIAN_POINT('Ctrl Pts',(-9.15391153174446,17.4370343584137,2.67442328908591));
#98377=CARTESIAN_POINT('Ctrl Pts',(-9.22833289443858,17.4432270880622,2.6044719750592));
#98378=CARTESIAN_POINT('Ctrl Pts',(-9.32174746321755,17.4507600878111,2.53706158439215));
#98379=CARTESIAN_POINT('Ctrl Pts',(-9.33281653587819,17.4516484883042,2.52935943999387));
#98380=CARTESIAN_POINT('Ctrl Pts',(-9.34936031547011,17.4529714636773,2.51826455415408));
#98381=CARTESIAN_POINT('Ctrl Pts',(-9.35473478414655,17.4534005116124,2.514723752873));
#98382=CARTESIAN_POINT('Ctrl Pts',(-9.36433928730087,17.4541660847305,2.50850841437812));
#98383=CARTESIAN_POINT('Ctrl Pts',(-9.36855788874728,17.4545019553831,2.50581643302681));
#98384=CARTESIAN_POINT('Ctrl Pts',(-9.3774772399631,17.4552113291997,2.50020447180118));
#98385=CARTESIAN_POINT('Ctrl Pts',(-9.38218165776093,17.4555850446643,2.49729058089947));
#98386=CARTESIAN_POINT('Ctrl Pts',(-9.39469879924941,17.4565783505446,2.48965906139158));
#98387=CARTESIAN_POINT('Ctrl Pts',(-9.40254599372701,17.4572000021982,2.48499898616939));
#98388=CARTESIAN_POINT('Ctrl Pts',(-9.44061947325637,17.4602117344973,2.4629834566206));
#98389=CARTESIAN_POINT('Ctrl Pts',(-9.47154917383984,17.4626457955063,2.44688596426713));
#98390=CARTESIAN_POINT('Ctrl Pts',(-9.56426336003494,17.4699110406619,2.40374595428708));
#98391=CARTESIAN_POINT('Ctrl Pts',(-9.62770498123338,17.4748515018915,2.38061004079575));
#98392=CARTESIAN_POINT('Ctrl Pts',(-9.73176023620944,17.4827656947702,2.35249233484872));
#98393=CARTESIAN_POINT('Ctrl Pts',(-9.77125785283919,17.4857257135124,2.34397156772625));
#98394=CARTESIAN_POINT('Ctrl Pts',(-9.81110409010019,17.488629053511,2.33749692571455));
#98395=CARTESIAN_POINT('Origin',(-10.,12.3756328852638,3.5));
#98396=CARTESIAN_POINT('',(-9.81110406180285,18.0875733665016,2.3374969303126));
#98397=CARTESIAN_POINT('',(-9.81110440024615,17.9879475328942,2.33749687531877));
#98398=CARTESIAN_POINT('',(-9.81110406371068,12.3756328852638,2.3374969300026));
#98399=CARTESIAN_POINT('Ctrl Pts',(-9.81110406180295,18.0875733665016,2.33749693031259));
#98400=CARTESIAN_POINT('Ctrl Pts',(-9.80411576776501,18.0871092595767,2.33863246310653));
#98401=CARTESIAN_POINT('Ctrl Pts',(-9.79714781030033,18.0866439604605,2.33982924799533));
#98402=CARTESIAN_POINT('Ctrl Pts',(-9.78457900609619,18.085799814295,2.34210480910901));
#98403=CARTESIAN_POINT('Ctrl Pts',(-9.77898416092229,18.0854223152074,2.34315970216565));
#98404=CARTESIAN_POINT('Ctrl Pts',(-9.76860887088543,18.0847189211277,2.34519394788202));
#98405=CARTESIAN_POINT('Ctrl Pts',(-9.76382641997234,18.0843933690987,2.34616252811452));
#98406=CARTESIAN_POINT('Ctrl Pts',(-9.7543469513773,18.0837453786588,2.34814378982686));
#98407=CARTESIAN_POINT('Ctrl Pts',(-9.74964983682037,18.083422974984,2.34915555185095));
#98408=CARTESIAN_POINT('Ctrl Pts',(-9.74029428288418,18.0827781235177,2.35123073065637));
#98409=CARTESIAN_POINT('Ctrl Pts',(-9.73563586249765,18.0824556919656,2.35229381140935));
#98410=CARTESIAN_POINT('Ctrl Pts',(-9.72311122132061,18.0815851196476,2.35523231143811));
#98411=CARTESIAN_POINT('Ctrl Pts',(-9.71525775263558,18.0810353104942,2.35716042096048));
#98412=CARTESIAN_POINT('Ctrl Pts',(-9.6857551707701,18.0789546778497,2.36472659120069));
#98413=CARTESIAN_POINT('Ctrl Pts',(-9.66424953609222,18.0774069270469,2.37089990130395));
#98414=CARTESIAN_POINT('Ctrl Pts',(-9.53566511287724,18.0679574477091,2.41180908384498));
#98415=CARTESIAN_POINT('Ctrl Pts',(-9.43385349669055,18.0595689109437,2.46113747362027));
#98416=CARTESIAN_POINT('Ctrl Pts',(-9.31081622845497,18.0487959780189,2.54427290530359));
#98417=CARTESIAN_POINT('Ctrl Pts',(-9.28195077056037,18.0462223388745,2.56576533165001));
#98418=CARTESIAN_POINT('Ctrl Pts',(-9.2493763596898,18.043301450093,2.59242264683703));
#98419=CARTESIAN_POINT('Ctrl Pts',(-9.24467125780358,18.0428791414985,2.59633468771121));
#98420=CARTESIAN_POINT('Ctrl Pts',(-9.23747131009495,18.042232548807,2.60241658430765));
#98421=CARTESIAN_POINT('Ctrl Pts',(-9.23495484127171,18.0420064886057,2.60456050073622));
#98422=CARTESIAN_POINT('Ctrl Pts',(-9.23032998835346,18.0415909543789,2.60853439258517));
#98423=CARTESIAN_POINT('Ctrl Pts',(-9.22821908935006,18.0414012716774,2.61036126304491));
#98424=CARTESIAN_POINT('Ctrl Pts',(-9.22344137210073,18.0409718815143,2.61452592568277));
#98425=CARTESIAN_POINT('Ctrl Pts',(-9.22077860474996,18.0407325124069,2.61686826754653));
#98426=CARTESIAN_POINT('Ctrl Pts',(-9.21388371865778,18.0401124230115,2.6229889168206));
#98427=CARTESIAN_POINT('Ctrl Pts',(-9.20966818703791,18.0397330291611,2.6267858931517));
#98428=CARTESIAN_POINT('Ctrl Pts',(-9.18113316722225,18.0371616909793,2.6528636315379));
#98429=CARTESIAN_POINT('Ctrl Pts',(-9.15772900839733,18.0350365285971,2.67612929158634));
#98430=CARTESIAN_POINT('Ctrl Pts',(-9.11432945725783,18.030988903081,2.72305762052059));
#98431=CARTESIAN_POINT('Ctrl Pts',(-9.09423036443751,18.0290636359274,2.74658556799021));
#98432=CARTESIAN_POINT('Ctrl Pts',(-9.04517756726749,18.024154224547,2.8088110062958));
#98433=CARTESIAN_POINT('Ctrl Pts',(-9.01763740792034,18.0211858772441,2.84854643952578));
#98434=CARTESIAN_POINT('Ctrl Pts',(-8.9740473722929,18.0159255826458,2.92051673623503));
#98435=CARTESIAN_POINT('Ctrl Pts',(-8.95689005064501,18.013660006794,2.95200276185415));
#98436=CARTESIAN_POINT('Ctrl Pts',(-8.9345101546078,18.0103647898004,2.99794471395833));
#98437=CARTESIAN_POINT('Ctrl Pts',(-8.92809223527411,18.0093726298812,3.01179734528906));
#98438=CARTESIAN_POINT('Ctrl Pts',(-8.91854321951504,18.0078176407391,3.03350488337976));
#98439=CARTESIAN_POINT('Ctrl Pts',(-8.91522424931074,18.0072609513128,3.04127565292638));
#98440=CARTESIAN_POINT('Ctrl Pts',(-8.90915996787377,18.0062122130788,3.05590800999441));
#98441=CARTESIAN_POINT('Ctrl Pts',(-8.90639505427279,18.0057208380292,3.06276106098184));
#98442=CARTESIAN_POINT('Ctrl Pts',(-8.90182819942725,18.0048861333767,3.07439471923412));
#98443=CARTESIAN_POINT('Ctrl Pts',(-8.89999251528954,18.0045439359986,3.07916191858856));
#98444=CARTESIAN_POINT('Ctrl Pts',(-8.89638616142106,18.0038580111336,3.08871230149107));
#98445=CARTESIAN_POINT('Ctrl Pts',(-8.89461543377078,18.00351429434,3.0934953444588));
#98446=CARTESIAN_POINT('Ctrl Pts',(-8.89077204816991,18.0027526120407,3.10408781551743));
#98447=CARTESIAN_POINT('Ctrl Pts',(-8.88871385948728,18.0023341803633,3.1099022964317));
#98448=CARTESIAN_POINT('Ctrl Pts',(-8.88188040603884,18.0009081886493,3.12970015931277));
#98449=CARTESIAN_POINT('Ctrl Pts',(-8.87732282605005,17.9998935823307,3.14375664644724));
#98450=CARTESIAN_POINT('Ctrl Pts',(-8.84947384722369,17.9932549225941,3.23549719002195));
#98451=CARTESIAN_POINT('Ctrl Pts',(-8.8339992366159,17.9873794006879,3.31531145062842));
#98452=CARTESIAN_POINT('Ctrl Pts',(-8.82201795511681,17.9774156360952,3.45055094926967));
#98453=CARTESIAN_POINT('Ctrl Pts',(-8.82099223672586,17.9733857360215,3.50530786869955));
#98454=CARTESIAN_POINT('Ctrl Pts',(-8.82459799146867,17.9683057693371,3.57606490475995));
#98455=CARTESIAN_POINT('Ctrl Pts',(-8.82575125828175,17.9671582550904,3.59217211647325));
#98456=CARTESIAN_POINT('Ctrl Pts',(-8.82822615749851,17.9652680938578,3.61898448011892));
#98457=CARTESIAN_POINT('Ctrl Pts',(-8.82936421732331,17.9645177737649,3.62970400731036));
#98458=CARTESIAN_POINT('Ctrl Pts',(-8.83114385746329,17.9634891274718,3.64452538643236));
#98459=CARTESIAN_POINT('Ctrl Pts',(-8.83166014318969,17.96320440937,3.64864134542963));
#98460=CARTESIAN_POINT('Ctrl Pts',(-8.83257149048436,17.9627241501477,3.65560855462035));
#98461=CARTESIAN_POINT('Ctrl Pts',(-8.83295527475605,17.9625279938959,3.65846121625734));
#98462=CARTESIAN_POINT('Ctrl Pts',(-8.83371180018087,17.9621527273921,3.66393258842002));
#98463=CARTESIAN_POINT('Ctrl Pts',(-8.83408290843956,17.9619735240023,3.66655147715855));
#98464=CARTESIAN_POINT('Ctrl Pts',(-8.83499435631392,17.9615447809174,3.672831147619));
#98465=CARTESIAN_POINT('Ctrl Pts',(-8.8355431363475,17.9612957070293,3.67649070520377));
#98466=CARTESIAN_POINT('Ctrl Pts',(-8.83760061054857,17.9603936228668,3.68978355142038));
#98467=CARTESIAN_POINT('Ctrl Pts',(-8.8392117224147,17.9597460167709,3.69940091986435));
#98468=CARTESIAN_POINT('Ctrl Pts',(-8.85179995574672,17.9550745952236,3.7692126977654));
#98469=CARTESIAN_POINT('Ctrl Pts',(-8.86733522570546,17.951264765726,3.82849857782535));
#98470=CARTESIAN_POINT('Ctrl Pts',(-8.90936975260595,17.9433310961337,3.94955829604754));
#98471=CARTESIAN_POINT('Ctrl Pts',(-8.93668015428111,17.9392222398299,4.01081041564168));
#98472=CARTESIAN_POINT('Ctrl Pts',(-8.98583327531172,17.9327590883663,4.09980554772121));
#98473=CARTESIAN_POINT('Ctrl Pts',(-9.00395612056176,17.9305170872061,4.12944187064315));
#98474=CARTESIAN_POINT('Ctrl Pts',(-9.02845617085175,17.9276261289549,4.1657933513373));
#98475=CARTESIAN_POINT('Ctrl Pts',(-9.03363958136156,17.9270216858615,4.17329468451222));
#98476=CARTESIAN_POINT('Ctrl Pts',(-9.04210754609234,17.9260451771105,4.18525011799301));
#98477=CARTESIAN_POINT('Ctrl Pts',(-9.04533737582244,17.9256751889192,4.18974266917796));
#98478=CARTESIAN_POINT('Ctrl Pts',(-9.05154982945142,17.9249680956219,4.19825668870298));
#98479=CARTESIAN_POINT('Ctrl Pts',(-9.05452668289495,17.9246312174058,4.20228223289569));
#98480=CARTESIAN_POINT('Ctrl Pts',(-9.06139298720138,17.923858519254,4.21144462343235));
#98481=CARTESIAN_POINT('Ctrl Pts',(-9.06529907761628,17.9234220592209,4.2165687402572));
#98482=CARTESIAN_POINT('Ctrl Pts',(-9.07752836170236,17.9220649333365,4.23234131485983));
#98483=CARTESIAN_POINT('Ctrl Pts',(-9.08599269692799,17.9211387494539,4.24287842098226));
#98484=CARTESIAN_POINT('Ctrl Pts',(-9.15955641909835,17.9131954505821,4.33129583125409));
#98485=CARTESIAN_POINT('Ctrl Pts',(-9.23427979769553,17.905760754493,4.40058992540698));
#98486=CARTESIAN_POINT('Ctrl Pts',(-9.3641878541863,17.8940621894593,4.49307736083118));
#98487=CARTESIAN_POINT('Ctrl Pts',(-9.41386803130244,17.8898326686735,4.52318651582399));
#98488=CARTESIAN_POINT('Ctrl Pts',(-9.47201008195407,17.8852906914201,4.55279339532869));
#98489=CARTESIAN_POINT('Ctrl Pts',(-9.4784801191875,17.8847907278865,4.55601340298587));
#98490=CARTESIAN_POINT('Ctrl Pts',(-9.48815724486811,17.8840514858372,4.56071887956098));
#98491=CARTESIAN_POINT('Ctrl Pts',(-9.49134189391957,17.883809574113,4.56224972552698));
#98492=CARTESIAN_POINT('Ctrl Pts',(-9.49681268654569,17.883396399321,4.56484926538973));
#98493=CARTESIAN_POINT('Ctrl Pts',(-9.49909542239117,17.8832247125377,4.56592496686999));
#98494=CARTESIAN_POINT('Ctrl Pts',(-9.50428753921127,17.8828358368276,4.56835130310064));
#98495=CARTESIAN_POINT('Ctrl Pts',(-9.50719899096266,17.8826189262557,4.5696973949353));
#98496=CARTESIAN_POINT('Ctrl Pts',(-9.51513328454796,17.8820308243359,4.57332649784314));
#98497=CARTESIAN_POINT('Ctrl Pts',(-9.52016680589226,17.8816610141385,4.57558617112916));
#98498=CARTESIAN_POINT('Ctrl Pts',(-9.54521779952762,17.8798358578718,4.58662132805739));
#98499=CARTESIAN_POINT('Ctrl Pts',(-9.56546241528391,17.8784091906423,4.5948744200728));
#98500=CARTESIAN_POINT('Ctrl Pts',(-9.60659485582774,17.875583885374,4.61032197373736));
#98501=CARTESIAN_POINT('Ctrl Pts',(-9.62747841984632,17.8741862407253,4.61750179535646));
#98502=CARTESIAN_POINT('Ctrl Pts',(-9.7435267706381,17.8665587824645,4.65378437489958));
#98503=CARTESIAN_POINT('Ctrl Pts',(-9.84187762461019,17.8605657183773,4.67132177802412));
#98504=CARTESIAN_POINT('Ctrl Pts',(-9.96880000747504,17.8524211489929,4.67765942916407));
#98505=CARTESIAN_POINT('Ctrl Pts',(-9.99637362433313,17.8506302551485,4.67806698838191));
#98506=CARTESIAN_POINT('Ctrl Pts',(-10.0323825152056,17.8482514033899,4.67733505562131));
#98507=CARTESIAN_POINT('Ctrl Pts',(-10.0408282216877,17.8476905967024,4.67707243218723));
#98508=CARTESIAN_POINT('Ctrl Pts',(-10.0546525339866,17.8467676380317,4.67649359684837));
#98509=CARTESIAN_POINT('Ctrl Pts',(-10.0600331889625,17.8464071646814,4.6762313112127));
#98510=CARTESIAN_POINT('Ctrl Pts',(-10.0704569982453,17.8457063348852,4.67565148189664));
#98511=CARTESIAN_POINT('Ctrl Pts',(-10.0755002890819,17.8453661239302,4.67533837700627));
#98512=CARTESIAN_POINT('Ctrl Pts',(-10.087176663426,17.8445757591754,4.67453800543552));
#98513=CARTESIAN_POINT('Ctrl Pts',(-10.0938078919757,17.8441248767153,4.67402698993955));
#98514=CARTESIAN_POINT('Ctrl Pts',(-10.1154214384111,17.8426484962089,4.67217712532677));
#98515=CARTESIAN_POINT('Ctrl Pts',(-10.1303819706907,17.8416158864112,4.6706074606143));
#98516=CARTESIAN_POINT('Ctrl Pts',(-10.2258570069655,17.8349544951473,4.65873730688055));
#98517=CARTESIAN_POINT('Ctrl Pts',(-10.3051407104166,17.829074017416,4.64042454488854));
#98518=CARTESIAN_POINT('Ctrl Pts',(-10.4336401811532,17.8191051179038,4.59637726004835));
#98519=CARTESIAN_POINT('Ctrl Pts',(-10.4840863978927,17.8150752203405,4.57505713107841));
#98520=CARTESIAN_POINT('Ctrl Pts',(-10.5472687349049,17.8099952564642,4.54300176558728));
#98521=CARTESIAN_POINT('Ctrl Pts',(-10.5615165047143,17.8088477426083,4.5354008988032));
#98522=CARTESIAN_POINT('Ctrl Pts',(-10.5850079534667,17.8069575819491,4.52224113535079));
#98523=CARTESIAN_POINT('Ctrl Pts',(-10.5943393840663,17.8062072620444,4.51684411867589));
#98524=CARTESIAN_POINT('Ctrl Pts',(-10.6071577347474,17.8051786159641,4.50919361591435));
#98525=CARTESIAN_POINT('Ctrl Pts',(-10.6107084729582,17.8048938978903,4.50704887251629));
#98526=CARTESIAN_POINT('Ctrl Pts',(-10.6167037077458,17.8044136387012,4.50338421551919));
#98527=CARTESIAN_POINT('Ctrl Pts',(-10.6191540778376,17.8042174824549,4.50187403183936));
#98528=CARTESIAN_POINT('Ctrl Pts',(-10.6238455546558,17.8038422159507,4.49895884926265));
#98529=CARTESIAN_POINT('Ctrl Pts',(-10.6260874879379,17.803663012555,4.49755526983949));
#98530=CARTESIAN_POINT('Ctrl Pts',(-10.631454504557,17.8032342694416,4.49416998751971));
#98531=CARTESIAN_POINT('Ctrl Pts',(-10.6345750386283,17.802985195531,4.49218107051237));
#98532=CARTESIAN_POINT('Ctrl Pts',(-10.6458838994318,17.8020831111688,4.48489802796709));
#98533=CARTESIAN_POINT('Ctrl Pts',(-10.654016050262,17.8014355048987,4.47951679836229));
#98534=CARTESIAN_POINT('Ctrl Pts',(-10.7126834119856,17.7967641004027,4.43963883518299));
#98535=CARTESIAN_POINT('Ctrl Pts',(-10.76053578613,17.792954286246,4.40134682148313));
#98536=CARTESIAN_POINT('Ctrl Pts',(-10.8540574977807,17.7850206203113,4.31373387201843));
#98537=CARTESIAN_POINT('Ctrl Pts',(-10.8989204011498,17.7809117527647,4.26388383497586));
#98538=CARTESIAN_POINT('Ctrl Pts',(-10.9602525442296,17.7744485858551,4.18280004077958));
#98539=CARTESIAN_POINT('Ctrl Pts',(-10.9799636855964,17.7722065812215,4.15419542725544));
#98540=CARTESIAN_POINT('Ctrl Pts',(-11.0032180383216,17.7693156190491,4.11703465567986));
#98541=CARTESIAN_POINT('Ctrl Pts',(-11.0079647995188,17.7687111756595,4.10924966468374));
#98542=CARTESIAN_POINT('Ctrl Pts',(-11.0154460157162,17.7677346665446,4.09665322142751));
#98543=CARTESIAN_POINT('Ctrl Pts',(-11.0182378460213,17.7673646782883,4.09187613959951));
#98544=CARTESIAN_POINT('Ctrl Pts',(-11.0234915783654,17.7666575849425,4.08273932280643));
#98545=CARTESIAN_POINT('Ctrl Pts',(-11.025959549915,17.7663207067433,4.07838320336483));
#98546=CARTESIAN_POINT('Ctrl Pts',(-11.031539899148,17.7655480087373,4.06838544415476));
#98547=CARTESIAN_POINT('Ctrl Pts',(-11.0346338828214,17.7651115488339,4.06273377569896));
#98548=CARTESIAN_POINT('Ctrl Pts',(-11.0440737868741,17.7637544237597,4.04514920178676));
#98549=CARTESIAN_POINT('Ctrl Pts',(-11.0502605992841,17.7628282405671,4.03313260241117));
#98550=CARTESIAN_POINT('Ctrl Pts',(-11.1011424803266,17.7548849371542,3.92998072691506));
#98551=CARTESIAN_POINT('Ctrl Pts',(-11.1340807275815,17.7474502350925,3.83354244262143));
#98552=CARTESIAN_POINT('Ctrl Pts',(-11.1657786386585,17.7357516688753,3.67725656013453));
#98553=CARTESIAN_POINT('Ctrl Pts',(-11.1730944875407,17.7315221526145,3.61962711772648));
#98554=CARTESIAN_POINT('Ctrl Pts',(-11.1765118980603,17.7269801796391,3.55447054712337));
#98555=CARTESIAN_POINT('Ctrl Pts',(-11.1768239908109,17.7264802162248,3.54725026979736));
#98556=CARTESIAN_POINT('Ctrl Pts',(-11.1771897000827,17.7257409743167,3.53649599231491));
#98557=CARTESIAN_POINT('Ctrl Pts',(-11.1772938969083,17.7254990626158,3.53296404956283));
#98558=CARTESIAN_POINT('Ctrl Pts',(-11.1774452594416,17.7250858878498,3.52690894722474));
#98559=CARTESIAN_POINT('Ctrl Pts',(-11.1775002128651,17.7249142010694,3.52438605274794));
#98560=CARTESIAN_POINT('Ctrl Pts',(-11.1776066004691,17.724525325347,3.51865596824399));
#98561=CARTESIAN_POINT('Ctrl Pts',(-11.1776530422394,17.72430841476,3.51544873280664));
#98562=CARTESIAN_POINT('Ctrl Pts',(-11.1777437268435,17.723720312759,3.50672433023728));
#98563=CARTESIAN_POINT('Ctrl Pts',(-11.1777623058643,17.7233505024961,3.50120689186058));
#98564=CARTESIAN_POINT('Ctrl Pts',(-11.1776621165944,17.7215253453811,3.47383322505357));
#98565=CARTESIAN_POINT('Ctrl Pts',(-11.1769737301889,17.7200986774005,3.45198180320903));
#98566=CARTESIAN_POINT('Ctrl Pts',(-11.1743682783242,17.7172733715659,3.4081216043102));
#98567=CARTESIAN_POINT('Ctrl Pts',(-11.1724395695005,17.7158757270746,3.3861226709214));
#98568=CARTESIAN_POINT('Ctrl Pts',(-11.1584188701966,17.7082482678743,3.26534573099039));
#98569=CARTESIAN_POINT('Ctrl Pts',(-11.1344649935851,17.7022552026835,3.16835776015286));
#98570=CARTESIAN_POINT('Ctrl Pts',(-11.0886647295067,17.6941106334478,3.04981750809907));
#98571=CARTESIAN_POINT('Ctrl Pts',(-11.0778291336374,17.6923197411514,3.02445890077501));
#98572=CARTESIAN_POINT('Ctrl Pts',(-11.0625237048422,17.6899408911618,2.99185647983035));
#98573=CARTESIAN_POINT('Ctrl Pts',(-11.0588507913954,17.6893800846437,2.98424671031694));
#98574=CARTESIAN_POINT('Ctrl Pts',(-11.0527027005779,17.6884571261806,2.97185124530459));
#98575=CARTESIAN_POINT('Ctrl Pts',(-11.0502759606193,17.6880966528669,2.96704175792726));
#98576=CARTESIAN_POINT('Ctrl Pts',(-11.0455091786332,17.6873958230908,2.95775360500639));
#98577=CARTESIAN_POINT('Ctrl Pts',(-11.0431731366546,17.687055612119,2.95327301047068));
#98578=CARTESIAN_POINT('Ctrl Pts',(-11.0376957167169,17.68626524725,2.94293007944702));
#98579=CARTESIAN_POINT('Ctrl Pts',(-11.0345333943406,17.6858143646916,2.93707909106465));
#98580=CARTESIAN_POINT('Ctrl Pts',(-11.024057880102,17.6843379835284,2.91808352830516));
#98581=CARTESIAN_POINT('Ctrl Pts',(-11.0165426558326,17.6833053731633,2.9050526794377));
#98582=CARTESIAN_POINT('Ctrl Pts',(-10.9668893240913,17.6766440032917,2.82264594396539));
#98583=CARTESIAN_POINT('Ctrl Pts',(-10.9179310513474,17.670763549706,2.75765134264615));
#98584=CARTESIAN_POINT('Ctrl Pts',(-10.8254550731689,17.6607946563338,2.65815033908663));
#98585=CARTESIAN_POINT('Ctrl Pts',(-10.7854704139677,17.6567647405241,2.62072545196242));
#98586=CARTESIAN_POINT('Ctrl Pts',(-10.7305004157303,17.6516847562364,2.57602765458157));
#98587=CARTESIAN_POINT('Ctrl Pts',(-10.7177644055167,17.6505372395401,2.56609954184605));
#98588=CARTESIAN_POINT('Ctrl Pts',(-10.6961921052441,17.6486470747133,2.54998536988366));
#98589=CARTESIAN_POINT('Ctrl Pts',(-10.6874680506366,17.6478967534409,2.54365333434536));
#98590=CARTESIAN_POINT('Ctrl Pts',(-10.6752677240596,17.6468681058139,2.53505141580833));
#98591=CARTESIAN_POINT('Ctrl Pts',(-10.6718648660031,17.6465833875367,2.53267902305687));
#98592=CARTESIAN_POINT('Ctrl Pts',(-10.6660796942342,17.6461031281056,2.52869099250927));
#98593=CARTESIAN_POINT('Ctrl Pts',(-10.6637038829593,17.6459069718193,2.52706603331727));
#98594=CARTESIAN_POINT('Ctrl Pts',(-10.6591334250081,17.6455317053185,2.52396455667966));
#98595=CARTESIAN_POINT('Ctrl Pts',(-10.6569397392817,17.6453525019657,2.5224867070541));
#98596=CARTESIAN_POINT('Ctrl Pts',(-10.651665181763,17.6449237590594,2.51895910061311));
#98597=CARTESIAN_POINT('Ctrl Pts',(-10.6485795678827,17.644674685312,2.51691643262635));
#98598=CARTESIAN_POINT('Ctrl Pts',(-10.6373285815162,17.6437726024014,2.50954433928428));
#98599=CARTESIAN_POINT('Ctrl Pts',(-10.6291064596758,17.6431249973965,2.5043016449291));
#98600=CARTESIAN_POINT('Ctrl Pts',(-10.5688230838811,17.6384534685661,2.46690788475853));
#98601=CARTESIAN_POINT('Ctrl Pts',(-10.5143845816141,17.6346435425509,2.43875096703978));
#98602=CARTESIAN_POINT('Ctrl Pts',(-10.3963210566087,17.6267098499502,2.38891653997269));
#98603=CARTESIAN_POINT('Ctrl Pts',(-10.3325406240363,17.6226010643856,2.36819041117671));
#98604=CARTESIAN_POINT('Ctrl Pts',(-10.2335292170158,17.6161380101065,2.34511259373766));
#98605=CARTESIAN_POINT('Ctrl Pts',(-10.1993825809055,17.6138960308008,2.33873041866766));
#98606=CARTESIAN_POINT('Ctrl Pts',(-10.1559783205597,17.6110050972218,2.33258877783548));
#98607=CARTESIAN_POINT('Ctrl Pts',(-10.1469360642581,17.6104006559921,2.3314162488708));
#98608=CARTESIAN_POINT('Ctrl Pts',(-10.1323862872003,17.6094241495307,2.32970108589526));
#98609=CARTESIAN_POINT('Ctrl Pts',(-10.1268868477128,17.6090541617477,2.32909206019663));
#98610=CARTESIAN_POINT('Ctrl Pts',(-10.1164033813455,17.6083470687559,2.32800580967398));
#98611=CARTESIAN_POINT('Ctrl Pts',(-10.1114201907177,17.6080101904338,2.32752156987279));
#98612=CARTESIAN_POINT('Ctrl Pts',(-10.1000173315549,17.6072374913649,2.32648685127655));
#98613=CARTESIAN_POINT('Ctrl Pts',(-10.093595976871,17.6068010305153,2.32595725500094));
#98614=CARTESIAN_POINT('Ctrl Pts',(-10.0736924512961,17.6054438995328,2.32448005154252));
#98615=CARTESIAN_POINT('Ctrl Pts',(-10.0601984856706,17.6045177113087,2.32371183698976));
#98616=CARTESIAN_POINT('Ctrl Pts',(-9.96781450314467,17.598132555985,2.32004616711968));
#98617=CARTESIAN_POINT('Ctrl Pts',(-9.88888725891994,17.5924370348984,2.32485788425224));
#98618=CARTESIAN_POINT('Ctrl Pts',(-9.81110406371068,17.5866589100326,2.3374969300026));
#98619=CARTESIAN_POINT('Ctrl Pts',(-9.81110409010019,17.488629053511,2.33749692571455));
#98620=CARTESIAN_POINT('Ctrl Pts',(-9.83100301365312,17.4900789605701,2.3342635361832));
#98621=CARTESIAN_POINT('Ctrl Pts',(-9.85098889505721,17.4915145218242,2.33154042954652));
#98622=CARTESIAN_POINT('Ctrl Pts',(-9.88075068876469,17.4936127359325,2.32826194785942));
#98623=CARTESIAN_POINT('Ctrl Pts',(-9.89047251007087,17.4942918938412,2.3273132534345));
#98624=CARTESIAN_POINT('Ctrl Pts',(-9.90389375181683,17.4952199036933,2.32617192319059));
#98625=CARTESIAN_POINT('Ctrl Pts',(-9.90758362860465,17.4954740422306,2.32587565391234));
#98626=CARTESIAN_POINT('Ctrl Pts',(-9.91391216649941,17.4959081385477,2.32539753862048));
#98627=CARTESIAN_POINT('Ctrl Pts',(-9.91655012696285,17.4960885559782,2.32520717724369));
#98628=CARTESIAN_POINT('Ctrl Pts',(-9.92205868388094,17.4964641654574,2.32482831497533));
#98629=CARTESIAN_POINT('Ctrl Pts',(-9.92492935769447,17.4966592594639,2.32464144324194));
#98630=CARTESIAN_POINT('Ctrl Pts',(-9.93193637675553,17.4971339443372,2.32421108445177));
#98631=CARTESIAN_POINT('Ctrl Pts',(-9.93607343056122,17.4974129151901,2.32397890080429));
#98632=CARTESIAN_POINT('Ctrl Pts',(-9.95095149768667,17.4984118161063,2.32322264291081));
#98633=CARTESIAN_POINT('Ctrl Pts',(-9.96169873869972,17.4991252105098,2.32282382908586));
#98634=CARTESIAN_POINT('Ctrl Pts',(-9.98854273719769,17.5008900864926,2.3221957298625));
#98635=CARTESIAN_POINT('Ctrl Pts',(-10.0046419522436,17.5019332897364,2.32214912920342));
#98636=CARTESIAN_POINT('Ctrl Pts',(-10.0751296890812,17.5064535852282,2.32339047285294));
#98637=CARTESIAN_POINT('Ctrl Pts',(-10.1293942273352,17.5098126276164,2.32811582350615));
#98638=CARTESIAN_POINT('Ctrl Pts',(-10.2637115757156,17.518217883783,2.34925949867592));
#98639=CARTESIAN_POINT('Ctrl Pts',(-10.3427361778212,17.5232598028131,2.37027556711188));
#98640=CARTESIAN_POINT('Ctrl Pts',(-10.4329982674911,17.5295589068715,2.40463090521283));
#98641=CARTESIAN_POINT('Ctrl Pts',(-10.4469406957582,17.5305472838744,2.41024547053482));
#98642=CARTESIAN_POINT('Ctrl Pts',(-10.4668889245423,17.5319855958489,2.41872575977277));
#98643=CARTESIAN_POINT('Ctrl Pts',(-10.4729842445534,17.5324283848964,2.42137812380982));
#98644=CARTESIAN_POINT('Ctrl Pts',(-10.48367102806,17.5332107086682,2.42613645535825));
#98645=CARTESIAN_POINT('Ctrl Pts',(-10.4882720471708,17.5335494984627,2.42822064654809));
#98646=CARTESIAN_POINT('Ctrl Pts',(-10.497750861408,17.5342516183721,2.43258810772595));
#98647=CARTESIAN_POINT('Ctrl Pts',(-10.5026266780322,17.5346150785005,2.43487536472795));
#98648=CARTESIAN_POINT('Ctrl Pts',(-10.51511086392,17.5355517035034,2.44083653568251));
#98649=CARTESIAN_POINT('Ctrl Pts',(-10.5226955873581,17.5361265263251,2.44455897239597));
#98650=CARTESIAN_POINT('Ctrl Pts',(-10.5548654137709,17.5385898402272,2.46077911703653));
#98651=CARTESIAN_POINT('Ctrl Pts',(-10.5790457141355,17.5405051338542,2.47405579497926));
#98652=CARTESIAN_POINT('Ctrl Pts',(-10.6882005363853,17.5494572057466,2.53907800328941));
#98653=CARTESIAN_POINT('Ctrl Pts',(-10.7668617734872,17.5568372297759,2.6006067872924));
#98654=CARTESIAN_POINT('Ctrl Pts',(-10.8523854214365,17.5656962387672,2.68696724661909));
#98655=CARTESIAN_POINT('Ctrl Pts',(-10.8674873018161,17.5672961810296,2.70310035784563));
#98656=CARTESIAN_POINT('Ctrl Pts',(-10.8966202717766,17.5704412699039,2.73603297017059));
#98657=CARTESIAN_POINT('Ctrl Pts',(-10.9106554197756,17.5719862294634,2.75281836830902));
#98658=CARTESIAN_POINT('Ctrl Pts',(-10.9276358720918,17.5738840726602,2.77431605024232));
#98659=CARTESIAN_POINT('Ctrl Pts',(-10.9310254881816,17.5742644213776,2.77866994414256));
#98660=CARTESIAN_POINT('Ctrl Pts',(-10.9363366669054,17.5748625778322,2.7855918582262));
#98661=CARTESIAN_POINT('Ctrl Pts',(-10.9382785002935,17.5750817432182,2.78814411336615));
#98662=CARTESIAN_POINT('Ctrl Pts',(-10.9417291026675,17.5754719965999,2.79271807397449));
#98663=CARTESIAN_POINT('Ctrl Pts',(-10.9432417938916,17.5756433519171,2.79473668454327));
#98664=CARTESIAN_POINT('Ctrl Pts',(-10.9468565946784,17.5760535124572,2.79959288855108));
#98665=CARTESIAN_POINT('Ctrl Pts',(-10.9489524398623,17.5762918854726,2.80243509237313));
#98666=CARTESIAN_POINT('Ctrl Pts',(-10.9552941345106,17.5770150370864,2.81111662617358));
#98667=CARTESIAN_POINT('Ctrl Pts',(-10.959499200563,17.5774971330373,2.8169857419205));
#98668=CARTESIAN_POINT('Ctrl Pts',(-10.9968899294645,17.5818111349828,2.8701997830073));
#98669=CARTESIAN_POINT('Ctrl Pts',(-11.0266060303766,17.5854383689854,2.91989673982626));
#98670=CARTESIAN_POINT('Ctrl Pts',(-11.0982026866433,17.5953431592931,3.06250989536388));
#98671=CARTESIAN_POINT('Ctrl Pts',(-11.1318724228655,17.6015370310837,3.15895819132559));
#98672=CARTESIAN_POINT('Ctrl Pts',(-11.1554945585162,17.6090712219406,3.27172571190887));
#98673=CARTESIAN_POINT('Ctrl Pts',(-11.1580318344068,17.609959452956,3.28496727807221));
#98674=CARTESIAN_POINT('Ctrl Pts',(-11.1614435802468,17.6112822237581,3.30458943678742));
#98675=CARTESIAN_POINT('Ctrl Pts',(-11.1624939908945,17.6117112391158,3.31093864309729));
#98676=CARTESIAN_POINT('Ctrl Pts',(-11.164268610167,17.6124767757069,3.32223974347204));
#98677=CARTESIAN_POINT('Ctrl Pts',(-11.1650133967928,17.6128126426386,3.3271882834147));
#98678=CARTESIAN_POINT('Ctrl Pts',(-11.1665153492769,17.6135220308798,3.33761888103181));
#98679=CARTESIAN_POINT('Ctrl Pts',(-11.1672654564537,17.6138957646291,3.3431018156406));
#98680=CARTESIAN_POINT('Ctrl Pts',(-11.1691503335468,17.614889171436,3.35764173560786));
#98681=CARTESIAN_POINT('Ctrl Pts',(-11.1702184834608,17.6155109064793,3.36670682437764));
#98682=CARTESIAN_POINT('Ctrl Pts',(-11.1748587628557,17.6185237424583,3.41045781029342));
#98683=CARTESIAN_POINT('Ctrl Pts',(-11.1769943377901,17.6209588630255,3.44527516423312));
#98684=CARTESIAN_POINT('Ctrl Pts',(-11.1787204378722,17.6282289792381,3.54758692397761));
#98685=CARTESIAN_POINT('Ctrl Pts',(-11.1740604166206,17.6331734412647,3.61500709026996));
#98686=CARTESIAN_POINT('Ctrl Pts',(-11.1543282571356,17.6425670100796,3.74141248401991));
#98687=CARTESIAN_POINT('Ctrl Pts',(-11.1404080268727,17.6469982779299,3.80037434751222));
#98688=CARTESIAN_POINT('Ctrl Pts',(-11.1190475394232,17.6519225596224,3.86731884001591));
#98689=CARTESIAN_POINT('Ctrl Pts',(-11.1159616712497,17.6526019510228,3.87659008164399));
#98690=CARTESIAN_POINT('Ctrl Pts',(-11.1115478807817,17.6535302197006,3.8893200183388));
#98691=CARTESIAN_POINT('Ctrl Pts',(-11.1103185980832,17.6537843874583,3.89281214292862));
#98692=CARTESIAN_POINT('Ctrl Pts',(-11.1081828754445,17.6542185206477,3.89878913289576));
#98693=CARTESIAN_POINT('Ctrl Pts',(-11.1072845034902,17.6543989458981,3.90127682044788));
#98694=CARTESIAN_POINT('Ctrl Pts',(-11.1053915689052,17.6547745568874,3.90646379529479));
#98695=CARTESIAN_POINT('Ctrl Pts',(-11.1043954877064,17.6549696446587,3.90916249151669));
#98696=CARTESIAN_POINT('Ctrl Pts',(-11.1019407322483,17.6554442902252,3.91573891956883));
#98697=CARTESIAN_POINT('Ctrl Pts',(-11.1004714467144,17.6557232282513,3.91961270583306));
#98698=CARTESIAN_POINT('Ctrl Pts',(-11.0951162488188,17.6567218789063,3.93351013249099));
#98699=CARTESIAN_POINT('Ctrl Pts',(-11.091113437866,17.6574350601812,3.94348857858813));
#98700=CARTESIAN_POINT('Ctrl Pts',(-11.0807799763132,17.6591993020098,3.96826125033395));
#98701=CARTESIAN_POINT('Ctrl Pts',(-11.0742815793299,17.6602420918645,3.98298353796955));
#98702=CARTESIAN_POINT('Ctrl Pts',(-11.0445176067774,17.6647594365688,4.04683911368431));
#98703=CARTESIAN_POINT('Ctrl Pts',(-11.0181665328738,17.6681160982642,4.09446437806296));
#98704=CARTESIAN_POINT('Ctrl Pts',(-10.9442595016032,17.6765221875922,4.20861150329932));
#98705=CARTESIAN_POINT('Ctrl Pts',(-10.8929064076063,17.681567221353,4.27231619189542));
#98706=CARTESIAN_POINT('Ctrl Pts',(-10.8247907581365,17.6878697503554,4.34085736850886));
#98707=CARTESIAN_POINT('Ctrl Pts',(-10.8139947267556,17.6888580315085,4.35131278638133));
#98708=CARTESIAN_POINT('Ctrl Pts',(-10.7981394080436,17.6902962289978,4.36609048736872));
#98709=CARTESIAN_POINT('Ctrl Pts',(-10.7932386358898,17.6907390010232,4.37058124863062));
#98710=CARTESIAN_POINT('Ctrl Pts',(-10.784547438861,17.6915213049355,4.37841100382307));
#98711=CARTESIAN_POINT('Ctrl Pts',(-10.7807730234685,17.6918600920117,4.38176757704264));
#98712=CARTESIAN_POINT('Ctrl Pts',(-10.772929690456,17.6925622162733,4.3886527795038));
#98713=CARTESIAN_POINT('Ctrl Pts',(-10.768857932976,17.692925683533,4.39217797895977));
#98714=CARTESIAN_POINT('Ctrl Pts',(-10.7583364824705,17.6938623481199,4.40116160239636));
#98715=CARTESIAN_POINT('Ctrl Pts',(-10.7518520618635,17.6944372036648,4.40657869204485));
#98716=CARTESIAN_POINT('Ctrl Pts',(-10.72395223163,17.6969008580603,4.42938102178373));
#98717=CARTESIAN_POINT('Ctrl Pts',(-10.7019894620115,17.6988164687031,4.44607953806297));
#98718=CARTESIAN_POINT('Ctrl Pts',(-10.5982105487315,17.7077686675846,4.51937948486913));
#98719=CARTESIAN_POINT('Ctrl Pts',(-10.5100227813261,17.7151484523054,4.56623694702003));
#98720=CARTESIAN_POINT('Ctrl Pts',(-10.3963578405525,17.724007235648,4.60927167305125));
#98721=CARTESIAN_POINT('Ctrl Pts',(-10.3754786773837,17.7256072038414,4.61651199678875));
#98722=CARTESIAN_POINT('Ctrl Pts',(-10.3335491836262,17.7287521575637,4.62974261753465));
#98723=CARTESIAN_POINT('Ctrl Pts',(-10.3125101311386,17.7302969606698,4.63574249173964));
#98724=CARTESIAN_POINT('Ctrl Pts',(-10.2859686582685,17.7321946402533,4.64251802201019));
#98725=CARTESIAN_POINT('Ctrl Pts',(-10.2806130525153,17.7325749763162,4.64384519139927));
#98726=CARTESIAN_POINT('Ctrl Pts',(-10.272130118479,17.7331731173264,4.64588417615998));
#98727=CARTESIAN_POINT('Ctrl Pts',(-10.2690089540329,17.733392279809,4.64662091810303));
#98728=CARTESIAN_POINT('Ctrl Pts',(-10.2634273508521,17.7337825307372,4.64791439426082));
#98729=CARTESIAN_POINT('Ctrl Pts',(-10.2609681454332,17.733953886483,4.64847596969939));
#98730=CARTESIAN_POINT('Ctrl Pts',(-10.2550618243977,17.7343640515367,4.64980476552377));
#98731=CARTESIAN_POINT('Ctrl Pts',(-10.2516130426483,17.7346024286095,4.65056438788727));
#98732=CARTESIAN_POINT('Ctrl Pts',(-10.2411029528239,17.7353256049204,4.65282980390785));
#98733=CARTESIAN_POINT('Ctrl Pts',(-10.2340310069864,17.7358077212436,4.65428622311128));
#98734=CARTESIAN_POINT('Ctrl Pts',(-10.1702020632865,17.7401224557555,4.66682061627781));
#98735=CARTESIAN_POINT('Ctrl Pts',(-10.1127061331978,17.7437503259744,4.67377097876649));
#98736=CARTESIAN_POINT('Ctrl Pts',(-9.9533067913942,17.7536548608026,4.68121276757545));
#98737=CARTESIAN_POINT('Ctrl Pts',(-9.85151409422792,17.7598479378296,4.67277182673046));
#98738=CARTESIAN_POINT('Ctrl Pts',(-9.7388927515219,17.7673812998558,4.64852073522732));
#98739=CARTESIAN_POINT('Ctrl Pts',(-9.72576130862969,17.7682696488174,4.64545623671794));
#98740=CARTESIAN_POINT('Ctrl Pts',(-9.70644438518839,17.7695925619886,4.6405970295336));
#98741=CARTESIAN_POINT('Ctrl Pts',(-9.70021605251052,17.7700216000187,4.63897588421517));
#98742=CARTESIAN_POINT('Ctrl Pts',(-9.68916894814907,17.7707871620305,4.63600359288551));
#98743=CARTESIAN_POINT('Ctrl Pts',(-9.6843448752707,17.7711230315515,4.63467261655085));
#98744=CARTESIAN_POINT('Ctrl Pts',(-9.67420446039413,17.7718324097526,4.63180517414995));
#98745=CARTESIAN_POINT('Ctrl Pts',(-9.66889018547529,17.7722061307756,4.63026190538948));
#98746=CARTESIAN_POINT('Ctrl Pts',(-9.654840429857,17.7731994673369,4.62607425762651));
#98747=CARTESIAN_POINT('Ctrl Pts',(-9.64612461963399,17.7738211443404,4.62336573276506));
#98748=CARTESIAN_POINT('Ctrl Pts',(-9.60427538744889,17.7768332120943,4.60982531482011));
#98749=CARTESIAN_POINT('Ctrl Pts',(-9.57160548376597,17.7792675951414,4.59762830670265));
#98750=CARTESIAN_POINT('Ctrl Pts',(-9.47746717023381,17.7865343204172,4.55763931968686));
#98751=CARTESIAN_POINT('Ctrl Pts',(-9.41779193248447,17.7914759972255,4.52599871519401));
#98752=CARTESIAN_POINT('Ctrl Pts',(-9.31029961705549,17.8008706988156,4.45659463956577));
#98753=CARTESIAN_POINT('Ctrl Pts',(-9.2620434936724,17.8053058647758,4.4198813094071));
#98754=CARTESIAN_POINT('Ctrl Pts',(-9.20952512712368,17.8102335552744,4.37312081382293));
#98755=CARTESIAN_POINT('Ctrl Pts',(-9.20231042653558,17.810912782223,4.36653438484952));
#98756=CARTESIAN_POINT('Ctrl Pts',(-9.19247559551547,17.8118408686077,4.35732905113829));
#98757=CARTESIAN_POINT('Ctrl Pts',(-9.189784864574,17.8120950157868,4.35478664064329));
#98758=CARTESIAN_POINT('Ctrl Pts',(-9.18519230823482,17.8125291230087,4.35040606945743));
#98759=CARTESIAN_POINT('Ctrl Pts',(-9.18328462643254,17.8127095427518,4.34857413138883));
#98760=CARTESIAN_POINT('Ctrl Pts',(-9.17931492594872,17.8130851526769,4.34473625890503));
#98761=CARTESIAN_POINT('Ctrl Pts',(-9.17725406525659,17.8132802448388,4.3427291765336));
#98762=CARTESIAN_POINT('Ctrl Pts',(-9.1722429370047,17.8137549180848,4.33781291120564));
#98763=CARTESIAN_POINT('Ctrl Pts',(-9.16930058981419,17.8140338792273,4.33489563463749));
#98764=CARTESIAN_POINT('Ctrl Pts',(-9.15877793866159,17.8150327061094,4.32435194331321));
#98765=CARTESIAN_POINT('Ctrl Pts',(-9.15128648566064,17.8157460374631,4.31663705141727));
#98766=CARTESIAN_POINT('Ctrl Pts',(-9.13284831473239,17.8175107258375,4.29712110728238));
#98767=CARTESIAN_POINT('Ctrl Pts',(-9.12203560278236,17.8185538067823,4.28519594756363));
#98768=CARTESIAN_POINT('Ctrl Pts',(-9.0757707842038,17.8230732291185,4.23202015213303));
#98769=CARTESIAN_POINT('Ctrl Pts',(-9.04295362409234,17.8264315670303,4.18856105035524));
#98770=CARTESIAN_POINT('Ctrl Pts',(-8.96871867297762,17.8348370694959,4.07463807381245));
#98771=CARTESIAN_POINT('Ctrl Pts',(-8.93140846709869,17.8398799100686,4.00185666486987));
#98772=CARTESIAN_POINT('Ctrl Pts',(-8.8964852328384,17.8461800275,3.91179618620671));
#98773=CARTESIAN_POINT('Ctrl Pts',(-8.89132043108675,17.8471683762383,3.89768143072672));
#98774=CARTESIAN_POINT('Ctrl Pts',(-8.88426296525698,17.8486066544528,3.8771871136755));
#98775=CARTESIAN_POINT('Ctrl Pts',(-8.88215190194974,17.8490494384809,3.87088391183506));
#98776=CARTESIAN_POINT('Ctrl Pts',(-8.87853082787826,17.8498317563965,3.85976029762559));
#98777=CARTESIAN_POINT('Ctrl Pts',(-8.87699824556304,17.8501705453894,3.85494736784152));
#98778=CARTESIAN_POINT('Ctrl Pts',(-8.87389561863522,17.850872666582,3.84498259434082));
#98779=CARTESIAN_POINT('Ctrl Pts',(-8.8723298606941,17.8512361288131,3.83982955047714));
#98780=CARTESIAN_POINT('Ctrl Pts',(-8.86839867114451,17.8521727654874,3.82656527856838));
#98781=CARTESIAN_POINT('Ctrl Pts',(-8.86608511506236,17.8527475979576,3.81843912427729));
#98782=CARTESIAN_POINT('Ctrl Pts',(-8.85659292161595,17.8552110122498,3.78368291579778));
#98783=CARTESIAN_POINT('Ctrl Pts',(-8.85026399791373,17.8571263993441,3.75683194695721));
#98784=CARTESIAN_POINT('Ctrl Pts',(-8.82547504892722,17.8660785086723,3.63221953184762));
#98785=CARTESIAN_POINT('Ctrl Pts',(-8.81850841326093,17.8734584621393,3.53259700562935));
#98786=CARTESIAN_POINT('Ctrl Pts',(-8.82539079220619,17.8823174045946,3.41125103427278));
#98787=CARTESIAN_POINT('Ctrl Pts',(-8.82726231850258,17.8839173545011,3.3892318002248));
#98788=CARTESIAN_POINT('Ctrl Pts',(-8.83221722202826,17.8870624035309,3.34554324231802));
#98789=CARTESIAN_POINT('Ctrl Pts',(-8.83528736489175,17.8886073169667,3.32388034180067));
#98790=CARTESIAN_POINT('Ctrl Pts',(-8.83988551679018,17.8905051119292,3.29687469043616));
#98791=CARTESIAN_POINT('Ctrl Pts',(-8.84084987028902,17.8908854569161,3.29144188980268));
#98792=CARTESIAN_POINT('Ctrl Pts',(-8.84243505093976,17.8914836088178,3.28286240433153));
#98793=CARTESIAN_POINT('Ctrl Pts',(-8.84303059665384,17.8917027733479,3.27971121887302));
#98794=CARTESIAN_POINT('Ctrl Pts',(-8.84411758018409,17.8920930260063,3.27408573027796));
#98795=CARTESIAN_POINT('Ctrl Pts',(-8.84460409318003,17.8922643814498,3.27161058608846));
#98796=CARTESIAN_POINT('Ctrl Pts',(-8.8457907818495,17.8926745433203,3.26567412964432));
#98797=CARTESIAN_POINT('Ctrl Pts',(-8.8464985764386,17.8929129175318,3.26221438344126));
#98798=CARTESIAN_POINT('Ctrl Pts',(-8.84859499979282,17.8936013404536,3.25219660451945));
#98799=CARTESIAN_POINT('Ctrl Pts',(-8.85002409727888,17.8940491928382,3.24564704510706));
#98800=CARTESIAN_POINT('Ctrl Pts',(-8.85350442342808,17.8950923553245,3.23032594889763));
#98801=CARTESIAN_POINT('Ctrl Pts',(-8.85560054263727,17.8956854080969,3.22156491954854));
#98802=CARTESIAN_POINT('Ctrl Pts',(-8.86307390784598,17.8976884382318,3.19184017313714));
#98803=CARTESIAN_POINT('Ctrl Pts',(-8.86892860749372,17.8990773229491,3.17099993999344));
#98804=CARTESIAN_POINT('Ctrl Pts',(-8.90182298871254,17.9061035945119,3.06520107757154));
#98805=CARTESIAN_POINT('Ctrl Pts',(-8.93787215315909,17.9114785743262,2.98334822380961));
#98806=CARTESIAN_POINT('Ctrl Pts',(-9.00576424095308,17.9199490216924,2.86702028851143));
#98807=CARTESIAN_POINT('Ctrl Pts',(-9.03097260801836,17.9228610952238,2.8290654022077));
#98808=CARTESIAN_POINT('Ctrl Pts',(-9.06439584052988,17.9265223527975,2.78456829284754));
#98809=CARTESIAN_POINT('Ctrl Pts',(-9.07058353047192,17.9271926022561,2.77654807592051));
#98810=CARTESIAN_POINT('Ctrl Pts',(-9.08048340227842,17.9282538131056,2.76405293998726));
#98811=CARTESIAN_POINT('Ctrl Pts',(-9.08412667999263,17.9286420576485,2.75952386380646));
#98812=CARTESIAN_POINT('Ctrl Pts',(-9.09091672521467,17.9293615443689,2.75120971618725));
#98813=CARTESIAN_POINT('Ctrl Pts',(-9.09405399762396,17.9296924013955,2.74741702840094));
#98814=CARTESIAN_POINT('Ctrl Pts',(-9.10107033368193,17.9304289446411,2.7390423411306));
#98815=CARTESIAN_POINT('Ctrl Pts',(-9.10496082191933,17.9308350889041,2.73447013711857));
#98816=CARTESIAN_POINT('Ctrl Pts',(-9.11578866546422,17.9319594032683,2.72194034514354));
#98817=CARTESIAN_POINT('Ctrl Pts',(-9.12279817762902,17.9326805223891,2.71404614586901));
#98818=CARTESIAN_POINT('Ctrl Pts',(-9.16898357371708,17.9373902989777,2.66341912299944));
#98819=CARTESIAN_POINT('Ctrl Pts',(-9.21115707305582,17.9415062888095,2.62354074563825));
#98820=CARTESIAN_POINT('Ctrl Pts',(-9.29204882337571,17.9490735359289,2.55763502943807));
#98821=CARTESIAN_POINT('Ctrl Pts',(-9.32970741111362,17.9524854535245,2.53048768757376));
#98822=CARTESIAN_POINT('Ctrl Pts',(-9.38108647417725,17.9569508411352,2.49787696078741));
#98823=CARTESIAN_POINT('Ctrl Pts',(-9.39344825642823,17.9580114744876,2.49034682639707));
#98824=CARTESIAN_POINT('Ctrl Pts',(-9.44544108949558,17.962408853302,2.45997517699205));
#98825=CARTESIAN_POINT('Ctrl Pts',(-9.4862517765319,17.9657108637688,2.43922152601819));
#98826=CARTESIAN_POINT('Ctrl Pts',(-9.53367794368512,17.9693085644532,2.41848489187108));
#98827=CARTESIAN_POINT('Ctrl Pts',(-9.53920358429843,17.9697241522026,2.41611907647317));
#98828=CARTESIAN_POINT('Ctrl Pts',(-9.54807424663757,17.9703853352421,2.41240118179785));
#98829=CARTESIAN_POINT('Ctrl Pts',(-9.55140770064966,17.9706324541602,2.41102202696952));
#98830=CARTESIAN_POINT('Ctrl Pts',(-9.55734108396712,17.9710698652058,2.40859906771301));
#98831=CARTESIAN_POINT('Ctrl Pts',(-9.55993846353534,17.9712605123008,2.40754919758599));
#98832=CARTESIAN_POINT('Ctrl Pts',(-9.56552813381234,17.9716689912033,2.40531300345106));
#98833=CARTESIAN_POINT('Ctrl Pts',(-9.56852155208188,17.9718866456502,2.40412967348693));
#98834=CARTESIAN_POINT('Ctrl Pts',(-9.57469601672108,17.9723334163409,2.40171806377634));
#98835=CARTESIAN_POINT('Ctrl Pts',(-9.57787762527539,17.97256244407,2.40049129557978));
#98836=CARTESIAN_POINT('Ctrl Pts',(-9.58600203777539,17.9731443690959,2.39739913848184));
#98837=CARTESIAN_POINT('Ctrl Pts',(-9.59095220804869,17.973496198362,2.39555313440607));
#98838=CARTESIAN_POINT('Ctrl Pts',(-9.60537548972847,17.9745138564587,2.3902847183569));
#98839=CARTESIAN_POINT('Ctrl Pts',(-9.61488053377607,17.975175189514,2.38695035048637));
#98840=CARTESIAN_POINT('Ctrl Pts',(-9.68538147067543,17.9800201456953,2.36322991948091));
#98841=CARTESIAN_POINT('Ctrl Pts',(-9.74786249841613,17.9839825748715,2.34776563038784));
#98842=CARTESIAN_POINT('Ctrl Pts',(-9.8111044001022,17.9879475322356,2.33749687418206));
#98843=CARTESIAN_POINT('Origin',(-10.,12.3756328852638,3.5));
#98844=CARTESIAN_POINT('',(-9.81110405347124,18.5858217457338,2.33749693166641));
#98845=CARTESIAN_POINT('',(-9.81110406374122,18.4867244625755,2.33749692999764));
#98846=CARTESIAN_POINT('',(-9.81110406371068,12.3756328852638,2.3374969300026));
#98847=CARTESIAN_POINT('Ctrl Pts',(-9.81110405343086,18.5858217463839,2.33749693167298));
#98848=CARTESIAN_POINT('Ctrl Pts',(-9.77349069906134,18.5834242261466,2.34360875225294));
#98849=CARTESIAN_POINT('Ctrl Pts',(-9.7361844295136,18.5810690906263,2.35154437023802));
#98850=CARTESIAN_POINT('Ctrl Pts',(-9.62087119967049,18.5736965981962,2.38199314469751));
#98851=CARTESIAN_POINT('Ctrl Pts',(-9.54478514597519,18.5686794602283,2.4107547070466));
#98852=CARTESIAN_POINT('Ctrl Pts',(-9.45881495506879,18.5624075265073,2.45384509380604));
#98853=CARTESIAN_POINT('Ctrl Pts',(-9.44549798619964,18.5614183188787,2.46084225270244));
#98854=CARTESIAN_POINT('Ctrl Pts',(-9.42649175251835,18.5599789256052,2.47129810515121));
#98855=CARTESIAN_POINT('Ctrl Pts',(-9.42069171163097,18.5595358991813,2.4745531694088));
#98856=CARTESIAN_POINT('Ctrl Pts',(-9.41053423289537,18.5587532066141,2.48036736758082));
#98857=CARTESIAN_POINT('Ctrl Pts',(-9.40616507516968,18.5584142865199,2.48290576819474));
#98858=CARTESIAN_POINT('Ctrl Pts',(-9.39717200900019,18.5577119450416,2.48820827456011));
#98859=CARTESIAN_POINT('Ctrl Pts',(-9.39255046766301,18.5573483938563,2.4909761418101));
#98860=CARTESIAN_POINT('Ctrl Pts',(-9.38072919374689,18.5564116345727,2.49816661790188));
#98861=CARTESIAN_POINT('Ctrl Pts',(-9.37355787603209,18.5558367686888,2.5026351140126));
#98862=CARTESIAN_POINT('Ctrl Pts',(-9.34319591591982,18.553374152951,2.52201049734209));
#98863=CARTESIAN_POINT('Ctrl Pts',(-9.32048612237669,18.5514596243354,2.53765092485362));
#98864=CARTESIAN_POINT('Ctrl Pts',(-9.21841478256243,18.5425053478852,2.61336351157382));
#98865=CARTESIAN_POINT('Ctrl Pts',(-9.14632789295126,18.5351219527637,2.68254192197185));
#98866=CARTESIAN_POINT('Ctrl Pts',(-9.06992351555006,18.5262594861745,2.77712990426883));
#98867=CARTESIAN_POINT('Ctrl Pts',(-9.0565229215821,18.5246591362309,2.79470960687341));
#98868=CARTESIAN_POINT('Ctrl Pts',(-9.03087925388811,18.5215162768187,2.83039044013339));
#98869=CARTESIAN_POINT('Ctrl Pts',(-9.01862882180434,18.5199738789571,2.84847659825261));
#98870=CARTESIAN_POINT('Ctrl Pts',(-9.00392254386255,18.5180786316875,2.87154539729453));
#98871=CARTESIAN_POINT('Ctrl Pts',(-9.00099014621973,18.517698408893,2.8762173444752));
#98872=CARTESIAN_POINT('Ctrl Pts',(-8.99640474476985,18.5171003607988,2.88363816463041));
#98873=CARTESIAN_POINT('Ctrl Pts',(-8.99473000714997,18.5168811792587,2.88637341116916));
#98874=CARTESIAN_POINT('Ctrl Pts',(-8.99175749543623,18.5164908404813,2.89127306378117));
#98875=CARTESIAN_POINT('Ctrl Pts',(-8.99045551103913,18.5163194161871,2.89343478843961));
#98876=CARTESIAN_POINT('Ctrl Pts',(-8.98734691054794,18.5159090125939,2.89863382916381));
#98877=CARTESIAN_POINT('Ctrl Pts',(-8.98554700613022,18.5156704664211,2.90167510911526));
#98878=CARTESIAN_POINT('Ctrl Pts',(-8.98010690339994,18.514946507767,2.9109623142101));
#98879=CARTESIAN_POINT('Ctrl Pts',(-8.97651041520775,18.5144637858156,2.91723383756804));
#98880=CARTESIAN_POINT('Ctrl Pts',(-8.9445371821246,18.5101308988543,2.97419757116948));
#98881=CARTESIAN_POINT('Ctrl Pts',(-8.91988556476199,18.5064873508038,3.02689887745853));
#98882=CARTESIAN_POINT('Ctrl Pts',(-8.86317525076844,18.4965894708289,3.17596077799349));
#98883=CARTESIAN_POINT('Ctrl Pts',(-8.8395151258666,18.4904163347123,3.27495614680011));
#98884=CARTESIAN_POINT('Ctrl Pts',(-8.82739449149161,18.4829037185242,3.38920989543255));
#98885=CARTESIAN_POINT('Ctrl Pts',(-8.82619916515082,18.4820123692791,3.40268760951448));
#98886=CARTESIAN_POINT('Ctrl Pts',(-8.82477758381623,18.4806857483324,3.42261211001609));
#98887=CARTESIAN_POINT('Ctrl Pts',(-8.82437164111217,18.4802560467876,3.42904528197074));
#98888=CARTESIAN_POINT('Ctrl Pts',(-8.82374424334731,18.4794896421377,3.4404808623872));
#98889=CARTESIAN_POINT('Ctrl Pts',(-8.82350184057688,18.4791535975777,3.44548199978562));
#98890=CARTESIAN_POINT('Ctrl Pts',(-8.82305877653664,18.4784442001713,3.45601116599528));
#98891=CARTESIAN_POINT('Ctrl Pts',(-8.8228651573261,18.4780706370321,3.46153935310707));
#98892=CARTESIAN_POINT('Ctrl Pts',(-8.82245573312975,18.4770785385819,3.47617617633316));
#98893=CARTESIAN_POINT('Ctrl Pts',(-8.82230667421296,18.4764579521033,3.48528615340469));
#98894=CARTESIAN_POINT('Ctrl Pts',(-8.82209851591881,18.4734619151482,3.52903835825502));
#98895=CARTESIAN_POINT('Ctrl Pts',(-8.82346218795207,18.4710430475044,3.56366694571281));
#98896=CARTESIAN_POINT('Ctrl Pts',(-8.83190686207788,18.4638476852932,3.66461288195093));
#98897=CARTESIAN_POINT('Ctrl Pts',(-8.84309368939802,18.4589646196837,3.73044504756727));
#98898=CARTESIAN_POINT('Ctrl Pts',(-8.87520753911197,18.4495493809486,3.8545820564606));
#98899=CARTESIAN_POINT('Ctrl Pts',(-8.89528188888828,18.4450352990063,3.91289945239814));
#98900=CARTESIAN_POINT('Ctrl Pts',(-8.92371248718268,18.4400364945684,3.978325511078));
#98901=CARTESIAN_POINT('Ctrl Pts',(-8.92770889949343,18.439358623463,3.98721855059252));
#98902=CARTESIAN_POINT('Ctrl Pts',(-8.93337393436904,18.4384319825849,3.99941725037453));
#98903=CARTESIAN_POINT('Ctrl Pts',(-8.93494826274736,18.4381779481164,4.00276590154947));
#98904=CARTESIAN_POINT('Ctrl Pts',(-8.93767497344222,18.4377439443733,4.00849542400908));
#98905=CARTESIAN_POINT('Ctrl Pts',(-8.93881963009903,18.4375635162429,4.01087990876534));
#98906=CARTESIAN_POINT('Ctrl Pts',(-8.94122671705154,18.4371877847573,4.01585122168124));
#98907=CARTESIAN_POINT('Ctrl Pts',(-8.94249060989853,18.436992580019,4.01843730352217));
#98908=CARTESIAN_POINT('Ctrl Pts',(-8.94559915049485,18.4365174570555,4.02473909697768));
#98909=CARTESIAN_POINT('Ctrl Pts',(-8.94745399709511,18.4362381609824,4.0284497936474));
#98910=CARTESIAN_POINT('Ctrl Pts',(-8.95419943843827,18.4352371573774,4.04176790742874));
#98911=CARTESIAN_POINT('Ctrl Pts',(-8.95920246102509,18.4345220202518,4.05131822329618));
#98912=CARTESIAN_POINT('Ctrl Pts',(-8.97202574889643,18.4327520512792,4.07499982415109));
#98913=CARTESIAN_POINT('Ctrl Pts',(-8.98000704092764,18.4317055576298,4.08904182919863));
#98914=CARTESIAN_POINT('Ctrl Pts',(-9.01628554696298,18.4271621727846,4.14991908915369));
#98915=CARTESIAN_POINT('Ctrl Pts',(-9.04753984874897,18.423784547491,4.19491694290226));
#98916=CARTESIAN_POINT('Ctrl Pts',(-9.13262463226795,18.4153861872425,4.30083586801072));
#98917=CARTESIAN_POINT('Ctrl Pts',(-9.18983058547563,18.4103689991484,4.35866264131626));
#98918=CARTESIAN_POINT('Ctrl Pts',(-9.26414599516599,18.404097010245,4.41969572333441));
#98919=CARTESIAN_POINT('Ctrl Pts',(-9.27595202709852,18.4031078040363,4.42901875080838));
#98920=CARTESIAN_POINT('Ctrl Pts',(-9.29323067446997,18.4016684124586,4.44213397074598));
#98921=CARTESIAN_POINT('Ctrl Pts',(-9.29856226968893,18.4012253862869,4.44611014463828));
#98922=CARTESIAN_POINT('Ctrl Pts',(-9.30800323592951,18.4004426940138,4.45302732080032));
#98923=CARTESIAN_POINT('Ctrl Pts',(-9.31209842758786,18.4001037739599,4.45598745859254));
#98924=CARTESIAN_POINT('Ctrl Pts',(-9.32059858058123,18.3994014324172,4.46204874809421));
#98925=CARTESIAN_POINT('Ctrl Pts',(-9.32500601650267,18.3990378811265,4.4651462080906));
#98926=CARTESIAN_POINT('Ctrl Pts',(-9.33638073686876,18.3981011212575,4.47302411618781));
#98927=CARTESIAN_POINT('Ctrl Pts',(-9.34337839692143,18.3975262548897,4.47775995058654));
#98928=CARTESIAN_POINT('Ctrl Pts',(-9.37342237787305,18.3950636341199,4.49762495922158));
#98929=CARTESIAN_POINT('Ctrl Pts',(-9.39694345623799,18.3931491008196,4.51201663078266));
#98930=CARTESIAN_POINT('Ctrl Pts',(-9.50760861202896,18.3841948224945,4.57450008185539));
#98931=CARTESIAN_POINT('Ctrl Pts',(-9.60011575229865,18.3768114309115,4.61224383759791));
#98932=CARTESIAN_POINT('Ctrl Pts',(-9.71759360527407,18.3679489676577,4.643603983339));
#98933=CARTESIAN_POINT('Ctrl Pts',(-9.73910252040602,18.3663486173295,4.64870189411356));
#98934=CARTESIAN_POINT('Ctrl Pts',(-9.78212622001024,18.3632057599128,4.65762817770039));
#98935=CARTESIAN_POINT('Ctrl Pts',(-9.80363031521089,18.3616633643626,4.66146936159186));
#98936=CARTESIAN_POINT('Ctrl Pts',(-9.83068509652546,18.3597681195106,4.66552904284654));
#98937=CARTESIAN_POINT('Ctrl Pts',(-9.83614562005127,18.3593878969035,4.66630923490543));
#98938=CARTESIAN_POINT('Ctrl Pts',(-9.8447895880421,18.358789849038,4.66748236664908));
#98939=CARTESIAN_POINT('Ctrl Pts',(-9.84796941679787,18.3585706675409,4.66790070246239));
#98940=CARTESIAN_POINT('Ctrl Pts',(-9.85365429363106,18.3581803287998,4.66862498908559));
#98941=CARTESIAN_POINT('Ctrl Pts',(-9.85615860318361,18.3580089044992,4.66893587661128));
#98942=CARTESIAN_POINT('Ctrl Pts',(-9.86217233772733,18.357598500839,4.66966280889915));
#98943=CARTESIAN_POINT('Ctrl Pts',(-9.86568265624522,18.3573599546059,4.67007111023077));
#98944=CARTESIAN_POINT('Ctrl Pts',(-9.87637929249081,18.3566359955851,4.67126651301685));
#98945=CARTESIAN_POINT('Ctrl Pts',(-9.88357123128922,18.3561532733312,4.67200327309138));
#98946=CARTESIAN_POINT('Ctrl Pts',(-9.9486133073264,18.3518203754249,4.67806170493588));
#98947=CARTESIAN_POINT('Ctrl Pts',(-10.0067849110766,18.3481768178725,4.67916319866799));
#98948=CARTESIAN_POINT('Ctrl Pts',(-10.1660283667076,18.3382789416503,4.67038731481509));
#98949=CARTESIAN_POINT('Ctrl Pts',(-10.2660937083242,18.332105817369,4.65176559017269));
#98950=CARTESIAN_POINT('Ctrl Pts',(-10.3754095839702,18.3245932135332,4.61639857167634));
#98951=CARTESIAN_POINT('Ctrl Pts',(-10.3882095555246,18.3237018625563,4.61201233939074));
#98952=CARTESIAN_POINT('Ctrl Pts',(-10.4069916827563,18.3223752395198,4.60521237020294));
#98953=CARTESIAN_POINT('Ctrl Pts',(-10.4130344381835,18.3219455376426,4.60296834187195));
#98954=CARTESIAN_POINT('Ctrl Pts',(-10.4237377209317,18.3211791326198,4.59889329630616));
#98955=CARTESIAN_POINT('Ctrl Pts',(-10.4284056016692,18.3208430880215,4.59708193492466));
#98956=CARTESIAN_POINT('Ctrl Pts',(-10.4382057939142,18.3201336907602,4.59320690775121));
#98957=CARTESIAN_POINT('Ctrl Pts',(-10.4433353876533,18.3197601278059,4.59113674359405));
#98958=CARTESIAN_POINT('Ctrl Pts',(-10.4568749047888,18.3187680303765,4.58556132768491));
#98959=CARTESIAN_POINT('Ctrl Pts',(-10.4652589228806,18.3181474447412,4.5819945477417));
#98960=CARTESIAN_POINT('Ctrl Pts',(-10.5053181178984,18.315151418866,4.56440063974568));
#98961=CARTESIAN_POINT('Ctrl Pts',(-10.5364025171527,18.3127325618501,4.54907913546556));
#98962=CARTESIAN_POINT('Ctrl Pts',(-10.6251998831324,18.3055372479804,4.50033195345198));
#98963=CARTESIAN_POINT('Ctrl Pts',(-10.6808006826714,18.3006542219303,4.46335221656612));
#98964=CARTESIAN_POINT('Ctrl Pts',(-10.7811667688113,18.2912389701846,4.383552533237));
#98965=CARTESIAN_POINT('Ctrl Pts',(-10.8262899906076,18.2867248357184,4.34150638684894));
#98966=CARTESIAN_POINT('Ctrl Pts',(-10.8745114468342,18.2817259830588,4.28893588721454));
#98967=CARTESIAN_POINT('Ctrl Pts',(-10.8810122389433,18.2810481120097,4.2816697225066));
#98968=CARTESIAN_POINT('Ctrl Pts',(-10.8898550346527,18.280121471194,4.27153533370644));
#98969=CARTESIAN_POINT('Ctrl Pts',(-10.8922746455954,18.2798674367325,4.26873578790931));
#98970=CARTESIAN_POINT('Ctrl Pts',(-10.8964011541252,18.2794334329983,4.2639155903449));
#98971=CARTESIAN_POINT('Ctrl Pts',(-10.8981144934879,18.2792530048699,4.26190052843531));
#98972=CARTESIAN_POINT('Ctrl Pts',(-10.901678173742,18.2788772733847,4.25768055181123));
#98973=CARTESIAN_POINT('Ctrl Pts',(-10.9035272382599,18.2786820686448,4.25547460417849));
#98974=CARTESIAN_POINT('Ctrl Pts',(-10.9080214050979,18.2782069456717,4.25007292926693));
#98975=CARTESIAN_POINT('Ctrl Pts',(-10.9106577798778,18.2779276495906,4.24686992213238));
#98976=CARTESIAN_POINT('Ctrl Pts',(-10.9200841850464,18.2769266459247,4.23529339214173));
#98977=CARTESIAN_POINT('Ctrl Pts',(-10.9267763451115,18.2762115087471,4.22684035842382));
#98978=CARTESIAN_POINT('Ctrl Pts',(-10.9432009857217,18.2744415396198,4.20549823478958));
#98979=CARTESIAN_POINT('Ctrl Pts',(-10.9527864412493,18.2733950458695,4.19249831084729));
#98980=CARTESIAN_POINT('Ctrl Pts',(-10.9936613983756,18.2688516603005,4.13460694451443));
#98981=CARTESIAN_POINT('Ctrl Pts',(-11.0220701539553,18.2654740344227,4.08776057943285));
#98982=CARTESIAN_POINT('Ctrl Pts',(-11.0842594467699,18.2570756743738,3.96696848501761));
#98983=CARTESIAN_POINT('Ctrl Pts',(-11.1138408013418,18.2520584870412,3.89119647104517));
#98984=CARTESIAN_POINT('Ctrl Pts',(-11.139397081249,18.2457864989762,3.79848891302892));
#98985=CARTESIAN_POINT('Ctrl Pts',(-11.1431163254308,18.2447972927459,3.78391261500665));
#98986=CARTESIAN_POINT('Ctrl Pts',(-11.148075872683,18.2433579011425,3.76279476575378));
#98987=CARTESIAN_POINT('Ctrl Pts',(-11.1495415937594,18.2429148749669,3.75630727556835));
#98988=CARTESIAN_POINT('Ctrl Pts',(-11.1520240419837,18.2421321826893,3.74486976613582));
#98989=CARTESIAN_POINT('Ctrl Pts',(-11.1530640160851,18.2417932626348,3.73992492393071));
#98990=CARTESIAN_POINT('Ctrl Pts',(-11.1551468898333,18.2410909210932,3.72969489616916));
#98991=CARTESIAN_POINT('Ctrl Pts',(-11.1561854106457,18.240727369804,3.72440895026488));
#98992=CARTESIAN_POINT('Ctrl Pts',(-11.1587596211645,18.239790609944,3.71081413007415));
#98993=CARTESIAN_POINT('Ctrl Pts',(-11.1602422021113,18.2392157435835,3.70249563708554));
#98994=CARTESIAN_POINT('Ctrl Pts',(-11.1661799907445,18.2367531228901,3.66697097036281));
#98995=CARTESIAN_POINT('Ctrl Pts',(-11.1697683934133,18.234838589661,3.63963080487817));
#98996=CARTESIAN_POINT('Ctrl Pts',(-11.1818745745313,18.2258843113643,3.51312231235816));
#98997=CARTESIAN_POINT('Ctrl Pts',(-11.1787578069356,18.2185009197276,3.41326016732601));
#98998=CARTESIAN_POINT('Ctrl Pts',(-11.1596586156403,18.2096384564231,3.29317800489739));
#98999=CARTESIAN_POINT('Ctrl Pts',(-11.1555735550435,18.2080381061008,3.2714539537016));
#99000=CARTESIAN_POINT('Ctrl Pts',(-11.1462411193192,18.2048952486538,3.22851652312526));
#99001=CARTESIAN_POINT('Ctrl Pts',(-11.1410097940751,18.2033528530685,3.20730770275499));
#99002=CARTESIAN_POINT('Ctrl Pts',(-11.1337218884577,18.2014576081798,3.18093861736378));
#99003=CARTESIAN_POINT('Ctrl Pts',(-11.1322151560517,18.2010773855698,3.17563241582836));
#99004=CARTESIAN_POINT('Ctrl Pts',(-11.1297734483135,18.2004793377008,3.16725790181794));
#99005=CARTESIAN_POINT('Ctrl Pts',(-11.128863146155,18.2002601562031,3.16418256999684));
#99006=CARTESIAN_POINT('Ctrl Pts',(-11.1272141411536,18.1998698174614,3.15869410952744));
#99007=CARTESIAN_POINT('Ctrl Pts',(-11.1264802489925,18.1996983931609,3.15627964899235));
#99008=CARTESIAN_POINT('Ctrl Pts',(-11.124699988925,18.1992879895017,3.15048964833436));
#99009=CARTESIAN_POINT('Ctrl Pts',(-11.1236461829439,18.1990494432695,3.14711643933805));
#99010=CARTESIAN_POINT('Ctrl Pts',(-11.1203904658806,18.1983254842543,3.13685742771944));
#99011=CARTESIAN_POINT('Ctrl Pts',(-11.1181402749674,18.1978427620049,3.12998695183104));
#99012=CARTESIAN_POINT('Ctrl Pts',(-11.0972376812962,18.1935098642643,3.06809787766158));
#99013=CARTESIAN_POINT('Ctrl Pts',(-11.0745987943013,18.1898663068556,3.01450096280877));
#99014=CARTESIAN_POINT('Ctrl Pts',(-11.0018524116027,18.1799684623845,2.87257388695619));
#99015=CARTESIAN_POINT('Ctrl Pts',(-10.9441647722163,18.1737953689029,2.7887176256973));
#99016=CARTESIAN_POINT('Ctrl Pts',(-10.8676030367396,18.1663009555454,2.70342253248312));
#99017=CARTESIAN_POINT('Ctrl Pts',(-10.8585850920111,18.1654280277789,2.69371077908075));
#99018=CARTESIAN_POINT('Ctrl Pts',(-10.844920008003,18.1641183259595,2.67948359509731));
#99019=CARTESIAN_POINT('Ctrl Pts',(-10.8403961773091,18.1636868101745,2.67485076926536));
#99020=CARTESIAN_POINT('Ctrl Pts',(-10.8323811372201,18.1629257230905,2.66677690183126));
#99021=CARTESIAN_POINT('Ctrl Pts',(-10.828906187939,18.1625968657817,2.66331988234828));
#99022=CARTESIAN_POINT('Ctrl Pts',(-10.8248741445703,18.1622165279818,2.65935841643118));
#99023=CARTESIAN_POINT('Ctrl Pts',(-10.824337982709,18.1621659775889,2.65883264645829));
#99024=CARTESIAN_POINT('Ctrl Pts',(-10.8236532523797,18.1621014517422,2.65816247097802));
#99025=CARTESIAN_POINT('Ctrl Pts',(-10.8235051471627,18.1620874968855,2.65801759043194));
#99026=CARTESIAN_POINT('Ctrl Pts',(-10.8232307964716,18.162061650367,2.65774935476712));
#99027=CARTESIAN_POINT('Ctrl Pts',(-10.8231045614585,18.1620497591706,2.65762598890958));
#99028=CARTESIAN_POINT('Ctrl Pts',(-10.8228696205998,18.162027630564,2.65739649118053));
#99029=CARTESIAN_POINT('Ctrl Pts',(-10.822760921931,18.1620173934736,2.65729035194553));
#99030=CARTESIAN_POINT('Ctrl Pts',(-10.8225578200812,18.1619982675225,2.65709210911373));
#99031=CARTESIAN_POINT('Ctrl Pts',(-10.8224634219369,18.1619893788856,2.65700000031386));
#99032=CARTESIAN_POINT('Ctrl Pts',(-10.8222864501071,18.161972716452,2.65682737842656));
#99033=CARTESIAN_POINT('Ctrl Pts',(-10.8222038800531,18.1619649428169,2.65674686159711));
#99034=CARTESIAN_POINT('Ctrl Pts',(-10.8220486389495,18.1619503285976,2.65659552526808));
#99035=CARTESIAN_POINT('Ctrl Pts',(-10.8219759705755,18.1619434881331,2.65652470303336));
#99036=CARTESIAN_POINT('Ctrl Pts',(-10.8218390072068,18.1619305962652,2.65639125372634));
#99037=CARTESIAN_POINT('Ctrl Pts',(-10.8217747141986,18.1619245449502,2.65632862460561));
#99038=CARTESIAN_POINT('Ctrl Pts',(-10.8216532749907,18.1619131156524,2.65621035526707));
#99039=CARTESIAN_POINT('Ctrl Pts',(-10.8215961303019,18.1619077377374,2.65615471350822));
#99040=CARTESIAN_POINT('Ctrl Pts',(-10.8214879890023,18.1618975610344,2.65604943776952));
#99041=CARTESIAN_POINT('Ctrl Pts',(-10.8214369935417,18.1618927622977,2.65599980260345));
#99042=CARTESIAN_POINT('Ctrl Pts',(-10.8213403283009,18.1618836663986,2.65590573294998));
#99043=CARTESIAN_POINT('Ctrl Pts',(-10.821294659397,18.1618793692745,2.65586129753099));
#99044=CARTESIAN_POINT('Ctrl Pts',(-10.8212079631434,18.1618712121021,2.65577695657751));
#99045=CARTESIAN_POINT('Ctrl Pts',(-10.8211669365161,18.1618673520873,2.65573705035193));
#99046=CARTESIAN_POINT('Ctrl Pts',(-10.8210434380328,18.1618557330906,2.65561694202383));
#99047=CARTESIAN_POINT('Ctrl Pts',(-10.8209609573237,18.1618479737121,2.65553674900314));
#99048=CARTESIAN_POINT('Ctrl Pts',(-10.8207975547961,18.1618326027557,2.6553779251808));
#99049=CARTESIAN_POINT('Ctrl Pts',(-10.8207166334206,18.1618249911975,2.65529929391654));
#99050=CARTESIAN_POINT('Ctrl Pts',(-10.8205562114074,18.1618099028211,2.65514345673258));
#99051=CARTESIAN_POINT('Ctrl Pts',(-10.8204767111811,18.1618024260221,2.65506625041332));
#99052=CARTESIAN_POINT('Ctrl Pts',(-10.8203190029885,18.1617875950225,2.65491313599457));
#99053=CARTESIAN_POINT('Ctrl Pts',(-10.8202407953796,18.161780240838,2.6548372275274));
#99054=CARTESIAN_POINT('Ctrl Pts',(-10.8200855525007,18.1617656437385,2.65468659031199));
#99055=CARTESIAN_POINT('Ctrl Pts',(-10.8200085175446,18.1617584008372,2.65461186122991));
#99056=CARTESIAN_POINT('Ctrl Pts',(-10.8153393870804,18.1613194351235,2.65008372970618));
#99057=CARTESIAN_POINT('Ctrl Pts',(-10.8107111758715,18.1608861007471,2.64566788123927));
#99058=CARTESIAN_POINT('Ctrl Pts',(-10.8009513909169,18.159975889463,2.63650664103468));
#99059=CARTESIAN_POINT('Ctrl Pts',(-10.7958131018888,18.1594987157767,2.63176880107858));
#99060=CARTESIAN_POINT('Ctrl Pts',(-10.7820523440761,18.15822599902,2.61930526121784));
#99061=CARTESIAN_POINT('Ctrl Pts',(-10.7733577941701,18.1574271648611,2.61166065185665));
#99062=CARTESIAN_POINT('Ctrl Pts',(-10.7000334764934,18.1507325484699,2.54908321115328));
#99063=CARTESIAN_POINT('Ctrl Pts',(-10.6297663587169,18.1445588070023,2.50116118129535));
#99064=CARTESIAN_POINT('Ctrl Pts',(-10.4970964304385,18.1335136388542,2.4302818706869));
#99065=CARTESIAN_POINT('Ctrl Pts',(-10.4367247341494,18.1286902129682,2.40424686192557));
#99066=CARTESIAN_POINT('Ctrl Pts',(-10.3652761292401,18.1234097713586,2.38028444595804));
#99067=CARTESIAN_POINT('Ctrl Pts',(-10.3560207567468,18.1227338289047,2.37730734006603));
#99068=CARTESIAN_POINT('Ctrl Pts',(-10.3431963543221,18.1218093283671,2.37335675993764));
#99069=CARTESIAN_POINT('Ctrl Pts',(-10.3396583306219,18.1215555375603,2.37228507708487));
#99070=CARTESIAN_POINT('Ctrl Pts',(-10.3335811907528,18.1211218412123,2.37047547943243));
#99071=CARTESIAN_POINT('Ctrl Pts',(-10.3310445555221,18.1209414782147,2.36972943239224));
#99072=CARTESIAN_POINT('Ctrl Pts',(-10.3257404762789,18.120565758728,2.36818884333892));
#99073=CARTESIAN_POINT('Ctrl Pts',(-10.3229726036237,18.1203705014787,2.36739589892121));
#99074=CARTESIAN_POINT('Ctrl Pts',(-10.3162057316406,18.1198950483606,2.36548413800484));
#99075=CARTESIAN_POINT('Ctrl Pts',(-10.312203618327,18.1196154767017,2.36437629126054));
#99076=CARTESIAN_POINT('Ctrl Pts',(-10.297764302382,18.1186123670068,2.36046136757202));
#99077=CARTESIAN_POINT('Ctrl Pts',(-10.287294053668,18.1178954357742,2.35777671979731));
#99078=CARTESIAN_POINT('Ctrl Pts',(-10.2610370337925,18.1161201219387,2.35142813809792));
#99079=CARTESIAN_POINT('Ctrl Pts',(-10.2452084354103,18.1150701423105,2.34794508244518));
#99080=CARTESIAN_POINT('Ctrl Pts',(-10.1753052305177,18.1105016912029,2.33406911861617));
#99081=CARTESIAN_POINT('Ctrl Pts',(-10.1206085605618,18.1071038267697,2.32714822764158));
#99082=CARTESIAN_POINT('Ctrl Pts',(-9.98053663495295,18.0984317542157,2.31933122154072));
#99083=CARTESIAN_POINT('Ctrl Pts',(-9.89520662422518,18.0931587899832,2.32383104602558));
#99084=CARTESIAN_POINT('Ctrl Pts',(-9.81110406180164,18.0875733665015,2.3374969303128));
#99085=CARTESIAN_POINT('Ctrl Pts',(-9.81110440024615,17.9879475328942,2.33749687531877));
#99086=CARTESIAN_POINT('Ctrl Pts',(-9.89624655459561,17.9932799162418,2.32366209245349));
#99087=CARTESIAN_POINT('Ctrl Pts',(-9.98262890818452,17.9986092040002,2.31922423813105));
#99088=CARTESIAN_POINT('Ctrl Pts',(-10.0775110639795,18.0048348360056,2.32477043396183));
#99089=CARTESIAN_POINT('Ctrl Pts',(-10.0862895802192,18.0054140870354,2.32538236028972));
#99090=CARTESIAN_POINT('Ctrl Pts',(-10.1008871800037,18.0063831519045,2.32656443916478));
#99091=CARTESIAN_POINT('Ctrl Pts',(-10.1067104492753,18.0067712805985,2.32707966319707));
#99092=CARTESIAN_POINT('Ctrl Pts',(-10.1181310954306,18.0075356525651,2.3281758779023));
#99093=CARTESIAN_POINT('Ctrl Pts',(-10.123728626005,18.0079117874567,2.32875367489248));
#99094=CARTESIAN_POINT('Ctrl Pts',(-10.1342783242733,18.0086236152886,2.32991912164577));
#99095=CARTESIAN_POINT('Ctrl Pts',(-10.1392313345299,18.0089590319524,2.3304981554405));
#99096=CARTESIAN_POINT('Ctrl Pts',(-10.1504082367705,18.009718753683,2.33187680435392));
#99097=CARTESIAN_POINT('Ctrl Pts',(-10.1566296744157,18.0101436225768,2.33269473558102));
#99098=CARTESIAN_POINT('Ctrl Pts',(-10.1726154039065,18.0112405480649,2.33492647329904));
#99099=CARTESIAN_POINT('Ctrl Pts',(-10.182368836859,18.0119148662445,2.33641330477323));
#99100=CARTESIAN_POINT('Ctrl Pts',(-10.2570175307998,18.0171158007603,2.34875448762267));
#99101=CARTESIAN_POINT('Ctrl Pts',(-10.3209080357674,18.0218095374206,2.36490547037418));
#99102=CARTESIAN_POINT('Ctrl Pts',(-10.427830953069,18.0300471456841,2.40168644266637));
#99103=CARTESIAN_POINT('Ctrl Pts',(-10.4715870104864,18.0335336224847,2.41975118561526));
#99104=CARTESIAN_POINT('Ctrl Pts',(-10.5592647438194,18.0406676563981,2.4622938759754));
#99105=CARTESIAN_POINT('Ctrl Pts',(-10.6029532176322,18.0443050612248,2.48705397359862));
#99106=CARTESIAN_POINT('Ctrl Pts',(-10.6510388957987,18.0483075126372,2.51852322725529));
#99107=CARTESIAN_POINT('Ctrl Pts',(-10.6571069916028,18.0488125319615,2.52257547217418));
#99108=CARTESIAN_POINT('Ctrl Pts',(-10.6661195342621,18.049562052046,2.5287158750594));
#99109=CARTESIAN_POINT('Ctrl Pts',(-10.6690925397554,18.0498092084123,2.5307615054033));
#99110=CARTESIAN_POINT('Ctrl Pts',(-10.6743311701619,18.0502444864554,2.53440163100622));
#99111=CARTESIAN_POINT('Ctrl Pts',(-10.6766006208901,18.0504329756944,2.53599048881924));
#99112=CARTESIAN_POINT('Ctrl Pts',(-10.6815185491109,18.0508412501147,2.53945948636753));
#99113=CARTESIAN_POINT('Ctrl Pts',(-10.6841648643626,18.0510608321134,2.54134257937088));
#99114=CARTESIAN_POINT('Ctrl Pts',(-10.6914308519375,18.0516635408586,2.54655839873518));
#99115=CARTESIAN_POINT('Ctrl Pts',(-10.6960342637986,18.0520451694833,2.54991378448837));
#99116=CARTESIAN_POINT('Ctrl Pts',(-10.7200556131997,18.0540364566971,2.567691032664));
#99117=CARTESIAN_POINT('Ctrl Pts',(-10.7390517520593,18.0556108103593,2.58267628412831));
#99118=CARTESIAN_POINT('Ctrl Pts',(-10.7700572192921,18.0582053337136,2.6087240954319));
#99119=CARTESIAN_POINT('Ctrl Pts',(-10.782321447387,18.0592385149888,2.61946944896289));
#99120=CARTESIAN_POINT('Ctrl Pts',(-10.8665400769098,18.0664141439465,2.69640704768386));
#99121=CARTESIAN_POINT('Ctrl Pts',(-10.9302287797529,18.072297639372,2.77107702809972));
#99122=CARTESIAN_POINT('Ctrl Pts',(-11.0012969513953,18.0805465736133,2.87911775893009));
#99123=CARTESIAN_POINT('Ctrl Pts',(-11.0175669802793,18.0825886942385,2.90615868717428));
#99124=CARTESIAN_POINT('Ctrl Pts',(-11.0368917332421,18.0852410942817,2.9414075683207));
#99125=CARTESIAN_POINT('Ctrl Pts',(-11.0409685778024,18.085815002005,2.94904230235077));
#99126=CARTESIAN_POINT('Ctrl Pts',(-11.0475137474967,18.0867607326882,2.96163150102086));
#99127=CARTESIAN_POINT('Ctrl Pts',(-11.050031996066,18.0871308034235,2.96655975278603));
#99128=CARTESIAN_POINT('Ctrl Pts',(-11.0547609299961,18.0878378101128,2.9759775909874));
#99129=CARTESIAN_POINT('Ctrl Pts',(-11.0569779239451,18.0881745176379,2.98046388811284));
#99130=CARTESIAN_POINT('Ctrl Pts',(-11.0619802149983,18.088946476539,2.9907510505271));
#99131=CARTESIAN_POINT('Ctrl Pts',(-11.064746675872,18.0893823647818,2.99656084483712));
#99132=CARTESIAN_POINT('Ctrl Pts',(-11.0731600540232,18.0907363857097,3.0146092005051));
#99133=CARTESIAN_POINT('Ctrl Pts',(-11.0786444231333,18.0916600018157,3.02692187541603));
#99134=CARTESIAN_POINT('Ctrl Pts',(-11.1237287054172,18.09961956489,3.13300020560193));
#99135=CARTESIAN_POINT('Ctrl Pts',(-11.1512224620096,18.1070757754673,3.23142357484736));
#99136=CARTESIAN_POINT('Ctrl Pts',(-11.1739626620484,18.1187789845062,3.38933301401143));
#99137=CARTESIAN_POINT('Ctrl Pts',(-11.1779796688525,18.122992580794,3.44707548108584));
#99138=CARTESIAN_POINT('Ctrl Pts',(-11.1777099224079,18.1275193761673,3.51210437389066));
#99139=CARTESIAN_POINT('Ctrl Pts',(-11.1776136034679,18.1280188069853,3.51932316421637));
#99140=CARTESIAN_POINT('Ctrl Pts',(-11.1773713344172,18.1287573690225,3.53007112707584));
#99141=CARTESIAN_POINT('Ctrl Pts',(-11.1772758804101,18.128999127416,3.53360110145967));
#99142=CARTESIAN_POINT('Ctrl Pts',(-11.1770850238677,18.1294120818648,3.53965188563967));
#99143=CARTESIAN_POINT('Ctrl Pts',(-11.1769973980032,18.1295837008919,3.54217287024685));
#99144=CARTESIAN_POINT('Ctrl Pts',(-11.1767799701779,18.1299724741011,3.54789832090751));
#99145=CARTESIAN_POINT('Ctrl Pts',(-11.176645179033,18.1301893498057,3.5511025502051));
#99146=CARTESIAN_POINT('Ctrl Pts',(-11.1762428663064,18.1307774616389,3.55981830479311));
#99147=CARTESIAN_POINT('Ctrl Pts',(-11.1759496930189,18.1311473159028,3.56532865053895));
#99148=CARTESIAN_POINT('Ctrl Pts',(-11.1743019023393,18.1329739809639,3.592675597958));
#99149=CARTESIAN_POINT('Ctrl Pts',(-11.1723776333173,18.1344020519729,3.61447513884007));
#99150=CARTESIAN_POINT('Ctrl Pts',(-11.1672940276228,18.1372284385312,3.65813595041488));
#99151=CARTESIAN_POINT('Ctrl Pts',(-11.1641250549916,18.1386258105676,3.67998688690251));
#99152=CARTESIAN_POINT('Ctrl Pts',(-11.1433098933133,18.1462488728141,3.79971086770836));
#99153=CARTESIAN_POINT('Ctrl Pts',(-11.113937697215,18.152238247045,3.89512961520169));
#99154=CARTESIAN_POINT('Ctrl Pts',(-11.0615380775325,18.1603808106143,4.01087592366385));
#99155=CARTESIAN_POINT('Ctrl Pts',(-11.0492717296893,18.1621741554056,4.03561734945052));
#99156=CARTESIAN_POINT('Ctrl Pts',(-11.0321300975534,18.1645556914776,4.06733937039312));
#99157=CARTESIAN_POINT('Ctrl Pts',(-11.0280321515678,18.1651166482754,4.07473157963259));
#99158=CARTESIAN_POINT('Ctrl Pts',(-11.0211929955393,18.1660397093128,4.08676140042664));
#99159=CARTESIAN_POINT('Ctrl Pts',(-11.0184988536213,18.1664001330915,4.09142553098409));
#99160=CARTESIAN_POINT('Ctrl Pts',(-11.0132165938155,18.1671007620256,4.10042710384001));
#99161=CARTESIAN_POINT('Ctrl Pts',(-11.0106323767912,18.1674408211155,4.10476670759857));
#99162=CARTESIAN_POINT('Ctrl Pts',(-11.0045834595305,18.168230677414,4.11477743966129));
#99163=CARTESIAN_POINT('Ctrl Pts',(-11.0010985400478,18.1686812014477,4.12043608651119));
#99164=CARTESIAN_POINT('Ctrl Pts',(-10.9895817743488,18.1701557052223,4.13878679549814));
#99165=CARTESIAN_POINT('Ctrl Pts',(-10.9813552755226,18.1711867736038,4.15135431612303));
#99166=CARTESIAN_POINT('Ctrl Pts',(-10.9267227928378,18.1778982903094,4.23143055451366));
#99167=CARTESIAN_POINT('Ctrl Pts',(-10.8736287694844,18.1838356198729,4.29408683982925));
#99168=CARTESIAN_POINT('Ctrl Pts',(-10.7753713026008,18.1938195071085,4.38815843873974));
#99169=CARTESIAN_POINT('Ctrl Pts',(-10.7337286537663,18.1978070430937,4.42285909312762));
#99170=CARTESIAN_POINT('Ctrl Pts',(-10.676832845844,18.2028394868716,4.46397618610012));
#99171=CARTESIAN_POINT('Ctrl Pts',(-10.6636295051111,18.2039802876305,4.4731129034171));
#99172=CARTESIAN_POINT('Ctrl Pts',(-10.6412944729006,18.2058605431677,4.48790264932902));
#99173=CARTESIAN_POINT('Ctrl Pts',(-10.6322651524079,18.206607576266,4.49370571249061));
#99174=CARTESIAN_POINT('Ctrl Pts',(-10.6196441671913,18.2076324459177,4.50157541405822));
#99175=CARTESIAN_POINT('Ctrl Pts',(-10.6161193657051,18.2079166159014,4.50374754420095));
#99176=CARTESIAN_POINT('Ctrl Pts',(-10.6101267082335,18.2083961748561,4.50739700919644));
#99177=CARTESIAN_POINT('Ctrl Pts',(-10.6076647823862,18.2085921754131,4.50888396119855));
#99178=CARTESIAN_POINT('Ctrl Pts',(-10.6029278669056,18.2089673181232,4.5117213294734));
#99179=CARTESIAN_POINT('Ctrl Pts',(-10.6006537516094,18.2091465523294,4.51307311297533));
#99180=CARTESIAN_POINT('Ctrl Pts',(-10.5951843999809,18.2095755934179,4.51629932359965));
#99181=CARTESIAN_POINT('Ctrl Pts',(-10.5919848121232,18.2098249326549,4.5181663755355));
#99182=CARTESIAN_POINT('Ctrl Pts',(-10.5802985309488,18.210729830924,4.52491194717597));
#99183=CARTESIAN_POINT('Ctrl Pts',(-10.5717596251167,18.211379938864,4.52969987422535));
#99184=CARTESIAN_POINT('Ctrl Pts',(-10.5103747872259,18.2159821661062,4.5631204312217));
#99185=CARTESIAN_POINT('Ctrl Pts',(-10.4554580488336,18.2197281853221,4.5877809253376));
#99186=CARTESIAN_POINT('Ctrl Pts',(-10.3351663407662,18.227645404358,4.63108167252156));
#99187=CARTESIAN_POINT('Ctrl Pts',(-10.2695844409577,18.2317996467166,4.64847979840075));
#99188=CARTESIAN_POINT('Ctrl Pts',(-10.1684502216729,18.2383249938015,4.66616496292897));
#99189=CARTESIAN_POINT('Ctrl Pts',(-10.1337799518953,18.24058082642,4.67064886017548));
#99190=CARTESIAN_POINT('Ctrl Pts',(-10.0898624353504,18.2434872683334,4.67435226128064));
#99191=CARTESIAN_POINT('Ctrl Pts',(-10.0807524246799,18.2440927560317,4.67501384204308));
#99192=CARTESIAN_POINT('Ctrl Pts',(-10.0661107185064,18.2450704674166,4.6759060658985));
#99193=CARTESIAN_POINT('Ctrl Pts',(-10.060583365428,18.2454406031612,4.67620379057935));
#99194=CARTESIAN_POINT('Ctrl Pts',(-10.0500556883709,18.2461476587458,4.67669644784738));
#99195=CARTESIAN_POINT('Ctrl Pts',(-10.0450558062762,18.2464843496313,4.67689849830154));
#99196=CARTESIAN_POINT('Ctrl Pts',(-10.0336256133754,18.2472561637289,4.6772874600654));
#99197=CARTESIAN_POINT('Ctrl Pts',(-10.0271948015114,18.2476919229504,4.67745355977199));
#99198=CARTESIAN_POINT('Ctrl Pts',(-10.0072965903409,18.2490451393374,4.67780440841259));
#99199=CARTESIAN_POINT('Ctrl Pts',(-9.99382754803064,18.2499680705262,4.67781082493407));
#99200=CARTESIAN_POINT('Ctrl Pts',(-9.87851607912541,18.2579320588304,4.67588781825329));
#99201=CARTESIAN_POINT('Ctrl Pts',(-9.7773397300021,18.2653941079817,4.6609841903134));
#99202=CARTESIAN_POINT('Ctrl Pts',(-9.62380994026725,18.2770984894761,4.61754636115816));
#99203=CARTESIAN_POINT('Ctrl Pts',(-9.56947619617376,18.2813076838934,4.59776120950571));
#99204=CARTESIAN_POINT('Ctrl Pts',(-9.51022586654913,18.2858303157477,4.57110618120037));
#99205=CARTESIAN_POINT('Ctrl Pts',(-9.50367100668084,18.2863296298738,4.5680845894087));
#99206=CARTESIAN_POINT('Ctrl Pts',(-9.49395128857164,18.2870680537542,4.56349528966235));
#99207=CARTESIAN_POINT('Ctrl Pts',(-9.49076518382856,18.2873097892858,4.56197336703647));
#99208=CARTESIAN_POINT('Ctrl Pts',(-9.48531472337242,18.2877227182769,4.55933964868881));
#99209=CARTESIAN_POINT('Ctrl Pts',(-9.48304704812351,18.2878943345572,4.55823488472557));
#99210=CARTESIAN_POINT('Ctrl Pts',(-9.47790413636035,18.288283119937,4.55570888883348));
#99211=CARTESIAN_POINT('Ctrl Pts',(-9.47503114506118,18.2885000104444,4.55428319286481));
#99212=CARTESIAN_POINT('Ctrl Pts',(-9.46723035984916,18.2890882019001,4.55037232988464));
#99213=CARTESIAN_POINT('Ctrl Pts',(-9.46231407576237,18.2894581203609,4.54786419477882));
#99214=CARTESIAN_POINT('Ctrl Pts',(-9.43798686714166,18.2912856192423,4.53523691572724));
#99215=CARTESIAN_POINT('Ctrl Pts',(-9.4188416518202,18.2927144285093,4.52461180745118));
#99216=CARTESIAN_POINT('Ctrl Pts',(-9.38100938219991,18.2955413722563,4.50221397226953));
#99217=CARTESIAN_POINT('Ctrl Pts',(-9.36233530163464,18.2969385898355,4.49043730791836));
#99218=CARTESIAN_POINT('Ctrl Pts',(-9.26139765913469,18.3045625736288,4.42274280095003));
#99219=CARTESIAN_POINT('Ctrl Pts',(-9.18614589061285,18.3105530304517,4.35710540261612));
#99220=CARTESIAN_POINT('Ctrl Pts',(-9.10170303908136,18.3186954464042,4.26218012688427));
#99221=CARTESIAN_POINT('Ctrl Pts',(-9.08409993934672,18.3204872710746,4.24093377808199));
#99222=CARTESIAN_POINT('Ctrl Pts',(-9.06210094078125,18.3228670699843,4.21239863223821));
#99223=CARTESIAN_POINT('Ctrl Pts',(-9.0570142691155,18.3234278606348,4.2056517283069));
#99224=CARTESIAN_POINT('Ctrl Pts',(-9.04880493339615,18.3243507181473,4.1945156690034));
#99225=CARTESIAN_POINT('Ctrl Pts',(-9.04563894558165,18.3247111060049,4.19015871029149));
#99226=CARTESIAN_POINT('Ctrl Pts',(-9.03956188737649,18.3254117151025,4.18167382754315));
#99227=CARTESIAN_POINT('Ctrl Pts',(-9.03664726509804,18.3257517906039,4.17754858285099));
#99228=CARTESIAN_POINT('Ctrl Pts',(-9.02995869865391,18.3265417587979,4.16795143513183));
#99229=CARTESIAN_POINT('Ctrl Pts',(-9.02620439401565,18.3269923789523,4.16246612036225));
#99230=CARTESIAN_POINT('Ctrl Pts',(-9.01411427830674,18.3284675252336,4.14447671868318));
#99231=CARTESIAN_POINT('Ctrl Pts',(-9.00597161324908,18.3294991485851,4.13184525569275));
#99232=CARTESIAN_POINT('Ctrl Pts',(-8.95516086036789,18.3361919565036,4.04961009884403));
#99233=CARTESIAN_POINT('Ctrl Pts',(-8.91959388633695,18.3421080836765,3.97589715996257));
#99234=CARTESIAN_POINT('Ctrl Pts',(-8.8735198630548,18.3520865123483,3.84798182249075));
#99235=CARTESIAN_POINT('Ctrl Pts',(-8.85866282121709,18.3560899583041,3.79563299143681));
#99236=CARTESIAN_POINT('Ctrl Pts',(-8.84416212533963,18.3611402196289,3.72669957180082));
#99237=CARTESIAN_POINT('Ctrl Pts',(-8.84117310622523,18.3622835156834,3.7108890068058));
#99238=CARTESIAN_POINT('Ctrl Pts',(-8.83672886962364,18.3641674345998,3.68442041156964));
#99239=CARTESIAN_POINT('Ctrl Pts',(-8.83509404162091,18.3649156713764,3.67379510826856));
#99240=CARTESIAN_POINT('Ctrl Pts',(-8.83303096585809,18.3659419026605,3.65904558680714));
#99241=CARTESIAN_POINT('Ctrl Pts',(-8.83247872274192,18.3662262521877,3.65493964562733));
#99242=CARTESIAN_POINT('Ctrl Pts',(-8.83157975420406,18.3667060246195,3.64797792508561));
#99243=CARTESIAN_POINT('Ctrl Pts',(-8.83122180818548,18.3669020603605,3.64512365801137));
#99244=CARTESIAN_POINT('Ctrl Pts',(-8.83055481796598,18.3672771996999,3.63964248761962));
#99245=CARTESIAN_POINT('Ctrl Pts',(-8.83024416166529,18.3674563957659,3.63701582815862));
#99246=CARTESIAN_POINT('Ctrl Pts',(-8.8295199078594,18.3678852529712,3.63071007167855));
#99247=CARTESIAN_POINT('Ctrl Pts',(-8.82911480095663,18.3681344473567,3.62702999850877));
#99248=CARTESIAN_POINT('Ctrl Pts',(-8.82770365067842,18.3690380497597,3.61363017070219));
#99249=CARTESIAN_POINT('Ctrl Pts',(-8.82680119339457,18.3696870276938,3.60389957572614));
#99250=CARTESIAN_POINT('Ctrl Pts',(-8.82118841703263,18.3743100207085,3.53391876247904));
#99251=CARTESIAN_POINT('Ctrl Pts',(-8.82100001393733,18.3780755183309,3.47338813801381));
#99252=CARTESIAN_POINT('Ctrl Pts',(-8.82930223483163,18.3850432005377,3.36117048309988));
#99253=CARTESIAN_POINT('Ctrl Pts',(-8.83658444193764,18.3882436265389,3.3095506956916));
#99254=CARTESIAN_POINT('Ctrl Pts',(-8.8538570894595,18.3935323922451,3.22707554986978));
#99255=CARTESIAN_POINT('Ctrl Pts',(-8.86174421446304,18.3955757670389,3.19585389264921));
#99256=CARTESIAN_POINT('Ctrl Pts',(-8.87493822674618,18.3985736378633,3.1513846675296));
#99257=CARTESIAN_POINT('Ctrl Pts',(-8.87922240176128,18.3994980844753,3.13784783269082));
#99258=CARTESIAN_POINT('Ctrl Pts',(-8.88735401788923,18.401172049723,3.11368189329267));
#99259=CARTESIAN_POINT('Ctrl Pts',(-8.89111178507049,18.401918680841,3.10302434163622));
#99260=CARTESIAN_POINT('Ctrl Pts',(-8.89709891113719,18.403069489924,3.08679271391117));
#99261=CARTESIAN_POINT('Ctrl Pts',(-8.89921856833119,18.4034700524006,3.08117866514559));
#99262=CARTESIAN_POINT('Ctrl Pts',(-8.90315471946913,18.4042017615654,3.07098983780693));
#99263=CARTESIAN_POINT('Ctrl Pts',(-8.90495717627639,18.4045324352286,3.06640975375854));
#99264=CARTESIAN_POINT('Ctrl Pts',(-8.9089515490497,18.4052558693646,3.05644374416888));
#99265=CARTESIAN_POINT('Ctrl Pts',(-8.91115474011382,18.4056490001597,3.05106250732625));
#99266=CARTESIAN_POINT('Ctrl Pts',(-8.91730879281347,18.4067313485794,3.03634320948005));
#99267=CARTESIAN_POINT('Ctrl Pts',(-8.92134045911533,18.4074232657645,3.02703969176047));
#99268=CARTESIAN_POINT('Ctrl Pts',(-8.94420991820909,18.4112574654107,2.97607972307845));
#99269=CARTESIAN_POINT('Ctrl Pts',(-8.96533847017534,18.4144770657886,2.9355004721414));
#99270=CARTESIAN_POINT('Ctrl Pts',(-9.03085482954009,18.4236590778649,2.82576497294438));
#99271=CARTESIAN_POINT('Ctrl Pts',(-9.08019497647052,18.4297550888367,2.75987024362528));
#99272=CARTESIAN_POINT('Ctrl Pts',(-9.16221862174384,18.4385294239397,2.67132123871332));
#99273=CARTESIAN_POINT('Ctrl Pts',(-9.18983972701976,18.4412990982674,2.64429728968606));
#99274=CARTESIAN_POINT('Ctrl Pts',(-9.22339103149082,18.4444113169594,2.61455538012551));
#99275=CARTESIAN_POINT('Ctrl Pts',(-9.22807301441973,18.4448402300817,2.61047068738269));
#99276=CARTESIAN_POINT('Ctrl Pts',(-9.23531010941911,18.4454947102431,2.60425701750173));
#99277=CARTESIAN_POINT('Ctrl Pts',(-9.2378421908074,18.4457221208378,2.60210156808752));
#99278=CARTESIAN_POINT('Ctrl Pts',(-9.24251491980092,18.4461388451465,2.5981578877948));
#99279=CARTESIAN_POINT('Ctrl Pts',(-9.24465278765459,18.4463283777685,2.5963665393551));
#99280=CARTESIAN_POINT('Ctrl Pts',(-9.24950251291036,18.4467558051354,2.5923321262458));
#99281=CARTESIAN_POINT('Ctrl Pts',(-9.25221807120943,18.4469933740409,2.59009361198067));
#99282=CARTESIAN_POINT('Ctrl Pts',(-9.25926933499607,18.4476058222775,2.58433393627761));
#99283=CARTESIAN_POINT('Ctrl Pts',(-9.26362018802743,18.447979427891,2.58083133545519));
#99284=CARTESIAN_POINT('Ctrl Pts',(-9.29249456489808,18.4504319288529,2.55792298962229));
#99285=CARTESIAN_POINT('Ctrl Pts',(-9.31776017914787,18.4524508247053,2.53946772444647));
#99286=CARTESIAN_POINT('Ctrl Pts',(-9.42384227091535,18.460557448076,2.46828068823577));
#99287=CARTESIAN_POINT('Ctrl Pts',(-9.51025497710065,18.4663519572449,2.42456781225349));
#99288=CARTESIAN_POINT('Ctrl Pts',(-9.63876069485742,18.4749879898778,2.37830091267319));
#99289=CARTESIAN_POINT('Ctrl Pts',(-9.67715047978829,18.4775655108535,2.36665524604034));
#99290=CARTESIAN_POINT('Ctrl Pts',(-9.7252929361676,18.4808340394498,2.35469581774253));
#99291=CARTESIAN_POINT('Ctrl Pts',(-9.73455670897024,18.4814645403141,2.35251340256812));
#99292=CARTESIAN_POINT('Ctrl Pts',(-9.74933048893811,18.4824729875636,2.34922137863148));
#99293=CARTESIAN_POINT('Ctrl Pts',(-9.75482387799382,18.4828486018293,2.34803849607988));
#99294=CARTESIAN_POINT('Ctrl Pts',(-9.76520904626305,18.4835599967895,2.34587992371218));
#99295=CARTESIAN_POINT('Ctrl Pts',(-9.77009898396429,18.4838955052308,2.34489590774025));
#99296=CARTESIAN_POINT('Ctrl Pts',(-9.78116678250418,18.4846561851731,2.34274176617434));
#99297=CARTESIAN_POINT('Ctrl Pts',(-9.78734801827866,18.4850819262733,2.341589999679));
#99298=CARTESIAN_POINT('Ctrl Pts',(-9.79938593191289,18.4859129265063,2.33944653728568));
#99299=CARTESIAN_POINT('Ctrl Pts',(-9.80524142726179,18.4863180005648,2.33844955389612));
#99300=CARTESIAN_POINT('Ctrl Pts',(-9.81110406377177,18.4867244625755,2.33749692999267));
#99301=CARTESIAN_POINT('Origin',(-10.,12.3756328852638,3.5));
#99302=CARTESIAN_POINT('',(-9.81110406371068,19.0863176770662,2.3374969300026));
#99303=CARTESIAN_POINT('',(-9.81110406413403,18.9883401336252,2.33749692993381));
#99304=CARTESIAN_POINT('',(-9.81110406371068,12.3756328852638,2.3374969300026));
#99305=CARTESIAN_POINT('Ctrl Pts',(-9.81110406371067,19.0863176770662,2.3374969300026));
#99306=CARTESIAN_POINT('Ctrl Pts',(-9.79998400258774,19.0854907841518,2.33930383650601));
#99307=CARTESIAN_POINT('Ctrl Pts',(-9.78888576509648,19.0846642194548,2.34127096453477));
#99308=CARTESIAN_POINT('Ctrl Pts',(-9.72816303969516,19.0801389074277,2.35293600888952));
#99309=CARTESIAN_POINT('Ctrl Pts',(-9.67917261129528,19.0764752257255,2.36566223870694));
#99310=CARTESIAN_POINT('Ctrl Pts',(-9.62482488272611,19.0724968665875,2.38358475133384));
#99311=CARTESIAN_POINT('Ctrl Pts',(-9.61852053254864,19.0720367550016,2.38572319545148));
#99312=CARTESIAN_POINT('Ctrl Pts',(-9.60896544392668,19.0713418497106,2.3890548959235));
#99313=CARTESIAN_POINT('Ctrl Pts',(-9.60570140454673,19.0711049067735,2.39020917884645));
#99314=CARTESIAN_POINT('Ctrl Pts',(-9.59981824651872,19.0706786892108,2.39231890929555));
#99315=CARTESIAN_POINT('Ctrl Pts',(-9.59719740566085,19.0704891283364,2.39326927169212));
#99316=CARTESIAN_POINT('Ctrl Pts',(-9.59140945740733,19.0700711831091,2.3953913662672));
#99317=CARTESIAN_POINT('Ctrl Pts',(-9.58824400559542,19.0698430556597,2.3965674161938));
#99318=CARTESIAN_POINT('Ctrl Pts',(-9.57904224954649,19.0691810904604,2.40003122565024));
#99319=CARTESIAN_POINT('Ctrl Pts',(-9.57301952247867,19.0687493122699,2.40235506255322));
#99320=CARTESIAN_POINT('Ctrl Pts',(-9.52303949310428,19.0651761876398,2.4221132215645));
#99321=CARTESIAN_POINT('Ctrl Pts',(-9.48014391937047,19.0621735933518,2.44213325427585));
#99322=CARTESIAN_POINT('Ctrl Pts',(-9.41448169321778,19.0575056016143,2.47774080300979));
#99323=CARTESIAN_POINT('Ctrl Pts',(-9.39086208190029,19.0558108590556,2.49163666484558));
#99324=CARTESIAN_POINT('Ctrl Pts',(-9.29702912408821,19.0489350406853,2.55134148710412));
#99325=CARTESIAN_POINT('Ctrl Pts',(-9.23132466535231,19.0437624975836,2.60375388754537));
#99326=CARTESIAN_POINT('Ctrl Pts',(-9.16110829012873,19.0373200254693,2.67321133735428));
#99327=CARTESIAN_POINT('Ctrl Pts',(-9.15067609718986,19.0363363046374,2.68393157842004));
#99328=CARTESIAN_POINT('Ctrl Pts',(-9.13591458038499,19.0349034661078,2.69969037993726));
#99329=CARTESIAN_POINT('Ctrl Pts',(-9.13141899381979,19.0344614154831,2.70457172980403));
#99330=CARTESIAN_POINT('Ctrl Pts',(-9.12357501119376,19.0336798607689,2.713234590327));
#99331=CARTESIAN_POINT('Ctrl Pts',(-9.12020921026243,19.0333410958976,2.71700016871379));
#99332=CARTESIAN_POINT('Ctrl Pts',(-9.11329974529456,19.0326385018901,2.72483111217792));
#99333=CARTESIAN_POINT('Ctrl Pts',(-9.10975958250047,19.0322745394522,2.72889939455472));
#99334=CARTESIAN_POINT('Ctrl Pts',(-9.1007270060145,19.031335497959,2.7394245589286));
#99335=CARTESIAN_POINT('Ctrl Pts',(-9.09527621637551,19.0307587455026,2.74591659077249));
#99336=CARTESIAN_POINT('Ctrl Pts',(-9.07223408091918,19.0282764271102,2.77396984100779));
#99337=CARTESIAN_POINT('Ctrl Pts',(-9.0553410949428,19.026343544825,2.79609040389123));
#99338=CARTESIAN_POINT('Ctrl Pts',(-8.98179620120832,19.0173818414405,2.89981473047593));
#99339=CARTESIAN_POINT('Ctrl Pts',(-8.93483146816138,19.0100122167057,2.98777791571953));
#99340=CARTESIAN_POINT('Ctrl Pts',(-8.89158921802332,19.0011627066966,3.10123939386179));
#99341=CARTESIAN_POINT('Ctrl Pts',(-8.88429422915025,18.9995608289268,3.12213069710084));
#99342=CARTESIAN_POINT('Ctrl Pts',(-8.87101429514304,18.996425836262,3.16390810003806));
#99343=CARTESIAN_POINT('Ctrl Pts',(-8.86500976498491,18.994892562184,3.18477975909209));
#99344=CARTESIAN_POINT('Ctrl Pts',(-8.85821020442655,18.9930068619418,3.211137693731));
#99345=CARTESIAN_POINT('Ctrl Pts',(-8.85687241657059,18.9926273814706,3.21647804275222));
#99346=CARTESIAN_POINT('Ctrl Pts',(-8.85481516921627,18.9920302394285,3.224941758712));
#99347=CARTESIAN_POINT('Ctrl Pts',(-8.85407094859939,18.9918112282617,3.22805893554562));
#99348=CARTESIAN_POINT('Ctrl Pts',(-8.85276335288098,18.9914210330536,3.23363651061897));
#99349=CARTESIAN_POINT('Ctrl Pts',(-8.85219516588755,18.9912495832095,3.23609566897549));
#99350=CARTESIAN_POINT('Ctrl Pts',(-8.85084959427549,18.9908389129372,3.24200596603605));
#99351=CARTESIAN_POINT('Ctrl Pts',(-8.85007984832411,18.9906001272704,3.24545880072074));
#99352=CARTESIAN_POINT('Ctrl Pts',(-8.84778056063179,18.989874709366,3.25599599922743));
#99353=CARTESIAN_POINT('Ctrl Pts',(-8.84630080768773,18.9893907835142,3.26309122211892));
#99354=CARTESIAN_POINT('Ctrl Pts',(-8.83342528632705,18.9850140235566,3.32781132193521));
#99355=CARTESIAN_POINT('Ctrl Pts',(-8.82628841603408,18.9813324031335,3.3862081527337));
#99356=CARTESIAN_POINT('Ctrl Pts',(-8.81883617117429,18.9714492689713,3.54532661765381));
#99357=CARTESIAN_POINT('Ctrl Pts',(-8.82701018842903,18.9653233945672,3.64592915043192));
#99358=CARTESIAN_POINT('Ctrl Pts',(-8.85040627704,18.957948760933,3.75628134001346));
#99359=CARTESIAN_POINT('Ctrl Pts',(-8.85314075385154,18.9571404936181,3.76825306017515));
#99360=CARTESIAN_POINT('Ctrl Pts',(-8.85755593364221,18.9559099267463,3.78627969302862));
#99361=CARTESIAN_POINT('Ctrl Pts',(-8.85909877664834,18.9554919885486,3.79236775367464));
#99362=CARTESIAN_POINT('Ctrl Pts',(-8.8618720366625,18.9547609796132,3.80295470449677));
#99363=CARTESIAN_POINT('Ctrl Pts',(-8.8630806322569,18.9544486118587,3.80745920719682));
#99364=CARTESIAN_POINT('Ctrl Pts',(-8.86566814277827,18.9537925125666,3.81687909683994));
#99365=CARTESIAN_POINT('Ctrl Pts',(-8.86705232373346,18.95344861751,3.82179292370729));
#99366=CARTESIAN_POINT('Ctrl Pts',(-8.87043021199245,18.9526258194779,3.83349239183901));
#99367=CARTESIAN_POINT('Ctrl Pts',(-8.87245316161597,18.9521459813136,3.84026931223404));
#99368=CARTESIAN_POINT('Ctrl Pts',(-8.87957439581595,18.9504994052089,3.86336456049646));
#99369=CARTESIAN_POINT('Ctrl Pts',(-8.8849666826012,18.9493232124068,3.87958923329227));
#99370=CARTESIAN_POINT('Ctrl Pts',(-8.91520067677335,18.943072253366,3.96434816573856));
#99371=CARTESIAN_POINT('Ctrl Pts',(-8.94600859246498,18.9378033393692,4.03057291809629));
#99372=CARTESIAN_POINT('Ctrl Pts',(-9.02206514510724,18.9267390668157,4.16093147815351));
#99373=CARTESIAN_POINT('Ctrl Pts',(-9.06800517295492,18.9209604702316,4.22427524741828));
#99374=CARTESIAN_POINT('Ctrl Pts',(-9.12600550551236,18.9148512896116,4.28950219229256));
#99375=CARTESIAN_POINT('Ctrl Pts',(-9.13221373951829,18.9142106830921,4.29632098260347));
#99376=CARTESIAN_POINT('Ctrl Pts',(-9.14097090452611,18.9133262088424,4.30571532787416));
#99377=CARTESIAN_POINT('Ctrl Pts',(-9.14345239949684,18.9130776712334,4.30835288419642));
#99378=CARTESIAN_POINT('Ctrl Pts',(-9.14775315307273,18.9126505816476,4.31288207119822));
#99379=CARTESIAN_POINT('Ctrl Pts',(-9.14956662319596,18.9124716021644,4.31477912450985));
#99380=CARTESIAN_POINT('Ctrl Pts',(-9.15339596494298,18.912096022413,4.31875824806223));
#99381=CARTESIAN_POINT('Ctrl Pts',(-9.15541320532642,18.9118995351367,4.32083896564153));
#99382=CARTESIAN_POINT('Ctrl Pts',(-9.16040591222934,18.911416508555,4.32595088924892));
#99383=CARTESIAN_POINT('Ctrl Pts',(-9.1633901732139,18.9111306409251,4.32897352357623));
#99384=CARTESIAN_POINT('Ctrl Pts',(-9.17448093381527,18.9100784027957,4.34008600254205));
#99385=CARTESIAN_POINT('Ctrl Pts',(-9.1826892674293,18.9093195185481,4.34807394191538));
#99386=CARTESIAN_POINT('Ctrl Pts',(-9.24234764927128,18.9039327368299,4.40445963977172));
#99387=CARTESIAN_POINT('Ctrl Pts',(-9.2979500151173,18.8995806610879,4.44826832722522));
#99388=CARTESIAN_POINT('Ctrl Pts',(-9.42457065689338,18.8902393084136,4.53075240296901));
#99389=CARTESIAN_POINT('Ctrl Pts',(-9.49630518013522,18.8852611271086,4.56764174058429));
#99390=CARTESIAN_POINT('Ctrl Pts',(-9.58526020020486,18.8790321186293,4.60241222742192));
#99391=CARTESIAN_POINT('Ctrl Pts',(-9.59938864416844,18.8780418803422,4.60762463345889));
#99392=CARTESIAN_POINT('Ctrl Pts',(-9.61989816254569,18.8766012561321,4.61474747307565));
#99393=CARTESIAN_POINT('Ctrl Pts',(-9.62620196734435,18.8761580468056,4.61687705827065));
#99394=CARTESIAN_POINT('Ctrl Pts',(-9.6373245850552,18.8753751407942,4.62052984955988));
#99395=CARTESIAN_POINT('Ctrl Pts',(-9.64213583194315,18.8750361914398,4.6220756820367));
#99396=CARTESIAN_POINT('Ctrl Pts',(-9.65209505100026,18.8743338964638,4.62520496665753));
#99397=CARTESIAN_POINT('Ctrl Pts',(-9.6572442259448,18.8739704216939,4.62678416221276));
#99398=CARTESIAN_POINT('Ctrl Pts',(-9.67049407031553,18.8730340866274,4.63074851911867));
#99399=CARTESIAN_POINT('Ctrl Pts',(-9.67860977203029,18.8724595714423,4.63308194146854));
#99400=CARTESIAN_POINT('Ctrl Pts',(-9.71327889665108,18.8700005993182,4.64264756109201));
#99401=CARTESIAN_POINT('Ctrl Pts',(-9.7400544190049,18.8680894623986,4.64903460181142));
#99402=CARTESIAN_POINT('Ctrl Pts',(-9.86461801156321,18.8591365406619,4.67417144747533));
#99403=CARTESIAN_POINT('Ctrl Pts',(-9.96430280832018,18.8517505804295,4.6814087477441));
#99404=CARTESIAN_POINT('Ctrl Pts',(-10.0857480728976,18.8428856952671,4.67483212468812));
#99405=CARTESIAN_POINT('Ctrl Pts',(-10.1077738939043,18.8412856229628,4.6730166813751));
#99406=CARTESIAN_POINT('Ctrl Pts',(-10.1514651602569,18.8381413205625,4.66817434421005));
#99407=CARTESIAN_POINT('Ctrl Pts',(-10.1731242356884,18.8365972515551,4.6651614231081));
#99408=CARTESIAN_POINT('Ctrl Pts',(-10.2001302772772,18.834700256385,4.66063490373656));
#99409=CARTESIAN_POINT('Ctrl Pts',(-10.2055657377183,18.8343198982049,4.65968454250745));
#99410=CARTESIAN_POINT('Ctrl Pts',(-10.2141501693984,18.8337216848738,4.65812134779758));
#99411=CARTESIAN_POINT('Ctrl Pts',(-10.2173035754431,18.8335024722693,4.65753380425885));
#99412=CARTESIAN_POINT('Ctrl Pts',(-10.2229334788012,18.8331121072638,4.65646102162653));
#99413=CARTESIAN_POINT('Ctrl Pts',(-10.2254108042875,18.8329406875773,4.65598070918241));
#99414=CARTESIAN_POINT('Ctrl Pts',(-10.2313531203559,18.8325303323802,4.65480876341944));
#99415=CARTESIAN_POINT('Ctrl Pts',(-10.2348165623519,18.8322918296986,4.65410949620656));
#99416=CARTESIAN_POINT('Ctrl Pts',(-10.2453533072506,18.8315681358634,4.65193273691118));
#99417=CARTESIAN_POINT('Ctrl Pts',(-10.2524163685677,18.8310856323672,4.65040569326551));
#99418=CARTESIAN_POINT('Ctrl Pts',(-10.3160182104771,18.8267606377487,4.63604090874528));
#99419=CARTESIAN_POINT('Ctrl Pts',(-10.3715593550871,18.823123942058,4.61910768173727));
#99420=CARTESIAN_POINT('Ctrl Pts',(-10.5202983234554,18.813223346089,4.56145766405397));
#99421=CARTESIAN_POINT('Ctrl Pts',(-10.6098106009705,18.8070416696428,4.51268539316257));
#99422=CARTESIAN_POINT('Ctrl Pts',(-10.7028913304139,18.7995201414882,4.44510389920806));
#99423=CARTESIAN_POINT('Ctrl Pts',(-10.7136865113828,18.7986300456772,4.4369787306138));
#99424=CARTESIAN_POINT('Ctrl Pts',(-10.7294190037176,18.7973049374349,4.42470778231506));
#99425=CARTESIAN_POINT('Ctrl Pts',(-10.7344661477864,18.7968754764958,4.42070410047622));
#99426=CARTESIAN_POINT('Ctrl Pts',(-10.7433767940649,18.7961093418461,4.41351577453718));
#99427=CARTESIAN_POINT('Ctrl Pts',(-10.7472533439593,18.7957733249903,4.41034749788038));
#99428=CARTESIAN_POINT('Ctrl Pts',(-10.7553716924883,18.795063822142,4.403625635235));
#99429=CARTESIAN_POINT('Ctrl Pts',(-10.7596088723576,18.7946901248327,4.40006668735827));
#99430=CARTESIAN_POINT('Ctrl Pts',(-10.7707626785591,18.7936972858277,4.39056337769105));
#99431=CARTESIAN_POINT('Ctrl Pts',(-10.7776354929931,18.7930760874858,4.38456840788581));
#99432=CARTESIAN_POINT('Ctrl Pts',(-10.8103581004241,18.7900719979608,4.35534926663345));
#99433=CARTESIAN_POINT('Ctrl Pts',(-10.835238742274,18.7876454046907,4.33107065226259));
#99434=CARTESIAN_POINT('Ctrl Pts',(-10.9048710026018,18.7804148113205,4.25683404185184));
#99435=CARTESIAN_POINT('Ctrl Pts',(-10.9464709948768,18.7755028892511,4.20411652783334));
#99436=CARTESIAN_POINT('Ctrl Pts',(-11.0169651658191,18.7660974286231,4.09716521431976));
#99437=CARTESIAN_POINT('Ctrl Pts',(-11.0465600502645,18.7616219072534,4.04363409649131));
#99438=CARTESIAN_POINT('Ctrl Pts',(-11.07591263311,18.7566582786299,3.97916821893319));
#99439=CARTESIAN_POINT('Ctrl Pts',(-11.079843753822,18.7559801494676,3.97024212799605));
#99440=CARTESIAN_POINT('Ctrl Pts',(-11.0851130618404,18.755053222373,3.9578628619176));
#99441=CARTESIAN_POINT('Ctrl Pts',(-11.0865463955926,18.754799155459,3.95445097475492));
#99442=CARTESIAN_POINT('Ctrl Pts',(-11.088976609975,18.7543651107791,3.94858890074289));
#99443=CARTESIAN_POINT('Ctrl Pts',(-11.0899813505894,18.7541846739709,3.94614203418176));
#99444=CARTESIAN_POINT('Ctrl Pts',(-11.0920621805362,18.753808940854,3.94102555574889));
#99445=CARTESIAN_POINT('Ctrl Pts',(-11.0931367377496,18.7536137430793,3.9383553579045));
#99446=CARTESIAN_POINT('Ctrl Pts',(-11.095735887596,18.7531386639463,3.9318276639923));
#99447=CARTESIAN_POINT('Ctrl Pts',(-11.0972499313141,18.7528594044669,3.92796595225371));
#99448=CARTESIAN_POINT('Ctrl Pts',(-11.1026241811366,18.7518586802466,3.91404240908337));
#99449=CARTESIAN_POINT('Ctrl Pts',(-11.1063667861951,18.7511437810916,3.90393533656195));
#99450=CARTESIAN_POINT('Ctrl Pts',(-11.1153672716648,18.7493745207204,3.87856501475415));
#99451=CARTESIAN_POINT('Ctrl Pts',(-11.1204512141427,18.748328489135,3.86324200218918));
#99452=CARTESIAN_POINT('Ctrl Pts',(-11.1413644571401,18.7437884174297,3.79558610926651));
#99453=CARTESIAN_POINT('Ctrl Pts',(-11.1538549141785,18.740413466457,3.74228858262037));
#99454=CARTESIAN_POINT('Ctrl Pts',(-11.1755803216177,18.7320141907098,3.60816092981128));
#99455=CARTESIAN_POINT('Ctrl Pts',(-11.1802383611547,18.7269935158248,3.52689208966883));
#99456=CARTESIAN_POINT('Ctrl Pts',(-11.1758097141291,18.7207176887387,3.43076987753496));
#99457=CARTESIAN_POINT('Ctrl Pts',(-11.1748297292917,18.7197285818846,3.41576006086347));
#99458=CARTESIAN_POINT('Ctrl Pts',(-11.1730022794265,18.7182893089736,3.39414657671874));
#99459=CARTESIAN_POINT('Ctrl Pts',(-11.1723858354497,18.7178463004401,3.38752447135021));
#99460=CARTESIAN_POINT('Ctrl Pts',(-11.171202399141,18.7170636287478,3.37588096249331));
#99461=CARTESIAN_POINT('Ctrl Pts',(-11.1706591098427,18.7167247115129,3.37085727893159));
#99462=CARTESIAN_POINT('Ctrl Pts',(-11.1694698460921,18.7160223654719,3.36048526011253));
#99463=CARTESIAN_POINT('Ctrl Pts',(-11.1688194706839,18.7156588068009,3.35513755888353));
#99464=CARTESIAN_POINT('Ctrl Pts',(-11.1670547579532,18.7147220059634,3.34141356518546));
#99465=CARTESIAN_POINT('Ctrl Pts',(-11.1658869361227,18.7141471057273,3.33304458360342));
#99466=CARTESIAN_POINT('Ctrl Pts',(-11.1605248860396,18.7116841327672,3.29742329998767));
#99467=CARTESIAN_POINT('Ctrl Pts',(-11.1554646833515,18.7097692715863,3.2703122204667));
#99468=CARTESIAN_POINT('Ctrl Pts',(-11.1277763200773,18.7008148620037,3.14627752970873));
#99469=CARTESIAN_POINT('Ctrl Pts',(-11.0938723854304,18.6934317180553,3.05229889351215));
#99470=CARTESIAN_POINT('Ctrl Pts',(-11.038508177659,18.684569488207,2.94404656152457));
#99471=CARTESIAN_POINT('Ctrl Pts',(-11.0278929506242,18.6829691109619,2.92465693991007));
#99472=CARTESIAN_POINT('Ctrl Pts',(-11.005716907244,18.6798263932201,2.88672568408536));
#99473=CARTESIAN_POINT('Ctrl Pts',(-10.9941728908451,18.6782841594691,2.86818333644014));
#99474=CARTESIAN_POINT('Ctrl Pts',(-10.9790748709384,18.6763890838603,2.84537195195708));
#99475=CARTESIAN_POINT('Ctrl Pts',(-10.975998338465,18.6760088743706,2.8407938634256));
#99476=CARTESIAN_POINT('Ctrl Pts',(-10.9710821949622,18.675410842515,2.83358817629996));
#99477=CARTESIAN_POINT('Ctrl Pts',(-10.9692638662058,18.6751916640279,2.83094626043057));
#99478=CARTESIAN_POINT('Ctrl Pts',(-10.9659955094781,18.6748013278273,2.82623883564534));
#99479=CARTESIAN_POINT('Ctrl Pts',(-10.9645496424637,18.6746299030794,2.8241705700943));
#99480=CARTESIAN_POINT('Ctrl Pts',(-10.9610630005252,18.6742194947261,2.81921702394936));
#99481=CARTESIAN_POINT('Ctrl Pts',(-10.9590158753862,18.6739809442761,2.81633626464712));
#99482=CARTESIAN_POINT('Ctrl Pts',(-10.9527415398683,18.6732569595755,2.8075905209288));
#99483=CARTESIAN_POINT('Ctrl Pts',(-10.9484731699149,18.6727742161372,2.80175507095913));
#99484=CARTESIAN_POINT('Ctrl Pts',(-10.9094167634968,18.6684405517692,2.74937863374166));
#99485=CARTESIAN_POINT('Ctrl Pts',(-10.8712775981772,18.6647963288094,2.70542555772147));
#99486=CARTESIAN_POINT('Ctrl Pts',(-10.7581357391074,18.654898715298,2.59302750797585));
#99487=CARTESIAN_POINT('Ctrl Pts',(-10.6773159606229,18.6487264197648,2.5311811623224));
#99488=CARTESIAN_POINT('Ctrl Pts',(-10.5778650907643,18.6412146809033,2.4736715369355));
#99489=CARTESIAN_POINT('Ctrl Pts',(-10.5660352579006,18.6403232086952,2.46710008258104));
#99490=CARTESIAN_POINT('Ctrl Pts',(-10.5484068660871,18.6389964393599,2.45770132548734));
#99491=CARTESIAN_POINT('Ctrl Pts',(-10.5426938133542,18.6385667142219,2.45471533072383));
#99492=CARTESIAN_POINT('Ctrl Pts',(-10.5325002272042,18.6378002830893,2.4494936262581));
#99493=CARTESIAN_POINT('Ctrl Pts',(-10.5280293723009,18.6374642358056,2.44723928934207));
#99494=CARTESIAN_POINT('Ctrl Pts',(-10.5185895044334,18.6367548487033,2.44255468945364));
#99495=CARTESIAN_POINT('Ctrl Pts',(-10.5136174858364,18.6363812986923,2.44013079328625));
#99496=CARTESIAN_POINT('Ctrl Pts',(-10.5004117612855,18.6353892727026,2.43380764943514));
#99497=CARTESIAN_POINT('Ctrl Pts',(-10.4921497068448,18.634768746092,2.42996882420994));
#99498=CARTESIAN_POINT('Ctrl Pts',(-10.4522700580434,18.6317734955339,2.41199899021114));
#99499=CARTESIAN_POINT('Ctrl Pts',(-10.4200869578729,18.629355382189,2.39917261952027));
#99500=CARTESIAN_POINT('Ctrl Pts',(-10.3244694947015,18.622163450117,2.36586877007432));
#99501=CARTESIAN_POINT('Ctrl Pts',(-10.2598109262317,18.617283191258,2.34933474197101));
#99502=CARTESIAN_POINT('Ctrl Pts',(-10.1333286962355,18.6078670296911,2.32819967738834));
#99503=CARTESIAN_POINT('Ctrl Pts',(-10.0718379974637,18.60334922107,2.32282822438742));
#99504=CARTESIAN_POINT('Ctrl Pts',(-10.0004555369352,18.5983469949769,2.32220974012492));
#99505=CARTESIAN_POINT('Ctrl Pts',(-9.99070591637658,18.5976691275771,2.32224631639192));
#99506=CARTESIAN_POINT('Ctrl Pts',(-9.97725779336423,18.5967424908091,2.32246378151545));
#99507=CARTESIAN_POINT('Ctrl Pts',(-9.9735583399493,18.5964884568067,2.32254104387882));
#99508=CARTESIAN_POINT('Ctrl Pts',(-9.96721516235065,18.5960544536518,2.32270343043901));
#99509=CARTESIAN_POINT('Ctrl Pts',(-9.96457127696026,18.5958740256461,2.32278002726015));
#99510=CARTESIAN_POINT('Ctrl Pts',(-9.95905075738442,18.5954982941839,2.32295857883695));
#99511=CARTESIAN_POINT('Ctrl Pts',(-9.95617421059215,18.5953030893455,2.32306217325309));
#99512=CARTESIAN_POINT('Ctrl Pts',(-9.94915294860697,18.594827965752,2.32334081027488));
#99513=CARTESIAN_POINT('Ctrl Pts',(-9.94500866980837,18.594548669153,2.3235272097041));
#99514=CARTESIAN_POINT('Ctrl Pts',(-9.93009850332987,18.5935476615325,2.3242767919371));
#99515=CARTESIAN_POINT('Ctrl Pts',(-9.91933908790185,18.5928325209864,2.32496590735998));
#99516=CARTESIAN_POINT('Ctrl Pts',(-9.8924896088628,18.5910625418283,2.32705610623543));
#99517=CARTESIAN_POINT('Ctrl Pts',(-9.87641566395351,18.590016041537,2.32864060664368));
#99518=CARTESIAN_POINT('Ctrl Pts',(-9.84390287006405,18.5879168049108,2.33252234842891));
#99519=CARTESIAN_POINT('Ctrl Pts',(-9.82747438054779,18.5868652106325,2.33483690563033));
#99520=CARTESIAN_POINT('Ctrl Pts',(-9.81110405343086,18.5858217463839,2.33749693167298));
#99521=CARTESIAN_POINT('Ctrl Pts',(-9.81110406377177,18.4867244625755,2.33749692999267));
#99522=CARTESIAN_POINT('Ctrl Pts',(-9.81502055737344,18.4869959966987,2.33686053621041));
#99523=CARTESIAN_POINT('Ctrl Pts',(-9.81894023795535,18.4872681500725,2.33624393924982));
#99524=CARTESIAN_POINT('Ctrl Pts',(-9.89385327067581,18.4924773252704,2.32484715925569));
#99525=CARTESIAN_POINT('Ctrl Pts',(-9.96566935042106,18.4976187432309,2.32056398740546));
#99526=CARTESIAN_POINT('Ctrl Pts',(-10.1040909410058,18.5077366739403,2.32496377705408));
#99527=CARTESIAN_POINT('Ctrl Pts',(-10.1704651577274,18.5126783721553,2.33274383280967));
#99528=CARTESIAN_POINT('Ctrl Pts',(-10.2627546373824,18.519458288938,2.35160521263381));
#99529=CARTESIAN_POINT('Ctrl Pts',(-10.2894864562524,18.5214096712654,2.35805058846731));
#99530=CARTESIAN_POINT('Ctrl Pts',(-10.3214770335043,18.5237112106892,2.36695973018287));
#99531=CARTESIAN_POINT('Ctrl Pts',(-10.3269724690046,18.5241053510851,2.36853336596239));
#99532=CARTESIAN_POINT('Ctrl Pts',(-10.3355438439853,18.52471795289,2.37105547119819));
#99533=CARTESIAN_POINT('Ctrl Pts',(-10.3386276304222,18.5249379162887,2.37197661864078));
#99534=CARTESIAN_POINT('Ctrl Pts',(-10.3443887632108,18.5253479840531,2.37372326163712));
#99535=CARTESIAN_POINT('Ctrl Pts',(-10.3470669189619,18.5255382524336,2.37454566259372));
#99536=CARTESIAN_POINT('Ctrl Pts',(-10.3531874757884,18.5259722942019,2.37644907221503));
#99537=CARTESIAN_POINT('Ctrl Pts',(-10.3566278654057,18.5262157022643,2.3775363494232));
#99538=CARTESIAN_POINT('Ctrl Pts',(-10.365788068929,18.5268624058227,2.38047764490603));
#99539=CARTESIAN_POINT('Ctrl Pts',(-10.3714988641808,18.5272641421922,2.38235971234764));
#99540=CARTESIAN_POINT('Ctrl Pts',(-10.4206598832273,18.5307120300276,2.39897982194325));
#99541=CARTESIAN_POINT('Ctrl Pts',(-10.4632345790552,18.5336280476373,2.41620344913844));
#99542=CARTESIAN_POINT('Ctrl Pts',(-10.5675707820091,18.5408501776574,2.46568848325332));
#99543=CARTESIAN_POINT('Ctrl Pts',(-10.6276750261111,18.5450886544862,2.50101988983706));
#99544=CARTESIAN_POINT('Ctrl Pts',(-10.7237486399299,18.5524872091298,2.56960697826571));
#99545=CARTESIAN_POINT('Ctrl Pts',(-10.7614083264604,18.5555747416005,2.60016680463221));
#99546=CARTESIAN_POINT('Ctrl Pts',(-10.8053616510598,18.5594948062132,2.64057325024989));
#99547=CARTESIAN_POINT('Ctrl Pts',(-10.8135372415315,18.5602384564028,2.64830823095255));
#99548=CARTESIAN_POINT('Ctrl Pts',(-10.825893209441,18.5613856238808,2.66033854129972));
#99549=CARTESIAN_POINT('Ctrl Pts',(-10.8301538932381,18.5617855617628,2.66455073767223));
#99550=CARTESIAN_POINT('Ctrl Pts',(-10.8378556874318,18.5625166274357,2.67228197291186));
#99551=CARTESIAN_POINT('Ctrl Pts',(-10.8413072514379,18.5628472865883,2.67579044367144));
#99552=CARTESIAN_POINT('Ctrl Pts',(-10.8487944014127,18.5635712820222,2.68349706901601));
#99553=CARTESIAN_POINT('Ctrl Pts',(-10.8528210271905,18.5639649926084,2.68770370821696));
#99554=CARTESIAN_POINT('Ctrl Pts',(-10.8637983875353,18.5650504682649,2.69934341338896));
#99555=CARTESIAN_POINT('Ctrl Pts',(-10.870684098414,18.5657449585784,2.70683683051033));
#99556=CARTESIAN_POINT('Ctrl Pts',(-10.9084484904098,18.5696316474158,2.74901854771153));
#99557=CARTESIAN_POINT('Ctrl Pts',(-10.9373476628373,18.5729037524011,2.78541609221565));
#99558=CARTESIAN_POINT('Ctrl Pts',(-11.0157691935003,18.5827173171535,2.89715449260702));
#99559=CARTESIAN_POINT('Ctrl Pts',(-11.0588828810836,18.589431328629,2.97657406568185));
#99560=CARTESIAN_POINT('Ctrl Pts',(-11.1038949888336,18.5981322731122,3.08837147933389));
#99561=CARTESIAN_POINT('Ctrl Pts',(-11.1141687062613,18.6003001263911,3.11705007426972));
#99562=CARTESIAN_POINT('Ctrl Pts',(-11.1250854278307,18.6028192841211,3.15170076397929));
#99563=CARTESIAN_POINT('Ctrl Pts',(-11.1268088936171,18.6032245361751,3.15731749592413));
#99564=CARTESIAN_POINT('Ctrl Pts',(-11.129421210619,18.6038505474558,3.16606381979828));
#99565=CARTESIAN_POINT('Ctrl Pts',(-11.130339217603,18.6040729146079,3.16918449667144));
#99566=CARTESIAN_POINT('Ctrl Pts',(-11.1320223298029,18.6044850443882,3.17499488202908));
#99567=CARTESIAN_POINT('Ctrl Pts',(-11.132790780747,18.6046749889997,3.17768349532472));
#99568=CARTESIAN_POINT('Ctrl Pts',(-11.1345310839594,18.6051093144321,3.18385547681247));
#99569=CARTESIAN_POINT('Ctrl Pts',(-11.1354964741756,18.6053533235141,3.1873406038143));
#99570=CARTESIAN_POINT('Ctrl Pts',(-11.1379970917406,18.6059937498227,3.19653236892446));
#99571=CARTESIAN_POINT('Ctrl Pts',(-11.1395054718017,18.60638869319,3.20224629772624));
#99572=CARTESIAN_POINT('Ctrl Pts',(-11.1508483744507,18.6094291367701,3.24656361659155));
#99573=CARTESIAN_POINT('Ctrl Pts',(-11.1587627493247,18.6119768778465,3.28563672548265));
#99574=CARTESIAN_POINT('Ctrl Pts',(-11.1745999321648,18.6186788460379,3.39106246825286));
#99575=CARTESIAN_POINT('Ctrl Pts',(-11.1788863393335,18.6227485357035,3.4578101689625));
#99576=CARTESIAN_POINT('Ctrl Pts',(-11.1763743507372,18.6302551840462,3.57822763442844));
#99577=CARTESIAN_POINT('Ctrl Pts',(-11.1715878064183,18.6336496524675,3.63174654587664));
#99578=CARTESIAN_POINT('Ctrl Pts',(-11.1610285414453,18.6380502199837,3.69822726476439));
#99579=CARTESIAN_POINT('Ctrl Pts',(-11.1586536362071,18.6389491892219,3.71166730640503));
#99580=CARTESIAN_POINT('Ctrl Pts',(-11.1548099979576,18.640284915843,3.73141035471224));
#99581=CARTESIAN_POINT('Ctrl Pts',(-11.1535219576905,18.6407159882934,3.73774771074581));
#99582=CARTESIAN_POINT('Ctrl Pts',(-11.1511439275649,18.6414838361605,3.74897349756806));
#99583=CARTESIAN_POINT('Ctrl Pts',(-11.1500748159385,18.6418199428225,3.75386622634108));
#99584=CARTESIAN_POINT('Ctrl Pts',(-11.1477623265163,18.6425284436076,3.76413471612076));
#99585=CARTESIAN_POINT('Ctrl Pts',(-11.1465123149345,18.6429010414789,3.76950884278542));
#99586=CARTESIAN_POINT('Ctrl Pts',(-11.1431117781274,18.6438881791984,3.78367671499674));
#99587=CARTESIAN_POINT('Ctrl Pts',(-11.1408975798915,18.6445047347936,3.79245464631184));
#99588=CARTESIAN_POINT('Ctrl Pts',(-11.1308347400008,18.6471987270005,3.8304929793025));
#99589=CARTESIAN_POINT('Ctrl Pts',(-11.1219605915897,18.6493086129913,3.85946760637358));
#99590=CARTESIAN_POINT('Ctrl Pts',(-11.1049243392197,18.6529656890843,3.90828400259256));
#99591=CARTESIAN_POINT('Ctrl Pts',(-11.097318730925,18.6544958026373,3.92830495938168));
#99592=CARTESIAN_POINT('Ctrl Pts',(-11.0590716621276,18.661738715238,4.02126864099925));
#99593=CARTESIAN_POINT('Ctrl Pts',(-11.0216765370403,18.6676118806604,4.09121010438067));
#99594=CARTESIAN_POINT('Ctrl Pts',(-10.9632796359642,18.675219229617,4.17811713285849));
#99595=CARTESIAN_POINT('Ctrl Pts',(-10.948310777399,18.6770625051985,4.19889723598452));
#99596=CARTESIAN_POINT('Ctrl Pts',(-10.9265126280757,18.6795884986067,4.227166606161));
#99597=CARTESIAN_POINT('Ctrl Pts',(-10.9202470233905,18.6802976610222,4.235079828692));
#99598=CARTESIAN_POINT('Ctrl Pts',(-10.9091273343962,18.6815258159335,4.24875852338272));
#99599=CARTESIAN_POINT('Ctrl Pts',(-10.9043182775691,18.6820474202172,4.25455967076355));
#99600=CARTESIAN_POINT('Ctrl Pts',(-10.8971343272435,18.6828121752383,4.26305830031935));
#99601=CARTESIAN_POINT('Ctrl Pts',(-10.8948023497106,18.6830582247048,4.26579156865528));
#99602=CARTESIAN_POINT('Ctrl Pts',(-10.8906345538917,18.6834940222957,4.27063153426628));
#99603=CARTESIAN_POINT('Ctrl Pts',(-10.888803710323,18.6836841202136,4.27274241198857));
#99604=CARTESIAN_POINT('Ctrl Pts',(-10.8848145076174,18.6840954153674,4.27730884279825));
#99605=CARTESIAN_POINT('Ctrl Pts',(-10.8826534308083,18.6843164090719,4.27976193272126));
#99606=CARTESIAN_POINT('Ctrl Pts',(-10.8766367905957,18.6849267677561,4.28653450160242));
#99607=CARTESIAN_POINT('Ctrl Pts',(-10.8727594828177,18.6853145720274,4.29083466881437));
#99608=CARTESIAN_POINT('Ctrl Pts',(-10.8516009129125,18.6874022835756,4.31395564946696));
#99609=CARTESIAN_POINT('Ctrl Pts',(-10.8337409417213,18.6890626938121,4.33224045987523));
#99610=CARTESIAN_POINT('Ctrl Pts',(-10.7417289868374,18.6972153842518,4.42050316569943));
#99611=CARTESIAN_POINT('Ctrl Pts',(-10.6593045206666,18.7033143794301,4.48122825725592));
#99612=CARTESIAN_POINT('Ctrl Pts',(-10.5343347039392,18.7123381733835,4.55035731373159));
#99613=CARTESIAN_POINT('Ctrl Pts',(-10.4975850708971,18.7149628484845,4.56825680352153));
#99614=CARTESIAN_POINT('Ctrl Pts',(-10.4511744412744,18.7182843198107,4.58794679838419));
#99615=CARTESIAN_POINT('Ctrl Pts',(-10.4423212024537,18.718918141663,4.59157618035455));
#99616=CARTESIAN_POINT('Ctrl Pts',(-10.4281896357665,18.7199306696061,4.59716926685864));
#99617=CARTESIAN_POINT('Ctrl Pts',(-10.4229396223855,18.7203070103151,4.5992037291893));
#99618=CARTESIAN_POINT('Ctrl Pts',(-10.4130131019117,18.7210190101658,4.60296876801733));
#99619=CARTESIAN_POINT('Ctrl Pts',(-10.4083397843936,18.7213543914444,4.60470744757937));
#99620=CARTESIAN_POINT('Ctrl Pts',(-10.3977653591543,18.7221137387072,4.60856533178555));
#99621=CARTESIAN_POINT('Ctrl Pts',(-10.3918581246791,18.7225382662599,4.61066717933961));
#99622=CARTESIAN_POINT('Ctrl Pts',(-10.3766287179769,18.723633722796,4.61594932053755));
#99623=CARTESIAN_POINT('Ctrl Pts',(-10.367283081658,18.7243069031887,4.61905996482451));
#99624=CARTESIAN_POINT('Ctrl Pts',(-10.2968215911285,18.7293906041109,4.64153497498529));
#99625=CARTESIAN_POINT('Ctrl Pts',(-10.2342651864853,18.7339593222223,4.6559941543712));
#99626=CARTESIAN_POINT('Ctrl Pts',(-10.0977616799265,18.7440012761968,4.67600800968173));
#99627=CARTESIAN_POINT('Ctrl Pts',(-10.0238263296714,18.7494865150083,4.67982389078537));
#99628=CARTESIAN_POINT('Ctrl Pts',(-9.92197565711148,18.7568285137915,4.67549786391979));
#99629=CARTESIAN_POINT('Ctrl Pts',(-9.89397906443406,18.7588224902347,4.67330425855927));
#99630=CARTESIAN_POINT('Ctrl Pts',(-9.86037324027178,18.7611670542721,4.6694582011128));
#99631=CARTESIAN_POINT('Ctrl Pts',(-9.85466600859611,18.7615635127172,4.66876265790381));
#99632=CARTESIAN_POINT('Ctrl Pts',(-9.84576501136729,18.762178913902,4.66761167993822));
#99633=CARTESIAN_POINT('Ctrl Pts',(-9.84256773184522,18.7623993804826,4.66718488185244));
#99634=CARTESIAN_POINT('Ctrl Pts',(-9.8365979672755,18.7628098721468,4.66636301400065));
#99635=CARTESIAN_POINT('Ctrl Pts',(-9.83382515877768,18.7630000650292,4.66597119479821));
#99636=CARTESIAN_POINT('Ctrl Pts',(-9.82749393809585,18.763433291044,4.66505350054097));
#99637=CARTESIAN_POINT('Ctrl Pts',(-9.82393651613221,18.7636759639573,4.66452121106781));
#99638=CARTESIAN_POINT('Ctrl Pts',(-9.81447676026642,18.7643194060786,4.66306142855582));
#99639=CARTESIAN_POINT('Ctrl Pts',(-9.80857885794919,18.7647186408972,4.66210529175673));
#99640=CARTESIAN_POINT('Ctrl Pts',(-9.76152998911399,18.7678898094255,4.65411006628227));
#99641=CARTESIAN_POINT('Ctrl Pts',(-9.7207675095226,18.7705543393162,4.64493145833517));
#99642=CARTESIAN_POINT('Ctrl Pts',(-9.58546529319722,18.7793755946881,4.6068062064459));
#99643=CARTESIAN_POINT('Ctrl Pts',(-9.49411002172692,18.7853269760098,4.56814553588639));
#99644=CARTESIAN_POINT('Ctrl Pts',(-9.38403353477632,18.7934757884722,4.50423644223821));
#99645=CARTESIAN_POINT('Ctrl Pts',(-9.35994180850256,18.7953236019816,4.48905551956549));
#99646=CARTESIAN_POINT('Ctrl Pts',(-9.32936823217239,18.7977673232605,4.46820506888624));
#99647=CARTESIAN_POINT('Ctrl Pts',(-9.32236407467754,18.7983341394577,4.46331592417238));
#99648=CARTESIAN_POINT('Ctrl Pts',(-9.31101506381247,18.7992643805696,4.45520890034256));
#99649=CARTESIAN_POINT('Ctrl Pts',(-9.30663800994663,18.7996260733591,4.45203646709418));
#99650=CARTESIAN_POINT('Ctrl Pts',(-9.29822023225099,18.8003274248761,4.44584652645403));
#99651=CARTESIAN_POINT('Ctrl Pts',(-9.29417673734981,18.8006669261074,4.44283297278198));
#99652=CARTESIAN_POINT('Ctrl Pts',(-9.28488814777285,18.8014529345546,4.43581709221581));
#99653=CARTESIAN_POINT('Ctrl Pts',(-9.27965712295027,18.8019001466999,4.43179650551133));
#99654=CARTESIAN_POINT('Ctrl Pts',(-9.262843366865,18.8033526300943,4.41864718527559));
#99655=CARTESIAN_POINT('Ctrl Pts',(-9.25139863752396,18.8043646990453,4.40934510419292));
#99656=CARTESIAN_POINT('Ctrl Pts',(-9.17259011493072,18.8115030777121,4.34279474460592));
#99657=CARTESIAN_POINT('Ctrl Pts',(-9.1116970333334,18.8179338696165,4.2783458041946));
#99658=CARTESIAN_POINT('Ctrl Pts',(-9.01698953687469,18.8295073344187,4.15236460862125));
#99659=CARTESIAN_POINT('Ctrl Pts',(-8.98034050004862,18.8345957388571,4.09345243026744));
#99660=CARTESIAN_POINT('Ctrl Pts',(-8.94582230754721,18.8399185740493,4.02522039534986));
#99661=CARTESIAN_POINT('Ctrl Pts',(-8.94262590536818,18.8404174881118,4.01875533874997));
#99662=CARTESIAN_POINT('Ctrl Pts',(-8.93795373797049,18.8411554383152,4.00908276226169));
#99663=CARTESIAN_POINT('Ctrl Pts',(-8.93643275453944,18.8413970954451,4.00589745673323));
#99664=CARTESIAN_POINT('Ctrl Pts',(-8.93384947230673,18.8418099371504,4.00042429689303));
#99665=CARTESIAN_POINT('Ctrl Pts',(-8.93278018035464,18.8419815440292,3.99813982135499));
#99666=CARTESIAN_POINT('Ctrl Pts',(-8.93036758694839,18.8423703712356,3.99294203986458));
#99667=CARTESIAN_POINT('Ctrl Pts',(-8.92902884404964,18.8425873125774,3.99002667015233));
#99668=CARTESIAN_POINT('Ctrl Pts',(-8.92541806257408,18.8431757774832,3.98207802010986));
#99669=CARTESIAN_POINT('Ctrl Pts',(-8.9231694495525,18.8435459164192,3.97703409344848));
#99670=CARTESIAN_POINT('Ctrl Pts',(-8.91216807814261,18.8453762827659,3.95188239101155));
#99671=CARTESIAN_POINT('Ctrl Pts',(-8.90394201365645,18.8468076310177,3.93154724570624));
#99672=CARTESIAN_POINT('Ctrl Pts',(-8.88858831600686,18.8496364922881,3.89031522561151));
#99673=CARTESIAN_POINT('Ctrl Pts',(-8.88147077724173,18.8510331798768,3.86942439229194));
#99674=CARTESIAN_POINT('Ctrl Pts',(-8.84550770964435,18.8586603570588,3.75327382426828));
#99675=CARTESIAN_POINT('Ctrl Pts',(-8.82824092380558,18.8646545588853,3.65485873449201));
#99676=CARTESIAN_POINT('Ctrl Pts',(-8.8222610540194,18.8727964767225,3.52797128486702));
#99677=CARTESIAN_POINT('Ctrl Pts',(-8.82192911420155,18.8745830559791,3.50046485942088));
#99678=CARTESIAN_POINT('Ctrl Pts',(-8.82275382667612,18.8769568598176,3.46453515242739));
#99679=CARTESIAN_POINT('Ctrl Pts',(-8.82303822485137,18.8775170760411,3.45609918345885));
#99680=CARTESIAN_POINT('Ctrl Pts',(-8.82365249826855,18.8784392299313,3.44228861600316));
#99681=CARTESIAN_POINT('Ctrl Pts',(-8.82392860320771,18.8787994936257,3.43691183407034));
#99682=CARTESIAN_POINT('Ctrl Pts',(-8.82453522350282,18.879500034427,3.42649392786755));
#99683=CARTESIAN_POINT('Ctrl Pts',(-8.82486132861812,18.8798401669265,3.42145265709528));
#99684=CARTESIAN_POINT('Ctrl Pts',(-8.82569194610124,18.8806305231952,3.40977857875488));
#99685=CARTESIAN_POINT('Ctrl Pts',(-8.82622023479299,18.8810814766345,3.40314769007917));
#99686=CARTESIAN_POINT('Ctrl Pts',(-8.82812743760418,18.8825588522177,3.38152458153715));
#99687=CARTESIAN_POINT('Ctrl Pts',(-8.82973760723348,18.8835924014127,3.36655479477446));
#99688=CARTESIAN_POINT('Ctrl Pts',(-8.84178115992368,18.8902113239789,3.27172173876614));
#99689=CARTESIAN_POINT('Ctrl Pts',(-8.86009520994865,18.8960441044976,3.19308881839438));
#99690=CARTESIAN_POINT('Ctrl Pts',(-8.90422769455571,18.9060013798844,3.06477244706115));
#99691=CARTESIAN_POINT('Ctrl Pts',(-8.92582023411268,18.9100678746802,3.01391526458323));
#99692=CARTESIAN_POINT('Ctrl Pts',(-8.95827258610392,18.9151886538216,2.95030715282623));
#99693=CARTESIAN_POINT('Ctrl Pts',(-8.9659432582124,18.9163417535588,2.9360098035996));
#99694=CARTESIAN_POINT('Ctrl Pts',(-8.97921656770736,18.9182400549069,2.91245150531441));
#99695=CARTESIAN_POINT('Ctrl Pts',(-8.98465566548599,18.9189930110098,2.90310138838998));
#99696=CARTESIAN_POINT('Ctrl Pts',(-8.9923604750014,18.9200245784108,2.89026653646036));
#99697=CARTESIAN_POINT('Ctrl Pts',(-8.99451676711371,18.9203096297034,2.88671721155589));
#99698=CARTESIAN_POINT('Ctrl Pts',(-8.99819938561159,18.9207902369444,2.88072713822424));
#99699=CARTESIAN_POINT('Ctrl Pts',(-8.99971595529528,18.92098641062,2.87828046604329));
#99700=CARTESIAN_POINT('Ctrl Pts',(-9.00264202663417,18.9213615385439,2.87359827650141));
#99701=CARTESIAN_POINT('Ctrl Pts',(-9.00405009653638,18.9215405868746,2.8713619193993));
#99702=CARTESIAN_POINT('Ctrl Pts',(-9.00744427543182,18.9219687309554,2.86601116742432));
#99703=CARTESIAN_POINT('Ctrl Pts',(-9.00943754722302,18.922217363406,2.86290131512426));
#99704=CARTESIAN_POINT('Ctrl Pts',(-9.0167209687425,18.9231159823095,2.85165472198858));
#99705=CARTESIAN_POINT('Ctrl Pts',(-9.02209718810573,18.9237606189912,2.84357379824361));
#99706=CARTESIAN_POINT('Ctrl Pts',(-9.0652349927705,18.9287964916085,2.78044038299123));
#99707=CARTESIAN_POINT('Ctrl Pts',(-9.10752085595098,18.9329318063801,2.72861481815714));
#99708=CARTESIAN_POINT('Ctrl Pts',(-9.19818303686321,18.9409909211741,2.63500154558711));
#99709=CARTESIAN_POINT('Ctrl Pts',(-9.24600791555207,18.9449037011179,2.59301157438885));
#99710=CARTESIAN_POINT('Ctrl Pts',(-9.31446399144532,18.9503384853983,2.54208032239438));
#99711=CARTESIAN_POINT('Ctrl Pts',(-9.33230027919226,18.9517401450621,2.52956364287481));
#99712=CARTESIAN_POINT('Ctrl Pts',(-9.36363722912782,18.9541873266529,2.5088458527334));
#99713=CARTESIAN_POINT('Ctrl Pts',(-9.37697488287497,18.9552242628136,2.50040819097376));
#99714=CARTESIAN_POINT('Ctrl Pts',(-9.39634012117295,18.9567254000042,2.48869551760604));
#99715=CARTESIAN_POINT('Ctrl Pts',(-9.40223341988969,18.9571816534026,2.48520094709104));
#99716=CARTESIAN_POINT('Ctrl Pts',(-9.41253599520039,18.9579784413068,2.47921267536463));
#99717=CARTESIAN_POINT('Ctrl Pts',(-9.41693153481843,18.9583181277069,2.4766956060828));
#99718=CARTESIAN_POINT('Ctrl Pts',(-9.42544709363859,18.9589757781765,2.47189192079601));
#99719=CARTESIAN_POINT('Ctrl Pts',(-9.42956487466947,18.9592935992385,2.46960151814644));
#99720=CARTESIAN_POINT('Ctrl Pts',(-9.43937487471307,18.9600503650681,2.46422180172666));
#99721=CARTESIAN_POINT('Ctrl Pts',(-9.44507900074691,18.960490081181,2.46115463672748));
#99722=CARTESIAN_POINT('Ctrl Pts',(-9.46549734818217,18.9620631627094,2.45039164019521));
#99723=CARTESIAN_POINT('Ctrl Pts',(-9.48034808147334,18.9632056552988,2.44296044141348));
#99724=CARTESIAN_POINT('Ctrl Pts',(-9.59547369030641,18.9720544317322,2.38836486407111));
#99725=CARTESIAN_POINT('Ctrl Pts',(-9.70177990851533,18.9802562432334,2.35526108830259));
#99726=CARTESIAN_POINT('Ctrl Pts',(-9.81110406455739,18.9883401336252,2.33749692986502));
#99727=CARTESIAN_POINT('Origin',(-10.,12.3756328852638,3.5));
#99728=CARTESIAN_POINT('',(-9.81110406371044,19.5876476368634,2.33749693000264));
#99729=CARTESIAN_POINT('',(-9.81110408816073,19.4882767440992,2.3374969260297));
#99730=CARTESIAN_POINT('',(-9.81110406371068,12.3756328852638,2.3374969300026));
#99731=CARTESIAN_POINT('Ctrl Pts',(-9.8111040637102,19.5876476368634,2.33749693000268));
#99732=CARTESIAN_POINT('Ctrl Pts',(-9.8106956841937,19.5876198932078,2.33756328787572));
#99733=CARTESIAN_POINT('Ctrl Pts',(-9.81028733975649,19.5875921427914,2.33762986092192));
#99734=CARTESIAN_POINT('Ctrl Pts',(-9.80493802576696,19.5872284921535,2.33850486206574));
#99735=CARTESIAN_POINT('Ctrl Pts',(-9.80000229175874,19.5868916146335,2.33934456249868));
#99736=CARTESIAN_POINT('Ctrl Pts',(-9.78872733839253,19.5861189224998,2.34133678830245));
#99737=CARTESIAN_POINT('Ctrl Pts',(-9.78239196873605,19.5856824678243,2.34250990606972));
#99738=CARTESIAN_POINT('Ctrl Pts',(-9.76279833730254,19.5843253753953,2.34630459606175));
#99739=CARTESIAN_POINT('Ctrl Pts',(-9.74957574175851,19.5833992200025,2.34910235978295));
#99740=CARTESIAN_POINT('Ctrl Pts',(-9.63747226563818,19.5754557336399,2.37484558205097));
#99741=CARTESIAN_POINT('Ctrl Pts',(-9.5419103071493,19.5680207909528,2.4102550182968));
#99742=CARTESIAN_POINT('Ctrl Pts',(-9.40074895210856,19.5563221770524,2.48444220930991));
#99743=CARTESIAN_POINT('Ctrl Pts',(-9.35146172340673,19.5520928430861,2.51518572825358));
#99744=CARTESIAN_POINT('Ctrl Pts',(-9.29880367410118,19.5475510424629,2.55370670596388));
#99745=CARTESIAN_POINT('Ctrl Pts',(-9.29301033178312,19.5470510838542,2.55802712279558));
#99746=CARTESIAN_POINT('Ctrl Pts',(-9.28444403644062,19.5463118476351,2.56453903857251));
#99747=CARTESIAN_POINT('Ctrl Pts',(-9.28164071803438,19.5460699368752,2.56669003531547));
#99748=CARTESIAN_POINT('Ctrl Pts',(-9.27685198211089,19.5456567631575,2.57039880882308));
#99749=CARTESIAN_POINT('Ctrl Pts',(-9.27486184923668,19.5454850764904,2.57195038216381));
#99750=CARTESIAN_POINT('Ctrl Pts',(-9.27035342446886,19.5450962002686,2.57548865583267));
#99751=CARTESIAN_POINT('Ctrl Pts',(-9.26783825203655,19.5448792890736,2.57747925436928));
#99752=CARTESIAN_POINT('Ctrl Pts',(-9.2610189228686,19.5442911838022,2.582921774973));
#99753=CARTESIAN_POINT('Ctrl Pts',(-9.25673077265675,19.5439213709027,2.58639375996656));
#99754=CARTESIAN_POINT('Ctrl Pts',(-9.23557728067456,19.542096179599,2.60376861916769));
#99755=CARTESIAN_POINT('Ctrl Pts',(-9.21907561138594,19.5406694813505,2.61810996780136));
#99756=CARTESIAN_POINT('Ctrl Pts',(-9.18672714268573,19.5378441526877,2.64784405864006));
#99757=CARTESIAN_POINT('Ctrl Pts',(-9.17089530889,19.5364465145444,2.66323958178222));
#99758=CARTESIAN_POINT('Ctrl Pts',(-9.08614423523973,19.5288190174745,2.75042365757527));
#99759=CARTESIAN_POINT('Ctrl Pts',(-9.02610783460518,19.5228259078037,2.83027498617237));
#99760=CARTESIAN_POINT('Ctrl Pts',(-8.96317202482156,19.5146813445591,2.94067642200042));
#99761=CARTESIAN_POINT('Ctrl Pts',(-8.95036472393774,19.5128905146499,2.96509747489161));
#99762=CARTESIAN_POINT('Ctrl Pts',(-8.93476737401636,19.5105117359612,2.99756004217785));
#99763=CARTESIAN_POINT('Ctrl Pts',(-8.9311901870933,19.5099509362705,3.005215161584));
#99764=CARTESIAN_POINT('Ctrl Pts',(-8.92546779331963,19.5090279861705,3.017812671825));
#99765=CARTESIAN_POINT('Ctrl Pts',(-8.92327354130888,19.5086675143326,3.02273255489377));
#99766=CARTESIAN_POINT('Ctrl Pts',(-8.91908664987462,19.5079666853692,3.03229611386409));
#99767=CARTESIAN_POINT('Ctrl Pts',(-8.91708998819997,19.5076264737208,3.03693790852968));
#99768=CARTESIAN_POINT('Ctrl Pts',(-8.91253458106892,19.5068361042433,3.04771882609351));
#99769=CARTESIAN_POINT('Ctrl Pts',(-8.90999786629261,19.5063852177268,3.05386701198037));
#99770=CARTESIAN_POINT('Ctrl Pts',(-8.9018941803872,19.5049088100926,3.07398950644592));
#99771=CARTESIAN_POINT('Ctrl Pts',(-8.89654302512441,19.5038761768603,3.08804854676251));
#99772=CARTESIAN_POINT('Ctrl Pts',(-8.86405164042408,19.4972156703019,3.17859259323325));
#99773=CARTESIAN_POINT('Ctrl Pts',(-8.84461417871865,19.4913361910959,3.25759442138906));
#99774=CARTESIAN_POINT('Ctrl Pts',(-8.82592424551814,19.481367545464,3.39213844431413));
#99775=CARTESIAN_POINT('Ctrl Pts',(-8.82218128266783,19.4773368932779,3.44678689843661));
#99776=CARTESIAN_POINT('Ctrl Pts',(-8.82227151734088,19.4722560852462,3.51764721967909));
#99777=CARTESIAN_POINT('Ctrl Pts',(-8.8226241623562,19.471108453926,3.53379342039898));
#99778=CARTESIAN_POINT('Ctrl Pts',(-8.82376574628731,19.4692181209239,3.56069795752622));
#99779=CARTESIAN_POINT('Ctrl Pts',(-8.82437058131702,19.4684677444576,3.57146154421775));
#99780=CARTESIAN_POINT('Ctrl Pts',(-8.82541272043861,19.4674390344187,3.58635388213993));
#99781=CARTESIAN_POINT('Ctrl Pts',(-8.82572416375481,19.46715430793,3.5904905077468));
#99782=CARTESIAN_POINT('Ctrl Pts',(-8.82628871929852,19.4666740387315,3.59749449619904));
#99783=CARTESIAN_POINT('Ctrl Pts',(-8.82653049699069,19.4664778808321,3.60036270930273));
#99784=CARTESIAN_POINT('Ctrl Pts',(-8.8270146263591,19.4661026144689,3.60586487455948));
#99785=CARTESIAN_POINT('Ctrl Pts',(-8.8272553379598,19.465923412848,3.60849892372828));
#99786=CARTESIAN_POINT('Ctrl Pts',(-8.82785408274519,19.4654946782989,3.61481595411492));
#99787=CARTESIAN_POINT('Ctrl Pts',(-8.8282206059166,19.4652456111362,3.61849813155037));
#99788=CARTESIAN_POINT('Ctrl Pts',(-8.82961591937848,19.4643435867982,3.63187579482989));
#99789=CARTESIAN_POINT('Ctrl Pts',(-8.83074777237364,19.4636960328355,3.64156046360809));
#99790=CARTESIAN_POINT('Ctrl Pts',(-8.83986891074685,19.4590182895021,3.71200592541082));
#99791=CARTESIAN_POINT('Ctrl Pts',(-8.85247072763083,19.4552027831496,3.77208311552354));
#99792=CARTESIAN_POINT('Ctrl Pts',(-8.88848401559368,19.4472677703029,3.8950944265588));
#99793=CARTESIAN_POINT('Ctrl Pts',(-8.91270515660466,19.4431630858671,3.95755512088264));
#99794=CARTESIAN_POINT('Ctrl Pts',(-8.95734718434812,19.4367056664832,4.0487936943912));
#99795=CARTESIAN_POINT('Ctrl Pts',(-8.97396849734466,19.4344649549755,4.07927403435532));
#99796=CARTESIAN_POINT('Ctrl Pts',(-8.99662360531662,19.4315754526703,4.11677708979781));
#99797=CARTESIAN_POINT('Ctrl Pts',(-9.00142761265321,19.4309711195921,4.12452489734398));
#99798=CARTESIAN_POINT('Ctrl Pts',(-9.00929092582271,19.4299947460041,4.13688397979329));
#99799=CARTESIAN_POINT('Ctrl Pts',(-9.01229369565801,19.4296247819132,4.14153092517949));
#99800=CARTESIAN_POINT('Ctrl Pts',(-9.01807594630742,19.4289177066454,4.15034243516118));
#99801=CARTESIAN_POINT('Ctrl Pts',(-9.0208494668279,19.428580822163,4.15451078084832));
#99802=CARTESIAN_POINT('Ctrl Pts',(-9.02725319283781,19.4278080698531,4.16400318888897));
#99803=CARTESIAN_POINT('Ctrl Pts',(-9.03090065749793,19.4273715616076,4.16931535705772));
#99804=CARTESIAN_POINT('Ctrl Pts',(-9.04233491616776,19.4260141346446,4.1856787962801));
#99805=CARTESIAN_POINT('Ctrl Pts',(-9.05026829596698,19.4250876943656,4.19662578785773));
#99806=CARTESIAN_POINT('Ctrl Pts',(-9.11934078999104,19.4171460840526,4.28856304071154));
#99807=CARTESIAN_POINT('Ctrl Pts',(-9.19051208496895,19.4097136085619,4.36145986912364));
#99808=CARTESIAN_POINT('Ctrl Pts',(-9.3156602931893,19.3980154833449,4.4602819690286));
#99809=CARTESIAN_POINT('Ctrl Pts',(-9.36380281102323,19.3937842799183,4.49283283272144));
#99810=CARTESIAN_POINT('Ctrl Pts',(-9.42042395604104,19.3892407118303,4.52529942222084));
#99811=CARTESIAN_POINT('Ctrl Pts',(-9.42672680911896,19.3887407039534,4.52883679518127));
#99812=CARTESIAN_POINT('Ctrl Pts',(-9.43615921276475,19.3880014094091,4.5340169800198));
#99813=CARTESIAN_POINT('Ctrl Pts',(-9.43926409502501,19.3877594890015,4.53570400888317));
#99814=CARTESIAN_POINT('Ctrl Pts',(-9.44459929430523,19.387346304537,4.53857184951618));
#99815=CARTESIAN_POINT('Ctrl Pts',(-9.44682585963015,19.3871746167073,4.53975949207676));
#99816=CARTESIAN_POINT('Ctrl Pts',(-9.4518911353612,19.386785745604,4.54244041680038));
#99817=CARTESIAN_POINT('Ctrl Pts',(-9.45473213902915,19.3865688406419,4.54392926507899));
#99818=CARTESIAN_POINT('Ctrl Pts',(-9.46247619763173,19.3859807688938,4.5479473558097));
#99819=CARTESIAN_POINT('Ctrl Pts',(-9.46739107478083,19.3856109830224,4.55045382307065));
#99820=CARTESIAN_POINT('Ctrl Pts',(-9.49185942519379,19.3837861421393,4.56271620129751));
#99821=CARTESIAN_POINT('Ctrl Pts',(-9.51166557592804,19.3823597541224,4.57196184925302));
#99822=CARTESIAN_POINT('Ctrl Pts',(-9.55197741244406,19.3795346594245,4.58943025924289));
#99823=CARTESIAN_POINT('Ctrl Pts',(-9.57247968743308,19.3781369562045,4.59763792233992));
#99824=CARTESIAN_POINT('Ctrl Pts',(-9.68657886661173,19.3705098470289,4.63963272065532));
#99825=CARTESIAN_POINT('Ctrl Pts',(-9.78393132078789,19.3645171930309,4.66202855537848));
#99826=CARTESIAN_POINT('Ctrl Pts',(-9.91038484356188,19.3563725682798,4.67465943783982));
#99827=CARTESIAN_POINT('Ctrl Pts',(-9.93791331513044,19.3545810991138,4.67643560114346));
#99828=CARTESIAN_POINT('Ctrl Pts',(-9.97392420066801,19.35220158984,4.6774916260664));
#99829=CARTESIAN_POINT('Ctrl Pts',(-9.98237349828021,19.3516407202029,4.6776484097632));
#99830=CARTESIAN_POINT('Ctrl Pts',(-9.9962106758143,19.3507176844233,4.67775622527403));
#99831=CARTESIAN_POINT('Ctrl Pts',(-10.0015979264835,19.3503571974653,4.67776123647286));
#99832=CARTESIAN_POINT('Ctrl Pts',(-10.0120377878676,19.3496563601732,4.67769931912421));
#99833=CARTESIAN_POINT('Ctrl Pts',(-10.0170903147317,19.3493161554538,4.67763683467039));
#99834=CARTESIAN_POINT('Ctrl Pts',(-10.0287914029237,19.348525833177,4.67741681019818));
#99835=CARTESIAN_POINT('Ctrl Pts',(-10.0354392901257,19.3480749872009,4.67723546641299));
#99836=CARTESIAN_POINT('Ctrl Pts',(-10.0571144547687,19.3465988506789,4.67646044123919));
#99837=CARTESIAN_POINT('Ctrl Pts',(-10.0721314311017,19.3455664516452,4.67563525421626));
#99838=CARTESIAN_POINT('Ctrl Pts',(-10.1681915179273,19.3388972049503,4.66850936938903));
#99839=CARTESIAN_POINT('Ctrl Pts',(-10.2484001980322,19.3330078572726,4.65412101550457));
#99840=CARTESIAN_POINT('Ctrl Pts',(-10.378943439907,19.3230366994419,4.61645828905838));
#99841=CARTESIAN_POINT('Ctrl Pts',(-10.4302987607397,19.3190135001058,4.59768884080807));
#99842=CARTESIAN_POINT('Ctrl Pts',(-10.4948981918747,19.3139410300771,4.56884567133155));
#99843=CARTESIAN_POINT('Ctrl Pts',(-10.509492291535,19.3127945597147,4.56196654809367));
#99844=CARTESIAN_POINT('Ctrl Pts',(-10.5335882617895,19.3109059301653,4.54999745630386));
#99845=CARTESIAN_POINT('Ctrl Pts',(-10.5431695788278,19.3101561128229,4.54507316522657));
#99846=CARTESIAN_POINT('Ctrl Pts',(-10.5563444570962,19.3091280350536,4.53807182093451));
#99847=CARTESIAN_POINT('Ctrl Pts',(-10.5599962784974,19.308843391771,4.53610637954867));
#99848=CARTESIAN_POINT('Ctrl Pts',(-10.5661648144221,19.3083632215399,4.53274428045651));
#99849=CARTESIAN_POINT('Ctrl Pts',(-10.5686869078735,19.3081670799818,4.53135762342437));
#99850=CARTESIAN_POINT('Ctrl Pts',(-10.5735172639854,19.3077918122062,4.52867876801562));
#99851=CARTESIAN_POINT('Ctrl Pts',(-10.5758262801741,19.3076125930233,4.5273880256599));
#99852=CARTESIAN_POINT('Ctrl Pts',(-10.581355634832,19.3071837737372,4.52427261408499));
#99853=CARTESIAN_POINT('Ctrl Pts',(-10.5845717841478,19.3069346398103,4.52244050791106));
#99854=CARTESIAN_POINT('Ctrl Pts',(-10.5962349840046,19.306032021093,4.51572344655203));
#99855=CARTESIAN_POINT('Ctrl Pts',(-10.6046301645907,19.305383949116,4.51074856188911));
#99856=CARTESIAN_POINT('Ctrl Pts',(-10.6661152699253,19.30064226317,4.47327295082016));
#99857=CARTESIAN_POINT('Ctrl Pts',(-10.716623094347,19.2967702573103,4.43670870784371));
#99858=CARTESIAN_POINT('Ctrl Pts',(-10.8143475464967,19.2888226885183,4.35340978179612));
#99859=CARTESIAN_POINT('Ctrl Pts',(-10.8609793736319,19.2847604850198,4.30633991809418));
#99860=CARTESIAN_POINT('Ctrl Pts',(-10.9180482090711,19.2791042454602,4.23810768157349));
#99861=CARTESIAN_POINT('Ctrl Pts',(-10.9321715940122,19.2776387399431,4.22018850604801));
#99862=CARTESIAN_POINT('Ctrl Pts',(-10.9555064872461,19.2750902707694,4.18874495398788));
#99863=CARTESIAN_POINT('Ctrl Pts',(-10.9649731051117,19.2740169116794,4.17541773927282));
#99864=CARTESIAN_POINT('Ctrl Pts',(-10.9780641416069,19.2724723249141,4.15615080749571));
#99865=CARTESIAN_POINT('Ctrl Pts',(-10.9819183274051,19.272009704083,4.15036892769035));
#99866=CARTESIAN_POINT('Ctrl Pts',(-10.988502919933,19.2712053595044,4.14029905347018));
#99867=CARTESIAN_POINT('Ctrl Pts',(-10.9912571751282,19.270864529619,4.1360268170144));
#99868=CARTESIAN_POINT('Ctrl Pts',(-10.9964996931501,19.2702072068537,4.12777816656594));
#99869=CARTESIAN_POINT('Ctrl Pts',(-10.9989920303147,19.2698908720284,4.12380444622677));
#99870=CARTESIAN_POINT('Ctrl Pts',(-11.0048226328033,19.2691416252343,4.11438371758833));
#99871=CARTESIAN_POINT('Ctrl Pts',(-11.0081404187772,19.2687079784874,4.10892427202413));
#99872=CARTESIAN_POINT('Ctrl Pts',(-11.0179275779915,19.2674064757458,4.09252016356392));
#99873=CARTESIAN_POINT('Ctrl Pts',(-11.0242641416544,19.2665339038608,4.08149775954924));
#99874=CARTESIAN_POINT('Ctrl Pts',(-11.0770612804849,19.2589972112251,3.98611622593119));
#99875=CARTESIAN_POINT('Ctrl Pts',(-11.11318201831,19.2519617598073,3.89646999741244));
#99876=CARTESIAN_POINT('Ctrl Pts',(-11.1539854625533,19.2403363299881,3.74345152269383));
#99877=CARTESIAN_POINT('Ctrl Pts',(-11.1652165621076,19.2357946717337,3.68227247097775));
#99878=CARTESIAN_POINT('Ctrl Pts',(-11.1723214424347,19.23095863704,3.61318722314911));
#99879=CARTESIAN_POINT('Ctrl Pts',(-11.1730039452346,19.2304508412068,3.60588041934202));
#99880=CARTESIAN_POINT('Ctrl Pts',(-11.1739156800366,19.2297023343447,3.59502462347152));
#99881=CARTESIAN_POINT('Ctrl Pts',(-11.1741971916666,19.2294588954618,3.59148037398434));
#99882=CARTESIAN_POINT('Ctrl Pts',(-11.1746711335742,19.2290258525456,3.58515037969062));
#99883=CARTESIAN_POINT('Ctrl Pts',(-11.1748697107118,19.2288359170841,3.58236517840755));
#99884=CARTESIAN_POINT('Ctrl Pts',(-11.1752812898076,19.2284227988759,3.57628784343758));
#99885=CARTESIAN_POINT('Ctrl Pts',(-11.1754903662571,19.2281998343281,3.57299551176822));
#99886=CARTESIAN_POINT('Ctrl Pts',(-11.1760358612897,19.2275789522069,3.56379451391262));
#99887=CARTESIAN_POINT('Ctrl Pts',(-11.1763415874712,19.2271826826438,3.55788402425024));
#99888=CARTESIAN_POINT('Ctrl Pts',(-11.177818798241,19.2249537298614,3.5244407718917));
#99889=CARTESIAN_POINT('Ctrl Pts',(-11.1780683239467,19.2231671307076,3.49687343688583));
#99890=CARTESIAN_POINT('Ctrl Pts',(-11.174745672095,19.21503415865,3.36936469083023));
#99891=CARTESIAN_POINT('Ctrl Pts',(-11.1594230897485,19.2090437502883,3.27014359740419));
#99892=CARTESIAN_POINT('Ctrl Pts',(-11.1205102474291,19.2001577518134,3.13503425940814));
#99893=CARTESIAN_POINT('Ctrl Pts',(-11.1072660814476,19.1975490029927,3.09663356699073));
#99894=CARTESIAN_POINT('Ctrl Pts',(-11.0884899344784,19.1942452733048,3.05013781052806));
#99895=CARTESIAN_POINT('Ctrl Pts',(-11.0848052020531,19.1936124253297,3.04132365256052));
#99896=CARTESIAN_POINT('Ctrl Pts',(-11.078779855658,19.1926010132917,3.02738941586182));
#99897=CARTESIAN_POINT('Ctrl Pts',(-11.0765090010053,19.1922248043069,3.02223948457464));
#99898=CARTESIAN_POINT('Ctrl Pts',(-11.0721559538404,19.1915127770178,3.01255609618663));
#99899=CARTESIAN_POINT('Ctrl Pts',(-11.0700816941445,19.1911772347577,3.00801919218443));
#99900=CARTESIAN_POINT('Ctrl Pts',(-11.0653318691927,19.1904171469972,2.99780233908241));
#99901=CARTESIAN_POINT('Ctrl Pts',(-11.0626395993961,19.1899920366627,2.9921303697872));
#99902=CARTESIAN_POINT('Ctrl Pts',(-11.0555969307692,19.1888943205306,2.97759433637464));
#99903=CARTESIAN_POINT('Ctrl Pts',(-11.0511802517357,19.1882194487497,2.96876311719355));
#99904=CARTESIAN_POINT('Ctrl Pts',(-11.0122489782288,19.1823828447992,2.89330628667435));
#99905=CARTESIAN_POINT('Ctrl Pts',(-10.9715577346623,19.1770001176065,2.83007690835861));
#99906=CARTESIAN_POINT('Ctrl Pts',(-10.8916610612483,19.1675561888095,2.72866209896345));
#99907=CARTESIAN_POINT('Ctrl Pts',(-10.8552950529299,19.1635605183903,2.68852475031126));
#99908=CARTESIAN_POINT('Ctrl Pts',(-10.7986896225448,19.1578623575284,2.63409775587127));
#99909=CARTESIAN_POINT('Ctrl Pts',(-10.7805569078029,19.1561059836174,2.61771723405829));
#99910=CARTESIAN_POINT('Ctrl Pts',(-10.7510466058762,19.1533698256869,2.59268107189906));
#99911=CARTESIAN_POINT('Ctrl Pts',(-10.7399990531984,19.1523711640608,2.58364849076324));
#99912=CARTESIAN_POINT('Ctrl Pts',(-10.725035338242,19.1510552117457,2.57186118516298));
#99913=CARTESIAN_POINT('Ctrl Pts',(-10.7212631507058,19.1507265161419,2.56892676403983));
#99914=CARTESIAN_POINT('Ctrl Pts',(-10.715321813714,19.1502136896766,2.56436271741215));
#99915=CARTESIAN_POINT('Ctrl Pts',(-10.7131647712895,19.1500285031694,2.56271752864176));
#99916=CARTESIAN_POINT('Ctrl Pts',(-10.7087431876435,19.1496509701811,2.55936926227273));
#99917=CARTESIAN_POINT('Ctrl Pts',(-10.7064781762765,19.1494586809308,2.55766689679374));
#99918=CARTESIAN_POINT('Ctrl Pts',(-10.7010840180038,19.1490033158699,2.55364306811529));
#99919=CARTESIAN_POINT('Ctrl Pts',(-10.6979494210103,19.1487407401611,2.55132890334686));
#99920=CARTESIAN_POINT('Ctrl Pts',(-10.6873697325875,19.1478611352126,2.54359910624135));
#99921=CARTESIAN_POINT('Ctrl Pts',(-10.679872411318,19.1472487570888,2.53825505659178));
#99922=CARTESIAN_POINT('Ctrl Pts',(-10.6615627362757,19.1457774943533,2.52552514797931));
#99923=CARTESIAN_POINT('Ctrl Pts',(-10.6506881834625,19.1449237666295,2.51823046994007));
#99924=CARTESIAN_POINT('Ctrl Pts',(-10.6075625500915,19.14160654792,2.4903330989449));
#99925=CARTESIAN_POINT('Ctrl Pts',(-10.574434766068,19.1392053375714,2.47112456541489));
#99926=CARTESIAN_POINT('Ctrl Pts',(-10.4591552371363,19.1311387053694,2.41158898337292));
#99927=CARTESIAN_POINT('Ctrl Pts',(-10.3732759380905,19.1255777229304,2.37922963955132));
#99928=CARTESIAN_POINT('Ctrl Pts',(-10.2622037901675,19.118203443365,2.35157801345508));
#99929=CARTESIAN_POINT('Ctrl Pts',(-10.2397321174924,19.1167044416958,2.3466777185466));
#99930=CARTESIAN_POINT('Ctrl Pts',(-10.2090874968363,19.1146437741221,2.34092947517724));
#99931=CARTESIAN_POINT('Ctrl Pts',(-10.2010270943222,19.1141002450309,2.33950434530639));
#99932=CARTESIAN_POINT('Ctrl Pts',(-10.188220260191,19.1132339742015,2.33737744326176));
#99933=CARTESIAN_POINT('Ctrl Pts',(-10.1834831654121,19.1129129720343,2.33662043913711));
#99934=CARTESIAN_POINT('Ctrl Pts',(-10.1737767020248,19.1122539802591,2.33513007075103));
#99935=CARTESIAN_POINT('Ctrl Pts',(-10.1688070082855,19.1119159098104,2.33439951662607));
#99936=CARTESIAN_POINT('Ctrl Pts',(-10.1573281499135,19.1111334316065,2.33278705375207));
#99937=CARTESIAN_POINT('Ctrl Pts',(-10.1508160280395,19.1106883260799,2.33192777137197));
#99938=CARTESIAN_POINT('Ctrl Pts',(-10.1302187937222,19.1092765389521,2.32938505497077));
#99939=CARTESIAN_POINT('Ctrl Pts',(-10.1161107285061,19.1083036794701,2.32790164581325));
#99940=CARTESIAN_POINT('Ctrl Pts',(-10.0048866778155,19.1005846743167,2.31823459263072));
#99941=CARTESIAN_POINT('Ctrl Pts',(-9.90717910965791,19.0934618621443,2.3218856286421));
#99942=CARTESIAN_POINT('Ctrl Pts',(-9.81110406371067,19.0863176770662,2.3374969300026));
#99943=CARTESIAN_POINT('Ctrl Pts',(-9.81110406455739,18.9883401336252,2.33749692986502));
#99944=CARTESIAN_POINT('Ctrl Pts',(-9.81189205314573,18.9883984008336,2.33736888904918));
#99945=CARTESIAN_POINT('Ctrl Pts',(-9.81268019879629,18.9884566579951,2.337241645059));
#99946=CARTESIAN_POINT('Ctrl Pts',(-9.81924205121837,18.9889415058973,2.33618909697252));
#99947=CARTESIAN_POINT('Ctrl Pts',(-9.82502247354454,18.9893674370338,2.33530599702566));
#99948=CARTESIAN_POINT('Ctrl Pts',(-9.84362289189887,18.99073382975,2.33260593164355));
#99949=CARTESIAN_POINT('Ctrl Pts',(-9.8564666697997,18.9916709747609,2.33095726650433));
#99950=CARTESIAN_POINT('Ctrl Pts',(-9.89543850473922,18.9944909464256,2.32660670646343));
#99951=CARTESIAN_POINT('Ctrl Pts',(-9.92163423104744,18.9963545400001,2.32456647167613));
#99952=CARTESIAN_POINT('Ctrl Pts',(-9.95371076337799,18.9985811855376,2.32314552655112));
#99953=CARTESIAN_POINT('Ctrl Pts',(-9.95954506704566,18.9989839461617,2.3229305258247));
#99954=CARTESIAN_POINT('Ctrl Pts',(-9.96865956607076,18.9996094102215,2.32266249580014));
#99955=CARTESIAN_POINT('Ctrl Pts',(-9.97193869398526,18.999833678247,2.32257977537113));
#99956=CARTESIAN_POINT('Ctrl Pts',(-9.97801059692306,19.0002475003697,2.32245198411027));
#99957=CARTESIAN_POINT('Ctrl Pts',(-9.98080317409126,19.00043725048,2.32240314804824));
#99958=CARTESIAN_POINT('Ctrl Pts',(-9.98717328333599,19.0008687997829,2.3223144149104));
#99959=CARTESIAN_POINT('Ctrl Pts',(-9.9907508414021,19.0011102454604,2.32228088412237));
#99960=CARTESIAN_POINT('Ctrl Pts',(-10.0017848540761,19.0018522371462,2.32222774932222));
#99961=CARTESIAN_POINT('Ctrl Pts',(-10.0092415629017,19.0023498924901,2.32226265204395));
#99962=CARTESIAN_POINT('Ctrl Pts',(-10.0266543470689,19.0035042382997,2.32250954841646));
#99963=CARTESIAN_POINT('Ctrl Pts',(-10.0366092002199,19.0041582419678,2.32277699695217));
#99964=CARTESIAN_POINT('Ctrl Pts',(-10.0716330933409,19.0064420711815,2.3241626748515));
#99965=CARTESIAN_POINT('Ctrl Pts',(-10.0966699822243,19.0080438064635,2.32595579348566));
#99966=CARTESIAN_POINT('Ctrl Pts',(-10.1747248343379,19.0129927559335,2.33406023796024));
#99967=CARTESIAN_POINT('Ctrl Pts',(-10.2273836816288,19.0162690350865,2.34317613279208));
#99968=CARTESIAN_POINT('Ctrl Pts',(-10.3519219515578,19.0242051509125,2.37357084010858));
#99969=CARTESIAN_POINT('Ctrl Pts',(-10.422733662362,19.0288827843279,2.39818979955342));
#99970=CARTESIAN_POINT('Ctrl Pts',(-10.4996716100713,19.0344432753646,2.43345410417092));
#99971=CARTESIAN_POINT('Ctrl Pts',(-10.5085637795759,19.0350932894676,2.43766543013439));
#99972=CARTESIAN_POINT('Ctrl Pts',(-10.5230315928306,19.0361635387493,2.44474065366962));
#99973=CARTESIAN_POINT('Ctrl Pts',(-10.528639100796,19.036581506668,2.44753858329002));
#99974=CARTESIAN_POINT('Ctrl Pts',(-10.5386674645924,19.0373348131293,2.45264271372318));
#99975=CARTESIAN_POINT('Ctrl Pts',(-10.543096540745,19.0376695747316,2.45493250521958));
#99976=CARTESIAN_POINT('Ctrl Pts',(-10.5524977666803,19.0383846159816,2.45986875564176));
#99977=CARTESIAN_POINT('Ctrl Pts',(-10.5574657228561,19.0387651586176,2.46252289008022));
#99978=CARTESIAN_POINT('Ctrl Pts',(-10.5708294608431,19.0397962109814,2.46978617697981));
#99979=CARTESIAN_POINT('Ctrl Pts',(-10.5791882178002,19.0404490692031,2.47446219307755));
#99980=CARTESIAN_POINT('Ctrl Pts',(-10.623021682264,19.0439157895418,2.49969011879592));
#99981=CARTESIAN_POINT('Ctrl Pts',(-10.6574583371417,19.0467914741873,2.52197969869417));
#99982=CARTESIAN_POINT('Ctrl Pts',(-10.7741743438869,19.0570929373783,2.60647913381633));
#99983=CARTESIAN_POINT('Ctrl Pts',(-10.8493761760381,19.0648120420495,2.67763645828133));
#99984=CARTESIAN_POINT('Ctrl Pts',(-10.9297271778065,19.0739596454404,2.77660689621544));
#99985=CARTESIAN_POINT('Ctrl Pts',(-10.9445128290272,19.0756872975698,2.79602136036394));
#99986=CARTESIAN_POINT('Ctrl Pts',(-10.9620032069501,19.0777745941901,2.82053145164619));
#99987=CARTESIAN_POINT('Ctrl Pts',(-10.9652867901641,19.0781684705743,2.82520440544327));
#99988=CARTESIAN_POINT('Ctrl Pts',(-10.9703861706662,19.0787831210101,2.83257486354273));
#99989=CARTESIAN_POINT('Ctrl Pts',(-10.972224956786,19.0790053761679,2.83525623955779));
#99990=CARTESIAN_POINT('Ctrl Pts',(-10.9756097071975,19.0794155940427,2.84023607698023));
#99991=CARTESIAN_POINT('Ctrl Pts',(-10.9771586579055,19.0796037487341,2.84253236397246));
#99992=CARTESIAN_POINT('Ctrl Pts',(-10.9807042762711,19.0800354588645,2.84782887810893));
#99993=CARTESIAN_POINT('Ctrl Pts',(-10.9826952859495,19.0802786385019,2.85083282155834));
#99994=CARTESIAN_POINT('Ctrl Pts',(-10.9888376573041,19.0810313860975,2.86019316497468));
#99995=CARTESIAN_POINT('Ctrl Pts',(-10.9929414709376,19.0815379411159,2.86658075384337));
#99996=CARTESIAN_POINT('Ctrl Pts',(-11.0024086577133,19.0827162764613,2.88163457344487));
#99997=CARTESIAN_POINT('Ctrl Pts',(-11.0077219599714,19.083385213998,2.8903317419825));
#99998=CARTESIAN_POINT('Ctrl Pts',(-11.0261747808898,19.0857400634209,2.92143704458738));
#99999=CARTESIAN_POINT('Ctrl Pts',(-11.0386859046591,19.0873959575151,2.94421087642474));
#100000=CARTESIAN_POINT('Ctrl Pts',(-11.0872208888072,19.0941554969275,
3.0399319193915));
#100001=CARTESIAN_POINT('Ctrl Pts',(-11.1163928819923,19.0990817094154,
3.11609928607263));
#100002=CARTESIAN_POINT('Ctrl Pts',(-11.1495653537033,19.1071215196411,
3.23967973298724));
#100003=CARTESIAN_POINT('Ctrl Pts',(-11.1589641652929,19.1100998799162,
3.28536444107205));
#100004=CARTESIAN_POINT('Ctrl Pts',(-11.1670888008747,19.1138350786317,
3.34156223592039));
#100005=CARTESIAN_POINT('Ctrl Pts',(-11.1684152444552,19.1145089297948,
3.35166052435051));
#100006=CARTESIAN_POINT('Ctrl Pts',(-11.1702941776619,19.1155745987537,
3.36755932671859));
#100007=CARTESIAN_POINT('Ctrl Pts',(-11.170934896874,19.1159636613248,3.37334906465146));
#100008=CARTESIAN_POINT('Ctrl Pts',(-11.1720376680692,19.1166839252601,
3.38403884597848));
#100009=CARTESIAN_POINT('Ctrl Pts',(-11.1725120074326,19.1170147355265,
3.3889375140874));
#100010=CARTESIAN_POINT('Ctrl Pts',(-11.1734954831971,19.1177502579421,
3.39980377255104));
#100011=CARTESIAN_POINT('Ctrl Pts',(-11.1739898273686,19.1181554216222,
3.4057725304668));
#100012=CARTESIAN_POINT('Ctrl Pts',(-11.1752812159359,19.1193253778963,
3.42295740986853));
#100013=CARTESIAN_POINT('Ctrl Pts',(-11.1759631689081,19.1200937140982,
3.43418125401113));
#100014=CARTESIAN_POINT('Ctrl Pts',(-11.180261697679,19.1264723334255,3.52682481585399));
#100015=CARTESIAN_POINT('Ctrl Pts',(-11.1755778781871,19.1323450055113,
3.60839299785585));
#100016=CARTESIAN_POINT('Ctrl Pts',(-11.1499528239173,19.1440623183262,
3.76616913206904));
#100017=CARTESIAN_POINT('Ctrl Pts',(-11.1296970892666,19.1498658833319,
3.84208768647109));
#100018=CARTESIAN_POINT('Ctrl Pts',(-11.0987993056824,19.1559965644812,
3.92405180790112));
#100019=CARTESIAN_POINT('Ctrl Pts',(-11.0954502411605,19.1566362585339,
3.93262990214132));
#100020=CARTESIAN_POINT('Ctrl Pts',(-11.0906453688245,19.1575196343418,
3.94452315474922));
#100021=CARTESIAN_POINT('Ctrl Pts',(-11.0892744744104,19.1577679723586,
3.94787194142619));
#100022=CARTESIAN_POINT('Ctrl Pts',(-11.0868832168156,19.1581947722519,
3.95363731753049));
#100023=CARTESIAN_POINT('Ctrl Pts',(-11.0858701841215,19.1583736607045,
3.95605688947068));
#100024=CARTESIAN_POINT('Ctrl Pts',(-11.083721164944,19.1587491081053,3.96114194573337));
#100025=CARTESIAN_POINT('Ctrl Pts',(-11.0825834118613,19.1589455538531,
3.96380665598274));
#100026=CARTESIAN_POINT('Ctrl Pts',(-11.0797533432997,19.1594285713811,
3.97036775556322));
#100027=CARTESIAN_POINT('Ctrl Pts',(-11.078049737449,19.1597144709575,3.9742592885987));
#100028=CARTESIAN_POINT('Ctrl Pts',(-11.0716717933705,19.1607673729671,
3.98861641891627));
#100029=CARTESIAN_POINT('Ctrl Pts',(-11.0668656263564,19.1615268752339,
3.99902324307275));
#100030=CARTESIAN_POINT('Ctrl Pts',(-11.0312913900265,19.1669245297216,
4.07318820303578));
#100031=CARTESIAN_POINT('Ctrl Pts',(-10.9949777285771,19.1712856660638,
4.13413615058105));
#100032=CARTESIAN_POINT('Ctrl Pts',(-10.9062645758237,19.1806261689906,
4.25645646733281));
#100033=CARTESIAN_POINT('Ctrl Pts',(-10.8526083893289,19.1855944090477,
4.31645497100776));
#100034=CARTESIAN_POINT('Ctrl Pts',(-10.7821386835598,19.1918123534832,
4.3806707465737));
#100035=CARTESIAN_POINT('Ctrl Pts',(-10.7708136174569,19.1928027293023,
4.39059992010049));
#100036=CARTESIAN_POINT('Ctrl Pts',(-10.754216055974,19.1942434285033,4.4045979567811));
#100037=CARTESIAN_POINT('Ctrl Pts',(-10.7490942725793,19.1946865722762,
4.40884382059606));
#100038=CARTESIAN_POINT('Ctrl Pts',(-10.740020354648,19.1954693100076,4.41623711978447));
#100039=CARTESIAN_POINT('Ctrl Pts',(-10.7360833913643,19.195808156552,4.41940297180304));
#100040=CARTESIAN_POINT('Ctrl Pts',(-10.727909268596,19.1965101862807,4.42588991865983));
#100041=CARTESIAN_POINT('Ctrl Pts',(-10.7236694693532,19.196873498213,4.42920748073001));
#100042=CARTESIAN_POINT('Ctrl Pts',(-10.7127254324685,19.1978093005164,
4.4376506481061));
#100043=CARTESIAN_POINT('Ctrl Pts',(-10.7059886753529,19.1983834432181,
4.4427334001706));
#100044=CARTESIAN_POINT('Ctrl Pts',(-10.6770794744032,19.2008396919502,
4.46406117779448));
#100045=CARTESIAN_POINT('Ctrl Pts',(-10.6543982050937,19.2027484090674,
4.47959856084791));
#100046=CARTESIAN_POINT('Ctrl Pts',(-10.5471510794701,19.2116978575062,
4.54767869105495));
#100047=CARTESIAN_POINT('Ctrl Pts',(-10.4566890148157,19.2190828585621,
4.59015326009959));
#100048=CARTESIAN_POINT('Ctrl Pts',(-10.340971990513,19.2279465635238,4.62752867021513));
#100049=CARTESIAN_POINT('Ctrl Pts',(-10.3197684044419,19.2295459706809,
4.63372442043447));
#100050=CARTESIAN_POINT('Ctrl Pts',(-10.2771986240006,19.2326938566424,
4.64487397446374));
#100051=CARTESIAN_POINT('Ctrl Pts',(-10.2558424465414,19.2342420526977,
4.64983489589336));
#100052=CARTESIAN_POINT('Ctrl Pts',(-10.2289477544548,19.2361432800371,
4.65529583793001));
#100053=CARTESIAN_POINT('Ctrl Pts',(-10.2235290632786,19.2365238901828,
4.65635647976024));
#100054=CARTESIAN_POINT('Ctrl Pts',(-10.2149506867973,19.2371223656953,
4.65797303707202));
#100055=CARTESIAN_POINT('Ctrl Pts',(-10.2117959303673,19.2373415910549,
4.65855420108203));
#100056=CARTESIAN_POINT('Ctrl Pts',(-10.2061562914261,19.2377318951477,
4.6595693202563));
#100057=CARTESIAN_POINT('Ctrl Pts',(-10.203672401958,19.2379032416432,4.66000818007255));
#100058=CARTESIAN_POINT('Ctrl Pts',(-10.1977088844212,19.2383133090819,
4.66104208397579));
#100059=CARTESIAN_POINT('Ctrl Pts',(-10.1942279711302,19.238551598389,4.66162946751131));
#100060=CARTESIAN_POINT('Ctrl Pts',(-10.1836263616881,19.2392742405756,
4.66336943969752));
#100061=CARTESIAN_POINT('Ctrl Pts',(-10.1764975080296,19.2397559163239,
4.6644722968057));
#100062=CARTESIAN_POINT('Ctrl Pts',(-10.1000787943225,19.24487822132,4.67557660500358));
#100063=CARTESIAN_POINT('Ctrl Pts',(-10.0300279354252,19.2492174251588,
4.67944794843017));
#100064=CARTESIAN_POINT('Ctrl Pts',(-9.87253636059848,19.2589635532404,
4.67410120691841));
#100065=CARTESIAN_POINT('Ctrl Pts',(-9.78564878657044,19.2643509490355,
4.6613836431938));
#100066=CARTESIAN_POINT('Ctrl Pts',(-9.68666921420075,19.2710279244627,
4.63540199575862));
#100067=CARTESIAN_POINT('Ctrl Pts',(-9.67243424658421,19.2720009560114,
4.63137726623645));
#100068=CARTESIAN_POINT('Ctrl Pts',(-9.65195794905035,19.2734209275381,
4.62516906585841));
#100069=CARTESIAN_POINT('Ctrl Pts',(-9.64565288833514,19.2738609775836,
4.62319936674547));
#100070=CARTESIAN_POINT('Ctrl Pts',(-9.63456289316034,19.2746401117231,
4.61963218417606));
#100071=CARTESIAN_POINT('Ctrl Pts',(-9.62977098717978,19.2749784700321,
4.61805678908035));
#100072=CARTESIAN_POINT('Ctrl Pts',(-9.61986804955209,19.2756813199378,
4.61473043841932));
#100073=CARTESIAN_POINT('Ctrl Pts',(-9.61475865923405,19.2760459514584,
4.6129750032105));
#100074=CARTESIAN_POINT('Ctrl Pts',(-9.60161688723282,19.2769890731157,
4.60835854370644));
#100075=CARTESIAN_POINT('Ctrl Pts',(-9.59360329032413,19.2775692657825,
4.60544537343507));
#100076=CARTESIAN_POINT('Ctrl Pts',(-9.55911100241798,19.2800891552865,
4.59248070731796));
#100077=CARTESIAN_POINT('Ctrl Pts',(-9.53297002011803,19.282057214737,4.58156366614755));
#100078=CARTESIAN_POINT('Ctrl Pts',(-9.41739377314355,19.291031086042,4.5283250180462));
#100079=CARTESIAN_POINT('Ctrl Pts',(-9.33311981038472,19.2983720385527,
4.47578042561953));
#100080=CARTESIAN_POINT('Ctrl Pts',(-9.22399339261876,19.3086266919065,
4.38693711660613));
#100081=CARTESIAN_POINT('Ctrl Pts',(-9.19298993233208,19.3116360642708,
4.35882434508971));
#100082=CARTESIAN_POINT('Ctrl Pts',(-9.15933723269075,19.3149582852632,
4.32487386684008));
#100083=CARTESIAN_POINT('Ctrl Pts',(-9.15516192169255,19.3153715039879,
4.32059698373091));
#100084=CARTESIAN_POINT('Ctrl Pts',(-9.14852579976048,19.3160296539579,
4.31369508497761));
#100085=CARTESIAN_POINT('Ctrl Pts',(-9.14604421024184,19.3162760874644,
4.3110903248079));
#100086=CARTESIAN_POINT('Ctrl Pts',(-9.14165218840433,19.3167127365933,
4.30643780861967));
#100087=CARTESIAN_POINT('Ctrl Pts',(-9.13973707864857,19.3169033025763,
4.30439456214863));
#100088=CARTESIAN_POINT('Ctrl Pts',(-9.13563206034962,19.3173121280907,
4.29998345552619));
#100089=CARTESIAN_POINT('Ctrl Pts',(-9.13344458219608,19.3175302068904,
4.29761342310487));
#100090=CARTESIAN_POINT('Ctrl Pts',(-9.12738613400547,19.3181349269486,
4.29099502872505));
#100091=CARTESIAN_POINT('Ctrl Pts',(-9.12353641936397,19.3185200185641,
4.28672720161164));
#100092=CARTESIAN_POINT('Ctrl Pts',(-9.10109168705945,19.3207713531377,
4.26147553435145));
#100093=CARTESIAN_POINT('Ctrl Pts',(-9.08321782752752,19.3225894053749,
4.23985936974546));
#100094=CARTESIAN_POINT('Ctrl Pts',(-9.02377539867595,19.3288093216091,
4.16250486355738));
#100095=CARTESIAN_POINT('Ctrl Pts',(-8.98637983303266,19.3330498770526,
4.10374059260751));
#100096=CARTESIAN_POINT('Ctrl Pts',(-8.92289268753821,19.3416065426909,
3.98126634574884));
#100097=CARTESIAN_POINT('Ctrl Pts',(-8.89675967625481,19.3459060019001,
3.91789513571142));
#100098=CARTESIAN_POINT('Ctrl Pts',(-8.87331662572205,19.3510497775196,
3.84318706946664));
#100099=CARTESIAN_POINT('Ctrl Pts',(-8.87047577616379,19.3517028384361,
3.83371815737684));
#100100=CARTESIAN_POINT('Ctrl Pts',(-8.86602549038059,19.3527770910535,
3.81817656162913));
#100101=CARTESIAN_POINT('Ctrl Pts',(-8.86434480985467,19.3531959862849,
3.81212465354827));
#100102=CARTESIAN_POINT('Ctrl Pts',(-8.86141659599306,19.3539503062828,
3.8012437021625));
#100103=CARTESIAN_POINT('Ctrl Pts',(-8.86015116890268,19.3542851476251,
3.79641959602214));
#100104=CARTESIAN_POINT('Ctrl Pts',(-8.8575241666918,19.3549996511248,3.78613922601779));
#100105=CARTESIAN_POINT('Ctrl Pts',(-8.8561709585977,19.3553795717486,3.78068097282013));
#100106=CARTESIAN_POINT('Ctrl Pts',(-8.85262845543941,19.356407177706,3.76594086858718));
#100107=CARTESIAN_POINT('Ctrl Pts',(-8.85051276119721,19.3570571846646,
3.75664193998796));
#100108=CARTESIAN_POINT('Ctrl Pts',(-8.84003089837772,19.3604783991102,
3.70783947056981));
#100109=CARTESIAN_POINT('Ctrl Pts',(-8.83358840206345,19.3633094933184,
3.66795498321577));
#100110=CARTESIAN_POINT('Ctrl Pts',(-8.81852289871263,19.373227556442,3.52996194804202));
#100111=CARTESIAN_POINT('Ctrl Pts',(-8.82015097849112,19.3805780282818,
3.43116287313408));
#100112=CARTESIAN_POINT('Ctrl Pts',(-8.83816885235124,19.3897844807032,
3.30481785220476));
#100113=CARTESIAN_POINT('Ctrl Pts',(-8.84336530088836,19.3918622349192,
3.27607102820146));
#100114=CARTESIAN_POINT('Ctrl Pts',(-8.85080117627748,19.3942692306733,
3.2421876559134));
#100115=CARTESIAN_POINT('Ctrl Pts',(-8.85201421312623,19.3946479314441,
3.23683887587118));
#100116=CARTESIAN_POINT('Ctrl Pts',(-8.85405992311323,19.395264236073,3.22810190695853));
#100117=CARTESIAN_POINT('Ctrl Pts',(-8.85487034871994,19.3955030285681,
3.22470867182289));
#100118=CARTESIAN_POINT('Ctrl Pts',(-8.85635549481777,19.3959310993064,
3.21861044826831));
#100119=CARTESIAN_POINT('Ctrl Pts',(-8.85702474919731,19.3961206771046,
3.21590422284104));
#100120=CARTESIAN_POINT('Ctrl Pts',(-8.85851961687754,19.3965369076787,
3.20995030462312));
#100121=CARTESIAN_POINT('Ctrl Pts',(-8.8593494833124,19.3967633158958,3.20670374989398));
#100122=CARTESIAN_POINT('Ctrl Pts',(-8.86178819406716,19.3974155310039,
3.1973300872187));
#100123=CARTESIAN_POINT('Ctrl Pts',(-8.86343266070185,19.3978393693575,
3.19121224289695));
#100124=CARTESIAN_POINT('Ctrl Pts',(-8.87650110290369,19.4010902412087,
3.14411349228073));
#100125=CARTESIAN_POINT('Ctrl Pts',(-8.89009007724601,19.4038051561101,
3.10376038917526));
#100126=CARTESIAN_POINT('Ctrl Pts',(-8.93993899352409,19.4122573436673,
2.97859678174298));
#100127=CARTESIAN_POINT('Ctrl Pts',(-8.98397580591143,19.4178218437441,
2.89726785762434));
#100128=CARTESIAN_POINT('Ctrl Pts',(-9.05616615819369,19.4258006561304,
2.79475139607661));
#100129=CARTESIAN_POINT('Ctrl Pts',(-9.07642483797551,19.4279459191167,
2.76842190042464));
#100130=CARTESIAN_POINT('Ctrl Pts',(-9.10377315968961,19.4307504735862,
2.73582736488738));
#100131=CARTESIAN_POINT('Ctrl Pts',(-9.10986371034737,19.4313696457649,
2.72874145510258));
#100132=CARTESIAN_POINT('Ctrl Pts',(-9.11972598759326,19.432364172045,2.71753985613129));
#100133=CARTESIAN_POINT('Ctrl Pts',(-9.12344386744931,19.4327373060001,
2.71337711810091));
#100134=CARTESIAN_POINT('Ctrl Pts',(-9.13020912907082,19.433413179582,2.70590988668082));
#100135=CARTESIAN_POINT('Ctrl Pts',(-9.13324612572637,19.4337154805079,
2.70259609501179));
#100136=CARTESIAN_POINT('Ctrl Pts',(-9.14045126032815,19.4344301393493,
2.6948240717936));
#100137=CARTESIAN_POINT('Ctrl Pts',(-9.14463519707527,19.4348431627808,
2.69038072977618));
#100138=CARTESIAN_POINT('Ctrl Pts',(-9.1570069699288,19.4360588763551,2.67744484957506));
#100139=CARTESIAN_POINT('Ctrl Pts',(-9.16528788553141,19.436865553463,2.66904278535773));
#100140=CARTESIAN_POINT('Ctrl Pts',(-9.23184320565395,19.4432961410119,
2.60351260582741));
#100141=CARTESIAN_POINT('Ctrl Pts',(-9.29577479141901,19.4491820735364,
2.55246819079272));
#100142=CARTESIAN_POINT('Ctrl Pts',(-9.42952397745353,19.4608305441315,
2.4667402010071));
#100143=CARTESIAN_POINT('Ctrl Pts',(-9.49854672400978,19.4665502601415,
2.43153600752212));
#100144=CARTESIAN_POINT('Ctrl Pts',(-9.57913666983085,19.4726083671997,
2.39997516681611));
#100145=CARTESIAN_POINT('Ctrl Pts',(-9.58778703949948,19.4732508394052,
2.39670445265449));
#100146=CARTESIAN_POINT('Ctrl Pts',(-9.5998811357328,19.474137421021,2.39229376684017));
#100147=CARTESIAN_POINT('Ctrl Pts',(-9.60329267978202,19.4743862293026,
2.39106740173889));
#100148=CARTESIAN_POINT('Ctrl Pts',(-9.60918399340608,19.4748136188465,
2.38898028778154));
#100149=CARTESIAN_POINT('Ctrl Pts',(-9.61166105268762,19.4749926293477,
2.38811204957746));
#100150=CARTESIAN_POINT('Ctrl Pts',(-9.61687680755017,19.4753680790314,
2.38630342265884));
#100151=CARTESIAN_POINT('Ctrl Pts',(-9.61961610212526,19.4755644062718,
2.38536484107397));
#100152=CARTESIAN_POINT('Ctrl Pts',(-9.62637404986326,19.4760467066566,
2.38307713733145));
#100153=CARTESIAN_POINT('Ctrl Pts',(-9.63039662931669,19.4763320121143,
2.38173957347419));
#100154=CARTESIAN_POINT('Ctrl Pts',(-9.64526308204525,19.4773801894911,
2.37688525269519));
#100155=CARTESIAN_POINT('Ctrl Pts',(-9.65615104800831,19.4781356484528,
2.37350413285198));
#100156=CARTESIAN_POINT('Ctrl Pts',(-9.71437430520808,19.4821192942717,
2.35634650847987));
#100157=CARTESIAN_POINT('Ctrl Pts',(-9.76247520181581,19.4852151258987,
2.34539866670362));
#100158=CARTESIAN_POINT('Ctrl Pts',(-9.81110408825476,19.4882767425658,
2.33749692601442));
#100159=CARTESIAN_POINT('Origin',(-10.,12.3756328852638,3.5));
#100160=CARTESIAN_POINT('',(-9.8111040599147,20.0861209582704,2.33749693061941));
#100161=CARTESIAN_POINT('',(-9.81110406371628,19.9867190062194,2.33749693000169));
#100162=CARTESIAN_POINT('',(-9.81110406371068,12.3756328852638,2.3374969300026));
#100163=CARTESIAN_POINT('Ctrl Pts',(-9.81110405611873,20.0861209582704,
2.33749693123622));
#100164=CARTESIAN_POINT('Ctrl Pts',(-9.80339163817242,20.0856358825423,
2.33875012747004));
#100165=CARTESIAN_POINT('Ctrl Pts',(-9.79569045090659,20.0851515754612,
2.34008027521026));
#100166=CARTESIAN_POINT('Ctrl Pts',(-9.72214789657499,20.0805229996855,
2.35353796094226));
#100167=CARTESIAN_POINT('Ctrl Pts',(-9.65744542390395,20.0764141432507,
2.37118082151058));
#100168=CARTESIAN_POINT('Ctrl Pts',(-9.56199150098702,20.0699509916069,
2.40617670742513));
#100169=CARTESIAN_POINT('Ctrl Pts',(-9.52993660473754,20.0677089904062,
2.41956449393576));
#100170=CARTESIAN_POINT('Ctrl Pts',(-9.49027198717962,20.0648180321093,
2.43822999119953));
#100171=CARTESIAN_POINT('Ctrl Pts',(-9.48206748339353,20.0642135890124,
2.4422079130821));
#100172=CARTESIAN_POINT('Ctrl Pts',(-9.46895979841029,20.0632370802572,
2.44875217871409));
#100173=CARTESIAN_POINT('Ctrl Pts',(-9.4640269681909,20.0628670920651,2.45125857101962));
#100174=CARTESIAN_POINT('Ctrl Pts',(-9.45466459853784,20.0621599987673,
2.45609893704234));
#100175=CARTESIAN_POINT('Ctrl Pts',(-9.45023191161884,20.0618231205514,
2.45842658588255));
#100176=CARTESIAN_POINT('Ctrl Pts',(-9.44012898191428,20.0610504224013,
2.46381419629831));
#100177=CARTESIAN_POINT('Ctrl Pts',(-9.43446878019102,20.0606139623696,
2.46689254516296));
#100178=CARTESIAN_POINT('Ctrl Pts',(-9.41701465362454,20.0592568364947,
2.4765715409358));
#100179=CARTESIAN_POINT('Ctrl Pts',(-9.4053092366131,20.0583306526201,2.48332866944659));
#100180=CARTESIAN_POINT('Ctrl Pts',(-9.30670098552378,20.0503873536954,
2.54253739057376));
#100181=CARTESIAN_POINT('Ctrl Pts',(-9.22681507711688,20.0429526575367,
2.60581058093292));
#100182=CARTESIAN_POINT('Ctrl Pts',(-9.11558580553999,20.0312540924891,
2.72008252877829));
#100183=CARTESIAN_POINT('Ctrl Pts',(-9.0782476741731,20.0270245717561,2.76458584413573));
#100184=CARTESIAN_POINT('Ctrl Pts',(-9.04011457419426,20.0224825945526,
2.81752856753465));
#100185=CARTESIAN_POINT('Ctrl Pts',(-9.03594489588116,20.0219826310204,
2.82343141545693));
#100186=CARTESIAN_POINT('Ctrl Pts',(-9.02981771699475,20.0212433889728,
2.8322770895193));
#100187=CARTESIAN_POINT('Ctrl Pts',(-9.02781879535383,20.0210014772488,
2.83519081414577));
#100188=CARTESIAN_POINT('Ctrl Pts',(-9.0244148110659,20.020588302457,2.84020081118961));
#100189=CARTESIAN_POINT('Ctrl Pts',(-9.02300334296982,20.0204166156738,
2.84229264637065));
#100190=CARTESIAN_POINT('Ctrl Pts',(-9.01981306202943,20.0200277399637,
2.84705366434144));
#100191=CARTESIAN_POINT('Ctrl Pts',(-9.01803842286806,20.0198108293916,
2.84972558694336));
#100192=CARTESIAN_POINT('Ctrl Pts',(-9.01324098203139,20.0192227274708,
2.85701310807822));
#100193=CARTESIAN_POINT('Ctrl Pts',(-9.01023961498612,20.0188529172726,
2.8616428225913));
#100194=CARTESIAN_POINT('Ctrl Pts',(-8.99551070237757,20.0170277609961,
2.88471631630304));
#100195=CARTESIAN_POINT('Ctrl Pts',(-8.98426476525646,20.0156010937578,
2.90346430017379));
#100196=CARTESIAN_POINT('Ctrl Pts',(-8.9627209616243,20.012775788483,2.94175749949464));
#100197=CARTESIAN_POINT('Ctrl Pts',(-8.9524382138839,20.011378143836,2.96130073828413));
#100198=CARTESIAN_POINT('Ctrl Pts',(-8.89887056809101,20.0037506855643,
3.07045270881068));
#100199=CARTESIAN_POINT('Ctrl Pts',(-8.86652933171974,19.9977576214643,
3.16497516888545));
#100200=CARTESIAN_POINT('Ctrl Pts',(-8.84089637897507,19.9896130520816,
3.28944367417763));
#100201=CARTESIAN_POINT('Ctrl Pts',(-8.83628560309965,19.9878221582552,
3.31663211255273));
#100202=CARTESIAN_POINT('Ctrl Pts',(-8.83151367051865,19.9854433065172,
3.35233091623306));
#100203=CARTESIAN_POINT('Ctrl Pts',(-8.83048432431036,19.9848824998316,
3.36071777350632));
#100204=CARTESIAN_POINT('Ctrl Pts',(-8.82894666077115,19.9839595411634,
3.37446849169533));
#100205=CARTESIAN_POINT('Ctrl Pts',(-8.82838473611101,19.9835990678135,
3.37982614811689));
#100206=CARTESIAN_POINT('Ctrl Pts',(-8.8273670033187,19.9828982380175,3.39021634647297));
#100207=CARTESIAN_POINT('Ctrl Pts',(-8.82690678755419,19.9825580270623,
3.3952483459377));
#100208=CARTESIAN_POINT('Ctrl Pts',(-8.82591586062558,19.9817676623063,
3.40691009438077));
#100209=CARTESIAN_POINT('Ctrl Pts',(-8.82540890318171,19.981316779845,3.4135416344194));
#100210=CARTESIAN_POINT('Ctrl Pts',(-8.8239386711868,19.979840399331,3.43518431935718));
#100211=CARTESIAN_POINT('Ctrl Pts',(-8.82320683328511,19.9788077895267,
3.45020915844231));
#100212=CARTESIAN_POINT('Ctrl Pts',(-8.82036756792613,19.9721463985116,
3.54637734953955));
#100213=CARTESIAN_POINT('Ctrl Pts',(-8.82636639331177,19.9662659210613,
3.62752706531917));
#100214=CARTESIAN_POINT('Ctrl Pts',(-8.8502875177255,19.9562970216206,3.76124339507507));
#100215=CARTESIAN_POINT('Ctrl Pts',(-8.86365935354226,19.9522671238449,
3.81435236792767));
#100216=CARTESIAN_POINT('Ctrl Pts',(-8.88569702970261,19.9471871597312,
3.88168657511586));
#100217=CARTESIAN_POINT('Ctrl Pts',(-8.89103452229348,19.9460396458423,
3.89692741852733));
#100218=CARTESIAN_POINT('Ctrl Pts',(-8.90045512658755,19.9441494851345,
3.92215200553805));
#100219=CARTESIAN_POINT('Ctrl Pts',(-8.90436486273141,19.9433991652139,
3.93219776853356));
#100220=CARTESIAN_POINT('Ctrl Pts',(-8.90996955252484,19.9423705191155,
3.94603351089719));
#100221=CARTESIAN_POINT('Ctrl Pts',(-8.91154729798638,19.9420858010394,
3.94986996572215));
#100222=CARTESIAN_POINT('Ctrl Pts',(-8.91425410075539,19.9416055418476,
3.95635423672192));
#100223=CARTESIAN_POINT('Ctrl Pts',(-8.91537264576085,19.9414093856008,
3.95900637273709));
#100224=CARTESIAN_POINT('Ctrl Pts',(-8.91753771859271,19.9410341190966,
3.96408778039762));
#100225=CARTESIAN_POINT('Ctrl Pts',(-8.91858271743203,19.9408549157014,
3.96651765229217));
#100226=CARTESIAN_POINT('Ctrl Pts',(-8.9211092898625,19.9404261725905,3.97233842844829));
#100227=CARTESIAN_POINT('Ctrl Pts',(-8.92259868732268,19.9401770986818,
3.97572593767233));
#100228=CARTESIAN_POINT('Ctrl Pts',(-8.92807058311616,19.9392750143365,
3.98801379309746));
#100229=CARTESIAN_POINT('Ctrl Pts',(-8.93214773819185,19.9386274080813,
3.99687191430081));
#100230=CARTESIAN_POINT('Ctrl Pts',(-8.96260541857004,19.9339560021355,
4.06093784989113));
#100231=CARTESIAN_POINT('Ctrl Pts',(-8.99314619730812,19.9301461866744,
4.11407344618222));
#100232=CARTESIAN_POINT('Ctrl Pts',(-9.06546062635027,19.9222125204287,
4.21987025281009));
#100233=CARTESIAN_POINT('Ctrl Pts',(-9.107880244488,19.918103653838,4.2718152243657));
#100234=CARTESIAN_POINT('Ctrl Pts',(-9.17865440184662,19.9116404882417,
4.34480308501752));
#100235=CARTESIAN_POINT('Ctrl Pts',(-9.20391585110715,19.9093984839035,
4.36864866872874));
#100236=CARTESIAN_POINT('Ctrl Pts',(-9.23709250909748,19.9065075220645,
4.3973017101519));
#100237=CARTESIAN_POINT('Ctrl Pts',(-9.24406191112564,19.9059030787001,
4.4031809324649));
#100238=CARTESIAN_POINT('Ctrl Pts',(-9.25536910357985,19.9049265696161,
4.4124968523613));
#100239=CARTESIAN_POINT('Ctrl Pts',(-9.25966417016777,19.9045565813654,
4.41598500793572));
#100240=CARTESIAN_POINT('Ctrl Pts',(-9.2678921952375,19.9038494880237,4.4225715644522));
#100241=CARTESIAN_POINT('Ctrl Pts',(-9.27182065428259,19.9035126098231,
4.42567541204627));
#100242=CARTESIAN_POINT('Ctrl Pts',(-9.28084969261911,19.9027399118046,
4.43271614763406));
#100243=CARTESIAN_POINT('Ctrl Pts',(-9.28596299022662,19.9023034518902,
4.43663638754346));
#100244=CARTESIAN_POINT('Ctrl Pts',(-9.30190097252241,19.9009463267472,
4.44864928846435));
#100245=CARTESIAN_POINT('Ctrl Pts',(-9.31283265216253,19.9000201434959,
4.45659747765247));
#100246=CARTESIAN_POINT('Ctrl Pts',(-9.4070112149981,19.892076840469,4.52262529160026));
#100247=CARTESIAN_POINT('Ctrl Pts',(-9.49729318952429,19.8846421389151,
4.56989509722444));
#100248=CARTESIAN_POINT('Ctrl Pts',(-9.64691103405417,19.8729435727985,
4.62507239997114));
#100249=CARTESIAN_POINT('Ctrl Pts',(-9.70274897772568,19.8687140561529,
4.64109734656486));
#100250=CARTESIAN_POINT('Ctrl Pts',(-9.76662081961227,19.8641720828138,
4.6544182279161));
#100251=CARTESIAN_POINT('Ctrl Pts',(-9.77370889480538,19.8636721193894,
4.65582854656554));
#100252=CARTESIAN_POINT('Ctrl Pts',(-9.78428139263669,19.8629328774693,
4.65783117503079));
#100253=CARTESIAN_POINT('Ctrl Pts',(-9.78775606294384,19.8626909657664,
4.65847315870684));
#100254=CARTESIAN_POINT('Ctrl Pts',(-9.79371714012995,19.8622777909982,
4.65954681326201));
#100255=CARTESIAN_POINT('Ctrl Pts',(-9.79620209652775,19.8621061042175,
4.65998614017859));
#100256=CARTESIAN_POINT('Ctrl Pts',(-9.80184882649107,19.8617172284962,
4.66096574585834));
#100257=CARTESIAN_POINT('Ctrl Pts',(-9.80501140682314,19.8615003179105,
4.66150109761973));
#100258=CARTESIAN_POINT('Ctrl Pts',(-9.81361977753592,19.8609122159163,
4.66292214503367));
#100259=CARTESIAN_POINT('Ctrl Pts',(-9.81906975252084,19.860542405659,4.6637825188793));
#100260=CARTESIAN_POINT('Ctrl Pts',(-9.84613806928921,19.8587172486159,
4.66786097940075));
#100261=CARTESIAN_POINT('Ctrl Pts',(-9.86783858980784,19.8572905806989,
4.67051538665244));
#100262=CARTESIAN_POINT('Ctrl Pts',(-9.91158265192551,19.8544652749122,
4.67463392820757));
#100263=CARTESIAN_POINT('Ctrl Pts',(-9.93361824205453,19.8530676304076,
4.67608505322905));
#100264=CARTESIAN_POINT('Ctrl Pts',(-10.0551201609284,19.8454401712868,
4.68066026965506));
#100265=CARTESIAN_POINT('Ctrl Pts',(-10.1546276556612,19.8394471061895,
4.67178824226758));
#100266=CARTESIAN_POINT('Ctrl Pts',(-10.2787689453709,19.8313025369412,
4.64461480179881));
#100267=CARTESIAN_POINT('Ctrl Pts',(-10.3054841319522,19.8295116445137,
4.63777608676271));
#100268=CARTESIAN_POINT('Ctrl Pts',(-10.3400404207402,19.8271327943743,
4.627625368954));
#100269=CARTESIAN_POINT('Ctrl Pts',(-10.3481215749565,19.8265719878419,
4.62515679943333));
#100270=CARTESIAN_POINT('Ctrl Pts',(-10.3613101030482,19.8256490293611,
4.62097238695968));
#100271=CARTESIAN_POINT('Ctrl Pts',(-10.3664335981194,19.8252885560443,
4.61930804491788));
#100272=CARTESIAN_POINT('Ctrl Pts',(-10.3763404105,19.8245877262665,4.61601455676634));
#100273=CARTESIAN_POINT('Ctrl Pts',(-10.381125023763,19.8242475152962,4.61438965823406));
#100274=CARTESIAN_POINT('Ctrl Pts',(-10.392182709015,19.8234571504368,4.61055482513273));
#100275=CARTESIAN_POINT('Ctrl Pts',(-10.3984477621367,19.8230062678867,
4.60832245965198));
#100276=CARTESIAN_POINT('Ctrl Pts',(-10.4188194824617,19.8215298867793,
4.60086854933664));
#100277=CARTESIAN_POINT('Ctrl Pts',(-10.4328445883031,19.8204972764622,
4.59542998303295));
#100278=CARTESIAN_POINT('Ctrl Pts',(-10.5218636455835,19.8138359047785,
4.55893428599914));
#100279=CARTESIAN_POINT('Ctrl Pts',(-10.593568449894,19.8079554491475,4.52046824730961));
#100280=CARTESIAN_POINT('Ctrl Pts',(-10.7060166537096,19.7979865552552,
4.44426024582946));
#100281=CARTESIAN_POINT('Ctrl Pts',(-10.7491051818362,19.7939566409911,
4.41045534012406));
#100282=CARTESIAN_POINT('Ctrl Pts',(-10.8016683311451,19.7888766584325,
4.36295054273845));
#100283=CARTESIAN_POINT('Ctrl Pts',(-10.8134237831107,19.7877291419767,
4.35187883911399));
#100284=CARTESIAN_POINT('Ctrl Pts',(-10.8326413335058,19.785838977503,4.33301839988183));
#100285=CARTESIAN_POINT('Ctrl Pts',(-10.840230570131,19.7850886563464,4.32536286234415));
#100286=CARTESIAN_POINT('Ctrl Pts',(-10.8505936130219,19.7840600088504,
4.31461817729191));
#100287=CARTESIAN_POINT('Ctrl Pts',(-10.8534575246255,19.7837752905904,
4.31161722767669));
#100288=CARTESIAN_POINT('Ctrl Pts',(-10.8582817126267,19.7832950311799,
4.306508430752));
#100289=CARTESIAN_POINT('Ctrl Pts',(-10.8602502089011,19.783098874897,4.30440843224425));
#100290=CARTESIAN_POINT('Ctrl Pts',(-10.8640128511282,19.7827236083958,
4.30036482410591));
#100291=CARTESIAN_POINT('Ctrl Pts',(-10.8658081670061,19.7825444050394,
4.29842236747187));
#100292=CARTESIAN_POINT('Ctrl Pts',(-10.8700993999265,19.7821156621156,
4.29374793835391));
#100293=CARTESIAN_POINT('Ctrl Pts',(-10.8725890348611,19.7818665883544,
4.29101019750494));
#100294=CARTESIAN_POINT('Ctrl Pts',(-10.8815917823888,19.7809645053208,
4.28101604715774));
#100295=CARTESIAN_POINT('Ctrl Pts',(-10.8880278403469,19.7803169002087,
4.27369031705033));
#100296=CARTESIAN_POINT('Ctrl Pts',(-10.9341832921174,19.7756453819506,
4.2198198220698));
#100297=CARTESIAN_POINT('Ctrl Pts',(-10.9703181327586,19.7718354654465,
4.17031612629714));
#100298=CARTESIAN_POINT('Ctrl Pts',(-11.0375864444072,19.7639017751128,
4.06124078745673));
#100299=CARTESIAN_POINT('Ctrl Pts',(-11.0678033570306,19.7597929825771,
4.00137034093373));
#100300=CARTESIAN_POINT('Ctrl Pts',(-11.1057209842605,19.7533299187207,
3.90704044478896));
#100301=CARTESIAN_POINT('Ctrl Pts',(-11.1172395101833,19.7510879372613,
3.87426772952716));
#100302=CARTESIAN_POINT('Ctrl Pts',(-11.1299331170329,19.7481970012508,
3.83230911694384));
#100303=CARTESIAN_POINT('Ctrl Pts',(-11.1324718450559,19.7475925598375,
3.82355171238884));
#100304=CARTESIAN_POINT('Ctrl Pts',(-11.1363873500754,19.7466160531505,
3.80943410928476));
#100305=CARTESIAN_POINT('Ctrl Pts',(-11.1378285078647,19.7462460653273,
3.80409202935022));
#100306=CARTESIAN_POINT('Ctrl Pts',(-11.1405019094315,19.7455389723053,
3.79389713154148));
#100307=CARTESIAN_POINT('Ctrl Pts',(-11.1417409584071,19.7452020939936,
3.78904621067819));
#100308=CARTESIAN_POINT('Ctrl Pts',(-11.1445037391334,19.7444293950151,
3.77793482677214));
#100309=CARTESIAN_POINT('Ctrl Pts',(-11.146007090309,19.743992934246,3.77166951046781));
#100310=CARTESIAN_POINT('Ctrl Pts',(-11.150504452496,19.7426358037659,3.752224565061));
#100311=CARTESIAN_POINT('Ctrl Pts',(-11.1533229723499,19.7417096159696,
3.73900590243519));
#100312=CARTESIAN_POINT('Ctrl Pts',(-11.1753687704391,19.7337663428555,
3.62612032282185));
#100313=CARTESIAN_POINT('Ctrl Pts',(-11.1818600735266,19.7263316806437,
3.52441964960938));
#100314=CARTESIAN_POINT('Ctrl Pts',(-11.1714577973445,19.7146331223228,
3.36529143487493));
#100315=CARTESIAN_POINT('Ctrl Pts',(-11.1634024523517,19.7104035758714,
3.30776029575101));
#100316=CARTESIAN_POINT('Ctrl Pts',(-11.1496108706964,19.7058615743522,
3.2439880219171));
#100317=CARTESIAN_POINT('Ctrl Pts',(-11.1480183003497,19.7053616101421,
3.23693864675703));
#100318=CARTESIAN_POINT('Ctrl Pts',(-11.1455505709564,19.7046223672919,
3.22646492577176));
#100319=CARTESIAN_POINT('Ctrl Pts',(-11.1447247612883,19.7043804554352,
3.22302929907591));
#100320=CARTESIAN_POINT('Ctrl Pts',(-11.1432826915567,19.7039672804955,
3.21714647322273));
#100321=CARTESIAN_POINT('Ctrl Pts',(-11.142674016126,19.7037955936963,3.21469748732636));
#100322=CARTESIAN_POINT('Ctrl Pts',(-11.1412737925602,19.7034067180566,
3.20914010069286));
#100323=CARTESIAN_POINT('Ctrl Pts',(-11.1404774148939,19.7031898075703,
3.2060329655415));
#100324=CARTESIAN_POINT('Ctrl Pts',(-11.1382766898464,19.702601706111,3.19759021177256));
#100325=CARTESIAN_POINT('Ctrl Pts',(-11.1368475060319,19.7022318962848,
3.19226106249127));
#100326=CARTESIAN_POINT('Ctrl Pts',(-11.1295712798933,19.7004067448321,
3.16587205869307));
#100327=CARTESIAN_POINT('Ctrl Pts',(-11.1231758255709,19.6989800818643,
3.14496624079025));
#100328=CARTESIAN_POINT('Ctrl Pts',(-11.1091579590717,19.6961547798103,
3.10332492490595));
#100329=CARTESIAN_POINT('Ctrl Pts',(-11.1015268879771,19.6947571342677,
3.08260198141742));
#100330=CARTESIAN_POINT('Ctrl Pts',(-11.0563197033247,19.6871296813386,
2.96973066768217));
#100331=CARTESIAN_POINT('Ctrl Pts',(-11.0077664858241,19.6811366235139,
2.88242078838443));
#100332=CARTESIAN_POINT('Ctrl Pts',(-10.9324788863872,19.6729920532858,
2.78004284522241));
#100333=CARTESIAN_POINT('Ctrl Pts',(-10.915371472707,19.6712011506575,2.75841382543352));
#100334=CARTESIAN_POINT('Ctrl Pts',(-10.8920507793595,19.6688222888599,
2.73096692673291));
#100335=CARTESIAN_POINT('Ctrl Pts',(-10.8865105460763,19.6682614812111,
2.72458688027257));
#100336=CARTESIAN_POINT('Ctrl Pts',(-10.8773265917048,19.667338521363,2.71423786397006));
#100337=CARTESIAN_POINT('Ctrl Pts',(-10.873723372428,19.6669780478048,2.71023323078161));
#100338=CARTESIAN_POINT('Ctrl Pts',(-10.8666873681529,19.6662772178942,
2.70252046963059));
#100339=CARTESIAN_POINT('Ctrl Pts',(-10.8632579372852,19.6659370070345,
2.6988094310242));
#100340=CARTESIAN_POINT('Ctrl Pts',(-10.8552595350308,19.6651466429285,
2.69026521348653));
#100341=CARTESIAN_POINT('Ctrl Pts',(-10.8506733289371,19.6646957610256,
2.68544847859021));
#100342=CARTESIAN_POINT('Ctrl Pts',(-10.8355824311164,19.6632193842461,
2.66986548017442));
#100343=CARTESIAN_POINT('Ctrl Pts',(-10.8249126090658,19.6621867776678,
2.65926194855719));
#100344=CARTESIAN_POINT('Ctrl Pts',(-10.7553824227598,19.6555252650437,
2.59276176086409));
#100345=CARTESIAN_POINT('Ctrl Pts',(-10.6910894853644,19.6496446503321,
2.54288213270714));
#100346=CARTESIAN_POINT('Ctrl Pts',(-10.5757529820029,19.6396757159865,
2.47111941540398));
#100347=CARTESIAN_POINT('Ctrl Pts',(-10.5273536555237,19.6356459219352,
2.445492793624));
#100348=CARTESIAN_POINT('Ctrl Pts',(-10.4625863905332,19.6305660738538,
2.41677815043175));
#100349=CARTESIAN_POINT('Ctrl Pts',(-10.4476925338677,19.6294185761121,
2.41053811709997));
#100350=CARTESIAN_POINT('Ctrl Pts',(-10.4226493720335,19.6275284390956,
2.40064621236914));
#100351=CARTESIAN_POINT('Ctrl Pts',(-10.412570083668,19.6267781269504,2.39682404448078));
#100352=CARTESIAN_POINT('Ctrl Pts',(-10.3985408956826,19.6257494896444,
2.39172321886773));
#100353=CARTESIAN_POINT('Ctrl Pts',(-10.3946349524379,19.6254647727251,
2.39032638818606));
#100354=CARTESIAN_POINT('Ctrl Pts',(-10.3880063499558,19.6249845149093,
2.38799531499366));
#100355=CARTESIAN_POINT('Ctrl Pts',(-10.3852875206404,19.6247883588897,
2.38705037212041));
#100356=CARTESIAN_POINT('Ctrl Pts',(-10.3800636100059,19.6244130923662,
2.38525621286648));
#100357=CARTESIAN_POINT('Ctrl Pts',(-10.3775591065739,19.6242338887269,
2.38440545895937));
#100358=CARTESIAN_POINT('Ctrl Pts',(-10.3715439610823,19.6238051444385,
2.38238475292391));
#100359=CARTESIAN_POINT('Ctrl Pts',(-10.3680306021654,19.6235560696021,
2.38122288533129));
#100360=CARTESIAN_POINT('Ctrl Pts',(-10.3552398004762,19.6226539770035,
2.37705974186617));
#100361=CARTESIAN_POINT('Ctrl Pts',(-10.3459303419297,19.6220063635559,
2.37415704783111));
#100362=CARTESIAN_POINT('Ctrl Pts',(-10.2779615202111,19.6173356462387,
2.35388705115075));
#100363=CARTESIAN_POINT('Ctrl Pts',(-10.2180562220649,19.6135264504694,
2.34099569901897));
#100364=CARTESIAN_POINT('Ctrl Pts',(-10.091059043873,19.6055929321073,2.32386806920044));
#100365=CARTESIAN_POINT('Ctrl Pts',(-10.0240662146888,19.601483611511,2.32059410611628));
#100366=CARTESIAN_POINT('Ctrl Pts',(-9.92245630101493,19.5950198221902,
2.32429256440615));
#100367=CARTESIAN_POINT('Ctrl Pts',(-9.88782851761291,19.5927776776006,
2.32708986039856));
#100368=CARTESIAN_POINT('Ctrl Pts',(-9.84433009853263,19.589886557428,2.33254760960661));
#100369=CARTESIAN_POINT('Ctrl Pts',(-9.83529664952736,19.5892821021039,
2.33378775488198));
#100370=CARTESIAN_POINT('Ctrl Pts',(-9.82121534134334,19.5883331559789,
2.33588775614029));
#100371=CARTESIAN_POINT('Ctrl Pts',(-9.81615701727274,19.5879909141281,
2.33667587204691));
#100372=CARTESIAN_POINT('Ctrl Pts',(-9.8111040637102,19.5876476368634,2.33749693000268));
#100373=CARTESIAN_POINT('Ctrl Pts',(-9.81110408825476,19.4882767425658,
2.33749692601442));
#100374=CARTESIAN_POINT('Ctrl Pts',(-9.8314222932125,19.4895559525066,2.33419540713123));
#100375=CARTESIAN_POINT('Ctrl Pts',(-9.85183268213264,19.4908290092334,
2.33142565391848));
#100376=CARTESIAN_POINT('Ctrl Pts',(-9.953143009874,19.4971287400356,2.32037699327464));
#100377=CARTESIAN_POINT('Ctrl Pts',(-10.0346566291727,19.5021558995863,
2.31995643091115));
#100378=CARTESIAN_POINT('Ctrl Pts',(-10.130523110947,19.508438767749,2.32940832202197));
#100379=CARTESIAN_POINT('Ctrl Pts',(-10.1454568499483,19.5094275866102,
2.33117005926822));
#100380=CARTESIAN_POINT('Ctrl Pts',(-10.1669389221768,19.5108664263385,
2.33412236378128));
#100381=CARTESIAN_POINT('Ctrl Pts',(-10.173517710403,19.511309293842,2.33508332164917));
#100382=CARTESIAN_POINT('Ctrl Pts',(-10.185079773689,19.5120917091539,2.33687229623325));
#100383=CARTESIAN_POINT('Ctrl Pts',(-10.1900665608985,19.5124305114833,
2.33767677517588));
#100384=CARTESIAN_POINT('Ctrl Pts',(-10.2003587733106,19.5131326113626,
2.33940514189671));
#100385=CARTESIAN_POINT('Ctrl Pts',(-10.2056633365375,19.5134960386458,
2.34033338711694));
#100386=CARTESIAN_POINT('Ctrl Pts',(-10.2192713714732,19.5144324813276,
2.34281095967114));
#100387=CARTESIAN_POINT('Ctrl Pts',(-10.2275647595564,19.5150071534281,
2.34441327320792));
#100388=CARTESIAN_POINT('Ctrl Pts',(-10.2628404000399,19.517468899703,2.3516231187118));
#100389=CARTESIAN_POINT('Ctrl Pts',(-10.2896366409912,19.5193827338782,
2.35808716009673));
#100390=CARTESIAN_POINT('Ctrl Pts',(-10.4120214363975,19.5283342217747,
2.3921947499258));
#100391=CARTESIAN_POINT('Ctrl Pts',(-10.5040827691871,19.5357153482304,
2.43094024442401));
#100392=CARTESIAN_POINT('Ctrl Pts',(-10.6092762727826,19.5445753968953,
2.49185045404422));
#100393=CARTESIAN_POINT('Ctrl Pts',(-10.6280796050488,19.5461752199412,
2.50345637978717));
#100394=CARTESIAN_POINT('Ctrl Pts',(-10.6648377401688,19.5493209306366,
2.52759846295841));
#100395=CARTESIAN_POINT('Ctrl Pts',(-10.6827923963382,19.5508666099407,
2.540120495292));
#100396=CARTESIAN_POINT('Ctrl Pts',(-10.7048255448218,19.5527652057932,
2.55641827768811));
#100397=CARTESIAN_POINT('Ctrl Pts',(-10.7092391114073,19.5531456127061,
2.55973120802322));
#100398=CARTESIAN_POINT('Ctrl Pts',(-10.7161806594788,19.5537438401859,
2.56501838999872));
#100399=CARTESIAN_POINT('Ctrl Pts',(-10.7187240732731,19.5539630189232,
2.56697210375359));
#100400=CARTESIAN_POINT('Ctrl Pts',(-10.723253665748,19.5543532835892,2.57048100583427));
#100401=CARTESIAN_POINT('Ctrl Pts',(-10.7252428187139,19.5545246369375,
2.57203217748863));
#100402=CARTESIAN_POINT('Ctrl Pts',(-10.730004516315,19.5549347767288,2.57577008443367));
#100403=CARTESIAN_POINT('Ctrl Pts',(-10.7327722265213,19.5551731310917,
2.57796290989698));
#100404=CARTESIAN_POINT('Ctrl Pts',(-10.7411675852092,19.5558961691738,
2.58467613587516));
#100405=CARTESIAN_POINT('Ctrl Pts',(-10.7467637051208,19.5563781714753,
2.58923595768833));
#100406=CARTESIAN_POINT('Ctrl Pts',(-10.7967634310582,19.5606888081975,
2.63074736166117));
#100407=CARTESIAN_POINT('Ctrl Pts',(-10.8384406400089,19.5643131194672,
2.67087317444984));
#100408=CARTESIAN_POINT('Ctrl Pts',(-10.9449613168303,19.5742190856175,
2.7897126931168));
#100409=CARTESIAN_POINT('Ctrl Pts',(-11.0027901641923,19.580416609729,2.8740049505218));
#100410=CARTESIAN_POINT('Ctrl Pts',(-11.055184346043,19.5879546091105,2.97668117235625));
#100411=CARTESIAN_POINT('Ctrl Pts',(-11.0611018464588,19.5888422972535,
2.98878630043618));
#100412=CARTESIAN_POINT('Ctrl Pts',(-11.069536221888,19.5901644127521,3.00681775390142));
#100413=CARTESIAN_POINT('Ctrl Pts',(-11.0722144109073,19.5905933237335,
3.01266776007505));
#100414=CARTESIAN_POINT('Ctrl Pts',(-11.0768901488104,19.5913587433108,
3.02310618490724));
#100415=CARTESIAN_POINT('Ctrl Pts',(-11.0789066540735,19.5916945983379,
3.02768597951232));
#100416=CARTESIAN_POINT('Ctrl Pts',(-11.0830919563164,19.5924040328762,
3.03735811749927));
#100417=CARTESIAN_POINT('Ctrl Pts',(-11.0852541584472,19.5927778252737,
3.04245316409917));
#100418=CARTESIAN_POINT('Ctrl Pts',(-11.0908882692075,19.593771555807,3.05599410745709));
#100419=CARTESIAN_POINT('Ctrl Pts',(-11.0942979429618,19.5943935583273,
3.06446532588785));
#100420=CARTESIAN_POINT('Ctrl Pts',(-11.1102686349562,19.5974099379914,
3.10551579292067));
#100421=CARTESIAN_POINT('Ctrl Pts',(-11.1214739789335,19.5998484609782,
3.13860007376705));
#100422=CARTESIAN_POINT('Ctrl Pts',(-11.150020170555,19.6071342427155,3.23708811206023));
#100423=CARTESIAN_POINT('Ctrl Pts',(-11.1632157029336,19.6120915781559,
3.30354038772696));
#100424=CARTESIAN_POINT('Ctrl Pts',(-11.1772481195622,19.6214797840134,
3.43063325644706));
#100425=CARTESIAN_POINT('Ctrl Pts',(-11.179255841517,19.6258929177163,3.49094275425309));
#100426=CARTESIAN_POINT('Ctrl Pts',(-11.1762140773131,19.6308014357199,
3.56091967566458));
#100427=CARTESIAN_POINT('Ctrl Pts',(-11.1756674744183,19.6314816817386,
3.57068781913781));
#100428=CARTESIAN_POINT('Ctrl Pts',(-11.174746215746,19.6324108976232,3.5841433769803));
#100429=CARTESIAN_POINT('Ctrl Pts',(-11.1744758010678,19.6326651722056,
3.58783719564363));
#100430=CARTESIAN_POINT('Ctrl Pts',(-11.1739823803604,19.6330994401997,
3.59416703616647));
#100431=CARTESIAN_POINT('Ctrl Pts',(-11.1737679117601,19.6332798940441,
3.59680366611608));
#100432=CARTESIAN_POINT('Ctrl Pts',(-11.1733017092714,19.6336555106059,
3.60230559372149));
#100433=CARTESIAN_POINT('Ctrl Pts',(-11.1730483602414,19.6338505756278,
3.60517071958557));
#100434=CARTESIAN_POINT('Ctrl Pts',(-11.1724046478051,19.6343250777062,
3.61215860850403));
#100435=CARTESIAN_POINT('Ctrl Pts',(-11.172003026203,19.6346038958872,3.61628034882937));
#100436=CARTESIAN_POINT('Ctrl Pts',(-11.1704818856396,19.6356016333146,
3.63108215866466));
#100437=CARTESIAN_POINT('Ctrl Pts',(-11.1692380126689,19.636314036907,3.6417493097949));
#100438=CARTESIAN_POINT('Ctrl Pts',(-11.1657694303742,19.6380759653208,
3.66832949514771));
#100439=CARTESIAN_POINT('Ctrl Pts',(-11.1633646282005,19.6391172472682,
3.68421720669907));
#100440=CARTESIAN_POINT('Ctrl Pts',(-11.1514269018134,19.6436238430998,
3.75347609685293));
#100441=CARTESIAN_POINT('Ctrl Pts',(-11.1385399351733,19.6469718338608,
3.8062054726742));
#100442=CARTESIAN_POINT('Ctrl Pts',(-11.0972058398895,19.6553809774893,
3.93580689827414));
#100443=CARTESIAN_POINT('Ctrl Pts',(-11.0642968278718,19.6604373674012,
4.01093879214562));
#100444=CARTESIAN_POINT('Ctrl Pts',(-11.0164468784094,19.6667523796445,
4.09511048235554));
#100445=CARTESIAN_POINT('Ctrl Pts',(-11.0087736910705,19.6677403037214,
4.10802660273766));
#100446=CARTESIAN_POINT('Ctrl Pts',(-10.9973526363589,19.6691780747029,
4.12643990362441));
#100447=CARTESIAN_POINT('Ctrl Pts',(-10.9938017561005,19.6696207833053,
4.13205798834511));
#100448=CARTESIAN_POINT('Ctrl Pts',(-10.9874689816378,19.6704030132263,
4.14189219043841));
#100449=CARTESIAN_POINT('Ctrl Pts',(-10.9847071350259,19.6707417901783,
4.14612106505734));
#100450=CARTESIAN_POINT('Ctrl Pts',(-10.9789440787966,19.6714439306755,
4.15482254361596));
#100451=CARTESIAN_POINT('Ctrl Pts',(-10.9759392230919,19.671807424522,4.15929257860341));
#100452=CARTESIAN_POINT('Ctrl Pts',(-10.9681410699812,19.6727442366819,
4.17072300746655));
#100453=CARTESIAN_POINT('Ctrl Pts',(-10.9633033927924,19.6733192142212,
4.17765260353574));
#100454=CARTESIAN_POINT('Ctrl Pts',(-10.9423499057712,19.6757841384546,
4.20698903212234));
#100455=CARTESIAN_POINT('Ctrl Pts',(-10.9255248777781,19.6777009314379,
4.22887606384999));
#100456=CARTESIAN_POINT('Ctrl Pts',(-10.8445964965762,19.6866536043635,
4.32682807504675));
#100457=CARTESIAN_POINT('Ctrl Pts',(-10.771792579397,19.6940324970517,4.39516378195481));
#100458=CARTESIAN_POINT('Ctrl Pts',(-10.6734014737404,19.7028904393982,
4.46649557861566));
#100459=CARTESIAN_POINT('Ctrl Pts',(-10.6551507405275,19.7044905044152,
4.47895906415409));
#100460=CARTESIAN_POINT('Ctrl Pts',(-10.6181642260564,19.7076349538169,
4.50271934070971));
#100461=CARTESIAN_POINT('Ctrl Pts',(-10.5994421264333,19.7091791730579,
4.51402286628597));
#100462=CARTESIAN_POINT('Ctrl Pts',(-10.575614483281,19.7110762420384,4.52751810850758));
#100463=CARTESIAN_POINT('Ctrl Pts',(-10.5707950419972,19.7114565308622,
4.53020314487165));
#100464=CARTESIAN_POINT('Ctrl Pts',(-10.5631445883315,19.7120546142186,
4.53439524273536));
#100465=CARTESIAN_POINT('Ctrl Pts',(-10.5603260577118,19.7122737658631,
4.53592473434785));
#100466=CARTESIAN_POINT('Ctrl Pts',(-10.5552792208171,19.7126640076338,
4.53863680504178));
#100467=CARTESIAN_POINT('Ctrl Pts',(-10.5530533737637,19.7128353649804,
4.53982373112309));
#100468=CARTESIAN_POINT('Ctrl Pts',(-10.5477021112782,19.7132455468889,
4.54265523160871));
#100469=CARTESIAN_POINT('Ctrl Pts',(-10.5445730943463,19.7134839391123,
4.54429290930887));
#100470=CARTESIAN_POINT('Ctrl Pts',(-10.5350238787731,19.7142072076487,
4.54923622530378));
#100471=CARTESIAN_POINT('Ctrl Pts',(-10.5285804560942,19.7146894000474,
4.55249699060958));
#100472=CARTESIAN_POINT('Ctrl Pts',(-10.4702362521768,19.7190068717558,
4.5813517585683));
#100473=CARTESIAN_POINT('Ctrl Pts',(-10.4165373495374,19.7226371190832,
4.60315107234167));
#100474=CARTESIAN_POINT('Ctrl Pts',(-10.2646766985676,19.7325407008603,
4.65211951200985));
#100475=CARTESIAN_POINT('Ctrl Pts',(-10.164285479955,19.7387308092398,4.67065851878124));
#100476=CARTESIAN_POINT('Ctrl Pts',(-10.0492923203816,19.7462610751277,
4.67679536232488));
#100477=CARTESIAN_POINT('Ctrl Pts',(-10.0358100500005,19.7471498640633,
4.67728275004208));
#100478=CARTESIAN_POINT('Ctrl Pts',(-10.0158868276254,19.7484733083011,
4.67766043836936));
#100479=CARTESIAN_POINT('Ctrl Pts',(-10.009450052787,19.7489024308902,4.6777296774391));
#100480=CARTESIAN_POINT('Ctrl Pts',(-9.99800866624269,19.7496680877224,
4.67775894902589));
#100481=CARTESIAN_POINT('Ctrl Pts',(-9.99300422924021,19.7500039669109,
4.67773985467367));
#100482=CARTESIAN_POINT('Ctrl Pts',(-9.98246726647646,19.750713307718,4.67763249001013));
#100483=CARTESIAN_POINT('Ctrl Pts',(-9.97693495101431,19.7510869813182,
4.67753712467072));
#100484=CARTESIAN_POINT('Ctrl Pts',(-9.96228252526964,19.7520800561195,
4.67718125093971));
#100485=CARTESIAN_POINT('Ctrl Pts',(-9.95316457014405,19.752701516847,4.67685374614358));
#100486=CARTESIAN_POINT('Ctrl Pts',(-9.90927040958652,19.7557107241877,
4.67476621863143));
#100487=CARTESIAN_POINT('Ctrl Pts',(-9.87458320834331,19.7581423614006,
4.67157062083553));
#100488=CARTESIAN_POINT('Ctrl Pts',(-9.77342230870075,19.7653964768915,
4.65770715480371));
#100489=CARTESIAN_POINT('Ctrl Pts',(-9.70766564010123,19.7703278005707,
4.64287446589006));
#100490=CARTESIAN_POINT('Ctrl Pts',(-9.58566361135629,19.7797266054412,
4.60413234679485));
#100491=CARTESIAN_POINT('Ctrl Pts',(-9.529286489425,19.7841761609002,4.5813016171111));
#100492=CARTESIAN_POINT('Ctrl Pts',(-9.46618039964194,19.789116514295,4.54986997633635));
#100493=CARTESIAN_POINT('Ctrl Pts',(-9.45749756252738,19.7897952092708,
4.54540970619246));
#100494=CARTESIAN_POINT('Ctrl Pts',(-9.44560020437287,19.790722705903,4.53911001597342));
#100495=CARTESIAN_POINT('Ctrl Pts',(-9.44233769905367,19.7909767864524,
4.53736277054947));
#100496=CARTESIAN_POINT('Ctrl Pts',(-9.43675805867344,19.7914108095985,
4.53434064587951));
#100497=CARTESIAN_POINT('Ctrl Pts',(-9.4344369077111,19.7915912115127,4.53307330097253));
#100498=CARTESIAN_POINT('Ctrl Pts',(-9.42959962153525,19.791966818013,4.53041096043378));
#100499=CARTESIAN_POINT('Ctrl Pts',(-9.42708430419931,19.7921619244093,
4.52901455037284));
#100500=CARTESIAN_POINT('Ctrl Pts',(-9.42095800466888,19.7926366873604,
4.52558403192004));
#100501=CARTESIAN_POINT('Ctrl Pts',(-9.41735254785636,19.7929157234149,
4.52354002691457));
#100502=CARTESIAN_POINT('Ctrl Pts',(-9.40442546891298,19.7939151215607,
4.51612096793535));
#100503=CARTESIAN_POINT('Ctrl Pts',(-9.39516647849559,19.7946289394325,
4.51063706398744));
#100504=CARTESIAN_POINT('Ctrl Pts',(-9.37223631340194,19.7963950756163,
4.49662798612296));
#100505=CARTESIAN_POINT('Ctrl Pts',(-9.35866212546349,19.7974391004056,
4.48794755613233));
#100506=CARTESIAN_POINT('Ctrl Pts',(-9.29998312044579,19.8019652652598,
4.44870416136977));
#100507=CARTESIAN_POINT('Ctrl Pts',(-9.25684901485212,19.8053290434821,
4.41530911333645));
#100508=CARTESIAN_POINT('Ctrl Pts',(-9.1553828257795,19.8137326492291,4.32483447172748));
#100509=CARTESIAN_POINT('Ctrl Pts',(-9.10038167563283,19.818768376362,4.26447029702423));
#100510=CARTESIAN_POINT('Ctrl Pts',(-9.04312986584215,19.8250606704396,
4.1868191808704));
#100511=CARTESIAN_POINT('Ctrl Pts',(-9.03444182074504,19.8260492352986,
4.17455052431923));
#100512=CARTESIAN_POINT('Ctrl Pts',(-9.02225389163279,19.82748777165,4.15662150801377));
#100513=CARTESIAN_POINT('Ctrl Pts',(-9.01856318507873,19.8279305940558,
4.15109218431998));
#100514=CARTESIAN_POINT('Ctrl Pts',(-9.012150976799,19.828712956748,4.14130716829582));
#100515=CARTESIAN_POINT('Ctrl Pts',(-9.00940964903017,19.829051751871,4.13706462148763));
#100516=CARTESIAN_POINT('Ctrl Pts',(-9.00380213034382,19.829753863258,4.12826258055273));
#100517=CARTESIAN_POINT('Ctrl Pts',(-9.00093975750705,19.8301173094164,
4.1237008063431));
#100518=CARTESIAN_POINT('Ctrl Pts',(-8.99366788701324,19.8310538568738,
4.11193309190051));
#100519=CARTESIAN_POINT('Ctrl Pts',(-8.98930451695686,19.8316286155903,
4.10469915219855));
#100520=CARTESIAN_POINT('Ctrl Pts',(-8.97103423981751,19.8340912626115,
4.07365900410973));
#100521=CARTESIAN_POINT('Ctrl Pts',(-8.95788876058976,19.8360059353588,
4.04941708511116));
#100522=CARTESIAN_POINT('Ctrl Pts',(-8.90128183863335,19.8449577586824,
3.93567278003121));
#100523=CARTESIAN_POINT('Ctrl Pts',(-8.86842553540125,19.8523382515614,
3.84135856033438));
#100524=CARTESIAN_POINT('Ctrl Pts',(-8.84323753409045,19.8611977026796,
3.72244938224359));
#100525=CARTESIAN_POINT('Ctrl Pts',(-8.8392682102299,19.8627975941922,3.70071107623423));
#100526=CARTESIAN_POINT('Ctrl Pts',(-8.83258978658459,19.8659429476777,
3.65724857194682));
#100527=CARTESIAN_POINT('Ctrl Pts',(-8.82986991932668,19.8674882135357,
3.63553399582588));
#100528=CARTESIAN_POINT('Ctrl Pts',(-8.8272234911941,19.8693863770422,3.6082625070403));
#100529=CARTESIAN_POINT('Ctrl Pts',(-8.82672912480367,19.8697667505298,
3.60276656291679));
#100530=CARTESIAN_POINT('Ctrl Pts',(-8.82600853391856,19.8703649372153,
3.59407116941341));
#100531=CARTESIAN_POINT('Ctrl Pts',(-8.82575672767739,19.8705841082841,
3.59087400825361));
#100532=CARTESIAN_POINT('Ctrl Pts',(-8.82533019478079,19.8709743664685,
3.58516028611495));
#100533=CARTESIAN_POINT('Ctrl Pts',(-8.82515049425902,19.8711457209473,
3.58264420527078));
#100534=CARTESIAN_POINT('Ctrl Pts',(-8.82473863113347,19.8715558726543,
3.57660448197468));
#100535=CARTESIAN_POINT('Ctrl Pts',(-8.82451423032849,19.8717942377292,
3.57308035253873));
#100536=CARTESIAN_POINT('Ctrl Pts',(-8.82387933802565,19.8725173410107,
3.56234874406912));
#100537=CARTESIAN_POINT('Ctrl Pts',(-8.82351925086111,19.8729993970934,
3.55513828769706));
#100538=CARTESIAN_POINT('Ctrl Pts',(-8.82087366611127,19.8773119659385,
3.49017693805894));
#100539=CARTESIAN_POINT('Ctrl Pts',(-8.82277551637046,19.8809379553014,
3.43232573194193));
#100540=CARTESIAN_POINT('Ctrl Pts',(-8.8397342467914,19.8908432126978,3.27364710826556));
#100541=CARTESIAN_POINT('Ctrl Pts',(-8.8636173534054,19.8970386072608,3.17429354386661));
#100542=CARTESIAN_POINT('Ctrl Pts',(-8.90468762747087,19.9045563031272,
3.06691783651471));
#100543=CARTESIAN_POINT('Ctrl Pts',(-8.90961085845438,19.9054259576994,
3.05466770734737));
#100544=CARTESIAN_POINT('Ctrl Pts',(-8.9172265018725,19.9067276320799,3.03660208529756));
#100545=CARTESIAN_POINT('Ctrl Pts',(-8.91976224021116,19.9071544107041,
3.03072134589832));
#100546=CARTESIAN_POINT('Ctrl Pts',(-8.92432829551426,19.9079115451808,
3.02036514318219));
#100547=CARTESIAN_POINT('Ctrl Pts',(-8.9263389163284,19.9082412280821,3.01588112218061));
#100548=CARTESIAN_POINT('Ctrl Pts',(-8.93030947881257,19.9088852132209,
3.00717250568848));
#100549=CARTESIAN_POINT('Ctrl Pts',(-8.93226653410931,19.9091994120708,
3.002946687963));
#100550=CARTESIAN_POINT('Ctrl Pts',(-8.93761240047505,19.9100491765944,
2.99158076800298));
#100551=CARTESIAN_POINT('Ctrl Pts',(-8.94104805609694,19.9105863410071,
2.98446309318307));
#100552=CARTESIAN_POINT('Ctrl Pts',(-8.95471086905163,19.912688732001,2.95687064307431));
#100553=CARTESIAN_POINT('Ctrl Pts',(-8.96546173993423,19.9142719213305,
2.93666233292482));
#100554=CARTESIAN_POINT('Ctrl Pts',(-8.99465638476766,19.9184010925096,
2.88544289330118));
#100555=CARTESIAN_POINT('Ctrl Pts',(-9.01394760968737,19.9209744989812,
2.85494459224756));
#100556=CARTESIAN_POINT('Ctrl Pts',(-9.0726024449445,19.9283784378158,2.77100819890187));
#100557=CARTESIAN_POINT('Ctrl Pts',(-9.11512363627019,19.9332845424425,
2.71994341536988));
#100558=CARTESIAN_POINT('Ctrl Pts',(-9.19328862141607,19.9414080419536,
2.64073719637236));
#100559=CARTESIAN_POINT('Ctrl Pts',(-9.22667392133962,19.9446511723571,
2.61057122740161));
#100560=CARTESIAN_POINT('Ctrl Pts',(-9.26638058771426,19.9481932641445,
2.57862406273584));
#100561=CARTESIAN_POINT('Ctrl Pts',(-9.27108396290685,19.9486080956115,
2.57489866798678));
#100562=CARTESIAN_POINT('Ctrl Pts',(-9.27865810334182,19.9492683105508,
2.56899306050476));
#100563=CARTESIAN_POINT('Ctrl Pts',(-9.28151068938987,19.9495152108158,
2.56678986038803));
#100564=CARTESIAN_POINT('Ctrl Pts',(-9.28659814469482,19.9499523785742,
2.56289771005367));
#100565=CARTESIAN_POINT('Ctrl Pts',(-9.28882897839037,19.950142999566,2.56120359628587));
#100566=CARTESIAN_POINT('Ctrl Pts',(-9.29363784592339,19.9505515880075,
2.5575786805811));
#100567=CARTESIAN_POINT('Ctrl Pts',(-9.29621776455562,19.9507693770259,
2.55565048752656));
#100568=CARTESIAN_POINT('Ctrl Pts',(-9.3034071771318,19.9513724662926,2.55032305334182));
#100569=CARTESIAN_POINT('Ctrl Pts',(-9.30803368176704,19.9517562304649,
2.54694675824155));
#100570=CARTESIAN_POINT('Ctrl Pts',(-9.33516370182266,19.9539826852576,
2.52744972804862));
#100571=CARTESIAN_POINT('Ctrl Pts',(-9.35820733967452,19.9557784206006,
2.51209119840029));
#100572=CARTESIAN_POINT('Ctrl Pts',(-9.43372348066762,19.9614378917222,
2.46551881474658));
#100573=CARTESIAN_POINT('Ctrl Pts',(-9.48808966504822,19.9651818522528,
2.43756445476573));
#100574=CARTESIAN_POINT('Ctrl Pts',(-9.61354454391748,19.9735993895092,
2.38493376537281));
#100575=CARTESIAN_POINT('Ctrl Pts',(-9.68531165407253,19.9782775217189,
2.3625952189228));
#100576=CARTESIAN_POINT('Ctrl Pts',(-9.76926308193124,19.9838973819999,
2.34502303630865));
#100577=CARTESIAN_POINT('Ctrl Pts',(-9.7798458273654,19.9846081061937,2.34295918836561));
#100578=CARTESIAN_POINT('Ctrl Pts',(-9.79415903839483,19.9855730677155,
2.34037129719402));
#100579=CARTESIAN_POINT('Ctrl Pts',(-9.79786609068529,19.985823321085,2.33971938221784));
#100580=CARTESIAN_POINT('Ctrl Pts',(-9.80475325438455,19.9862889044853,
2.33854222651863));
#100581=CARTESIAN_POINT('Ctrl Pts',(-9.80792268465862,19.9865034181986,
2.33801387450814));
#100582=CARTESIAN_POINT('Ctrl Pts',(-9.81110406371627,19.9867190062195,
2.33749693000169));
#100583=CARTESIAN_POINT('Origin',(-10.,12.3756328852638,3.5));
#100584=CARTESIAN_POINT('',(-9.81110406363821,20.5859883433483,2.33749693001438));
#100585=CARTESIAN_POINT('',(-9.81110406371067,20.4880078480432,2.3374969300026));
#100586=CARTESIAN_POINT('',(-9.81110406371068,12.3756328852638,2.3374969300026));
#100587=CARTESIAN_POINT('',(-11.1777499562264,20.2253931554249,3.50032110538681));
#100588=CARTESIAN_POINT('Ctrl Pts',(-9.81110406356574,20.5859883433483,
2.33749693002615));
#100589=CARTESIAN_POINT('Ctrl Pts',(-9.81073639201826,20.5859611875483,
2.33755667323291));
#100590=CARTESIAN_POINT('Ctrl Pts',(-9.81036874354825,20.5859340342295,
2.33761659172366));
#100591=CARTESIAN_POINT('Ctrl Pts',(-9.78819126391139,20.584296126581,2.34124182772966));
#100592=CARTESIAN_POINT('Ctrl Pts',(-9.76648498696821,20.5826957762589,
2.34542030371084));
#100593=CARTESIAN_POINT('Ctrl Pts',(-9.72358810022636,20.5795529188105,
2.35493736263092));
#100594=CARTESIAN_POINT('Ctrl Pts',(-9.70240198035234,20.5780105232236,
2.36025987622409));
#100595=CARTESIAN_POINT('Ctrl Pts',(-9.67606449026354,20.5761152783333,
2.36766114974818));
#100596=CARTESIAN_POINT('Ctrl Pts',(-9.67076481953176,20.5757350557232,
2.36919069459232));
#100597=CARTESIAN_POINT('Ctrl Pts',(-9.66240088682049,20.5751370078541,
2.37166840547774));
#100598=CARTESIAN_POINT('Ctrl Pts',(-9.65932949942044,20.5749178263563,
2.37259192876942));
#100599=CARTESIAN_POINT('Ctrl Pts',(-9.65384818347541,20.5745274876146,
2.37426452893913));
#100600=CARTESIAN_POINT('Ctrl Pts',(-9.65143690236066,20.5743560633141,
2.37500880090948));
#100601=CARTESIAN_POINT('Ctrl Pts',(-9.64565461365473,20.5739456596549,
2.37681395210539));
#100602=CARTESIAN_POINT('Ctrl Pts',(-9.64228596916589,20.5737071134228,
2.37788225930862));
#100603=CARTESIAN_POINT('Ctrl Pts',(-9.6320410580193,20.5729831544079,2.38118207877461));
#100604=CARTESIAN_POINT('Ctrl Pts',(-9.62518032564575,20.5725004321587,
2.38346180448838));
#100605=CARTESIAN_POINT('Ctrl Pts',(-9.56338174365886,20.568167534426,2.40463044101418));
#100606=CARTESIAN_POINT('Ctrl Pts',(-9.5098827134921,20.5645239770243,2.4274996833194));
#100607=CARTESIAN_POINT('Ctrl Pts',(-9.36826943834004,20.5546261007426,
2.50085617483137));
#100608=CARTESIAN_POINT('Ctrl Pts',(-9.28466172697889,20.5484529762735,
2.5589043661014));
#100609=CARTESIAN_POINT('Ctrl Pts',(-9.19949069819513,20.5409403722419,
2.63601910652487));
#100610=CARTESIAN_POINT('Ctrl Pts',(-9.18961845546957,20.5400490212924,
2.64527205835372));
#100611=CARTESIAN_POINT('Ctrl Pts',(-9.17528165568518,20.538722398289,2.65918119334069));
#100612=CARTESIAN_POINT('Ctrl Pts',(-9.17069218880232,20.5382926964171,
2.66370748862447));
#100613=CARTESIAN_POINT('Ctrl Pts',(-9.16260421545907,20.5375262914002,
2.67181618414751));
#100614=CARTESIAN_POINT('Ctrl Pts',(-9.15909093659463,20.5371902468025,
2.67538367796762));
#100615=CARTESIAN_POINT('Ctrl Pts',(-9.15174440813035,20.5364808495389,
2.68293934629228));
#100616=CARTESIAN_POINT('Ctrl Pts',(-9.14791630381486,20.5361072865817,
2.68693233131387));
#100617=CARTESIAN_POINT('Ctrl Pts',(-9.13785770776994,20.5351151891361,
2.69757321658443));
#100618=CARTESIAN_POINT('Ctrl Pts',(-9.13167609047031,20.5344946034875,
2.70426659313226));
#100619=CARTESIAN_POINT('Ctrl Pts',(-9.10236646992905,20.5314985774366,
2.73675091351327));
#100620=CARTESIAN_POINT('Ctrl Pts',(-9.0803084136442,20.5290797202521,2.76347974975143));
#100621=CARTESIAN_POINT('Ctrl Pts',(-9.01933954962103,20.521884405616,2.8443751124926));
#100622=CARTESIAN_POINT('Ctrl Pts',(-8.98381342920913,20.5170013789387,
2.900915767923));
#100623=CARTESIAN_POINT('Ctrl Pts',(-8.92503898786656,20.5075861273993,
3.01487587079966));
#100624=CARTESIAN_POINT('Ctrl Pts',(-8.90114669271512,20.5030719937658,
3.07173658175227));
#100625=CARTESIAN_POINT('Ctrl Pts',(-8.87874830853151,20.4980731418707,
3.13946602218613));
#100626=CARTESIAN_POINT('Ctrl Pts',(-8.87580224687535,20.4973952708207,
3.14876000779916));
#100627=CARTESIAN_POINT('Ctrl Pts',(-8.87189762322351,20.4964686300041,
3.16163070268488));
#100628=CARTESIAN_POINT('Ctrl Pts',(-8.87084010504099,20.4962145955425,
3.16517663402755));
#100629=CARTESIAN_POINT('Ctrl Pts',(-8.86905533645555,20.4957805918083,
3.17126572084837));
#100630=CARTESIAN_POINT('Ctrl Pts',(-8.86831991767989,20.4956001636798,
3.17380642262139));
#100631=CARTESIAN_POINT('Ctrl Pts',(-8.86680206358188,20.4952244321945,
3.17911717949799));
#100632=CARTESIAN_POINT('Ctrl Pts',(-8.86602121610177,20.4950292274547,
3.18188765269964));
#100633=CARTESIAN_POINT('Ctrl Pts',(-8.86413981711003,20.4945541044818,
3.18865787907789));
#100634=CARTESIAN_POINT('Ctrl Pts',(-8.86305021194824,20.4942748084008,
3.19266068899818));
#100635=CARTESIAN_POINT('Ctrl Pts',(-8.85920524850811,20.493273804736,3.20708599373197));
#100636=CARTESIAN_POINT('Ctrl Pts',(-8.85657177002975,20.4925586675594,
3.21754082879346));
#100637=CARTESIAN_POINT('Ctrl Pts',(-8.85035289272333,20.4907886984349,
3.24374351230246));
#100638=CARTESIAN_POINT('Ctrl Pts',(-8.84694705317454,20.4897422046864,
3.2595320915986));
#100639=CARTESIAN_POINT('Ctrl Pts',(-8.83343166562671,20.4851988191307,
3.32909865458305));
#100640=CARTESIAN_POINT('Ctrl Pts',(-8.82675138717847,20.4818211932636,
3.38347708022054));
#100641=CARTESIAN_POINT('Ctrl Pts',(-8.81961388951547,20.4734228332111,
3.51915056457533));
#100642=CARTESIAN_POINT('Ctrl Pts',(-8.8237354357337,20.4684056458646,3.60038767146555));
#100643=CARTESIAN_POINT('Ctrl Pts',(-8.83847783693928,20.4621336577842,
3.69541649029305));
#100644=CARTESIAN_POINT('Ctrl Pts',(-8.84106837096647,20.4611444515543,
3.71023507236384));
#100645=CARTESIAN_POINT('Ctrl Pts',(-8.8452125274448,20.4597050599514,3.73152794987668));
#100646=CARTESIAN_POINT('Ctrl Pts',(-8.84653840336031,20.4592620337759,
3.73804545861996));
#100647=CARTESIAN_POINT('Ctrl Pts',(-8.84896861495758,20.4584793414984,
3.74949418094076));
#100648=CARTESIAN_POINT('Ctrl Pts',(-8.85004962696088,20.4581404214439,
3.7544302141268));
#100649=CARTESIAN_POINT('Ctrl Pts',(-8.85234866049798,20.4574380799022,
3.76461384196006));
#100650=CARTESIAN_POINT('Ctrl Pts',(-8.85357098716073,20.457074528613,3.76986033289352));
#100651=CARTESIAN_POINT('Ctrl Pts',(-8.85680288337753,20.4561377687528,
3.78331397711061));
#100652=CARTESIAN_POINT('Ctrl Pts',(-8.85886483060423,20.4555629023922,
3.79150810583378));
#100653=CARTESIAN_POINT('Ctrl Pts',(-8.8680295003182,20.4531002816974,3.82634010419797));
#100654=CARTESIAN_POINT('Ctrl Pts',(-8.87597765704857,20.4511857484672,
3.85274442369307));
#100655=CARTESIAN_POINT('Ctrl Pts',(-8.9168572180483,20.44223147017,3.97307654656362));
#100656=CARTESIAN_POINT('Ctrl Pts',(-8.96068296716125,20.4348480785342,
4.06286221336357));
#100657=CARTESIAN_POINT('Ctrl Pts',(-9.02738149002707,20.4259856152306,
4.16452740842275));
#100658=CARTESIAN_POINT('Ctrl Pts',(-9.04002225594907,20.4243852649082,
4.18266116582207));
#100659=CARTESIAN_POINT('Ctrl Pts',(-9.0661541278816,20.4212424074616,4.21798598103389));
#100660=CARTESIAN_POINT('Ctrl Pts',(-9.07962872689841,20.419700011877,4.23517946835515));
#100661=CARTESIAN_POINT('Ctrl Pts',(-9.09709651131694,20.4178047669889,
4.25623460406264));
#100662=CARTESIAN_POINT('Ctrl Pts',(-9.10064818012581,20.417424544379,4.2604549910044));
#100663=CARTESIAN_POINT('Ctrl Pts',(-9.10631169703765,20.4168264965101,
4.26708967244059));
#100664=CARTESIAN_POINT('Ctrl Pts',(-9.10840392629794,20.4166073150124,
4.2695204938142));
#100665=CARTESIAN_POINT('Ctrl Pts',(-9.11216013350364,20.4162169762707,
4.27384869473795));
#100666=CARTESIAN_POINT('Ctrl Pts',(-9.11382027117275,20.4160455519702,
4.27574926315319));
#100667=CARTESIAN_POINT('Ctrl Pts',(-9.11781992301642,20.415635148311,4.28029857284411));
#100668=CARTESIAN_POINT('Ctrl Pts',(-9.12016526331128,20.4153966020788,
4.28294213575833));
#100669=CARTESIAN_POINT('Ctrl Pts',(-9.12734447967006,20.4146726430635,
4.29096122956591));
#100670=CARTESIAN_POINT('Ctrl Pts',(-9.13221609224328,20.4141899208141,
4.29630296982863));
#100671=CARTESIAN_POINT('Ctrl Pts',(-9.17667662839121,20.4098570230704,
4.34416147643956));
#100672=CARTESIAN_POINT('Ctrl Pts',(-9.21931738628219,20.4062134656592,
4.38374574424509));
#100673=CARTESIAN_POINT('Ctrl Pts',(-9.34390263378271,20.3963155893812,
4.48331486915842));
#100674=CARTESIAN_POINT('Ctrl Pts',(-9.43092347771074,20.390142464924,4.53610894636061));
#100675=CARTESIAN_POINT('Ctrl Pts',(-9.53600015323943,20.3826298609046,
4.58258129892083));
#100676=CARTESIAN_POINT('Ctrl Pts',(-9.54846704058526,20.3817385099534,
4.587840102455));
#100677=CARTESIAN_POINT('Ctrl Pts',(-9.567002835052,20.380411886948,4.59528538209383));
#100678=CARTESIAN_POINT('Ctrl Pts',(-9.57300384122338,20.3799821850758,
4.59763877969319));
#100679=CARTESIAN_POINT('Ctrl Pts',(-9.58370000472881,20.3792157800584,
4.60173247512458));
#100680=CARTESIAN_POINT('Ctrl Pts',(-9.58838754724043,20.3788797354607,
4.60349232902307));
#100681=CARTESIAN_POINT('Ctrl Pts',(-9.59827705223126,20.3781703381972,
4.60713338591671));
#100682=CARTESIAN_POINT('Ctrl Pts',(-9.60348131846986,20.3777967752402,
4.60900793250761));
#100683=CARTESIAN_POINT('Ctrl Pts',(-9.61729205581241,20.3768046777957,
4.61387284025146));
#100684=CARTESIAN_POINT('Ctrl Pts',(-9.62592021066983,20.3761840921479,
4.61680006173027));
#100685=CARTESIAN_POINT('Ctrl Pts',(-9.66751351904539,20.3731880661081,
4.6303750980549));
#100686=CARTESIAN_POINT('Ctrl Pts',(-9.70090068297981,20.3707692089342,
4.6396641134947));
#100687=CARTESIAN_POINT('Ctrl Pts',(-9.7995940032379,20.3635738943464,4.662487139047));
#100688=CARTESIAN_POINT('Ctrl Pts',(-9.86569352156252,20.3586908677085,
4.67196366563134));
#100689=CARTESIAN_POINT('Ctrl Pts',(-9.99370486433329,20.3492756161562,
4.67934175271247));
#100690=CARTESIAN_POINT('Ctrl Pts',(-10.0553679516324,20.3447614824703,
4.67805880004219));
#100691=CARTESIAN_POINT('Ctrl Pts',(-10.126354147867,20.3397626305271,4.67099305467454));
#100692=CARTESIAN_POINT('Ctrl Pts',(-10.1360432093052,20.3390847594772,
4.66990699008668));
#100693=CARTESIAN_POINT('Ctrl Pts',(-10.1493898054675,20.3381581186605,
4.66824288565207));
#100694=CARTESIAN_POINT('Ctrl Pts',(-10.1530594427439,20.337904084199,4.66776776876737));
#100695=CARTESIAN_POINT('Ctrl Pts',(-10.1593482735527,20.3374700804647,
4.66692338480501));
#100696=CARTESIAN_POINT('Ctrl Pts',(-10.161968545464,20.3372896523362,4.6665625782286));
#100697=CARTESIAN_POINT('Ctrl Pts',(-10.1674377517585,20.336913920851,4.66579069600065));
#100698=CARTESIAN_POINT('Ctrl Pts',(-10.1702864227244,20.3367187161112,
4.6653779996516));
#100699=CARTESIAN_POINT('Ctrl Pts',(-10.1772368627187,20.3362435931382,
4.66434503727578));
#100700=CARTESIAN_POINT('Ctrl Pts',(-10.1813369751643,20.3359642970572,
4.66371352749561));
#100701=CARTESIAN_POINT('Ctrl Pts',(-10.1960797090151,20.3349632933923,
4.6613630043238));
#100702=CARTESIAN_POINT('Ctrl Pts',(-10.2067023374316,20.3342481562155,
4.65951948849165));
#100703=CARTESIAN_POINT('Ctrl Pts',(-10.2331705512951,20.3324781870907,
4.6545507146789));
#100704=CARTESIAN_POINT('Ctrl Pts',(-10.2489803646816,20.331431693342,4.65124484413915));
#100705=CARTESIAN_POINT('Ctrl Pts',(-10.318034356667,20.3268883077846,4.63531629804634));
#100706=CARTESIAN_POINT('Ctrl Pts',(-10.3704332252228,20.3235106819161,
4.61931636456147));
#100707=CARTESIAN_POINT('Ctrl Pts',(-10.4972422789575,20.3151157560082,
4.57070967965573));
#100708=CARTESIAN_POINT('Ctrl Pts',(-10.5697429070831,20.3101020242223,
4.53395358826934));
#100709=CARTESIAN_POINT('Ctrl Pts',(-10.6503039417934,20.3038520009428,
4.48204781746084));
#100710=CARTESIAN_POINT('Ctrl Pts',(-10.6625656104499,20.3028811077379,
4.47381718645982));
#100711=CARTESIAN_POINT('Ctrl Pts',(-10.6797232635003,20.301492672393,4.46182606148965));
#100712=CARTESIAN_POINT('Ctrl Pts',(-10.6847497667246,20.301082197161,4.45825405923838));
#100713=CARTESIAN_POINT('Ctrl Pts',(-10.6938817081131,20.3003294969477,
4.45165605479284));
#100714=CARTESIAN_POINT('Ctrl Pts',(-10.6979960077748,20.2999877531958,
4.44864252656639));
#100715=CARTESIAN_POINT('Ctrl Pts',(-10.706111119976,20.2993083979176,4.44261722087401));
#100716=CARTESIAN_POINT('Ctrl Pts',(-10.7101125548101,20.2989708304174,
4.43960645857975));
#100717=CARTESIAN_POINT('Ctrl Pts',(-10.7195738353497,20.298166411297,4.43239263873652));
#100718=CARTESIAN_POINT('Ctrl Pts',(-10.7250161857706,20.2976986852138,
4.42816704539047));
#100719=CARTESIAN_POINT('Ctrl Pts',(-10.7367662851646,20.2966777604459,
4.41887753845133));
#100720=CARTESIAN_POINT('Ctrl Pts',(-10.74305953437,20.2961238765409,4.41379593582132));
#100721=CARTESIAN_POINT('Ctrl Pts',(-10.7603594095017,20.2945812436423,
4.39952994473833));
#100722=CARTESIAN_POINT('Ctrl Pts',(-10.77125114399,20.2935871237598,4.39020907371781));
#100723=CARTESIAN_POINT('Ctrl Pts',(-10.8063814603399,20.2903036980953,
4.35901674010213));
#100724=CARTESIAN_POINT('Ctrl Pts',(-10.8298794568478,20.2879831761069,
4.33633759967157));
#100725=CARTESIAN_POINT('Ctrl Pts',(-10.8880092789477,20.2819160964715,
4.27536892577747));
#100726=CARTESIAN_POINT('Ctrl Pts',(-10.9211203220358,20.2781283063199,
4.23572696446686));
#100727=CARTESIAN_POINT('Ctrl Pts',(-10.9869707754897,20.269923810293,4.14544713108034));
#100728=CARTESIAN_POINT('Ctrl Pts',(-11.0186466983019,20.2655179635429,
4.09420005360497));
#100729=CARTESIAN_POINT('Ctrl Pts',(-11.0507649879144,20.2606156713285,
4.03205622332839));
#100730=CARTESIAN_POINT('Ctrl Pts',(-11.0551510492866,20.2599349840516,
4.02330408316218));
#100731=CARTESIAN_POINT('Ctrl Pts',(-11.0610462800738,20.2590052211678,
4.01116492726664));
#100732=CARTESIAN_POINT('Ctrl Pts',(-11.0626491987577,20.2587508339966,
4.00782425369417));
#100733=CARTESIAN_POINT('Ctrl Pts',(-11.0653698643929,20.2583163851987,
4.00208477116824));
#100734=CARTESIAN_POINT('Ctrl Pts',(-11.0664953284914,20.2581358626886,
3.99968968375993));
#100735=CARTESIAN_POINT('Ctrl Pts',(-11.0688276000355,20.257760113066,3.99468262790467));
#100736=CARTESIAN_POINT('Ctrl Pts',(-11.0700329205486,20.2575649836713,
3.99207000531205));
#100737=CARTESIAN_POINT('Ctrl Pts',(-11.0729501651884,20.2570903355296,
3.98568525278006));
#100738=CARTESIAN_POINT('Ctrl Pts',(-11.074651807787,20.2568114359766,3.9819084094135));
#100739=CARTESIAN_POINT('Ctrl Pts',(-11.0806939252721,20.2558134563131,
3.96830659757076));
#100740=CARTESIAN_POINT('Ctrl Pts',(-11.0849200372567,20.255100894536,3.95843097886897));
#100741=CARTESIAN_POINT('Ctrl Pts',(-11.0951300998453,20.253338589886,3.93363966575459));
#100742=CARTESIAN_POINT('Ctrl Pts',(-11.1009451393259,20.2522970928123,
3.91865636169414));
#100743=CARTESIAN_POINT('Ctrl Pts',(-11.1250327618003,20.2477894196621,
3.8526143081343));
#100744=CARTESIAN_POINT('Ctrl Pts',(-11.1400745078617,20.2444406105812,
3.80044403117779));
#100745=CARTESIAN_POINT('Ctrl Pts',(-11.1689200755283,20.235952615356,3.66619924109002));
#100746=CARTESIAN_POINT('Ctrl Pts',(-11.1777273103824,20.2308183329953,
3.58338150555677));
#100747=CARTESIAN_POINT('Ctrl Pts',(-11.1777499562264,20.2253931554248,
3.50032110538561));
#100748=CARTESIAN_POINT('Ctrl Pts',(-11.1777499534635,20.2253938071954,
3.50033108412358));
#100749=CARTESIAN_POINT('Ctrl Pts',(-11.1777523518846,20.2248192267006,
3.49153415808618));
#100750=CARTESIAN_POINT('Ctrl Pts',(-11.1776563394807,20.2242418447553,
3.48273767565964));
#100751=CARTESIAN_POINT('Ctrl Pts',(-11.177311702439,20.2232141367527,3.46716407569449));
#100752=CARTESIAN_POINT('Ctrl Pts',(-11.1771031404095,20.2227650352233,
3.46038641281238));
#100753=CARTESIAN_POINT('Ctrl Pts',(-11.176641596819,20.2219858195418,3.44867756679113));
#100754=CARTESIAN_POINT('Ctrl Pts',(-11.1764161088448,20.2216565567637,
3.44374542585233));
#100755=CARTESIAN_POINT('Ctrl Pts',(-11.1759125429501,20.2210082332279,
3.43406538971739));
#100756=CARTESIAN_POINT('Ctrl Pts',(-11.1756367041683,20.2206892478258,
3.42931746908353));
#100757=CARTESIAN_POINT('Ctrl Pts',(-11.1749898935703,20.2200099539317,
3.41923883372543));
#100758=CARTESIAN_POINT('Ctrl Pts',(-11.1746113855777,20.2196494182659,
3.41390872742487));
#100759=CARTESIAN_POINT('Ctrl Pts',(-11.1735563648502,20.2187294442943,
3.40035784672447));
#100760=CARTESIAN_POINT('Ctrl Pts',(-11.1728297454345,20.2181684615175,
3.39214137779059));
#100761=CARTESIAN_POINT('Ctrl Pts',(-11.1696953433932,20.2159948809686,
3.36049082475049));
#100762=CARTESIAN_POINT('Ctrl Pts',(-11.1666711296417,20.2143633473612,
3.33712476093965));
#100763=CARTESIAN_POINT('Ctrl Pts',(-11.1453991290257,20.2049225232183,
3.20421887261046));
#100764=CARTESIAN_POINT('Ctrl Pts',(-11.1124310011361,20.1966476684144,
3.09761418234751));
#100765=CARTESIAN_POINT('Ctrl Pts',(-11.0496962918253,20.1859860650669,
2.96471931192452));
#100766=CARTESIAN_POINT('Ctrl Pts',(-11.0328656342338,20.1834132787226,
2.93292252538709));
#100767=CARTESIAN_POINT('Ctrl Pts',(-11.0114977457662,20.1804932262176,
2.89667189172198));
#100768=CARTESIAN_POINT('Ctrl Pts',(-11.0083497920221,20.1800709487296,
2.89142527417603));
#100769=CARTESIAN_POINT('Ctrl Pts',(-11.0034381886883,20.1794243934314,
2.88338197244157));
#100770=CARTESIAN_POINT('Ctrl Pts',(-11.0017034691587,20.1791983398307,
2.88056788024476));
#100771=CARTESIAN_POINT('Ctrl Pts',(-10.9984819636587,20.1787828117124,
2.87539082273478));
#100772=CARTESIAN_POINT('Ctrl Pts',(-10.9969986293577,20.1785931285669,
2.87302584627628));
#100773=CARTESIAN_POINT('Ctrl Pts',(-10.9936118006294,20.1781637298038,
2.86766841817856));
#100774=CARTESIAN_POINT('Ctrl Pts',(-10.9917031907188,20.1779243525982,
2.86467927621879));
#100775=CARTESIAN_POINT('Ctrl Pts',(-10.9867061658118,20.177304228134,2.85693064544739));
#100776=CARTESIAN_POINT('Ctrl Pts',(-10.9835967652343,20.17692480756,2.85218470301725));
#100777=CARTESIAN_POINT('Ctrl Pts',(-10.9621735290283,20.1743528001997,
2.81999584029923));
#100778=CARTESIAN_POINT('Ctrl Pts',(-10.9427459774541,20.1722270350799,
2.79330768335623));
#100779=CARTESIAN_POINT('Ctrl Pts',(-10.9029881733635,20.1681793530997,
2.74325458082259));
#100780=CARTESIAN_POINT('Ctrl Pts',(-10.8828080299801,20.166254594905,2.71980680567824));
#100781=CARTESIAN_POINT('Ctrl Pts',(-10.8287989665469,20.1613453636956,
2.66183481145911));
#100782=CARTESIAN_POINT('Ctrl Pts',(-10.7937276135609,20.1583766945129,
2.62855006666824));
#100783=CARTESIAN_POINT('Ctrl Pts',(-10.7292512219788,20.153116349402,2.5744882739032));
#100784=CARTESIAN_POINT('Ctrl Pts',(-10.7007559414711,20.150851067681,2.5527301848657));
#100785=CARTESIAN_POINT('Ctrl Pts',(-10.6587724170758,20.1475562426524,
2.52360511000773));
#100786=CARTESIAN_POINT('Ctrl Pts',(-10.6460625868608,20.1465641701671,
2.51514915858278));
#100787=CARTESIAN_POINT('Ctrl Pts',(-10.6260681542754,20.1450093039898,
2.50240032121892));
#100788=CARTESIAN_POINT('Ctrl Pts',(-10.6188953512204,20.1444526488642,
2.49793463729409));
#100789=CARTESIAN_POINT('Ctrl Pts',(-10.6053610733062,20.1434040053986,
2.4897091365988));
#100790=CARTESIAN_POINT('Ctrl Pts',(-10.5990110293552,20.1429126909859,
2.48593124478903));
#100791=CARTESIAN_POINT('Ctrl Pts',(-10.5882113704168,20.1420780469897,
2.47964293387874));
#100792=CARTESIAN_POINT('Ctrl Pts',(-10.5837801470256,20.1417358490932,
2.47710122827033));
#100793=CARTESIAN_POINT('Ctrl Pts',(-10.5748919949981,20.141049924237,2.47207963846551));
#100794=CARTESIAN_POINT('Ctrl Pts',(-10.5704352142344,20.140706207977,2.46959971830454));
#100795=CARTESIAN_POINT('Ctrl Pts',(-10.560553386624,20.1399445282237,2.46418485851698));
#100796=CARTESIAN_POINT('Ctrl Pts',(-10.5551211381641,20.1395260985697,
2.46126344724633));
#100797=CARTESIAN_POINT('Ctrl Pts',(-10.5365981999868,20.1381001203648,
2.45148878630345));
#100798=CARTESIAN_POINT('Ctrl Pts',(-10.5234020433121,20.1370855257098,
2.44483950984686));
#100799=CARTESIAN_POINT('Ctrl Pts',(-10.4369860569791,20.1304468619343,
2.40331618431191));
#100800=CARTESIAN_POINT('Ctrl Pts',(-10.3604680323456,20.1245713221996,
2.37584232468672));
#100801=CARTESIAN_POINT('Ctrl Pts',(-10.2286408593251,20.1146075391549,
2.34336251829231));
#100802=CARTESIAN_POINT('Ctrl Pts',(-10.174681864276,20.1105776391098,2.33399239900307));
#100803=CARTESIAN_POINT('Ctrl Pts',(-10.1042033625551,20.1054976724573,
2.32675773574855));
#100804=CARTESIAN_POINT('Ctrl Pts',(-10.0881088219053,20.1043501582151,
2.32543938343628));
#100805=CARTESIAN_POINT('Ctrl Pts',(-10.0612328296991,20.102459996989,2.3237934768731));
#100806=CARTESIAN_POINT('Ctrl Pts',(-10.0504651861512,20.1017096768983,
2.32328230650614));
#100807=CARTESIAN_POINT('Ctrl Pts',(-10.0355458261914,20.1006810306076,
2.32277922057519));
#100808=CARTESIAN_POINT('Ctrl Pts',(-10.0313992890752,20.1003963125062,
2.32266132517946));
#100809=CARTESIAN_POINT('Ctrl Pts',(-10.0243746095345,20.0999160532842,
2.32249873651406));
#100810=CARTESIAN_POINT('Ctrl Pts',(-10.0214967932199,20.0997198970324,
2.32244268264397));
#100811=CARTESIAN_POINT('Ctrl Pts',(-10.0159740566195,20.0993446305287,
2.32235536425518));
#100812=CARTESIAN_POINT('Ctrl Pts',(-10.0133292094032,20.0991654271388,
2.32232245877186));
#100813=CARTESIAN_POINT('Ctrl Pts',(-10.0069839998146,20.0987366840536,
2.32226489431862));
#100814=CARTESIAN_POINT('Ctrl Pts',(-10.0032835591551,20.0984876101652,
2.32224876371534));
#100815=CARTESIAN_POINT('Ctrl Pts',(-9.98983242764523,20.0975855260004,
2.32225352581305));
#100816=CARTESIAN_POINT('Ctrl Pts',(-9.98008184060888,20.0969379199024,
2.32237806612254));
#100817=CARTESIAN_POINT('Ctrl Pts',(-9.91697863991762,20.0927810965579,
2.32396808339277));
#100818=CARTESIAN_POINT('Ctrl Pts',(-9.86377934673636,20.0894339925388,
2.32893768609718));
#100819=CARTESIAN_POINT('Ctrl Pts',(-9.81110405611873,20.0861209582704,
2.33749693123622));
#100820=CARTESIAN_POINT('Ctrl Pts',(-9.81110406371629,19.9867190062195,
2.33749693000169));
#100821=CARTESIAN_POINT('Ctrl Pts',(-9.81408300875001,19.9869208761798,
2.33701287914126));
#100822=CARTESIAN_POINT('Ctrl Pts',(-9.81705392288393,19.9871224338232,
2.33654183422988));
#100823=CARTESIAN_POINT('Ctrl Pts',(-9.82309926517953,19.9875330584984,
2.33560711199982));
#100824=CARTESIAN_POINT('Ctrl Pts',(-9.82616391250262,19.9877414753334,
2.33514563915785));
#100825=CARTESIAN_POINT('Ctrl Pts',(-9.83479260505729,19.9883290187378,
2.33388114559629));
#100826=CARTESIAN_POINT('Ctrl Pts',(-9.84036056911844,19.9887090093696,
2.33310586763523));
#100827=CARTESIAN_POINT('Ctrl Pts',(-9.85546971521399,19.9897425786891,
2.33111224817086));
#100828=CARTESIAN_POINT('Ctrl Pts',(-9.86502044376763,19.9903985412879,
2.32997090231419));
#100829=CARTESIAN_POINT('Ctrl Pts',(-9.91336983910424,19.9937333288174,
2.32479283269449));
#100830=CARTESIAN_POINT('Ctrl Pts',(-9.95233393031936,19.9964676509658,
2.32256889282159));
#100831=CARTESIAN_POINT('Ctrl Pts',(-10.018655010393,20.0012028304539,2.32208082198291));
#100832=CARTESIAN_POINT('Ctrl Pts',(-10.0459743199467,20.0031764240022,
2.32283059498433));
#100833=CARTESIAN_POINT('Ctrl Pts',(-10.124754668176,20.0089225545093,2.32773925788832));
#100834=CARTESIAN_POINT('Ctrl Pts',(-10.176000535015,20.0127307415939,2.33433171477298));
#100835=CARTESIAN_POINT('Ctrl Pts',(-10.274516425143,20.0200715734531,2.35365126031592));
#100836=CARTESIAN_POINT('Ctrl Pts',(-10.3217628265244,20.0236003465914,
2.36600505292262));
#100837=CARTESIAN_POINT('Ctrl Pts',(-10.3742721558786,20.0274405126005,
2.38328272301918));
#100838=CARTESIAN_POINT('Ctrl Pts',(-10.3804159976824,20.0278885001588,
2.38536068754047));
#100839=CARTESIAN_POINT('Ctrl Pts',(-10.3897375670332,20.0285658396979,
2.38859947276409));
#100840=CARTESIAN_POINT('Ctrl Pts',(-10.3929278544304,20.028797235171,2.38972336553565));
#100841=CARTESIAN_POINT('Ctrl Pts',(-10.3987376679093,20.0292177997846,
2.39179825825361));
#100842=CARTESIAN_POINT('Ctrl Pts',(-10.4013586685951,20.0294072164162,
2.39274481362838));
#100843=CARTESIAN_POINT('Ctrl Pts',(-10.4072202674116,20.0298301334735,
2.39488523569953));
#100844=CARTESIAN_POINT('Ctrl Pts',(-10.4104589853413,20.0300633394703,
2.39608405637648));
#100845=CARTESIAN_POINT('Ctrl Pts',(-10.4198905754388,20.0307412275494,
2.39962243245576));
#100846=CARTESIAN_POINT('Ctrl Pts',(-10.4260691775891,20.0311837454883,
2.402000023942));
#100847=CARTESIAN_POINT('Ctrl Pts',(-10.4766953198986,20.0347993334587,
2.42197319592836));
#100848=CARTESIAN_POINT('Ctrl Pts',(-10.5200597499876,20.0378314754941,
2.44221019948332));
#100849=CARTESIAN_POINT('Ctrl Pts',(-10.5765731057789,20.041847787994,2.47290187046837));
#100850=CARTESIAN_POINT('Ctrl Pts',(-10.5909007814633,20.0428718525454,
2.48107733463048));
#100851=CARTESIAN_POINT('Ctrl Pts',(-10.6543390126385,20.0474517738232,
2.51906386232927));
#100852=CARTESIAN_POINT('Ctrl Pts',(-10.701398714838,20.0509786062734,2.55214198555983));
#100853=CARTESIAN_POINT('Ctrl Pts',(-10.768702724543,20.0564548063042,2.60721634288663));
#100854=CARTESIAN_POINT('Ctrl Pts',(-10.7908368869545,20.0583347070313,
2.62676271132575));
#100855=CARTESIAN_POINT('Ctrl Pts',(-10.8265638269669,20.06152904765,2.66078604611313));
#100856=CARTESIAN_POINT('Ctrl Pts',(-10.8405673593004,20.0628256887809,
2.67481259074185));
#100857=CARTESIAN_POINT('Ctrl Pts',(-10.859364479507,20.0646334520825,2.69461573330649));
#100858=CARTESIAN_POINT('Ctrl Pts',(-10.8644672203786,20.0651313392117,
2.7000952892779));
#100859=CARTESIAN_POINT('Ctrl Pts',(-10.8726631368383,20.0659429628049,
2.70906645928169));
#100860=CARTESIAN_POINT('Ctrl Pts',(-10.8757884822136,20.066255340196,2.71252850871705));
#100861=CARTESIAN_POINT('Ctrl Pts',(-10.8821691430148,20.0668991033908,
2.7196815486718));
#100862=CARTESIAN_POINT('Ctrl Pts',(-10.8854220477254,20.0672305803329,
2.72337455713588));
#100863=CARTESIAN_POINT('Ctrl Pts',(-10.8930565966765,20.0680164372405,
2.73215233893186));
#100864=CARTESIAN_POINT('Ctrl Pts',(-10.8974180674657,20.0684716303779,
2.73725435142679));
#100865=CARTESIAN_POINT('Ctrl Pts',(-10.9112304151462,20.0699335698288,
2.75369439265886));
#100866=CARTESIAN_POINT('Ctrl Pts',(-10.9205115355617,20.0709470651928,
2.765172532161));
#100867=CARTESIAN_POINT('Ctrl Pts',(-10.9796620141083,20.0776171570177,
2.8412046106869));
#100868=CARTESIAN_POINT('Ctrl Pts',(-11.0229166368048,20.0835284843486,
2.9106054093291));
#100869=CARTESIAN_POINT('Ctrl Pts',(-11.0824657962154,20.0935019930941,
3.03275624847548));
#100870=CARTESIAN_POINT('Ctrl Pts',(-11.1028729623652,20.0975054917523,
3.08320181648758));
#100871=CARTESIAN_POINT('Ctrl Pts',(-11.1247113915923,20.1025558120831,
3.1501740752645));
#100872=CARTESIAN_POINT('Ctrl Pts',(-11.1293853240724,20.103699116389,3.16557102945672));
#100873=CARTESIAN_POINT('Ctrl Pts',(-11.1366535284029,20.1055830474175,
3.19140743925264));
#100874=CARTESIAN_POINT('Ctrl Pts',(-11.1394228461299,20.1063312881727,
3.20179501940523));
#100875=CARTESIAN_POINT('Ctrl Pts',(-11.1430619584465,20.1073575239572,
3.21623674559256));
#100876=CARTESIAN_POINT('Ctrl Pts',(-11.1440530612351,20.1076418740774,
3.22025937051169));
#100877=CARTESIAN_POINT('Ctrl Pts',(-11.1456963428356,20.1081216472144,
3.22708384598744));
#100878=CARTESIAN_POINT('Ctrl Pts',(-11.1463595142758,20.1083176830717,
3.229882984959));
#100879=CARTESIAN_POINT('Ctrl Pts',(-11.1476127595621,20.1086928224003,
3.23526048233931));
#100880=CARTESIAN_POINT('Ctrl Pts',(-11.1482044099068,20.1088720183405,
3.23783842473664));
#100881=CARTESIAN_POINT('Ctrl Pts',(-11.1496033633604,20.1093008749394,
3.24402954109379));
#100882=CARTESIAN_POINT('Ctrl Pts',(-11.1504023303726,20.1095500688471,
3.24764459966185));
#100883=CARTESIAN_POINT('Ctrl Pts',(-11.1532479620208,20.1104536669804,
3.26081454202171));
#100884=CARTESIAN_POINT('Ctrl Pts',(-11.1551928111408,20.1111026411918,
3.27039135549404));
#100885=CARTESIAN_POINT('Ctrl Pts',(-11.1683076970161,20.1157257102722,
3.3393622053945));
#100886=CARTESIAN_POINT('Ctrl Pts',(-11.1750121087517,20.1194912788742,
3.39952190241154));
#100887=CARTESIAN_POINT('Ctrl Pts',(-11.1788398896702,20.1264591643744,
3.51198444674158));
#100888=CARTESIAN_POINT('Ctrl Pts',(-11.1771573165793,20.1296597207046,
3.56409033097425));
#100889=CARTESIAN_POINT('Ctrl Pts',(-11.1688640836789,20.1349485057596,
3.64794577320532));
#100890=CARTESIAN_POINT('Ctrl Pts',(-11.1643843926207,20.1369917582415,
3.67983310386289));
#100891=CARTESIAN_POINT('Ctrl Pts',(-11.1560551926117,20.1399894647762,
3.72546178889879));
#100892=CARTESIAN_POINT('Ctrl Pts',(-11.1532534539623,20.1409138732699,
3.73938059836828));
#100893=CARTESIAN_POINT('Ctrl Pts',(-11.1477711096285,20.1425877754625,
3.76428059411462));
#100894=CARTESIAN_POINT('Ctrl Pts',(-11.1451827087457,20.143334381969,3.7752804053697));
#100895=CARTESIAN_POINT('Ctrl Pts',(-11.1409780685346,20.1444851609889,
3.79206184151576));
#100896=CARTESIAN_POINT('Ctrl Pts',(-11.1394751874696,20.1448857183128,
3.79787139344392));
#100897=CARTESIAN_POINT('Ctrl Pts',(-11.1366589162444,20.1456174221612,
3.80842470196323));
#100898=CARTESIAN_POINT('Ctrl Pts',(-11.1353600517123,20.1459480956969,
3.81317222158315));
#100899=CARTESIAN_POINT('Ctrl Pts',(-11.132461868853,20.1466715344259,3.82351041838368));
#100900=CARTESIAN_POINT('Ctrl Pts',(-11.1308508351427,20.1470646699743,
3.82909764776214));
#100901=CARTESIAN_POINT('Ctrl Pts',(-11.1263171974171,20.1481470440211,
3.84439431831523));
#100902=CARTESIAN_POINT('Ctrl Pts',(-11.1233105327971,20.1488389822901,
3.8540781148118));
#100903=CARTESIAN_POINT('Ctrl Pts',(-11.1060586405339,20.1526736104553,
3.90720999113355));
#100904=CARTESIAN_POINT('Ctrl Pts',(-11.08941935221,20.155893639222,3.94983353891075));
#100905=CARTESIAN_POINT('Ctrl Pts',(-11.0360962360304,20.1650757658672,
4.06598498997737));
#100906=CARTESIAN_POINT('Ctrl Pts',(-10.9941393022134,20.1711714078078,
4.13680418674648));
#100907=CARTESIAN_POINT('Ctrl Pts',(-10.9295804304549,20.1790374335794,
4.22364202174625));
#100908=CARTESIAN_POINT('Ctrl Pts',(-10.9132995177798,20.1809194933138,
4.24408448819899));
#100909=CARTESIAN_POINT('Ctrl Pts',(-10.889715200559,20.1834931464585,4.27175551686923));
#100910=CARTESIAN_POINT('Ctrl Pts',(-10.8829778820513,20.1842121825738,
4.27945480422612));
#100911=CARTESIAN_POINT('Ctrl Pts',(-10.8710522641739,20.1854557171142,
4.29273008994474));
#100912=CARTESIAN_POINT('Ctrl Pts',(-10.8659087006168,20.185982913356,4.29834527132948));
#100913=CARTESIAN_POINT('Ctrl Pts',(-10.8582480389391,20.1867542555335,
4.30654719927686));
#100914=CARTESIAN_POINT('Ctrl Pts',(-10.8557730595638,20.1870013705768,
4.30917275807191));
#100915=CARTESIAN_POINT('Ctrl Pts',(-10.8513765439187,20.1874366033143,
4.31379402640196));
#100916=CARTESIAN_POINT('Ctrl Pts',(-10.8494599915744,20.1876250882883,
4.31579437374684));
#100917=CARTESIAN_POINT('Ctrl Pts',(-10.8452808539616,20.1880333853966,
4.32012553408611));
#100918=CARTESIAN_POINT('Ctrl Pts',(-10.8430156773208,20.1882529941397,
4.322453756858));
#100919=CARTESIAN_POINT('Ctrl Pts',(-10.8367505510495,20.1888558475691,
4.32884018092068));
#100920=CARTESIAN_POINT('Ctrl Pts',(-10.8327306730747,20.1892375929605,
4.33287883846769));
#100921=CARTESIAN_POINT('Ctrl Pts',(-10.8114767218962,20.191230638834,4.35392436846089));
#100922=CARTESIAN_POINT('Ctrl Pts',(-10.7937491855621,20.192806560208,4.37042732231724));
#100923=CARTESIAN_POINT('Ctrl Pts',(-10.6978053803539,20.2009741845307,
4.45437245742323));
#100924=CARTESIAN_POINT('Ctrl Pts',(-10.6114770902727,20.2071463496645,
4.51185899883369));
#100925=CARTESIAN_POINT('Ctrl Pts',(-10.4819244698483,20.2162628072759,
4.57541920215516));
#100926=CARTESIAN_POINT('Ctrl Pts',(-10.4441832936141,20.2188977988785,
4.59154857396462));
#100927=CARTESIAN_POINT('Ctrl Pts',(-10.3966876876106,20.2222308495901,
4.60897506787026));
#100928=CARTESIAN_POINT('Ctrl Pts',(-10.3876550550953,20.2228653870541,
4.61216472339869));
#100929=CARTESIAN_POINT('Ctrl Pts',(-10.3732508514827,20.2238787942883,
4.61705442713079));
#100930=CARTESIAN_POINT('Ctrl Pts',(-10.3679041268828,20.2242552914831,
4.61882677070917));
#100931=CARTESIAN_POINT('Ctrl Pts',(-10.3578011438012,20.2249674224564,
4.62209547880374));
#100932=CARTESIAN_POINT('Ctrl Pts',(-10.3530476810428,20.2253027771668,
4.62360013156433));
#100933=CARTESIAN_POINT('Ctrl Pts',(-10.342298847887,20.2260618413406,4.62692760528669));
#100934=CARTESIAN_POINT('Ctrl Pts',(-10.3362982351857,20.2264861106638,
4.62873283960243));
#100935=CARTESIAN_POINT('Ctrl Pts',(-10.3208411291097,20.2275804562918,
4.63324878254392));
#100936=CARTESIAN_POINT('Ctrl Pts',(-10.3113647224266,20.2282527763244,
4.63588900543347));
#100937=CARTESIAN_POINT('Ctrl Pts',(-10.2407967050034,20.2332708730553,
4.65460055847349));
#100938=CARTESIAN_POINT('Ctrl Pts',(-10.1785436077392,20.2377699938798,
4.665849600437));
#100939=CARTESIAN_POINT('Ctrl Pts',(-10.0413742919882,20.247797484014,4.67939013168238));
#100940=CARTESIAN_POINT('Ctrl Pts',(-9.96652313616605,20.2533444194973,
4.67964065471822));
#100941=CARTESIAN_POINT('Ctrl Pts',(-9.86406307194417,20.2607559088937,
4.67021874913391));
#100942=CARTESIAN_POINT('Ctrl Pts',(-9.83607242537982,20.2627599277497,
4.66662711229075));
#100943=CARTESIAN_POINT('Ctrl Pts',(-9.80255525819089,20.2651146206243,
4.66109593850998));
#100944=CARTESIAN_POINT('Ctrl Pts',(-9.79688197649627,20.2655116157713,
4.66011692359825));
#100945=CARTESIAN_POINT('Ctrl Pts',(-9.78803982648218,20.266127664956,4.65852421746741));
#100946=CARTESIAN_POINT('Ctrl Pts',(-9.78486601127488,20.2663482479126,
4.65793905070471));
#100947=CARTESIAN_POINT('Ctrl Pts',(-9.77894299369496,20.2667588382207,
4.65682181132248));
#100948=CARTESIAN_POINT('Ctrl Pts',(-9.77619330403156,20.2669490142444,
4.65629298460916));
#100949=CARTESIAN_POINT('Ctrl Pts',(-9.76991815316187,20.2673820542309,
4.65506290999898));
#100950=CARTESIAN_POINT('Ctrl Pts',(-9.76639399518316,20.2676245591421,
4.65435532557077));
#100951=CARTESIAN_POINT('Ctrl Pts',(-9.75702926421882,20.2682672567095,
4.65243042176241));
#100952=CARTESIAN_POINT('Ctrl Pts',(-9.75119451603392,20.268665920597,4.65118482020051));
#100953=CARTESIAN_POINT('Ctrl Pts',(-9.70483843885487,20.2718209449277,
4.64091981363938));
#100954=CARTESIAN_POINT('Ctrl Pts',(-9.66480537073408,20.2744711113973,
4.62980695412016));
#100955=CARTESIAN_POINT('Ctrl Pts',(-9.53209473436853,20.2832570607057,
4.58528947107605));
#100956=CARTESIAN_POINT('Ctrl Pts',(-9.44304826250539,20.2891869346684,
4.54239816186425));
#100957=CARTESIAN_POINT('Ctrl Pts',(-9.33604811866747,20.2973402573462,
4.47319182797513));
#100958=CARTESIAN_POINT('Ctrl Pts',(-9.31231178609172,20.2992199279908,
4.45656632586875));
#100959=CARTESIAN_POINT('Ctrl Pts',(-9.28236234030519,20.3016999669239,
4.43389779413292));
#100960=CARTESIAN_POINT('Ctrl Pts',(-9.27556786939737,20.3022701271856,
4.42863716388637));
#100961=CARTESIAN_POINT('Ctrl Pts',(-9.26458504300649,20.3032044681092,
4.41993980634557));
#100962=CARTESIAN_POINT('Ctrl Pts',(-9.26036168228592,20.3035668868986,
4.41654763300599));
#100963=CARTESIAN_POINT('Ctrl Pts',(-9.25225531093067,20.3042686700832,
4.40994413650025));
#100964=CARTESIAN_POINT('Ctrl Pts',(-9.24836920554888,20.3046078705389,
4.4067367859831));
#100965=CARTESIAN_POINT('Ctrl Pts',(-9.23946281579941,20.305391765671,4.39928940514371));
#100966=CARTESIAN_POINT('Ctrl Pts',(-9.23445723598799,20.3058371532488,
4.39503213136836));
#100967=CARTESIAN_POINT('Ctrl Pts',(-9.21844644696224,20.3072776016231,
4.3811822938852));
#100968=CARTESIAN_POINT('Ctrl Pts',(-9.20758425686547,20.3082793037851,
4.37142724768611));
#100969=CARTESIAN_POINT('Ctrl Pts',(-9.13049733805307,20.3155708501724,
4.29956430879739));
#100970=CARTESIAN_POINT('Ctrl Pts',(-9.07148163118422,20.3221840277917,
4.23019545948758));
#100971=CARTESIAN_POINT('Ctrl Pts',(-8.98373250859426,20.3337744633714,
4.0989955050327));
#100972=CARTESIAN_POINT('Ctrl Pts',(-8.95126630111046,20.3386971347639,
4.04014340697384));
#100973=CARTESIAN_POINT('Ctrl Pts',(-8.9210555250416,20.3438695204285,3.97225610637989));
#100974=CARTESIAN_POINT('Ctrl Pts',(-8.91818558161619,20.3443681380605,
3.96564426416064));
#100975=CARTESIAN_POINT('Ctrl Pts',(-8.91400110583827,20.3451057372637,
3.95575642344514));
#100976=CARTESIAN_POINT('Ctrl Pts',(-8.91264037301394,20.3453473362789,
3.9525003403922));
#100977=CARTESIAN_POINT('Ctrl Pts',(-8.91033219988537,20.3457601133023,
3.94690660046814));
#100978=CARTESIAN_POINT('Ctrl Pts',(-8.90937761380526,20.3459317132304,
3.94457196866307));
#100979=CARTESIAN_POINT('Ctrl Pts',(-8.90722572103314,20.3463205715296,
3.93926043824021));
#100980=CARTESIAN_POINT('Ctrl Pts',(-8.90603307456667,20.3465375506226,
3.93628170263555));
#100981=CARTESIAN_POINT('Ctrl Pts',(-8.90282003305195,20.3471262186187,
3.9281608403798));
#100982=CARTESIAN_POINT('Ctrl Pts',(-8.90082359108345,20.3474965213031,
3.92300923177427));
#100983=CARTESIAN_POINT('Ctrl Pts',(-8.89107253009644,20.349329021177,3.89731241876125));
#100984=CARTESIAN_POINT('Ctrl Pts',(-8.88385676699028,20.3507622587048,
3.87656569779962));
#100985=CARTESIAN_POINT('Ctrl Pts',(-8.87056402833909,20.3535925480839,
3.83459834429438));
#100986=CARTESIAN_POINT('Ctrl Pts',(-8.86449496176476,20.354988842516,3.81338486116286));
#100987=CARTESIAN_POINT('Ctrl Pts',(-8.83433743056372,20.3626184203353,
3.69555088010709));
#100988=CARTESIAN_POINT('Ctrl Pts',(-8.82198209778227,20.368615430995,3.59635181199653));
#100989=CARTESIAN_POINT('Ctrl Pts',(-8.82232944552952,20.3767569879161,
3.46933919565376));
#100990=CARTESIAN_POINT('Ctrl Pts',(-8.8233634238491,20.3785396462803,3.44191214365526));
#100991=CARTESIAN_POINT('Ctrl Pts',(-8.82596604229665,20.3809089681309,
3.40613593337647));
#100992=CARTESIAN_POINT('Ctrl Pts',(-8.82666831108206,20.3814687538488,
3.39773104833931));
#100993=CARTESIAN_POINT('Ctrl Pts',(-8.82796652857682,20.3823903804405,
3.38397597169515));
#100994=CARTESIAN_POINT('Ctrl Pts',(-8.82850900309326,20.3827505511097,
3.37862094163837));
#100995=CARTESIAN_POINT('Ctrl Pts',(-8.82963181697876,20.383451041018,3.368246800042));
#100996=CARTESIAN_POINT('Ctrl Pts',(-8.83020778602453,20.3837912164987,
3.36322732627408));
#100997=CARTESIAN_POINT('Ctrl Pts',(-8.83161728091387,20.384581864851,3.35160464816089));
#100998=CARTESIAN_POINT('Ctrl Pts',(-8.83247451198979,20.3850330690549,
3.34500454719157));
#100999=CARTESIAN_POINT('Ctrl Pts',(-8.83545608008461,20.3865121235132,
3.3234785788683));
#101000=CARTESIAN_POINT('Ctrl Pts',(-8.83781100190216,20.3875471233238,
3.30858670494187));
#101001=CARTESIAN_POINT('Ctrl Pts',(-8.85437118664686,20.3940947090039,
3.21548680961937));
#101002=CARTESIAN_POINT('Ctrl Pts',(-8.87617538606468,20.399847606979,3.13885309593576));
#101003=CARTESIAN_POINT('Ctrl Pts',(-8.92620128444489,20.4097850789373,
3.01298250203244));
#101004=CARTESIAN_POINT('Ctrl Pts',(-8.95056442064478,20.4139127774069,
2.96249162144857));
#101005=CARTESIAN_POINT('Ctrl Pts',(-8.98656465152177,20.4191018740922,
2.89974070847826));
#101006=CARTESIAN_POINT('Ctrl Pts',(-8.9949962953391,20.4202643623101,2.88572804625186));
#101007=CARTESIAN_POINT('Ctrl Pts',(-9.00951969146962,20.422176421368,2.86269144936422));
#101008=CARTESIAN_POINT('Ctrl Pts',(-9.01544944947884,20.4229338824131,
2.85356851481118));
#101009=CARTESIAN_POINT('Ctrl Pts',(-9.02382163013007,20.4239705398153,
2.84107042965553));
#101010=CARTESIAN_POINT('Ctrl Pts',(-9.02615658320928,20.4242562577699,
2.8376244347983));
#101011=CARTESIAN_POINT('Ctrl Pts',(-9.03013814158257,20.4247376586581,
2.83181489493639));
#101012=CARTESIAN_POINT('Ctrl Pts',(-9.03177522318189,20.4249339639694,
2.82944490064837));
#101013=CARTESIAN_POINT('Ctrl Pts',(-9.03492973482754,20.4253090837398,
2.82491376965978));
#101014=CARTESIAN_POINT('Ctrl Pts',(-9.03644575406605,20.4254879938058,
2.82275170682457));
#101015=CARTESIAN_POINT('Ctrl Pts',(-9.04009525359847,20.4259154687999,
2.81758405259375));
#101016=CARTESIAN_POINT('Ctrl Pts',(-9.04223561305342,20.4261635736663,
2.81458331837639));
#101017=CARTESIAN_POINT('Ctrl Pts',(-9.0500273488531,20.4270576235192,2.80376725143966));
#101018=CARTESIAN_POINT('Ctrl Pts',(-9.05576077101138,20.4276982915424,
2.7960111000178));
#101019=CARTESIAN_POINT('Ctrl Pts',(-9.1031808361541,20.4328674015646,2.73348316548014));
#101020=CARTESIAN_POINT('Ctrl Pts',(-9.14950639622086,20.4371231263793,
2.68238398189278));
#101021=CARTESIAN_POINT('Ctrl Pts',(-9.20411829190496,20.4417237355264,
2.63184201009508));
#101022=CARTESIAN_POINT('Ctrl Pts',(-9.20822645376329,20.4420674728578,
2.62809367461966));
#101023=CARTESIAN_POINT('Ctrl Pts',(-9.2753123662906,20.4476453646053,2.56774882981793));
#101024=CARTESIAN_POINT('Ctrl Pts',(-9.3441769549188,20.4528936258488,2.51808455820018));
#101025=CARTESIAN_POINT('Ctrl Pts',(-9.42762960266571,20.4591959935333,
2.47062350448235));
#101026=CARTESIAN_POINT('Ctrl Pts',(-9.43757425852956,20.4599457259568,
2.46515647951714));
#101027=CARTESIAN_POINT('Ctrl Pts',(-9.4529047014324,20.4611003228303,2.45701489633801));
#101028=CARTESIAN_POINT('Ctrl Pts',(-9.45823473956995,20.4615015340753,
2.45423635916133));
#101029=CARTESIAN_POINT('Ctrl Pts',(-9.46796793061911,20.4622339136259,
2.44925684888665));
#101030=CARTESIAN_POINT('Ctrl Pts',(-9.47236408450377,20.4625646043538,
2.44704243586168));
#101031=CARTESIAN_POINT('Ctrl Pts',(-9.48197568793369,20.4632874651336,
2.44227622395185));
#101032=CARTESIAN_POINT('Ctrl Pts',(-9.48719636264972,20.4636800014172,
2.43973531524629));
#101033=CARTESIAN_POINT('Ctrl Pts',(-9.50155067995783,20.4647591458223,
2.43287986859508));
#101034=CARTESIAN_POINT('Ctrl Pts',(-9.51072120002847,20.4654484273041,
2.42864415607073));
#101035=CARTESIAN_POINT('Ctrl Pts',(-9.56101938236463,20.4692291430415,
2.40619272905638));
#101036=CARTESIAN_POINT('Ctrl Pts',(-9.60310528787536,20.4723953026317,
2.39022885037411));
#101037=CARTESIAN_POINT('Ctrl Pts',(-9.70005177390833,20.4796933059368,
2.35967622004625));
#101038=CARTESIAN_POINT('Ctrl Pts',(-9.7552330849743,20.4838522304599,2.34657544438436));
#101039=CARTESIAN_POINT('Ctrl Pts',(-9.81110406371067,20.4880078480432,
2.3374969300026));
#101040=CARTESIAN_POINT('Origin',(-10.,12.3756328852638,3.5));
#101041=CARTESIAN_POINT('',(-9.81110406342901,21.0876323086995,2.33749693004837));
#101042=CARTESIAN_POINT('',(-9.81110406371115,20.988570409963,2.33749693000252));
#101043=CARTESIAN_POINT('',(-9.81110406371068,12.3756328852638,2.3374969300026));
#101044=CARTESIAN_POINT('Ctrl Pts',(-9.81110406314734,21.0876323086995,
2.33749693009414));
#101045=CARTESIAN_POINT('Ctrl Pts',(-9.78669199051518,21.0859356484233,
2.34146366484929));
#101046=CARTESIAN_POINT('Ctrl Pts',(-9.76241192458018,21.0842152344288,
2.34619821170569));
#101047=CARTESIAN_POINT('Ctrl Pts',(-9.64130261182356,21.0754627572677,
2.37379915618023));
#101048=CARTESIAN_POINT('Ctrl Pts',(-9.54750680248557,21.0680820720503,
2.40810433745266));
#101049=CARTESIAN_POINT('Ctrl Pts',(-9.43952359959329,21.0592221588631,
2.46392575164076));
#101050=CARTESIAN_POINT('Ctrl Pts',(-9.42017684661617,21.0576215132717,
2.47462745874384));
#101051=CARTESIAN_POINT('Ctrl Pts',(-9.3823584273696,21.0544801858814,2.49695972201989));
#101052=CARTESIAN_POINT('Ctrl Pts',(-9.3638852206975,21.0529395630909,2.50857221755907));
#101053=CARTESIAN_POINT('Ctrl Pts',(-9.34115921590794,21.0510461726802,
2.52375500780569));
#101054=CARTESIAN_POINT('Ctrl Pts',(-9.33659597150281,21.0506660938874,
2.52685018546233));
#101055=CARTESIAN_POINT('Ctrl Pts',(-9.3294134132817,21.0500682215491,2.5317960054331));
#101056=CARTESIAN_POINT('Ctrl Pts',(-9.3267797034674,21.0498490730532,2.533625446143));
#101057=CARTESIAN_POINT('Ctrl Pts',(-9.32208668480273,21.0494587621584,
2.53691383128695));
#101058=CARTESIAN_POINT('Ctrl Pts',(-9.32002460373643,21.0492873329456,
2.53836862990898));
#101059=CARTESIAN_POINT('Ctrl Pts',(-9.3150855375975,21.048876877795,2.54187697286218));
#101060=CARTESIAN_POINT('Ctrl Pts',(-9.31221310412364,21.0486382852997,
2.54393685217884));
#101061=CARTESIAN_POINT('Ctrl Pts',(-9.30349134601167,21.0479140445281,
2.55025104902241));
#101062=CARTESIAN_POINT('Ctrl Pts',(-9.29767176419438,21.0474310898435,
2.55454644183668));
#101063=CARTESIAN_POINT('Ctrl Pts',(-9.24537163718046,21.0430897716534,
2.59389821806427));
#101064=CARTESIAN_POINT('Ctrl Pts',(-9.20150380175031,21.0394389045419,
2.63230757303238));
#101065=CARTESIAN_POINT('Ctrl Pts',(-9.08965148198178,21.0295439043259,
2.74594117131653));
#101066=CARTESIAN_POINT('Ctrl Pts',(-9.02825244561503,21.0233798784461,
2.82691473257492));
#101067=CARTESIAN_POINT('Ctrl Pts',(-8.97122768240046,21.0158767722741,
2.92649655635056));
#101068=CARTESIAN_POINT('Ctrl Pts',(-8.96469762492873,21.0149840942198,
2.93837054138884));
#101069=CARTESIAN_POINT('Ctrl Pts',(-8.9553640054531,21.0136558697823,2.95605854900735));
#101070=CARTESIAN_POINT('Ctrl Pts',(-8.9524008723563,21.0132259133756,2.96178746931989));
#101071=CARTESIAN_POINT('Ctrl Pts',(-8.94722110563449,21.012459222582,2.97200687770881));
#101072=CARTESIAN_POINT('Ctrl Pts',(-8.94498575674969,21.0121231485311,
2.97648774339135));
#101073=CARTESIAN_POINT('Ctrl Pts',(-8.94034228998832,21.0114138621029,
2.98594632966647));
#101074=CARTESIAN_POINT('Ctrl Pts',(-8.93794052322276,21.0110404405146,
2.99092701471001));
#101075=CARTESIAN_POINT('Ctrl Pts',(-8.9316784008216,21.0100491233369,3.0041503597757));
#101076=CARTESIAN_POINT('Ctrl Pts',(-8.92787843399149,21.0094291823531,
3.01242103759702));
#101077=CARTESIAN_POINT('Ctrl Pts',(-8.91012395421612,21.0064416101893,
3.05227520173655));
#101078=CARTESIAN_POINT('Ctrl Pts',(-8.89746831222553,21.004030860246,3.08441518026381));
#101079=CARTESIAN_POINT('Ctrl Pts',(-8.86469628629428,20.996872323369,3.17973098606907));
#101080=CARTESIAN_POINT('Ctrl Pts',(-8.84847909249629,20.9920193651218,
3.24410053370179));
#101081=CARTESIAN_POINT('Ctrl Pts',(-8.8277159923457,20.9825942490547,3.37076540366857));
#101082=CARTESIAN_POINT('Ctrl Pts',(-8.82253212118833,20.9780401745215,
3.43275166958482));
#101083=CARTESIAN_POINT('Ctrl Pts',(-8.82221868157714,20.9730046328318,
3.50461158542088));
#101084=CARTESIAN_POINT('Ctrl Pts',(-8.8222972006709,20.9723267763767,3.51436080324933));
#101085=CARTESIAN_POINT('Ctrl Pts',(-8.82257251350386,20.9714001517486,
3.52780769143182));
#101086=CARTESIAN_POINT('Ctrl Pts',(-8.82266568946645,20.971146119123,3.53150675848965));
#101087=CARTESIAN_POINT('Ctrl Pts',(-8.82285536156098,20.9707121177052,
3.53784915383879));
#101088=CARTESIAN_POINT('Ctrl Pts',(-8.82294333124047,20.9705316900678,
3.54049268001567));
#101089=CARTESIAN_POINT('Ctrl Pts',(-8.8231456298481,20.9701559586746,3.54601237969055));
#101090=CARTESIAN_POINT('Ctrl Pts',(-8.82326159811414,20.9699607535405,
3.54888845874206));
#101091=CARTESIAN_POINT('Ctrl Pts',(-8.82357043861667,20.9694856280864,
3.55590848502478));
#101092=CARTESIAN_POINT('Ctrl Pts',(-8.82377466590847,20.969206329934,3.56005194700047));
#101093=CARTESIAN_POINT('Ctrl Pts',(-8.82458839400337,20.9682053104522,
3.57495892906291));
#101094=CARTESIAN_POINT('Ctrl Pts',(-8.82532380242086,20.967490159803,3.58571543497015));
#101095=CARTESIAN_POINT('Ctrl Pts',(-8.82752953646553,20.9657201505589,
3.6125561386714));
#101096=CARTESIAN_POINT('Ctrl Pts',(-8.8291832165579,20.9646736306487,3.62862342797687));
#101097=CARTESIAN_POINT('Ctrl Pts',(-8.83788757522245,20.9601300574398,
3.69895713798967));
#101098=CARTESIAN_POINT('Ctrl Pts',(-8.84838514535335,20.9567522800959,
3.75273188740912));
#101099=CARTESIAN_POINT('Ctrl Pts',(-8.88363617234454,20.9483539718096,
3.88393927337368));
#101100=CARTESIAN_POINT('Ctrl Pts',(-8.91272408536712,20.9433369819059,
3.959898404717));
#101101=CARTESIAN_POINT('Ctrl Pts',(-8.95618275692231,20.9370652111846,
4.04568022285635));
#101102=CARTESIAN_POINT('Ctrl Pts',(-8.96323716672006,20.9360759993633,
4.05896702636032));
#101103=CARTESIAN_POINT('Ctrl Pts',(-8.97377471958143,20.934636601082,4.07792817233288));
#101104=CARTESIAN_POINT('Ctrl Pts',(-8.97705470975434,20.9341935739138,
4.08371416691566));
#101105=CARTESIAN_POINT('Ctrl Pts',(-8.98291255601862,20.9334108804781,
4.09384655172591));
#101106=CARTESIAN_POINT('Ctrl Pts',(-8.98546972927173,20.933071960265,4.09820475099651));
#101107=CARTESIAN_POINT('Ctrl Pts',(-8.99081087149148,20.9323696189764,
4.10717492146276));
#101108=CARTESIAN_POINT('Ctrl Pts',(-8.9935985916655,20.9320060681025,4.11178450943681));
#101109=CARTESIAN_POINT('Ctrl Pts',(-9.00083984051157,20.9310693105475,
4.12357472070711));
#101110=CARTESIAN_POINT('Ctrl Pts',(-9.00533913346802,20.9304944460926,
4.13072673220846));
#101111=CARTESIAN_POINT('Ctrl Pts',(-9.02484482951817,20.9280318452134,
4.16100488266863));
#101112=CARTESIAN_POINT('Ctrl Pts',(-9.04058268662516,20.9261173304307,
4.18364702908351));
#101113=CARTESIAN_POINT('Ctrl Pts',(-9.11673357592585,20.9171630595168,
4.28539172899552));
#101114=CARTESIAN_POINT('Ctrl Pts',(-9.1862215247651,20.9097796539466,4.35718049325871));
#101115=CARTESIAN_POINT('Ctrl Pts',(-9.28113739330453,20.9009171775087,
4.43317736478721));
#101116=CARTESIAN_POINT('Ctrl Pts',(-9.29877456296343,20.8993168287003,
4.44650220380941));
#101117=CARTESIAN_POINT('Ctrl Pts',(-9.33456543634704,20.8961739633963,
4.47199219586792));
#101118=CARTESIAN_POINT('Ctrl Pts',(-9.35270420292256,20.8946315587097,
4.48416476650416));
#101119=CARTESIAN_POINT('Ctrl Pts',(-9.37583613841283,20.892736304301,4.49877172580266));
#101120=CARTESIAN_POINT('Ctrl Pts',(-9.38052066368577,20.8923560809533,
4.50168400269279));
#101121=CARTESIAN_POINT('Ctrl Pts',(-9.38796114902377,20.8917580321838,
4.50623744381136));
#101122=CARTESIAN_POINT('Ctrl Pts',(-9.39070357622337,20.8915388505167,
4.50790040035192));
#101123=CARTESIAN_POINT('Ctrl Pts',(-9.39561597200463,20.8911485116321,
4.51085180792733));
#101124=CARTESIAN_POINT('Ctrl Pts',(-9.39778327729904,20.8909770873568,
4.51214448077551));
#101125=CARTESIAN_POINT('Ctrl Pts',(-9.40299563997969,20.8905666839615,
4.51523068565759));
#101126=CARTESIAN_POINT('Ctrl Pts',(-9.40604463233112,20.8903281379665,
4.5170174890443));
#101127=CARTESIAN_POINT('Ctrl Pts',(-9.41535513971012,20.8896041803956,
4.52241758147703));
#101128=CARTESIAN_POINT('Ctrl Pts',(-9.42164206456965,20.8891214593377,
4.52598705088422));
#101129=CARTESIAN_POINT('Ctrl Pts',(-9.4787423845804,20.8847886046984,4.55771470497031));
#101130=CARTESIAN_POINT('Ctrl Pts',(-9.53154880003644,20.8811450847087,
4.58213921619906));
#101131=CARTESIAN_POINT('Ctrl Pts',(-9.68085334373629,20.8712471936509,
4.63820800628006));
#101132=CARTESIAN_POINT('Ctrl Pts',(-9.77995017932046,20.8650740225832,
4.66144224191181));
#101133=CARTESIAN_POINT('Ctrl Pts',(-9.8942555546854,20.8575613699168,4.67307128342787));
#101134=CARTESIAN_POINT('Ctrl Pts',(-9.90773820770885,20.856670025786,4.67420861041895));
#101135=CARTESIAN_POINT('Ctrl Pts',(-9.92766854568426,20.8553434110113,
4.67554445834274));
#101136=CARTESIAN_POINT('Ctrl Pts',(-9.93410338948209,20.8549137104477,
4.67592272142389));
#101137=CARTESIAN_POINT('Ctrl Pts',(-9.94554154627658,20.8541473068993,
4.67650091780684));
#101138=CARTESIAN_POINT('Ctrl Pts',(-9.95054367834808,20.8538112624526,
4.6767218038702));
#101139=CARTESIAN_POINT('Ctrl Pts',(-9.96107465919125,20.8531018646175,
4.67711956866531));
#101140=CARTESIAN_POINT('Ctrl Pts',(-9.96660363597277,20.8527283009321,
4.67728940458727));
#101141=CARTESIAN_POINT('Ctrl Pts',(-9.98124212897334,20.8517361994674,
4.67763585965445));
#101142=CARTESIAN_POINT('Ctrl Pts',(-9.99035269901281,20.8511156104981,
4.67774572685489));
#101143=CARTESIAN_POINT('Ctrl Pts',(-10.0341058688489,20.8481195408211,
4.6777656611274));
#101144=CARTESIAN_POINT('Ctrl Pts',(-10.0687287069652,20.8457006417903,
4.67625299079235));
#101145=CARTESIAN_POINT('Ctrl Pts',(-10.1696393247567,20.838505136811,4.66737384005766));
#101146=CARTESIAN_POINT('Ctrl Pts',(-10.2354242297465,20.8336219543693,
4.65590344173378));
#101147=CARTESIAN_POINT('Ctrl Pts',(-10.3594212786417,20.8242067540599,
4.62325536219842));
#101148=CARTESIAN_POINT('Ctrl Pts',(-10.4176497959986,20.8196928272384,
4.60293085007448));
#101149=CARTESIAN_POINT('Ctrl Pts',(-10.4829510851236,20.8146941652146,
4.57421988169029));
#101150=CARTESIAN_POINT('Ctrl Pts',(-10.4918268526413,20.8140162939421,
4.57018524907338));
#101151=CARTESIAN_POINT('Ctrl Pts',(-10.5040010719596,20.8130896528785,
4.56446778876622));
#101152=CARTESIAN_POINT('Ctrl Pts',(-10.5073429199312,20.8128356183889,
4.56287906950114));
#101153=CARTESIAN_POINT('Ctrl Pts',(-10.5130606598763,20.8124016146193,
4.56012773644353));
#101154=CARTESIAN_POINT('Ctrl Pts',(-10.5154401985236,20.8122211864834,
4.55897283269668));
#101155=CARTESIAN_POINT('Ctrl Pts',(-10.5204011105725,20.8118454549967,
4.55654438227177));
#101156=CARTESIAN_POINT('Ctrl Pts',(-10.5229817313711,20.8116502502629,
4.55526937626742));
#101157=CARTESIAN_POINT('Ctrl Pts',(-10.5292700937233,20.8111751273278,
4.55213375538536));
#101158=CARTESIAN_POINT('Ctrl Pts',(-10.532972776506,20.8108958312784,4.55026296332753));
#101159=CARTESIAN_POINT('Ctrl Pts',(-10.5462617468962,20.8098948278548,
4.54346029340332));
#101160=CARTESIAN_POINT('Ctrl Pts',(-10.5557904501707,20.8091796908837,
4.5384162344275));
#101161=CARTESIAN_POINT('Ctrl Pts',(-10.5794166621264,20.807409722371,4.52549119459981));
#101162=CARTESIAN_POINT('Ctrl Pts',(-10.5934241990498,20.8063632290216,
4.51744957267208));
#101163=CARTESIAN_POINT('Ctrl Pts',(-10.6541448030729,20.8018198463276,
4.48090953759299));
#101164=CARTESIAN_POINT('Ctrl Pts',(-10.6990077672982,20.7984422227704,
4.44946197147516));
#101165=CARTESIAN_POINT('Ctrl Pts',(-10.8045597075815,20.7900438619284,
4.36392233407427));
#101166=CARTESIAN_POINT('Ctrl Pts',(-10.8621398859975,20.7850266715709,
4.30646812406288));
#101167=CARTESIAN_POINT('Ctrl Pts',(-10.922852734733,20.7787546801758,4.23189081830266));
#101168=CARTESIAN_POINT('Ctrl Pts',(-10.9321248877533,20.7777654740312,
4.22004479028557));
#101169=CARTESIAN_POINT('Ctrl Pts',(-10.9451656558038,20.7763260825301,
4.20270988425559));
#101170=CARTESIAN_POINT('Ctrl Pts',(-10.9491188571776,20.7758830563697,
4.19736123367942));
#101171=CARTESIAN_POINT('Ctrl Pts',(-10.9559953557734,20.7751003641099,
4.18789059843499));
#101172=CARTESIAN_POINT('Ctrl Pts',(-10.9589378493359,20.7747614440578,
4.18378271067947));
#101173=CARTESIAN_POINT('Ctrl Pts',(-10.9649625165531,20.7740591025123,
4.1752565616609));
#101174=CARTESIAN_POINT('Ctrl Pts',(-10.9680409878828,20.7736955512168,
4.17083584171462));
#101175=CARTESIAN_POINT('Ctrl Pts',(-10.9758698911761,20.7727587913214,
4.15942733684858));
#101176=CARTESIAN_POINT('Ctrl Pts',(-10.9805755791749,20.7721839249317,
4.15240936851923));
#101177=CARTESIAN_POINT('Ctrl Pts',(-11.0003111616451,20.7697213039345,
4.12228020687205));
#101178=CARTESIAN_POINT('Ctrl Pts',(-11.0146015177673,20.7678067704228,
4.09869743298553));
#101179=CARTESIAN_POINT('Ctrl Pts',(-11.0766083272837,20.7588524920129,
3.98776450673754));
#101180=CARTESIAN_POINT('Ctrl Pts',(-11.113953782313,20.7514691005898,3.89509585705224));
#101181=CARTESIAN_POINT('Ctrl Pts',(-11.1448082671561,20.7426066374866,
3.77748418685354));
#101182=CARTESIAN_POINT('Ctrl Pts',(-11.1498136030304,20.741006287141,3.75595354011343));
#101183=CARTESIAN_POINT('Ctrl Pts',(-11.1585547229448,20.7378634298144,
3.71289184036065));
#101184=CARTESIAN_POINT('Ctrl Pts',(-11.1623033640226,20.7363210343686,
3.69137142142811));
#101185=CARTESIAN_POINT('Ctrl Pts',(-11.16624662239,20.7344257896258,3.66429942793547));
#101186=CARTESIAN_POINT('Ctrl Pts',(-11.1670033169644,20.7340455670272,
3.65883559880181));
#101187=CARTESIAN_POINT('Ctrl Pts',(-11.1681392529466,20.7334475191722,
3.65018666432755));
#101188=CARTESIAN_POINT('Ctrl Pts',(-11.1685439058007,20.733228337677,3.64700506541206));
#101189=CARTESIAN_POINT('Ctrl Pts',(-11.169243730342,20.7328379989375,3.64131712544456));
#101190=CARTESIAN_POINT('Ctrl Pts',(-11.169543841876,20.7326665746366,3.6388115016741));
#101191=CARTESIAN_POINT('Ctrl Pts',(-11.1702448973753,20.7322561709733,
3.63279469558978));
#101192=CARTESIAN_POINT('Ctrl Pts',(-11.1706380941375,20.7320176247375,
3.62928265306836));
#101193=CARTESIAN_POINT('Ctrl Pts',(-11.1717874707703,20.7312936657002,
3.61858097313007));
#101194=CARTESIAN_POINT('Ctrl Pts',(-11.1724932855425,20.7308109434326,
3.61138593125368));
#101195=CARTESIAN_POINT('Ctrl Pts',(-11.1782718619546,20.726478045031,3.54631838721667));
#101196=CARTESIAN_POINT('Ctrl Pts',(-11.1791231006365,20.7228344870486,
3.48814257594677));
#101197=CARTESIAN_POINT('Ctrl Pts',(-11.1696622566802,20.7129366109962,
3.32893834853862));
#101198=CARTESIAN_POINT('Ctrl Pts',(-11.1506102412773,20.7067634872503,
3.22895404992128));
#101199=CARTESIAN_POINT('Ctrl Pts',(-11.1147732947727,20.6992508839734,
3.11979133640583));
#101200=CARTESIAN_POINT('Ctrl Pts',(-11.1103320394087,20.6983595329181,
3.10701035095923));
#101201=CARTESIAN_POINT('Ctrl Pts',(-11.1034513351487,20.697032909787,3.08825764846938));
#101202=CARTESIAN_POINT('Ctrl Pts',(-11.1011813325995,20.6966032078948,
3.08222460216686));
#101203=CARTESIAN_POINT('Ctrl Pts',(-11.0970602809505,20.6958368028551,
3.07153894836502));
#101204=CARTESIAN_POINT('Ctrl Pts',(-11.0952288558923,20.695500758255,3.06687890296038));
#101205=CARTESIAN_POINT('Ctrl Pts',(-11.0913117058529,20.6947913610003,
3.05709547118812));
#101206=CARTESIAN_POINT('Ctrl Pts',(-11.0892194942599,20.6944177980544,
3.05197483051768));
#101207=CARTESIAN_POINT('Ctrl Pts',(-11.0835858855088,20.6934257006712,
3.0384594237697));
#101208=CARTESIAN_POINT('Ctrl Pts',(-11.0799830721792,20.6928051150741,
3.03009082743686));
#101209=CARTESIAN_POINT('Ctrl Pts',(-11.0622170021731,20.6898090897004,
2.99010769568831));
#101210=CARTESIAN_POINT('Ctrl Pts',(-11.046761923195,20.6873902331655,2.95908950041533));
#101211=CARTESIAN_POINT('Ctrl Pts',(-10.9976332173596,20.6801949214837,
2.87050268350627));
#101212=CARTESIAN_POINT('Ctrl Pts',(-10.9604146532626,20.675311897224,2.81506149664753));
#101213=CARTESIAN_POINT('Ctrl Pts',(-10.8801839534461,20.6658966448895,
2.71503961143204));
#101214=CARTESIAN_POINT('Ctrl Pts',(-10.8379440639796,20.6613825080462,
2.67009765805338));
#101215=CARTESIAN_POINT('Ctrl Pts',(-10.7851665871949,20.6563836532042,
2.62210277644192));
#101216=CARTESIAN_POINT('Ctrl Pts',(-10.777872524441,20.6557057821577,2.61563330231711));
#101217=CARTESIAN_POINT('Ctrl Pts',(-10.7677001892355,20.6547791413448,
2.6068341848783));
#101218=CARTESIAN_POINT('Ctrl Pts',(-10.7648902605897,20.6545251068836,
2.60442663949853));
#101219=CARTESIAN_POINT('Ctrl Pts',(-10.7600523560907,20.6540911031498,
2.60032090482777));
#101220=CARTESIAN_POINT('Ctrl Pts',(-10.7580299423317,20.6539106750215,
2.5986162497739));
#101221=CARTESIAN_POINT('Ctrl Pts',(-10.7537946744062,20.6535349435363,
2.59507075611822));
#101222=CARTESIAN_POINT('Ctrl Pts',(-10.7515807928218,20.6533397387963,
2.59323119832141));
#101223=CARTESIAN_POINT('Ctrl Pts',(-10.7461598347427,20.6528646158228,
2.58876031015327));
#101224=CARTESIAN_POINT('Ctrl Pts',(-10.7429455160034,20.6525853197413,
2.58613773855769));
#101225=CARTESIAN_POINT('Ctrl Pts',(-10.7313285422993,20.6515843160726,
2.57676122085405));
#101226=CARTESIAN_POINT('Ctrl Pts',(-10.722846798229,20.6508691788926,2.57010548620676));
#101227=CARTESIAN_POINT('Ctrl Pts',(-10.7014342159617,20.6490992097581,
2.55377280770514));
#101228=CARTESIAN_POINT('Ctrl Pts',(-10.6883931772399,20.6480527160031,
2.5442433642989));
#101229=CARTESIAN_POINT('Ctrl Pts',(-10.6303265089846,20.6435093304007,
2.50361782394039));
#101230=CARTESIAN_POINT('Ctrl Pts',(-10.5833583672972,20.6401317044958,
2.47541085614956));
#101231=CARTESIAN_POINT('Ctrl Pts',(-10.462299862807,20.6317333444562,2.41374176612588));
#101232=CARTESIAN_POINT('Ctrl Pts',(-10.3864012965253,20.6267161571588,
2.38448664390032));
#101233=CARTESIAN_POINT('Ctrl Pts',(-10.2935846581144,20.6204441691326,
2.35932941281007));
#101234=CARTESIAN_POINT('Ctrl Pts',(-10.2789924953926,20.6194549629014,
2.35567290780066));
#101235=CARTESIAN_POINT('Ctrl Pts',(-10.2578535063922,20.6180155712967,
2.3508042518414));
#101236=CARTESIAN_POINT('Ctrl Pts',(-10.2513597709488,20.6175725451209,
2.34936645240946));
#101237=CARTESIAN_POINT('Ctrl Pts',(-10.239911688272,20.6167898528432,2.34693322938069));
#101238=CARTESIAN_POINT('Ctrl Pts',(-10.2349624180284,20.6164509327887,
2.34591453677483));
#101239=CARTESIAN_POINT('Ctrl Pts',(-10.2247235247551,20.615748591247,2.34387569014433));
#101240=CARTESIAN_POINT('Ctrl Pts',(-10.2194331602217,20.6153850399579,
2.34285991818444));
#101241=CARTESIAN_POINT('Ctrl Pts',(-10.2058273920115,20.6144482800983,
2.34034421409722));
#101242=CARTESIAN_POINT('Ctrl Pts',(-10.1975025981861,20.6138734137381,
2.33889743161582));
#101243=CARTESIAN_POINT('Ctrl Pts',(-10.16195271686,20.6114107930482,2.33311251902508));
#101244=CARTESIAN_POINT('Ctrl Pts',(-10.1345973676973,20.6094962598224,
2.32964176231973));
#101245=CARTESIAN_POINT('Ctrl Pts',(-10.0084090380317,20.6005682353893,
2.3181138105309));
#101246=CARTESIAN_POINT('Ctrl Pts',(-9.90893778836096,20.5932142303674,
2.32159985969802));
#101247=CARTESIAN_POINT('Ctrl Pts',(-9.81110406356574,20.5859883433483,
2.33749693002615));
#101248=CARTESIAN_POINT('Ctrl Pts',(-9.81110406371067,20.4880078480432,
2.3374969300026));
#101249=CARTESIAN_POINT('Ctrl Pts',(-9.8367688653645,20.4899167657576,2.33332663844536));
#101250=CARTESIAN_POINT('Ctrl Pts',(-9.8625792519295,20.4918241056207,2.33000503893528));
#101251=CARTESIAN_POINT('Ctrl Pts',(-9.91463091193593,20.4956255539049,
2.32505466557443));
#101252=CARTESIAN_POINT('Ctrl Pts',(-9.94084622985053,20.4975173421905,
2.32344339867565));
#101253=CARTESIAN_POINT('Ctrl Pts',(-9.97735538488933,20.5001029330583,
2.32242297945779));
#101254=CARTESIAN_POINT('Ctrl Pts',(-9.98761936861823,20.500824430773,2.32227033911966));
#101255=CARTESIAN_POINT('Ctrl Pts',(-10.0055186560579,20.502071795745,2.32223818678792));
#101256=CARTESIAN_POINT('Ctrl Pts',(-10.0131530979203,20.5026003824754,
2.32229870173733));
#101257=CARTESIAN_POINT('Ctrl Pts',(-10.0243980035323,20.5033733614566,
2.32249719924083));
#101258=CARTESIAN_POINT('Ctrl Pts',(-10.0280090966784,20.5036207404338,
2.32257756104498));
#101259=CARTESIAN_POINT('Ctrl Pts',(-10.0344146930225,20.504057984682,2.32274959828643));
#101260=CARTESIAN_POINT('Ctrl Pts',(-10.0372092988945,20.5042482088913,
2.32283461310697));
#101261=CARTESIAN_POINT('Ctrl Pts',(-10.0432576214514,20.5046587396627,
2.32304017013204));
#101262=CARTESIAN_POINT('Ctrl Pts',(-10.0465111511223,20.5048788495448,
2.32316425257967));
#101263=CARTESIAN_POINT('Ctrl Pts',(-10.0554902725033,20.5054844157735,
2.32354399189579));
#101264=CARTESIAN_POINT('Ctrl Pts',(-10.0612146713599,20.5058683507546,
2.32382795617791));
#101265=CARTESIAN_POINT('Ctrl Pts',(-10.0915815731029,20.5078948468639,
2.32555664015501));
#101266=CARTESIAN_POINT('Ctrl Pts',(-10.1161781609322,20.5095006017224,
2.32773414647287));
#101267=CARTESIAN_POINT('Ctrl Pts',(-10.2427526680802,20.5176627460296,
2.34296336822354));
#101268=CARTESIAN_POINT('Ctrl Pts',(-10.3427737739851,20.523808994165,2.36855297663871));
#101269=CARTESIAN_POINT('Ctrl Pts',(-10.476228585395,20.5328926521535,2.42204859696507));
#101270=CARTESIAN_POINT('Ctrl Pts',(-10.5134243088481,20.5355240344521,
2.43926072632925));
#101271=CARTESIAN_POINT('Ctrl Pts',(-10.5581138524258,20.5388530341706,
2.46284250135655));
#101272=CARTESIAN_POINT('Ctrl Pts',(-10.5665274360215,20.5394873217159,
2.46741421443008));
#101273=CARTESIAN_POINT('Ctrl Pts',(-10.5797996117623,20.5405004218694,
2.47483699243526));
#101274=CARTESIAN_POINT('Ctrl Pts',(-10.5846952270175,20.5408768644156,
2.47762126806619));
#101275=CARTESIAN_POINT('Ctrl Pts',(-10.5938869645842,20.5415889495649,
2.482936483509));
#101276=CARTESIAN_POINT('Ctrl Pts',(-10.5981873644444,20.5419243135208,
2.48545980908448));
#101277=CARTESIAN_POINT('Ctrl Pts',(-10.6078570255081,20.5426834763975,
2.49121648420734));
#101278=CARTESIAN_POINT('Ctrl Pts',(-10.6132167239919,20.5431078357741,
2.49446551925175));
#101279=CARTESIAN_POINT('Ctrl Pts',(-10.6269251041777,20.5442025687766,
2.50292586431846));
#101280=CARTESIAN_POINT('Ctrl Pts',(-10.635234717728,20.5448751888077,2.50819923298898));
#101281=CARTESIAN_POINT('Ctrl Pts',(-10.6966403883498,20.5499145881241,
2.54825618553653));
#101282=CARTESIAN_POINT('Ctrl Pts',(-10.7469040976486,20.5544362763313,
2.5871714491312));
#101283=CARTESIAN_POINT('Ctrl Pts',(-10.8487600637358,20.5644684224261,
2.68009765299182));
#101284=CARTESIAN_POINT('Ctrl Pts',(-10.8988590583217,20.5699952926391,
2.73535251369354));
#101285=CARTESIAN_POINT('Ctrl Pts',(-10.9602686012246,20.5773841979994,
2.81752474544325));
#101286=CARTESIAN_POINT('Ctrl Pts',(-10.9763152413395,20.5793849670838,
2.84068436430025));
#101287=CARTESIAN_POINT('Ctrl Pts',(-10.9946228561666,20.581736382843,2.8692436683158));
#101288=CARTESIAN_POINT('Ctrl Pts',(-10.9976929049926,20.5821332047154,
2.87411099491157));
#101289=CARTESIAN_POINT('Ctrl Pts',(-11.0024285983117,20.5827490446988,
2.88174246512797));
#101290=CARTESIAN_POINT('Ctrl Pts',(-11.0041187149545,20.5829695900886,
2.88449120148253));
#101291=CARTESIAN_POINT('Ctrl Pts',(-11.0072544171624,20.5833801485293,
2.88963826890152));
#101292=CARTESIAN_POINT('Ctrl Pts',(-11.0087027355991,20.5835703299706,
2.89203479120434));
#101293=CARTESIAN_POINT('Ctrl Pts',(-11.0119910985509,20.584003429901,2.89752012098032));
#101294=CARTESIAN_POINT('Ctrl Pts',(-11.0138255580918,20.5842459889622,
2.90061220667193));
#101295=CARTESIAN_POINT('Ctrl Pts',(-11.0186678149814,20.5848889264806,
2.9088599391441));
#101296=CARTESIAN_POINT('Ctrl Pts',(-11.0216506750877,20.5852877743589,
2.91403021358801));
#101297=CARTESIAN_POINT('Ctrl Pts',(-11.0451027827353,20.5884480326347,
2.95540391806346));
#101298=CARTESIAN_POINT('Ctrl Pts',(-11.0636830910198,20.5911028574166,
2.9926501902343));
#101299=CARTESIAN_POINT('Ctrl Pts',(-11.1195236602504,20.5999001260097,
3.12121543004571));
#101300=CARTESIAN_POINT('Ctrl Pts',(-11.1472862253339,20.6058368508171,
3.2161939511381));
#101301=CARTESIAN_POINT('Ctrl Pts',(-11.1674551277628,20.6139886567099,
3.34196957809833));
#101302=CARTESIAN_POINT('Ctrl Pts',(-11.1709710869934,20.6158580953257,
3.37057207799114));
#101303=CARTESIAN_POINT('Ctrl Pts',(-11.1741682671452,20.6183264736807,
3.40781811257545));
#101304=CARTESIAN_POINT('Ctrl Pts',(-11.1748083983981,20.6188955664282,
3.41637081531469));
#101305=CARTESIAN_POINT('Ctrl Pts',(-11.1757001041675,20.6198285984352,
3.43033198180438));
#101306=CARTESIAN_POINT('Ctrl Pts',(-11.176007902314,20.620190785339,3.43573663774638));
#101307=CARTESIAN_POINT('Ctrl Pts',(-11.176530298103,20.6208924292544,3.44617693267445));
#101308=CARTESIAN_POINT('Ctrl Pts',(-11.1767498525556,20.6212317243772,
3.45121221382854));
#101309=CARTESIAN_POINT('Ctrl Pts',(-11.1771814960005,20.6220162878001,
3.46282368527109));
#101310=CARTESIAN_POINT('Ctrl Pts',(-11.1773708084431,20.6224622528056,
3.46940050205389));
#101311=CARTESIAN_POINT('Ctrl Pts',(-11.1778037200537,20.6239065026286,
3.49062125976624));
#101312=CARTESIAN_POINT('Ctrl Pts',(-11.1778292663653,20.6249114779892,
3.50526776684372));
#101313=CARTESIAN_POINT('Ctrl Pts',(-11.1760585623524,20.6321588531749,
3.60999444967978));
#101314=CARTESIAN_POINT('Ctrl Pts',(-11.164203775215,20.6387190329531,3.69958965366465));
#101315=CARTESIAN_POINT('Ctrl Pts',(-11.1257664630346,20.6503042282052,
3.85260280017017));
#101316=CARTESIAN_POINT('Ctrl Pts',(-11.1036382937098,20.655274555616,3.91672946722192));
#101317=CARTESIAN_POINT('Ctrl Pts',(-11.0731897566169,20.6604902367094,
3.98519148125711));
#101318=CARTESIAN_POINT('Ctrl Pts',(-11.0701998569949,20.6609889377655,
3.99175125805172));
#101319=CARTESIAN_POINT('Ctrl Pts',(-11.065656714068,20.6617266357524,4.0014810914199));
#101320=CARTESIAN_POINT('Ctrl Pts',(-11.0641492149745,20.6619682511247,
4.00467213751262));
#101321=CARTESIAN_POINT('Ctrl Pts',(-11.0615397501101,20.6623810463519,
4.01013212329531));
#101322=CARTESIAN_POINT('Ctrl Pts',(-11.060444817488,20.6625526482349,4.01240434598668));
#101323=CARTESIAN_POINT('Ctrl Pts',(-11.0579404988381,20.662941497775,4.01755894085841));
#101324=CARTESIAN_POINT('Ctrl Pts',(-11.056526629411,20.6631584662363,4.02043908222931));
#101325=CARTESIAN_POINT('Ctrl Pts',(-11.0526464772791,20.663747077036,4.028262218281));
#101326=CARTESIAN_POINT('Ctrl Pts',(-11.0501571214138,20.6641173336036,
4.03319377407471));
#101327=CARTESIAN_POINT('Ctrl Pts',(-11.0376036523578,20.6659492322764,
4.05763391574211));
#101328=CARTESIAN_POINT('Ctrl Pts',(-11.0270294717712,20.6673819374167,
4.07687740211616));
#101329=CARTESIAN_POINT('Ctrl Pts',(-11.004762407217,20.6702118242537,4.11484489007165));
#101330=CARTESIAN_POINT('Ctrl Pts',(-10.9930690558708,20.6716082293708,
4.13355795401394));
#101331=CARTESIAN_POINT('Ctrl Pts',(-10.9257473074405,20.6792371285798,
4.23484601747686));
#101332=CARTESIAN_POINT('Ctrl Pts',(-10.8603502715243,20.685233345798,4.31043484337156));
#101333=CARTESIAN_POINT('Ctrl Pts',(-10.7657791081188,20.6933750035747,
4.39522697423042));
#101334=CARTESIAN_POINT('Ctrl Pts',(-10.7447022177137,20.6951587683679,
4.41283481310521));
#101335=CARTESIAN_POINT('Ctrl Pts',(-10.7163714195351,20.6975293550459,
4.43486802143705));
#101336=CARTESIAN_POINT('Ctrl Pts',(-10.7096569472813,20.6980892623452,
4.4399751269331));
#101337=CARTESIAN_POINT('Ctrl Pts',(-10.6985692081646,20.6990110378513,
4.4482220726343));
#101338=CARTESIAN_POINT('Ctrl Pts',(-10.6942281723531,20.6993712347896,
4.4514048984));
#101339=CARTESIAN_POINT('Ctrl Pts',(-10.6857707134083,20.7000717390455,
4.45751716247405));
#101340=CARTESIAN_POINT('Ctrl Pts',(-10.6816569519441,20.7004119023647,
4.46045009568194));
#101341=CARTESIAN_POINT('Ctrl Pts',(-10.6720813548095,20.70120246812,4.46718457263074));
#101342=CARTESIAN_POINT('Ctrl Pts',(-10.666605960808,20.7016536014184,4.47096644374171));
#101343=CARTESIAN_POINT('Ctrl Pts',(-10.6486267859144,20.7031321810286,
4.4831609577789));
#101344=CARTESIAN_POINT('Ctrl Pts',(-10.6359939781741,20.7041667705274,
4.49137974528929));
#101345=CARTESIAN_POINT('Ctrl Pts',(-10.5554821045012,20.7107366545475,
4.54158780089417));
#101346=CARTESIAN_POINT('Ctrl Pts',(-10.4836511126367,20.7165144601256,
4.57682068307146));
#101347=CARTESIAN_POINT('Ctrl Pts',(-10.3420275033499,20.7275946246151,
4.62924105330901));
#101348=CARTESIAN_POINT('Ctrl Pts',(-10.2731202322393,20.7328535035932,
4.647856772218));
#101349=CARTESIAN_POINT('Ctrl Pts',(-10.191628991443,20.7386693490162,4.66211249168484));
#101350=CARTESIAN_POINT('Ctrl Pts',(-10.1802806184288,20.7394701285077,
4.66392698962636));
#101351=CARTESIAN_POINT('Ctrl Pts',(-10.1646987256062,20.7405555494079,
4.6661850083173));
#101352=CARTESIAN_POINT('Ctrl Pts',(-10.1604871120029,20.7408475213601,
4.66677205663001));
#101353=CARTESIAN_POINT('Ctrl Pts',(-10.1533997190042,20.7413363935927,
4.66772085212518));
#101354=CARTESIAN_POINT('Ctrl Pts',(-10.1505256469116,20.7415339601047,
4.66809481315633));
#101355=CARTESIAN_POINT('Ctrl Pts',(-10.1450486253927,20.7419091240841,
4.66878690738286));
#101356=CARTESIAN_POINT('Ctrl Pts',(-10.142445958736,20.74208683103,4.66910696165161));
#101357=CARTESIAN_POINT('Ctrl Pts',(-10.1362525066815,20.7425084036835,
4.66984759143203));
#101358=CARTESIAN_POINT('Ctrl Pts',(-10.1326607842979,20.7427518377742,
4.67026033425424));
#101359=CARTESIAN_POINT('Ctrl Pts',(-10.1199335018557,20.7436109287352,
4.6716635418858));
#101360=CARTESIAN_POINT('Ctrl Pts',(-10.1107880236469,20.7442218336206,
4.67256365580787));
#101361=CARTESIAN_POINT('Ctrl Pts',(-10.0230935293739,20.7500263970944,
4.68015948742423));
#101362=CARTESIAN_POINT('Ctrl Pts',(-9.94405766944615,20.7548575072673,
4.67906060174838));
#101363=CARTESIAN_POINT('Ctrl Pts',(-9.7854191155167,20.7647309284812,4.66085420586738));
#101364=CARTESIAN_POINT('Ctrl Pts',(-9.7062965599428,20.7697563286272,4.64339986845356));
#101365=CARTESIAN_POINT('Ctrl Pts',(-9.6187844980767,20.7758078957804,4.6144053852409));
#101366=CARTESIAN_POINT('Ctrl Pts',(-9.60803248210983,20.7765598602351,
4.6106691999123));
#101367=CARTESIAN_POINT('Ctrl Pts',(-9.59168132916687,20.7777171826537,
4.60472039038266));
#101368=CARTESIAN_POINT('Ctrl Pts',(-9.586041995808,20.7781188601552,4.6026196290512));
#101369=CARTESIAN_POINT('Ctrl Pts',(-9.57622719731688,20.778822487287,4.5988775184938));
#101370=CARTESIAN_POINT('Ctrl Pts',(-9.57204451424204,20.7791237953439,
4.59725534411934));
#101371=CARTESIAN_POINT('Ctrl Pts',(-9.56262378810786,20.7798057694444,
4.5935396340685));
#101372=CARTESIAN_POINT('Ctrl Pts',(-9.55739134348373,20.7801868902638,
4.59143229623557));
#101373=CARTESIAN_POINT('Ctrl Pts',(-9.54328057766385,20.7812211479528,
4.58563110652246));
#101374=CARTESIAN_POINT('Ctrl Pts',(-9.53443218967265,20.781876658423,4.5818660428249));
#101375=CARTESIAN_POINT('Ctrl Pts',(-9.49238672129402,20.7850256794751,
4.56336401268124));
#101376=CARTESIAN_POINT('Ctrl Pts',(-9.45984029088913,20.787566807976,4.54720640821779));
#101377=CARTESIAN_POINT('Ctrl Pts',(-9.35910668954076,20.7957715993893,
4.491251108654));
#101378=CARTESIAN_POINT('Ctrl Pts',(-9.29415054255041,20.8015963585646,
4.44609562928631));
#101379=CARTESIAN_POINT('Ctrl Pts',(-9.19828206009965,20.8108344645681,
4.36404812852664));
#101380=CARTESIAN_POINT('Ctrl Pts',(-9.16423835392765,20.8142659561741,
4.33116439182139));
#101381=CARTESIAN_POINT('Ctrl Pts',(-9.12581283732179,20.8182446058098,
4.28929260992186));
#101382=CARTESIAN_POINT('Ctrl Pts',(-9.11944976186729,20.8189071842837,
4.28218751727656));
#101383=CARTESIAN_POINT('Ctrl Pts',(-9.11057362648706,20.8198358394714,
4.27203069752461));
#101384=CARTESIAN_POINT('Ctrl Pts',(-9.10798874194613,20.8201068203273,
4.26904264411427));
#101385=CARTESIAN_POINT('Ctrl Pts',(-9.10357062155876,20.8205708345567,
4.26388317615764));
#101386=CARTESIAN_POINT('Ctrl Pts',(-9.10173013264509,20.8207643883875,
4.26171804722446));
#101387=CARTESIAN_POINT('Ctrl Pts',(-9.09791276827517,20.8211663444236,
4.25719426800012));
#101388=CARTESIAN_POINT('Ctrl Pts',(-9.09593728488424,20.8213746483992,
4.25483451220988));
#101389=CARTESIAN_POINT('Ctrl Pts',(-9.09072759071522,20.8219248436071,
4.24856163416063));
#101390=CARTESIAN_POINT('Ctrl Pts',(-9.087509347654,20.8222656106025,4.24463524368693));
#101391=CARTESIAN_POINT('Ctrl Pts',(-9.07379722871105,20.8237219905988,
4.22768349145525));
#101392=CARTESIAN_POINT('Ctrl Pts',(-9.06355550127781,20.824821138523,4.21445546284441));
#101393=CARTESIAN_POINT('Ctrl Pts',(-8.98746808428698,20.8331147779856,
4.11173374650378));
#101394=CARTESIAN_POINT('Ctrl Pts',(-8.93429645710424,20.8397177421073,
4.01353798502857));
#101395=CARTESIAN_POINT('Ctrl Pts',(-8.88111974510063,20.8493760551488,
3.87007450989365));
#101396=CARTESIAN_POINT('Ctrl Pts',(-8.86867289843669,20.8520638670126,
3.83007053489452));
#101397=CARTESIAN_POINT('Ctrl Pts',(-8.85601480671824,20.8554561853596,
3.78015310424117));
#101398=CARTESIAN_POINT('Ctrl Pts',(-8.85376140333662,20.8560943262768,
3.77078580960637));
#101399=CARTESIAN_POINT('Ctrl Pts',(-8.85037039066297,20.8571121610184,
3.75588803929416));
#101400=CARTESIAN_POINT('Ctrl Pts',(-8.84915715843412,20.8574894459042,
3.75037507753535));
#101401=CARTESIAN_POINT('Ctrl Pts',(-8.84694740443567,20.8582022412135,
3.73997836747467));
#101402=CARTESIAN_POINT('Ctrl Pts',(-8.84594215928674,20.8585374665223,
3.73509658433723));
#101403=CARTESIAN_POINT('Ctrl Pts',(-8.84374674489691,20.8592951266807,
3.72408147173955));
#101404=CARTESIAN_POINT('Ctrl Pts',(-8.84257433982359,20.8597181129003,
3.71794479683222));
#101405=CARTESIAN_POINT('Ctrl Pts',(-8.83969283270423,20.8608069433553,
3.7021828492199));
#101406=CARTESIAN_POINT('Ctrl Pts',(-8.83805467422681,20.8614749933599,
3.69254525928092));
#101407=CARTESIAN_POINT('Ctrl Pts',(-8.82719874844838,20.8662795359316,
3.62348426713597));
#101408=CARTESIAN_POINT('Ctrl Pts',(-8.82242551438339,20.8705542842563,
3.56346170745649));
#101409=CARTESIAN_POINT('Ctrl Pts',(-8.82203501085231,20.8805375701437,
3.42598683872903));
#101410=CARTESIAN_POINT('Ctrl Pts',(-8.82943731780189,20.8862874589667,
3.34879781870742));
#101411=CARTESIAN_POINT('Ctrl Pts',(-8.84987800239737,20.8939265285851,
3.24478425553931));
#101412=CARTESIAN_POINT('Ctrl Pts',(-8.85642619911104,20.8959625499864,
3.21688348762403));
#101413=CARTESIAN_POINT('Ctrl Pts',(-8.86551145253675,20.8983494830781,
3.18367071219165));
#101414=CARTESIAN_POINT('Ctrl Pts',(-8.86707786727827,20.8987481641312,
3.1781057203367));
#101415=CARTESIAN_POINT('Ctrl Pts',(-8.86958395688524,20.8993662484761,
3.1694473099146));
#101416=CARTESIAN_POINT('Ctrl Pts',(-8.87049547170255,20.8995871966833,
3.16634593866105));
#101417=CARTESIAN_POINT('Ctrl Pts',(-8.87222015067925,20.8999980980351,
3.16056589749218));
#101418=CARTESIAN_POINT('Ctrl Pts',(-8.87303008972077,20.9001882225889,
3.15788639308306));
#101419=CARTESIAN_POINT('Ctrl Pts',(-8.87489957134157,20.9006206850331,
3.15178031192174));
#101420=CARTESIAN_POINT('Ctrl Pts',(-8.87596521854471,20.9008626675028,
3.14835566737631));
#101421=CARTESIAN_POINT('Ctrl Pts',(-8.87883698777103,20.9015030515399,
3.13927318576526));
#101422=CARTESIAN_POINT('Ctrl Pts',(-8.880670317713,20.9018999417412,3.13362396303219));
#101423=CARTESIAN_POINT('Ctrl Pts',(-8.89541671779103,20.9050025287569,
3.08932848361827));
#101424=CARTESIAN_POINT('Ctrl Pts',(-8.91028628324103,20.9076059251985,
3.05135746611207));
#101425=CARTESIAN_POINT('Ctrl Pts',(-8.96727488464075,20.9162844605701,
2.92548874689851));
#101426=CARTESIAN_POINT('Ctrl Pts',(-9.01830618231569,20.9221514653709,
2.84207728254627));
#101427=CARTESIAN_POINT('Ctrl Pts',(-9.09805110011913,20.9303225203821,
2.74203243946404));
#101428=CARTESIAN_POINT('Ctrl Pts',(-9.1179946762363,20.9323001187201,2.71891550015676));
#101429=CARTESIAN_POINT('Ctrl Pts',(-9.14477734480224,20.9348915715385,
2.69020635858557));
#101430=CARTESIAN_POINT('Ctrl Pts',(-9.15081338828464,20.9354716447545,
2.68387891628739));
#101431=CARTESIAN_POINT('Ctrl Pts',(-9.16072482523161,20.936418146161,2.67371799768141));
#101432=CARTESIAN_POINT('Ctrl Pts',(-9.16455743023023,20.9367827231718,
2.66984310082046));
#101433=CARTESIAN_POINT('Ctrl Pts',(-9.17197673779533,20.9374858618342,
2.66244533703686));
#101434=CARTESIAN_POINT('Ctrl Pts',(-9.17555938063965,20.9378242407662,
2.65891855328911));
#101435=CARTESIAN_POINT('Ctrl Pts',(-9.18382319967626,20.9386022005231,
2.65088711138032));
#101436=CARTESIAN_POINT('Ctrl Pts',(-9.18851925316926,20.9390424404358,
2.646398066081));
#101437=CARTESIAN_POINT('Ctrl Pts',(-9.20358649965861,20.9404492939567,
2.63223170829749));
#101438=CARTESIAN_POINT('Ctrl Pts',(-9.21409515549528,20.9414221224794,
2.62270311958018));
#101439=CARTESIAN_POINT('Ctrl Pts',(-9.29675864365264,20.9490140239718,
2.55042634696519));
#101440=CARTESIAN_POINT('Ctrl Pts',(-9.376128382834,20.955996950912,2.49649835125264));
#101441=CARTESIAN_POINT('Ctrl Pts',(-9.51683441024283,20.9676140339523,
2.42409476199778));
#101442=CARTESIAN_POINT('Ctrl Pts',(-9.57475449239545,20.9721985892043,
2.3999140255961));
#101443=CARTESIAN_POINT('Ctrl Pts',(-9.64131736904383,20.9770747493859,
2.3781729762258));
#101444=CARTESIAN_POINT('Ctrl Pts',(-9.64832660261297,20.9775834490114,
2.37595599308374));
#101445=CARTESIAN_POINT('Ctrl Pts',(-9.65875777723135,20.9783329743605,
2.37276379534378));
#101446=CARTESIAN_POINT('Ctrl Pts',(-9.66216395478507,20.9785765393113,
2.37173827367811));
#101447=CARTESIAN_POINT('Ctrl Pts',(-9.66825137869082,20.9790096576048,
2.36993552961538));
#101448=CARTESIAN_POINT('Ctrl Pts',(-9.67093078760381,20.9791995436096,
2.36915239356958));
#101449=CARTESIAN_POINT('Ctrl Pts',(-9.67677934710888,20.9796123760741,
2.36746552745444));
#101450=CARTESIAN_POINT('Ctrl Pts',(-9.67994951510487,20.9798351056841,
2.36656556883547));
#101451=CARTESIAN_POINT('Ctrl Pts',(-9.68881119841782,20.9804549091218,
2.36409002684421));
#101452=CARTESIAN_POINT('Ctrl Pts',(-9.69451094658588,20.9808503433781,
2.36254390010009));
#101453=CARTESIAN_POINT('Ctrl Pts',(-9.72669115817815,20.9830660952592,
2.35407396458365));
#101454=CARTESIAN_POINT('Ctrl Pts',(-9.75339736526943,20.984840961702,2.34803141727121));
#101455=CARTESIAN_POINT('Ctrl Pts',(-9.79053812481558,20.9872520692737,
2.34097905577803));
#101456=CARTESIAN_POINT('Ctrl Pts',(-9.8008096501287,20.9879128975803,2.33916967646004));
#101457=CARTESIAN_POINT('Ctrl Pts',(-9.81110406371161,20.988570409963,2.33749693000245));
#101458=CARTESIAN_POINT('Origin',(-10.,12.3756328852638,3.5));
#101459=CARTESIAN_POINT('',(-9.81110406371042,21.5864520766487,2.33749693000264));
#101460=CARTESIAN_POINT('',(-9.8111040680739,21.4868028556135,2.33749692929362));
#101461=CARTESIAN_POINT('',(-9.81110406371068,12.3756328852638,2.3374969300026));
#101462=CARTESIAN_POINT('Ctrl Pts',(-9.81110406371016,21.5864520766487,
2.33749693000268));
#101463=CARTESIAN_POINT('Ctrl Pts',(-9.81060766089596,21.5864209889335,
2.33757759084289));
#101464=CARTESIAN_POINT('Ctrl Pts',(-9.81011130921745,21.5863899011916,
2.33765856972403));
#101465=CARTESIAN_POINT('Ctrl Pts',(-9.72529092088347,21.5810768181492,
2.35155264421486));
#101466=CARTESIAN_POINT('Ctrl Pts',(-9.64273262524373,21.5757844251671,
2.37449841993186));
#101467=CARTESIAN_POINT('Ctrl Pts',(-9.55279108763647,21.5694278398515,
2.41039941934661));
#101468=CARTESIAN_POINT('Ctrl Pts',(-9.54225700543766,21.5686741209824,
2.41478270717911));
#101469=CARTESIAN_POINT('Ctrl Pts',(-9.52626035112546,21.567514573904,2.42171334733196));
#101470=CARTESIAN_POINT('Ctrl Pts',(-9.52075069016363,21.567112447069,2.424150820525));
#101471=CARTESIAN_POINT('Ctrl Pts',(-9.51116959311343,21.5664082378757,
2.4284776996498));
#101472=CARTESIAN_POINT('Ctrl Pts',(-9.50708976996682,21.5661067996405,
2.43034832257606));
#101473=CARTESIAN_POINT('Ctrl Pts',(-9.49790811575377,21.5654248026092,
2.4346218490978));
#101474=CARTESIAN_POINT('Ctrl Pts',(-9.49281268076681,21.5650437904338,
2.4370381540536));
#101475=CARTESIAN_POINT('Ctrl Pts',(-9.47908744396125,21.5640105046256,
2.44366795134327));
#101476=CARTESIAN_POINT('Ctrl Pts',(-9.47049166045894,21.5633558662003,
2.4479504779268));
#101477=CARTESIAN_POINT('Ctrl Pts',(-9.42981017407345,21.560220877665,2.46884336836683));
#101478=CARTESIAN_POINT('Ctrl Pts',(-9.39845078724527,21.557693438203,2.48681763870582));
#101479=CARTESIAN_POINT('Ctrl Pts',(-9.29254781678088,21.5487588127927,
2.55416930938222));
#101480=CARTESIAN_POINT('Ctrl Pts',(-9.22283677679343,21.5421268174682,
2.6105630143172));
#101481=CARTESIAN_POINT('Ctrl Pts',(-9.13077231293729,21.5325595642172,
2.7041996059016));
#101482=CARTESIAN_POINT('Ctrl Pts',(-9.1029756882655,21.5295418364413,2.73566810806177));
#101483=CARTESIAN_POINT('Ctrl Pts',(-9.07299056895803,21.5261894181262,
2.77350945504996));
#101484=CARTESIAN_POINT('Ctrl Pts',(-9.06910572105483,21.5257530613272,
2.77849404505435));
#101485=CARTESIAN_POINT('Ctrl Pts',(-9.06322409983174,21.5250896032388,
2.78616725579008));
#101486=CARTESIAN_POINT('Ctrl Pts',(-9.06119843339019,21.5248605817397,
2.78883342803537));
#101487=CARTESIAN_POINT('Ctrl Pts',(-9.05750642348659,21.5244422556921,
2.79373609835053));
#101488=CARTESIAN_POINT('Ctrl Pts',(-9.0558366527482,21.524252721047,2.79596987664177));
#101489=CARTESIAN_POINT('Ctrl Pts',(-9.05209267020263,21.5238269598399,
2.80101576120915));
#101490=CARTESIAN_POINT('Ctrl Pts',(-9.05002303005636,21.5235910468645,
2.80383117756344));
#101491=CARTESIAN_POINT('Ctrl Pts',(-9.04472757167543,21.5229858717687,
2.81110239570888));
#101492=CARTESIAN_POINT('Ctrl Pts',(-9.04152034091558,21.5226178329765,
2.81557172213832));
#101493=CARTESIAN_POINT('Ctrl Pts',(-9.021313262602,21.5202881579029,2.84415122569372));
#101494=CARTESIAN_POINT('Ctrl Pts',(-9.0051914315643,21.5183798443153,2.86887276120704));
#101495=CARTESIAN_POINT('Ctrl Pts',(-8.9395345757537,21.5102622948452,2.97833115784914));
#101496=CARTESIAN_POINT('Ctrl Pts',(-8.89976923487954,21.5043752016211,
3.0684678189506));
#101497=CARTESIAN_POINT('Ctrl Pts',(-8.86008415261758,21.4956207998367,
3.20114524339427));
#101498=CARTESIAN_POINT('Ctrl Pts',(-8.85051866639125,21.4930281097516,
3.24035711906565));
#101499=CARTESIAN_POINT('Ctrl Pts',(-8.84120256186922,21.4897424105239,
3.28934745860847));
#101500=CARTESIAN_POINT('Ctrl Pts',(-8.83953500549171,21.4891106940761,
3.29873653211263));
#101501=CARTESIAN_POINT('Ctrl Pts',(-8.8370654379355,21.4881006724145,3.31369406097109));
#101502=CARTESIAN_POINT('Ctrl Pts',(-8.83618897134081,21.4877247109436,
3.31924993424982));
#101503=CARTESIAN_POINT('Ctrl Pts',(-8.83461021506429,21.4870128896893,
3.32974547392619));
#101504=CARTESIAN_POINT('Ctrl Pts',(-8.8338994501011,21.4866773040379,3.33468375552347));
#101505=CARTESIAN_POINT('Ctrl Pts',(-8.83236433442107,21.4859167618943,
3.34585231103746));
#101506=CARTESIAN_POINT('Ctrl Pts',(-8.83155843726905,21.4854912378293,
3.35208492514912));
#101507=CARTESIAN_POINT('Ctrl Pts',(-8.82961230260852,21.484391740244,3.36814557904493));
#101508=CARTESIAN_POINT('Ctrl Pts',(-8.82854597816542,21.4837154883602,
3.37798190768718));
#101509=CARTESIAN_POINT('Ctrl Pts',(-8.82043654673883,21.4778622293617,
3.46274154140933));
#101510=CARTESIAN_POINT('Ctrl Pts',(-8.82046679861231,21.4724628834874,
3.53815303662331));
#101511=CARTESIAN_POINT('Ctrl Pts',(-8.83290441303645,21.4629824137846,
3.66714860287829));
#101512=CARTESIAN_POINT('Ctrl Pts',(-8.84186292123912,21.4589667569451,
3.72083792206369));
#101513=CARTESIAN_POINT('Ctrl Pts',(-8.86279869579375,21.4524326404411,
3.80845393113823));
#101514=CARTESIAN_POINT('Ctrl Pts',(-8.87267588599687,21.4498774591765,
3.84279954364262));
#101515=CARTESIAN_POINT('Ctrl Pts',(-8.88605380159144,21.4469746775545,
3.88243463509204));
#101516=CARTESIAN_POINT('Ctrl Pts',(-8.8880525474143,21.4465530461188,3.88820774050974));
#101517=CARTESIAN_POINT('Ctrl Pts',(-8.89120131201368,21.445907267494,3.89707864075277));
#101518=CARTESIAN_POINT('Ctrl Pts',(-8.89231955928833,21.4456813510246,
3.9001874802726));
#101519=CARTESIAN_POINT('Ctrl Pts',(-8.89440689617213,21.4452659496934,
3.90591470257956));
#101520=CARTESIAN_POINT('Ctrl Pts',(-8.89537221088707,21.4450762572026,
3.90853433738499));
#101521=CARTESIAN_POINT('Ctrl Pts',(-8.89758580801163,21.4446466792264,
3.91447630458804));
#101522=CARTESIAN_POINT('Ctrl Pts',(-8.89883979767756,21.4444071333578,
3.91779644255815));
#101523=CARTESIAN_POINT('Ctrl Pts',(-8.9021404518251,21.4437862783744,3.92641735530025));
#101524=CARTESIAN_POINT('Ctrl Pts',(-8.90421053184145,21.4434063010936,
3.93170915333724));
#101525=CARTESIAN_POINT('Ctrl Pts',(-8.91863544540237,21.4408203143358,
3.96781159030337));
#101526=CARTESIAN_POINT('Ctrl Pts',(-8.93225107484958,21.4386819589838,
3.99810608855455));
#101527=CARTESIAN_POINT('Ctrl Pts',(-8.9817222821857,21.4316931874244,4.09679491866861));
#101528=CARTESIAN_POINT('Ctrl Pts',(-9.02301624192878,21.427010037129,4.16223686438359));
#101529=CARTESIAN_POINT('Ctrl Pts',(-9.10165924243954,21.4190121596264,
4.26332656869609));
#101530=CARTESIAN_POINT('Ctrl Pts',(-9.13546501107661,21.4157866785003,
4.30141244229991));
#101531=CARTESIAN_POINT('Ctrl Pts',(-9.18106887098913,21.4115900099408,
4.3465361201954));
#101532=CARTESIAN_POINT('Ctrl Pts',(-9.19067065934757,21.4107144363865,
4.35572051037113));
#101533=CARTESIAN_POINT('Ctrl Pts',(-9.20512417298615,21.4094068662907,
4.36908482657173));
#101534=CARTESIAN_POINT('Ctrl Pts',(-9.20985813780862,21.4089802072176,
4.37339100695769));
#101535=CARTESIAN_POINT('Ctrl Pts',(-9.21835397157798,21.4082172066396,
4.38099350928657));
#101536=CARTESIAN_POINT('Ctrl Pts',(-9.22210221612152,21.4078815023235,
4.38430487597133));
#101537=CARTESIAN_POINT('Ctrl Pts',(-9.23005910452318,21.4071707219209,
4.39124461112308));
#101538=CARTESIAN_POINT('Ctrl Pts',(-9.2342725519246,21.4067954223185,4.39486725963459));
#101539=CARTESIAN_POINT('Ctrl Pts',(-9.24554928228974,21.4057937413676,
4.40442483890571));
#101540=CARTESIAN_POINT('Ctrl Pts',(-9.2526568288875,21.4051652361289,4.41030673472405));
#101541=CARTESIAN_POINT('Ctrl Pts',(-9.28788994388713,21.402062738911,4.43877336380849));
#101542=CARTESIAN_POINT('Ctrl Pts',(-9.31697099058934,21.3995414810387,
4.46013907845837));
#101543=CARTESIAN_POINT('Ctrl Pts',(-9.40679276896362,21.3918633201409,
4.51998293881145));
#101544=CARTESIAN_POINT('Ctrl Pts',(-9.47011789267306,21.3865802960843,
4.55426885899629));
#101545=CARTESIAN_POINT('Ctrl Pts',(-9.53861643345747,21.3811126577436,
4.58361773137528));
#101546=CARTESIAN_POINT('Ctrl Pts',(-9.54107281093733,21.3809169202154,
4.58466032397677));
#101547=CARTESIAN_POINT('Ctrl Pts',(-9.59590647481775,21.3765551259045,
4.60771448176959));
#101548=CARTESIAN_POINT('Ctrl Pts',(-9.6498116723613,21.3724186632665,4.62591858503384));
#101549=CARTESIAN_POINT('Ctrl Pts',(-9.71128686315043,21.3680038433719,
4.64183375466668));
#101550=CARTESIAN_POINT('Ctrl Pts',(-9.71776170521399,21.3675425608669,
4.64345141953894));
#101551=CARTESIAN_POINT('Ctrl Pts',(-9.72761945962613,21.3668462466509,
4.64582542932428));
#101552=CARTESIAN_POINT('Ctrl Pts',(-9.73099240499729,21.3666090529338,
4.64662198996523));
#101553=CARTESIAN_POINT('Ctrl Pts',(-9.73708496443484,21.3661825770929,
4.64803245560088));
#101554=CARTESIAN_POINT('Ctrl Pts',(-9.7398032683243,21.3659930069641,4.64865159919433));
#101555=CARTESIAN_POINT('Ctrl Pts',(-9.74581574850585,21.3655752714533,
4.64999861277007));
#101556=CARTESIAN_POINT('Ctrl Pts',(-9.74911086286419,21.3653473613673,
4.65072198408916));
#101557=CARTESIAN_POINT('Ctrl Pts',(-9.75870468653502,21.3646866608307,
4.65278493280844));
#101558=CARTESIAN_POINT('Ctrl Pts',(-9.76501145436277,21.3642559179237,
4.65408704943447));
#101559=CARTESIAN_POINT('Ctrl Pts',(-9.81703417466507,21.3607299443617,
4.66438369511787));
#101560=CARTESIAN_POINT('Ctrl Pts',(-9.86324229880007,21.3577693813007,
4.67071103809498));
#101561=CARTESIAN_POINT('Ctrl Pts',(-9.98333399929278,21.3502382887052,
4.67994489720296));
#101562=CARTESIAN_POINT('Ctrl Pts',(-10.0573273847919,21.3457466972263,
4.67866939681464));
#101563=CARTESIAN_POINT('Ctrl Pts',(-10.1760339882518,21.3382354977675,
4.66541259719002));
#101564=CARTESIAN_POINT('Ctrl Pts',(-10.2210159069323,21.3353190849814,
4.65772436870066));
#101565=CARTESIAN_POINT('Ctrl Pts',(-10.2753100425379,21.3316528537621,
4.64516469027391));
#101566=CARTESIAN_POINT('Ctrl Pts',(-10.2851544486379,21.3309822295945,
4.64275313048984));
#101567=CARTESIAN_POINT('Ctrl Pts',(-10.3005960155963,21.3299204749674,
4.63875849640265));
#101568=CARTESIAN_POINT('Ctrl Pts',(-10.3062148225051,21.3295320647968,
4.63726046187481));
#101569=CARTESIAN_POINT('Ctrl Pts',(-10.3165702959627,21.3288122995571,
4.63441727502301));
#101570=CARTESIAN_POINT('Ctrl Pts',(-10.3213100860692,21.328481330143,4.63308390398976));
#101571=CARTESIAN_POINT('Ctrl Pts',(-10.3318115787902,21.3277445709373,
4.63005849322923));
#101572=CARTESIAN_POINT('Ctrl Pts',(-10.3375689498991,21.3273383230373,
4.62835203889783));
#101573=CARTESIAN_POINT('Ctrl Pts',(-10.3541355561356,21.326162502829,4.62330364396763));
#101574=CARTESIAN_POINT('Ctrl Pts',(-10.3649097564031,21.3253893328993,
4.61984995548207));
#101575=CARTESIAN_POINT('Ctrl Pts',(-10.4607946775943,21.3184303199654,
4.58758322931835));
#101576=CARTESIAN_POINT('Ctrl Pts',(-10.5423805778352,21.3119203202055,
4.54927878819919));
#101577=CARTESIAN_POINT('Ctrl Pts',(-10.677781617431,21.3002375554488,4.46566658218919));
#101578=CARTESIAN_POINT('Ctrl Pts',(-10.7334347878888,21.295131361341,4.42410772875779));
#101579=CARTESIAN_POINT('Ctrl Pts',(-10.7922887529663,21.2896000151356,
4.37147361930295));
#101580=CARTESIAN_POINT('Ctrl Pts',(-10.7993858571999,21.2889307652949,
4.36496820950128));
#101581=CARTESIAN_POINT('Ctrl Pts',(-10.8090878294552,21.2880137168224,
4.35585367917322));
#101582=CARTESIAN_POINT('Ctrl Pts',(-10.8117611785812,21.287760795513,4.35331847852627));
#101583=CARTESIAN_POINT('Ctrl Pts',(-10.8163302160157,21.2873281954461,
4.34894464741933));
#101584=CARTESIAN_POINT('Ctrl Pts',(-10.8182316770991,21.2871480642184,
4.34711212888631));
#101585=CARTESIAN_POINT('Ctrl Pts',(-10.8221954761754,21.2867723837437,
4.34326624977039));
#101586=CARTESIAN_POINT('Ctrl Pts',(-10.8242566087649,21.2865769359695,
4.34125169373057));
#101587=CARTESIAN_POINT('Ctrl Pts',(-10.8292799916466,21.2861002901267,
4.33630564158192));
#101588=CARTESIAN_POINT('Ctrl Pts',(-10.832234155061,21.2858197237098,4.33336591192429));
#101589=CARTESIAN_POINT('Ctrl Pts',(-10.8428636179949,21.2848089815148,
4.3226754916312));
#101590=CARTESIAN_POINT('Ctrl Pts',(-10.8504470414974,21.2840855453392,
4.31483366018202));
#101591=CARTESIAN_POINT('Ctrl Pts',(-10.8691610897656,21.2822908142297,
4.29493599764574));
#101592=CARTESIAN_POINT('Ctrl Pts',(-10.8801510704906,21.2812281599641,
4.28275052868337));
#101593=CARTESIAN_POINT('Ctrl Pts',(-10.9277274622911,21.2765674968214,
4.22772925870101));
#101594=CARTESIAN_POINT('Ctrl Pts',(-10.9614701114316,21.2730950872831,
4.18252790778383));
#101595=CARTESIAN_POINT('Ctrl Pts',(-11.034464058166,21.2647272749209,4.06852837226142));
#101596=CARTESIAN_POINT('Ctrl Pts',(-11.0702664090662,21.2598325230113,
3.99786359865141));
#101597=CARTESIAN_POINT('Ctrl Pts',(-11.1041550809007,21.2536957138836,
3.91007825678255));
#101598=CARTESIAN_POINT('Ctrl Pts',(-11.1093166522239,21.2527037635114,
3.89590295610612));
#101599=CARTESIAN_POINT('Ctrl Pts',(-11.1163619332114,21.251261094752,3.87533375995834));
#101600=CARTESIAN_POINT('Ctrl Pts',(-11.1184660082218,21.2508175818711,
3.8690165073243));
#101601=CARTESIAN_POINT('Ctrl Pts',(-11.1220728033281,21.2500343215023,
3.85787320683798));
#101602=CARTESIAN_POINT('Ctrl Pts',(-11.1235982473083,21.2496953234722,
3.85305464934382));
#101603=CARTESIAN_POINT('Ctrl Pts',(-11.1266845267381,21.2489931051004,
3.84308312128736));
#101604=CARTESIAN_POINT('Ctrl Pts',(-11.1282411338635,21.2486297566912,
3.83792897640752));
#101605=CARTESIAN_POINT('Ctrl Pts',(-11.1321458661258,21.2476941232236,
3.82467209187733));
#101606=CARTESIAN_POINT('Ctrl Pts',(-11.1344423379403,21.2471201880642,
3.81655458434204));
#101607=CARTESIAN_POINT('Ctrl Pts',(-11.1438374067516,21.2446672292287,
3.78192923535056));
#101608=CARTESIAN_POINT('Ctrl Pts',(-11.1500950833864,21.2427616881632,
3.75520421058968));
#101609=CARTESIAN_POINT('Ctrl Pts',(-11.1747225928471,21.2338109893741,
3.63055861103171));
#101610=CARTESIAN_POINT('Ctrl Pts',(-11.1815519657687,21.2264207830843,
3.53078472805198));
#101611=CARTESIAN_POINT('Ctrl Pts',(-11.1744612972435,21.2175518910583,
3.40931590665271));
#101612=CARTESIAN_POINT('Ctrl Pts',(-11.1725539858955,21.2159522736708,
3.38730489248347));
#101613=CARTESIAN_POINT('Ctrl Pts',(-11.1675250740633,21.2128055979059,
3.34360352561482));
#101614=CARTESIAN_POINT('Ctrl Pts',(-11.1644149784763,21.2112587818767,
3.32191978207275));
#101615=CARTESIAN_POINT('Ctrl Pts',(-11.1597657451936,21.2093589140312,
3.29489281092851));
#101616=CARTESIAN_POINT('Ctrl Pts',(-11.1587915082088,21.2089783336941,
3.2894583503408));
#101617=CARTESIAN_POINT('Ctrl Pts',(-11.1571907403435,21.2083798492295,
3.28087686924934));
#101618=CARTESIAN_POINT('Ctrl Pts',(-11.1565895182251,21.2081605856563,
3.27772529850798));
#101619=CARTESIAN_POINT('Ctrl Pts',(-11.1554924375407,21.2077701775835,
3.27209945878811));
#101620=CARTESIAN_POINT('Ctrl Pts',(-11.1550015086394,21.2075987654235,
3.26962433913444));
#101621=CARTESIAN_POINT('Ctrl Pts',(-11.1538042781537,21.2071884894799,
3.2636882853228));
#101622=CARTESIAN_POINT('Ctrl Pts',(-11.1530903581196,21.206950058039,3.26022893083061));
#101623=CARTESIAN_POINT('Ctrl Pts',(-11.1508697206862,21.2062267978725,
3.24970800420805));
#101624=CARTESIAN_POINT('Ctrl Pts',(-11.1493135846269,21.2057446521037,
3.2426568675873));
#101625=CARTESIAN_POINT('Ctrl Pts',(-11.1347205305769,21.2014325364851,
3.17930730219187));
#101626=CARTESIAN_POINT('Ctrl Pts',(-11.1176194348603,21.1978070249937,
3.1240170554102));
#101627=CARTESIAN_POINT('Ctrl Pts',(-11.0593837445126,21.1879019542428,
2.97544375652879));
#101628=CARTESIAN_POINT('Ctrl Pts',(-11.0101226965424,21.1817063151812,
2.88591264915616));
#101629=CARTESIAN_POINT('Ctrl Pts',(-10.9420019277671,21.1741702234808,
2.79295749048992));
#101630=CARTESIAN_POINT('Ctrl Pts',(-10.9338487750669,21.1732821932321,
2.78222344484587));
#101631=CARTESIAN_POINT('Ctrl Pts',(-10.9215330394064,21.1719595781677,
2.76657424038097));
#101632=CARTESIAN_POINT('Ctrl Pts',(-10.9175112892476,21.1715305141533,
2.76154924407858));
#101633=CARTESIAN_POINT('Ctrl Pts',(-10.9102887396569,21.1707648246262,
2.75267508316271));
#101634=CARTESIAN_POINT('Ctrl Pts',(-10.9071041811297,21.1704288531802,
2.74881285679101));
#101635=CARTESIAN_POINT('Ctrl Pts',(-10.9003456555051,21.169719174951,2.74072177781364));
#101636=CARTESIAN_POINT('Ctrl Pts',(-10.896766304651,21.1693452551555,2.73649760242505));
#101637=CARTESIAN_POINT('Ctrl Pts',(-10.8872030542396,21.1683511880839,
2.72537154404571));
#101638=CARTESIAN_POINT('Ctrl Pts',(-10.881168514265,21.1677289750639,2.71851388655775));
#101639=CARTESIAN_POINT('Ctrl Pts',(-10.8516763584051,21.1647114692983,
2.68577489064124));
#101640=CARTESIAN_POINT('Ctrl Pts',(-10.827157148463,21.1622719974959,2.66087798256142));
#101641=CARTESIAN_POINT('Ctrl Pts',(-10.7519895419738,21.1549822660332,
2.59105209623496));
#101642=CARTESIAN_POINT('Ctrl Pts',(-10.6985365808187,21.1500217906373,
2.54935847792475));
#101643=CARTESIAN_POINT('Ctrl Pts',(-10.5913465241177,21.1406355005657,
2.47969309061722));
#101644=CARTESIAN_POINT('Ctrl Pts',(-10.5384409198096,21.1362273893005,
2.45080994710929));
#101645=CARTESIAN_POINT('Ctrl Pts',(-10.4746300737837,21.1313231392644,
2.42207739369234));
#101646=CARTESIAN_POINT('Ctrl Pts',(-10.4656557121155,21.1306425690593,
2.41817024188138));
#101647=CARTESIAN_POINT('Ctrl Pts',(-10.4532181071734,21.1297129359121,
2.41293876110759));
#101648=CARTESIAN_POINT('Ctrl Pts',(-10.4497960688404,21.1294585633578,
2.41151835699353));
#101649=CARTESIAN_POINT('Ctrl Pts',(-10.443918502564,21.1290241330062,2.40911117515022));
#101650=CARTESIAN_POINT('Ctrl Pts',(-10.4414662740918,21.1288436144095,
2.40811649234232));
#101651=CARTESIAN_POINT('Ctrl Pts',(-10.4363407705603,21.1284678655562,
2.40605755491009));
#101652=CARTESIAN_POINT('Ctrl Pts',(-10.4336669221798,21.1282727330546,
2.40499482098623));
#101653=CARTESIAN_POINT('Ctrl Pts',(-10.4271339065682,21.1277980653066,
2.40242592520942));
#101654=CARTESIAN_POINT('Ctrl Pts',(-10.4232705862356,21.1275191493763,
2.40093028614284));
#101655=CARTESIAN_POINT('Ctrl Pts',(-10.4093610559541,21.1265210449645,
2.39562959549805));
#101656=CARTESIAN_POINT('Ctrl Pts',(-10.3992704201818,21.1258083769603,
2.3919415104663));
#101657=CARTESIAN_POINT('Ctrl Pts',(-10.3739600414459,21.1240457563599,
2.38308134222335));
#101658=CARTESIAN_POINT('Ctrl Pts',(-10.3586818657378,21.1230040533606,
2.37808165466593));
#101659=CARTESIAN_POINT('Ctrl Pts',(-10.2914146014787,21.118494913406,2.35758357973594));
#101660=CARTESIAN_POINT('Ctrl Pts',(-10.2384891239259,21.1151449211672,
2.34537381825059));
#101661=CARTESIAN_POINT('Ctrl Pts',(-10.1041615685227,21.106736958698,2.32401955978369));
#101662=CARTESIAN_POINT('Ctrl Pts',(-10.0223096222156,21.1016836574985,
2.3196272665717));
#101663=CARTESIAN_POINT('Ctrl Pts',(-9.92566052898394,21.0953719452171,
2.32450245495432));
#101664=CARTESIAN_POINT('Ctrl Pts',(-9.91067031644554,21.0943838234684,
2.3255465059992));
#101665=CARTESIAN_POINT('Ctrl Pts',(-9.88908277236535,21.0929457271959,
2.32746572423783));
#101666=CARTESIAN_POINT('Ctrl Pts',(-9.88246604931636,21.0925028936094,
2.32811048873557));
#101667=CARTESIAN_POINT('Ctrl Pts',(-9.8708308498433,21.0917204260234,2.32934380734268));
#101668=CARTESIAN_POINT('Ctrl Pts',(-9.86580999521794,21.0913815367225,
2.32990870782936));
#101669=CARTESIAN_POINT('Ctrl Pts',(-9.85544259007978,21.0906791459331,
2.33114275884775));
#101670=CARTESIAN_POINT('Ctrl Pts',(-9.85009669501997,21.0903155139542,
2.33181632760801));
#101671=CARTESIAN_POINT('Ctrl Pts',(-9.83637456789667,21.089378306202,2.33364102195471));
#101672=CARTESIAN_POINT('Ctrl Pts',(-9.82800588999497,21.0888030695785,
2.33484568947816));
#101673=CARTESIAN_POINT('Ctrl Pts',(-9.81680032626574,21.088027758761,2.33658207678296));
#101674=CARTESIAN_POINT('Ctrl Pts',(-9.81395129694457,21.0878301939243,
2.33703428108315));
#101675=CARTESIAN_POINT('Ctrl Pts',(-9.81110406314734,21.0876323086995,
2.33749693009414));
#101676=CARTESIAN_POINT('Ctrl Pts',(-9.81110406371161,20.988570409963,2.33749693000245));
#101677=CARTESIAN_POINT('Ctrl Pts',(-9.81154564090745,20.9885986138497,
2.33742517781529));
#101678=CARTESIAN_POINT('Ctrl Pts',(-9.81198726021747,20.9886268116318,
2.33735367703001));
#101679=CARTESIAN_POINT('Ctrl Pts',(-9.89061252215599,20.9936455543156,
2.32466974970649));
#101680=CARTESIAN_POINT('Ctrl Pts',(-9.96987033142047,20.9984459045583,
2.31997459421931));
#101681=CARTESIAN_POINT('Ctrl Pts',(-10.0714622469342,21.0048223705121,
2.32420514394297));
#101682=CARTESIAN_POINT('Ctrl Pts',(-10.0938901091305,21.0062429994486,
2.32578325338818));
#101683=CARTESIAN_POINT('Ctrl Pts',(-10.1454347139656,21.0095536917515,
2.33089630592362));
#101684=CARTESIAN_POINT('Ctrl Pts',(-10.1744907577607,21.0114539862627,
2.33487878170737));
#101685=CARTESIAN_POINT('Ctrl Pts',(-10.2121854611868,21.0139787103814,
2.34148691748549));
#101686=CARTESIAN_POINT('Ctrl Pts',(-10.2209866004524,21.0145724376907,
2.34313347901222));
#101687=CARTESIAN_POINT('Ctrl Pts',(-10.2351582057523,21.0155357024768,
2.34595239022433));
#101688=CARTESIAN_POINT('Ctrl Pts',(-10.2405408480495,21.0159032629769,
2.3470622887425));
#101689=CARTESIAN_POINT('Ctrl Pts',(-10.2508187068302,21.0166084346186,
2.34925668513458));
#101690=CARTESIAN_POINT('Ctrl Pts',(-10.2557151638454,21.0169458378856,
2.35033485133998));
#101691=CARTESIAN_POINT('Ctrl Pts',(-10.2669532748006,21.0177236479194,
2.35288475151277));
#101692=CARTESIAN_POINT('Ctrl Pts',(-10.2732898602838,21.0181647261048,
2.35437785742977));
#101693=CARTESIAN_POINT('Ctrl Pts',(-10.2930945040031,21.0195513562585,
2.35921813503534));
#101694=CARTESIAN_POINT('Ctrl Pts',(-10.3065155617127,21.0205027794733,
2.36275076017877));
#101695=CARTESIAN_POINT('Ctrl Pts',(-10.3732860600221,21.025297086593,2.38159353656787));
#101696=CARTESIAN_POINT('Ctrl Pts',(-10.4255613565746,21.0292513415884,
2.40042215953935));
#101697=CARTESIAN_POINT('Ctrl Pts',(-10.5327527806387,21.037763712179,2.44782202949778));
#101698=CARTESIAN_POINT('Ctrl Pts',(-10.587147324562,21.0423279138933,2.4771795833104));
#101699=CARTESIAN_POINT('Ctrl Pts',(-10.6574821338285,21.0484322724202,
2.52260702654373));
#101700=CARTESIAN_POINT('Ctrl Pts',(-10.6756386939345,21.0500272416079,
2.53506879640161));
#101701=CARTESIAN_POINT('Ctrl Pts',(-10.7114594161842,21.0531989351113,
2.56116147982816));
#101702=CARTESIAN_POINT('Ctrl Pts',(-10.7291078168543,21.0547745707211,
2.57480044467821));
#101703=CARTESIAN_POINT('Ctrl Pts',(-10.7506549218015,21.0567044539238,
2.59245215959245));
#101704=CARTESIAN_POINT('Ctrl Pts',(-10.7549254166935,21.0570872537584,
2.59600137580944));
#101705=CARTESIAN_POINT('Ctrl Pts',(-10.7616286837894,21.0576884012062,
2.6016531034189));
#101706=CARTESIAN_POINT('Ctrl Pts',(-10.7640781544275,21.0579081285107,
2.60373554509684));
#101707=CARTESIAN_POINT('Ctrl Pts',(-10.7684332777394,21.0582988592766,
2.60746892670866));
#101708=CARTESIAN_POINT('Ctrl Pts',(-10.7703421477392,21.0584701341852,
2.60911594765053));
#101709=CARTESIAN_POINT('Ctrl Pts',(-10.7749031601599,21.0588794325035,
2.61307692414931));
#101710=CARTESIAN_POINT('Ctrl Pts',(-10.7775502337982,21.0591170290067,
2.61539665112905));
#101711=CARTESIAN_POINT('Ctrl Pts',(-10.7855509635379,21.0598354626007,
2.62247164203893));
#101712=CARTESIAN_POINT('Ctrl Pts',(-10.7908718103145,21.0603136679155,
2.62726400252087));
#101713=CARTESIAN_POINT('Ctrl Pts',(-10.8401253760307,21.0647479041644,
2.67244591334805));
#101714=CARTESIAN_POINT('Ctrl Pts',(-10.8809788604181,21.0684853233663,
2.71607735761498));
#101715=CARTESIAN_POINT('Ctrl Pts',(-10.9806828145175,21.078362541328,2.8402520021803));
#101716=CARTESIAN_POINT('Ctrl Pts',(-11.0329121469552,21.0844331029509,
2.92545966933217));
#101717=CARTESIAN_POINT('Ctrl Pts',(-11.0794508365027,21.0918383931154,
3.02875686773288));
#101718=CARTESIAN_POINT('Ctrl Pts',(-11.0848797272695,21.0927441592198,
3.04139325160445));
#101719=CARTESIAN_POINT('Ctrl Pts',(-11.0925153469007,21.094083459204,3.0600608466953));
#101720=CARTESIAN_POINT('Ctrl Pts',(-11.0948961450542,21.0945111708585,
3.06601996517926));
#101721=CARTESIAN_POINT('Ctrl Pts',(-11.0990508773686,21.0952761030237,
3.07667106149437));
#101722=CARTESIAN_POINT('Ctrl Pts',(-11.1008437731231,21.095612683287,3.08135551232209));
#101723=CARTESIAN_POINT('Ctrl Pts',(-11.1045356614451,21.0963196453872,
3.09118933909534));
#101724=CARTESIAN_POINT('Ctrl Pts',(-11.1064286877198,21.0966902152309,
3.09634081070988));
#101725=CARTESIAN_POINT('Ctrl Pts',(-11.1113034018002,21.0976661609161,
3.10989826783242));
#101726=CARTESIAN_POINT('Ctrl Pts',(-11.1142256797146,21.0982734709802,
3.11832508684376));
#101727=CARTESIAN_POINT('Ctrl Pts',(-11.1273248236092,21.1011028537429,
3.15753140946153));
#101728=CARTESIAN_POINT('Ctrl Pts',(-11.136322926937,21.1033626812468,3.18868690122713));
#101729=CARTESIAN_POINT('Ctrl Pts',(-11.1587195841948,21.110042016487,3.28025119861834));
#101730=CARTESIAN_POINT('Ctrl Pts',(-11.1686579903668,21.1145542407696,
3.34138883224352));
#101731=CARTESIAN_POINT('Ctrl Pts',(-11.1794438209105,21.1241702078613,
3.47192558831706));
#101732=CARTESIAN_POINT('Ctrl Pts',(-11.1790587667774,21.1292631194004,
3.54120840115635));
#101733=CARTESIAN_POINT('Ctrl Pts',(-11.1716958218964,21.1347827839524,
3.61965260157989));
#101734=CARTESIAN_POINT('Ctrl Pts',(-11.1706780137146,21.1354524242924,
3.62923175796202));
#101735=CARTESIAN_POINT('Ctrl Pts',(-11.1691085773061,21.1363698526213,
3.6424562035722));
#101736=CARTESIAN_POINT('Ctrl Pts',(-11.1686572292205,21.1366227701528,
3.64611268588511));
#101737=CARTESIAN_POINT('Ctrl Pts',(-11.16785299283,21.1370553265834,3.65238576045523));
#101738=CARTESIAN_POINT('Ctrl Pts',(-11.1675084537776,21.1372354181284,
3.65500336629065));
#101739=CARTESIAN_POINT('Ctrl Pts',(-11.1667695710616,21.1376109702939,
3.6604747005108));
#101740=CARTESIAN_POINT('Ctrl Pts',(-11.1663735553362,21.1378063297447,
3.6633281700207));
#101741=CARTESIAN_POINT('Ctrl Pts',(-11.1653794727514,21.1382826797727,
3.67030293401405));
#101742=CARTESIAN_POINT('Ctrl Pts',(-11.1647700016236,21.1385630399553,
3.67442261745356));
#101743=CARTESIAN_POINT('Ctrl Pts',(-11.162487402374,21.1395725799719,3.68930598295207));
#101744=CARTESIAN_POINT('Ctrl Pts',(-11.1606867584251,21.1402950397002,
3.70004995796409));
#101745=CARTESIAN_POINT('Ctrl Pts',(-11.1558063064342,21.1420869486675,
3.72688118864197));
#101746=CARTESIAN_POINT('Ctrl Pts',(-11.1525394399606,21.1431477903619,
3.74293247528852));
#101747=CARTESIAN_POINT('Ctrl Pts',(-11.1365940327204,21.1477956352903,
3.81369146068927));
#101748=CARTESIAN_POINT('Ctrl Pts',(-11.1203464074761,21.1512577245616,
3.86752313020131));
#101749=CARTESIAN_POINT('Ctrl Pts',(-11.0720527831591,21.1596291581774,
3.9940449992541));
#101750=CARTESIAN_POINT('Ctrl Pts',(-11.0363880347072,21.1645376023556,
4.06504461538111));
#101751=CARTESIAN_POINT('Ctrl Pts',(-10.9857756510308,21.170689469143,4.14464628008067));
#101752=CARTESIAN_POINT('Ctrl Pts',(-10.9774413006887,21.1716810807169,
4.15721452397165));
#101753=CARTESIAN_POINT('Ctrl Pts',(-10.9650838299278,21.1731232556094,
4.1750944883846));
#101754=CARTESIAN_POINT('Ctrl Pts',(-10.9612531316651,21.1735666184544,
4.18053786143023));
#101755=CARTESIAN_POINT('Ctrl Pts',(-10.9544338540055,21.1743496119374,
4.19005551146871));
#101756=CARTESIAN_POINT('Ctrl Pts',(-10.9514647856071,21.1746884936265,
4.19414360975794));
#101757=CARTESIAN_POINT('Ctrl Pts',(-10.9452787790403,21.1753904681497,
4.20254683867452));
#101758=CARTESIAN_POINT('Ctrl Pts',(-10.9420583871401,21.1757536889523,
4.20685926759882));
#101759=CARTESIAN_POINT('Ctrl Pts',(-10.9337165852982,21.17668898526,4.21787151784638));
#101760=CARTESIAN_POINT('Ctrl Pts',(-10.9285526431293,21.1772627096449,
4.22453858440401));
#101761=CARTESIAN_POINT('Ctrl Pts',(-10.9062892814536,21.1797146238594,
4.2526534307638));
#101762=CARTESIAN_POINT('Ctrl Pts',(-10.8885162073047,21.1816193076829,
4.27355425230225));
#101763=CARTESIAN_POINT('Ctrl Pts',(-10.8029055706081,21.1905671575275,
4.36738465427131));
#101764=CARTESIAN_POINT('Ctrl Pts',(-10.7267254541968,21.1979552228097,
4.43213606072194));
#101765=CARTESIAN_POINT('Ctrl Pts',(-10.6248350759737,21.2068218217987,
4.49858084636574));
#101766=CARTESIAN_POINT('Ctrl Pts',(-10.6060039454294,21.2084209034416,
4.51011974061249));
#101767=CARTESIAN_POINT('Ctrl Pts',(-10.5678311798878,21.2115704985386,
4.53205835324206));
#101768=CARTESIAN_POINT('Ctrl Pts',(-10.5485001835475,21.2131206708753,
4.54246073941665));
#101769=CARTESIAN_POINT('Ctrl Pts',(-10.5239529926709,21.2150239642162,
4.55479800627797));
#101770=CARTESIAN_POINT('Ctrl Pts',(-10.5190001609658,21.2154047336667,
4.55724377912728));
#101771=CARTESIAN_POINT('Ctrl Pts',(-10.5111435854824,21.2160034035956,
4.56105494236738));
#101772=CARTESIAN_POINT('Ctrl Pts',(-10.5082512326133,21.2162226654962,
4.56244342949355));
#101773=CARTESIAN_POINT('Ctrl Pts',(-10.5030748862707,21.2166130005149,
4.5649023820717));
#101774=CARTESIAN_POINT('Ctrl Pts',(-10.5007931395268,21.2167843416638,
4.56597732439389));
#101775=CARTESIAN_POINT('Ctrl Pts',(-10.4953103495957,21.2171943525046,
4.56853880411862));
#101776=CARTESIAN_POINT('Ctrl Pts',(-10.4921060596624,21.217432590908,4.57001829198612));
#101777=CARTESIAN_POINT('Ctrl Pts',(-10.4823362115003,21.2181549234049,
4.57447606626499));
#101778=CARTESIAN_POINT('Ctrl Pts',(-10.4757497641976,21.218636343718,4.57740856048036));
#101779=CARTESIAN_POINT('Ctrl Pts',(-10.406689354833,21.223630695253,4.60739962892105));
#101780=CARTESIAN_POINT('Ctrl Pts',(-10.3419981526692,21.2278586349213,
4.62905724252357));
#101781=CARTESIAN_POINT('Ctrl Pts',(-10.1886170451612,21.2376195215725,
4.66600108341388));
#101782=CARTESIAN_POINT('Ctrl Pts',(-10.0993433749463,21.2431279394555,
4.67697221023942));
#101783=CARTESIAN_POINT('Ctrl Pts',(-9.9950210428757,21.2499363005898,4.67783087533478));
#101784=CARTESIAN_POINT('Ctrl Pts',(-9.98034807543187,21.2509016250325,
4.67767743103788));
#101785=CARTESIAN_POINT('Ctrl Pts',(-9.95910072027127,21.2523123764753,
4.67705805534586));
#101786=CARTESIAN_POINT('Ctrl Pts',(-9.95252096252726,21.2527510403674,
4.67681101064465));
#101787=CARTESIAN_POINT('Ctrl Pts',(-9.94090819259789,21.2535285650007,
4.67627744643598));
#101788=CARTESIAN_POINT('Ctrl Pts',(-9.93587425784356,21.2538667096216,
4.67601375865072));
#101789=CARTESIAN_POINT('Ctrl Pts',(-9.92544019535183,21.2545699523815,
4.67540000895739));
#101790=CARTESIAN_POINT('Ctrl Pts',(-9.92004048721214,21.2549351955567,
4.67504502898794));
#101791=CARTESIAN_POINT('Ctrl Pts',(-9.90609885812247,21.2558817055601,
4.6740319562832));
#101792=CARTESIAN_POINT('Ctrl Pts',(-9.89756145409032,21.256464698335,4.67331785820197));
#101793=CARTESIAN_POINT('Ctrl Pts',(-9.86044273670116,21.2590146620994,
4.66980491764224));
#101794=CARTESIAN_POINT('Ctrl Pts',(-9.83196356980939,21.2610108445436,
4.66605458075093));
#101795=CARTESIAN_POINT('Ctrl Pts',(-9.70638529070889,21.2699968738891,
4.64482170220833));
#101796=CARTESIAN_POINT('Ctrl Pts',(-9.61157926070604,21.2773176200586,
4.61622131678748));
#101797=CARTESIAN_POINT('Ctrl Pts',(-9.48342597116334,21.2875371123037,
4.55923542330977));
#101798=CARTESIAN_POINT('Ctrl Pts',(-9.44630315176044,21.2905328236377,
4.54031197377109));
#101799=CARTESIAN_POINT('Ctrl Pts',(-9.4050893413494,21.2938417619775,4.51647036939357));
#101800=CARTESIAN_POINT('Ctrl Pts',(-9.39994436455622,21.2942545056208,
4.51344163212387));
#101801=CARTESIAN_POINT('Ctrl Pts',(-9.39173790569342,21.2949120471539,
4.5085262591544));
#101802=CARTESIAN_POINT('Ctrl Pts',(-9.3886617278601,21.2951583430357,4.50666454624072));
#101803=CARTESIAN_POINT('Ctrl Pts',(-9.38320510005982,21.2955948394334,
4.50332793993167));
#101804=CARTESIAN_POINT('Ctrl Pts',(-9.38082132794078,21.2957853893846,
4.5018586109474));
#101805=CARTESIAN_POINT('Ctrl Pts',(-9.37570217889202,21.2961942856514,
4.49867797770765));
#101806=CARTESIAN_POINT('Ctrl Pts',(-9.37296858404418,21.2964124505531,
4.49696392945528));
#101807=CARTESIAN_POINT('Ctrl Pts',(-9.36538026488416,21.2970176554021,
4.49216226250676));
#101808=CARTESIAN_POINT('Ctrl Pts',(-9.36054098793095,21.297403141663,4.48905022045298));
#101809=CARTESIAN_POINT('Ctrl Pts',(-9.33216500349244,21.2996619525451,
4.47050686126541));
#101810=CARTESIAN_POINT('Ctrl Pts',(-9.30916259113074,21.301486711869,4.45426994197139));
#101811=CARTESIAN_POINT('Ctrl Pts',(-9.22763760337343,21.3080175628248,
4.39222844277644));
#101812=CARTESIAN_POINT('Ctrl Pts',(-9.17289961975558,21.312536437468,4.34173737174336));
#101813=CARTESIAN_POINT('Ctrl Pts',(-9.08080888038258,21.3211081214306,
4.23907279221526));
#101814=CARTESIAN_POINT('Ctrl Pts',(-9.04224760145529,21.3251195339991,
4.18836735335184));
#101815=CARTESIAN_POINT('Ctrl Pts',(-9.00266521871272,21.3299443197606,
4.12651040437049));
#101816=CARTESIAN_POINT('Ctrl Pts',(-8.99746402292412,21.3305946209163,
4.11815334490128));
#101817=CARTESIAN_POINT('Ctrl Pts',(-8.98912324854826,21.3316652474119,
4.10436954359671));
#101818=CARTESIAN_POINT('Ctrl Pts',(-8.98592110023948,21.3320833027469,
4.09898108012593));
#101819=CARTESIAN_POINT('Ctrl Pts',(-8.98024924889666,21.3328367046411,
4.08926083308064));
#101820=CARTESIAN_POINT('Ctrl Pts',(-8.97776373635961,21.3331714736486,
4.08493841023257));
#101821=CARTESIAN_POINT('Ctrl Pts',(-8.97252951700681,21.3338864636661,
4.07570060328802));
#101822=CARTESIAN_POINT('Ctrl Pts',(-8.96978847818066,21.3342669472355,
4.07078104072404));
#101823=CARTESIAN_POINT('Ctrl Pts',(-8.96248321550514,21.3352976722442,
4.05744563989258));
#101824=CARTESIAN_POINT('Ctrl Pts',(-8.95798623633236,21.3359502596197,
4.0489936488159));
#101825=CARTESIAN_POINT('Ctrl Pts',(-8.93480562539564,21.339412618335,4.00411502754312));
#101826=CARTESIAN_POINT('Ctrl Pts',(-8.91792976471142,21.3422840251816,
3.9667915223606));
#101827=CARTESIAN_POINT('Ctrl Pts',(-8.86567853363002,21.3525466616692,
3.83308018475613));
#101828=CARTESIAN_POINT('Ctrl Pts',(-8.84098351146032,21.3602280785029,
3.7330335261323));
#101829=CARTESIAN_POINT('Ctrl Pts',(-8.82679678713881,21.3693812433472,
3.60633953495458));
#101830=CARTESIAN_POINT('Ctrl Pts',(-8.82481225723331,21.3711437800464,
3.58153439140686));
#101831=CARTESIAN_POINT('Ctrl Pts',(-8.82333834893399,21.3732669246141,
3.55094526049342));
#101832=CARTESIAN_POINT('Ctrl Pts',(-8.82310385595059,21.3736631351421,
3.54520542167043));
#101833=CARTESIAN_POINT('Ctrl Pts',(-8.82280216638695,21.3742806281274,
3.53620694740019));
#101834=CARTESIAN_POINT('Ctrl Pts',(-8.82270648660259,21.3745034134395,
3.53294945324659));
#101835=CARTESIAN_POINT('Ctrl Pts',(-8.82255385112819,21.3749159110755,
3.52689691407597));
#101836=CARTESIAN_POINT('Ctrl Pts',(-8.82249332592416,21.3751058084816,
3.52410207966527));
#101837=CARTESIAN_POINT('Ctrl Pts',(-8.82237748541622,21.3755395033274,
3.51770000197227));
#101838=CARTESIAN_POINT('Ctrl Pts',(-8.82232879223608,21.3757829331426,
3.51409270020506));
#101839=CARTESIAN_POINT('Ctrl Pts',(-8.82222891109429,21.3765372402006,
3.50287396588964));
#101840=CARTESIAN_POINT('Ctrl Pts',(-8.82223493142859,21.3770450865625,
3.49526203499083));
#101841=CARTESIAN_POINT('Ctrl Pts',(-8.8224219643369,21.3782269110615,3.4774260861938));
#101842=CARTESIAN_POINT('Ctrl Pts',(-8.822662327604,21.378898023308,3.46720316192881));
#101843=CARTESIAN_POINT('Ctrl Pts',(-8.82398925523013,21.3812632906469,
3.43089674910637));
#101844=CARTESIAN_POINT('Ctrl Pts',(-8.82580985829891,21.3829271398711,
3.40484628954157));
#101845=CARTESIAN_POINT('Ctrl Pts',(-8.8369296966279,21.3897358894272,3.2972956070754));
#101846=CARTESIAN_POINT('Ctrl Pts',(-8.85386275014144,21.3947014451756,
3.21681821422124));
#101847=CARTESIAN_POINT('Ctrl Pts',(-8.89307350196077,21.4027389105031,
3.09514477982906));
#101848=CARTESIAN_POINT('Ctrl Pts',(-8.90965692252478,21.4056685141406,
3.05240057632517));
#101849=CARTESIAN_POINT('Ctrl Pts',(-8.93290010578409,21.409349318696,3.00150648525169));
#101850=CARTESIAN_POINT('Ctrl Pts',(-8.93723320736266,21.4100205244395,
2.99233406420002));
#101851=CARTESIAN_POINT('Ctrl Pts',(-8.94423608637796,21.4110829190323,
2.97799286790172));
#101852=CARTESIAN_POINT('Ctrl Pts',(-8.94682666505395,21.4114713808675,
2.97278580086486));
#101853=CARTESIAN_POINT('Ctrl Pts',(-8.9516806384427,21.4121910735635,2.96320785734931));
#101854=CARTESIAN_POINT('Ctrl Pts',(-8.95393308207187,21.4125219176924,
2.95883155101292));
#101855=CARTESIAN_POINT('Ctrl Pts',(-8.95899186883728,21.4132581874936,
2.9491523542884));
#101856=CARTESIAN_POINT('Ctrl Pts',(-8.96181141905327,21.4136640694684,
2.94385655985796));
#101857=CARTESIAN_POINT('Ctrl Pts',(-8.97005511184859,21.4148381740305,
2.92865408769705));
#101858=CARTESIAN_POINT('Ctrl Pts',(-8.97558132892231,21.415609979382,2.91880382399427));
#101859=CARTESIAN_POINT('Ctrl Pts',(-9.0229852836873,21.4221081608214,2.83708519005339));
#101860=CARTESIAN_POINT('Ctrl Pts',(-9.07221869555927,21.4281086586544,
2.76977365273283));
#101861=CARTESIAN_POINT('Ctrl Pts',(-9.17954640257612,21.4398163832943,
2.65158794907028));
#101862=CARTESIAN_POINT('Ctrl Pts',(-9.2363744279862,21.4454750502884,2.60009718495586));
#101863=CARTESIAN_POINT('Ctrl Pts',(-9.30525363052713,21.4514809814556,
2.54894334776844));
#101864=CARTESIAN_POINT('Ctrl Pts',(-9.31277330588414,21.4521261099288,
2.54349555254843));
#101865=CARTESIAN_POINT('Ctrl Pts',(-9.32332281259553,21.4530157526779,
2.53604137278203));
#101866=CARTESIAN_POINT('Ctrl Pts',(-9.32629844172185,21.4532650067609,
2.5339593889506));
#101867=CARTESIAN_POINT('Ctrl Pts',(-9.33144261961252,21.4536929556091,
2.53039544672466));
#101868=CARTESIAN_POINT('Ctrl Pts',(-9.33360656086063,21.4538720821405,
2.52890693277009));
#101869=CARTESIAN_POINT('Ctrl Pts',(-9.338165246464,21.4542475358484,2.52579355566578));
#101870=CARTESIAN_POINT('Ctrl Pts',(-9.34056102896826,21.4544437522708,
2.5241702602653));
#101871=CARTESIAN_POINT('Ctrl Pts',(-9.34647387744535,21.4549253799471,
2.52019564828033));
#101872=CARTESIAN_POINT('Ctrl Pts',(-9.34999772057944,21.455210127747,2.51785439030807));
#101873=CARTESIAN_POINT('Ctrl Pts',(-9.36301452579025,21.4562538868665,
2.50930670683235));
#101874=CARTESIAN_POINT('Ctrl Pts',(-9.37258474779524,21.4570055662909,
2.50321826845062));
#101875=CARTESIAN_POINT('Ctrl Pts',(-9.39696813417252,21.4588854081707,
2.48819626184515));
#101876=CARTESIAN_POINT('Ctrl Pts',(-9.41189329411615,21.4600038422507,
2.47944877470532));
#101877=CARTESIAN_POINT('Ctrl Pts',(-9.48141641054314,21.4650927957274,
2.44073394308111));
#101878=CARTESIAN_POINT('Ctrl Pts',(-9.5381479879789,21.4689133235716,2.41479613307216));
#101879=CARTESIAN_POINT('Ctrl Pts',(-9.66624522916771,21.4773478406234,
2.36810473132451));
#101880=CARTESIAN_POINT('Ctrl Pts',(-9.73804036721294,21.4819622223032,
2.34936910054604));
#101881=CARTESIAN_POINT('Ctrl Pts',(-9.81110407243713,21.4868028556135,
2.33749692858463));
#101882=CARTESIAN_POINT('Origin',(-10.,12.3756328852638,3.5));
#101883=CARTESIAN_POINT('',(-9.8111040636317,22.0857064764352,2.33749693001543));
#101884=CARTESIAN_POINT('',(-9.81110406961625,21.9876672748128,2.337496929043));
#101885=CARTESIAN_POINT('',(-9.81110406371068,12.3756328852638,2.3374969300026));
#101886=CARTESIAN_POINT('Ctrl Pts',(-9.81110406355273,22.0857064764352,
2.33749693002826));
#101887=CARTESIAN_POINT('Ctrl Pts',(-9.8103247751117,22.0856498195303,2.33762355715178));
#101888=CARTESIAN_POINT('Ctrl Pts',(-9.80954560011318,22.0855931853744,
2.33775097013001));
#101889=CARTESIAN_POINT('Ctrl Pts',(-9.79283541045386,22.0843789276208,
2.34050072497862));
#101890=CARTESIAN_POINT('Ctrl Pts',(-9.77695900832715,22.0832314482922,
2.34344973863966));
#101891=CARTESIAN_POINT('Ctrl Pts',(-9.75059291391459,22.0813413382915,
2.34891036631903));
#101892=CARTESIAN_POINT('Ctrl Pts',(-9.74006838971411,22.0805910350128,
2.35124118369179));
#101893=CARTESIAN_POINT('Ctrl Pts',(-9.72553964738539,22.0795624077329,
2.35466870128597));
#101894=CARTESIAN_POINT('Ctrl Pts',(-9.72150738656724,22.0792776921328,
2.35564247957726));
#101895=CARTESIAN_POINT('Ctrl Pts',(-9.71468602652686,22.0787974358861,
2.35732800699329));
#101896=CARTESIAN_POINT('Ctrl Pts',(-9.71189426241367,22.0786012801257,
2.35802870801962));
#101897=CARTESIAN_POINT('Ctrl Pts',(-9.70654196415059,22.0782260135799,
2.35939295117848));
#101898=CARTESIAN_POINT('Ctrl Pts',(-9.70398107014798,22.0780468096624,
2.36005489073016));
#101899=CARTESIAN_POINT('Ctrl Pts',(-9.69784286012353,22.0776180640313,
2.36166357413394));
#101900=CARTESIAN_POINT('Ctrl Pts',(-9.69426770543513,22.0773689881369,
2.3626185685466));
#101901=CARTESIAN_POINT('Ctrl Pts',(-9.68128846490411,22.0764668861262,
2.3661512009867));
#101902=CARTESIAN_POINT('Ctrl Pts',(-9.67191166545329,22.0758192644764,
2.3688288362949));
#101903=CARTESIAN_POINT('Ctrl Pts',(-9.60396894989899,22.0711492975925,
2.38914649991693));
#101904=CARTESIAN_POINT('Ctrl Pts',(-9.54681501114852,22.0673407774482,
2.41121101967124));
#101905=CARTESIAN_POINT('Ctrl Pts',(-9.43122370003349,22.0594074206221,
2.46652395825332));
#101906=CARTESIAN_POINT('Ctrl Pts',(-9.37339822592928,22.0552976053787,
2.50052573707119));
#101907=CARTESIAN_POINT('Ctrl Pts',(-9.29044656281656,22.048833136515,2.55934326753237));
#101908=CARTESIAN_POINT('Ctrl Pts',(-9.26302129996159,22.0465908391404,
2.58067241863764));
#101909=CARTESIAN_POINT('Ctrl Pts',(-9.22963691461689,22.0436995464849,
2.60909095729312));
#101910=CARTESIAN_POINT('Ctrl Pts',(-9.22276266541128,22.0430950781334,
2.61508174180841));
#101911=CARTESIAN_POINT('Ctrl Pts',(-9.21182992672751,22.0421185383506,
2.62483509325445));
#101912=CARTESIAN_POINT('Ctrl Pts',(-9.20772709699707,22.0417485446261,
2.62854757801004));
#101913=CARTESIAN_POINT('Ctrl Pts',(-9.19996196585082,22.0410414471881,
2.63567409326709));
#101914=CARTESIAN_POINT('Ctrl Pts',(-9.19629496727374,22.0407045704094,
2.63908284476846));
#101915=CARTESIAN_POINT('Ctrl Pts',(-9.18795891131913,22.0399318846853,
2.64693151218014));
#101916=CARTESIAN_POINT('Ctrl Pts',(-9.18330436444943,22.039495435716,2.65138653638812));
#101917=CARTESIAN_POINT('Ctrl Pts',(-9.16900058793069,22.0381383789181,
2.66530384018087));
#101918=CARTESIAN_POINT('Ctrl Pts',(-9.15947779084611,22.0372122538678,
2.67489389075329));
#101919=CARTESIAN_POINT('Ctrl Pts',(-9.07984663606967,22.0292685678515,
2.75789670383281));
#101920=CARTESIAN_POINT('Ctrl Pts',(-9.01934912951955,22.0218333625618,
2.83991299501524));
#101921=CARTESIAN_POINT('Ctrl Pts',(-8.94198618195627,22.0101346966179,
2.97936010306964));
#101922=CARTESIAN_POINT('Ctrl Pts',(-8.91763002963586,22.0059055615872,
3.03209403724379));
#101923=CARTESIAN_POINT('Ctrl Pts',(-8.89471958978426,22.0013639490506,
3.09318001584837));
#101924=CARTESIAN_POINT('Ctrl Pts',(-8.89224413626641,22.0008639956864,
3.09996970409996));
#101925=CARTESIAN_POINT('Ctrl Pts',(-8.88865156322865,22.000124765676,3.11011258122135));
#101926=CARTESIAN_POINT('Ctrl Pts',(-8.88748684223309,21.9998828559432,
3.11344855212162));
#101927=CARTESIAN_POINT('Ctrl Pts',(-8.88551605898633,21.9994696833693,
3.11917592561827));
#101928=CARTESIAN_POINT('Ctrl Pts',(-8.88470265195474,21.999297996826,3.12156472641531));
#101929=CARTESIAN_POINT('Ctrl Pts',(-8.88287277281675,21.9989091200592,
3.12699583242468));
#101930=CARTESIAN_POINT('Ctrl Pts',(-8.88186104704888,21.9986922082007,
3.13003968691543));
#101931=CARTESIAN_POINT('Ctrl Pts',(-8.87914289687149,21.9981040993601,
3.1383304574281));
#101932=CARTESIAN_POINT('Ctrl Pts',(-8.8774608600233,21.9977342835829,3.14358537369414));
#101933=CARTESIAN_POINT('Ctrl Pts',(-8.86929898277906,21.9959090549653,
3.16971525283914));
#101934=CARTESIAN_POINT('Ctrl Pts',(-8.8633637300722,21.9944823236821,3.19075747016308));
#101935=CARTESIAN_POINT('Ctrl Pts',(-8.85261760544848,21.991656970104,3.23336143327061));
#101936=CARTESIAN_POINT('Ctrl Pts',(-8.84782074009101,21.9902593388887,
3.25491728925781));
#101937=CARTESIAN_POINT('Ctrl Pts',(-8.82475682652325,21.9826318004815,
3.37429918182883));
#101938=CARTESIAN_POINT('Ctrl Pts',(-8.81833950296988,21.9766386422591,
3.47399664970996));
#101939=CARTESIAN_POINT('Ctrl Pts',(-8.82625031172498,21.9684940855511,
3.60083017933001));
#101940=CARTESIAN_POINT('Ctrl Pts',(-8.82893183874177,21.9667033237362,
3.62827402932933));
#101941=CARTESIAN_POINT('Ctrl Pts',(-8.83368978543899,21.9643246228715,
3.66397237620907));
#101942=CARTESIAN_POINT('Ctrl Pts',(-8.83489615623078,21.9637638306331,
3.67233538173899));
#101943=CARTESIAN_POINT('Ctrl Pts',(-8.83701882998091,21.9628408896615,
3.68600774328032));
#101944=CARTESIAN_POINT('Ctrl Pts',(-8.83788177904923,21.9624804194345,
3.69132517155686));
#101945=CARTESIAN_POINT('Ctrl Pts',(-8.83962481761764,21.9617795913581,
3.70161853040299));
#101946=CARTESIAN_POINT('Ctrl Pts',(-8.84050051241438,21.9614393789712,
3.70659509337616));
#101947=CARTESIAN_POINT('Ctrl Pts',(-8.84260295194821,21.9606490044631,
3.71810862347875));
#101948=CARTESIAN_POINT('Ctrl Pts',(-8.84385309035559,21.9601981136261,
3.72464108849274));
#101949=CARTESIAN_POINT('Ctrl Pts',(-8.84811095153056,21.958721677096,3.74591250977103));
#101950=CARTESIAN_POINT('Ctrl Pts',(-8.85134562441883,21.9576890189019,
3.76060397433992));
#101951=CARTESIAN_POINT('Ctrl Pts',(-8.87382280160247,21.9510294572635,
3.85412431780265));
#101952=CARTESIAN_POINT('Ctrl Pts',(-8.90088399175274,21.9451510444456,
3.93083474910885));
#101953=CARTESIAN_POINT('Ctrl Pts',(-8.95902781007525,21.9351826698706,
4.05359376450294));
#101954=CARTESIAN_POINT('Ctrl Pts',(-8.98586914502017,21.931151211646,4.10135541725436));
#101955=CARTESIAN_POINT('Ctrl Pts',(-9.02480804608973,21.9260695019658,
4.16057286638449));
#101956=CARTESIAN_POINT('Ctrl Pts',(-9.03395780744671,21.9249217451991,
4.17388307301617));
#101957=CARTESIAN_POINT('Ctrl Pts',(-9.04966730272038,21.9230312281458,
4.19575789218673));
#101958=CARTESIAN_POINT('Ctrl Pts',(-9.05607592125321,21.9222807912769,
4.20442787731998));
#101959=CARTESIAN_POINT('Ctrl Pts',(-9.06511437510329,21.9212520129367,
4.21631078429671));
#101960=CARTESIAN_POINT('Ctrl Pts',(-9.06764326070904,21.9209672774621,
4.21959932139397));
#101961=CARTESIAN_POINT('Ctrl Pts',(-9.07195617667646,21.920486997575,4.22514688813352));
#101962=CARTESIAN_POINT('Ctrl Pts',(-9.07373119394163,21.9202908379102,
4.2274128449363));
#101963=CARTESIAN_POINT('Ctrl Pts',(-9.07715321574078,21.9199155716973,
4.23174850260919));
#101964=CARTESIAN_POINT('Ctrl Pts',(-9.07879890168456,21.9197363719713,
4.23381918420263));
#101965=CARTESIAN_POINT('Ctrl Pts',(-9.08276352632826,21.9193076465659,
4.23877331111639));
#101966=CARTESIAN_POINT('Ctrl Pts',(-9.08508912329468,21.9190585866078,
4.2416514292178));
#101967=CARTESIAN_POINT('Ctrl Pts',(-9.09359112434942,21.9181566263438,
4.25207250642525));
#101968=CARTESIAN_POINT('Ctrl Pts',(-9.09984776648703,21.9175091282161,
4.25954991706177));
#101969=CARTESIAN_POINT('Ctrl Pts',(-9.14630040786892,21.9128115822555,
4.31368587186263));
#101970=CARTESIAN_POINT('Ctrl Pts',(-9.19001369223749,21.9089783890553,
4.35721169676561));
#101971=CARTESIAN_POINT('Ctrl Pts',(-9.28770567613959,21.9010392725421,
4.44030531977779));
#101972=CARTESIAN_POINT('Ctrl Pts',(-9.34204561852476,21.8969476846134,
4.47909790200215));
#101973=CARTESIAN_POINT('Ctrl Pts',(-9.42916919979026,21.8905082673321,
4.53075075722707));
#101974=CARTESIAN_POINT('Ctrl Pts',(-9.45972751884151,21.8882716146272,
4.54709131037607));
#101975=CARTESIAN_POINT('Ctrl Pts',(-9.49917526252393,21.8853866947294,
4.56599843030483));
#101976=CARTESIAN_POINT('Ctrl Pts',(-9.50743643005745,21.8847827083907,
4.56984073250448));
#101977=CARTESIAN_POINT('Ctrl Pts',(-9.52078347699878,21.8838067607989,
4.57586113628776));
#101978=CARTESIAN_POINT('Ctrl Pts',(-9.52584168407093,21.8834368726653,
4.57809997224384));
#101979=CARTESIAN_POINT('Ctrl Pts',(-9.53550815665088,21.8827298541608,
4.58229730682978));
#101980=CARTESIAN_POINT('Ctrl Pts',(-9.54011351929205,21.8823929498681,
4.58426221756415));
#101981=CARTESIAN_POINT('Ctrl Pts',(-9.55067618437587,21.8816200265718,
4.58868945198816));
#101982=CARTESIAN_POINT('Ctrl Pts',(-9.55664140962897,21.8811833661382,
4.59113233460971));
#101983=CARTESIAN_POINT('Ctrl Pts',(-9.57518925560504,21.8798249885159,
4.59855085017303));
#101984=CARTESIAN_POINT('Ctrl Pts',(-9.58783740389136,21.8788977386115,
4.6033585576613));
#101985=CARTESIAN_POINT('Ctrl Pts',(-9.6959403248465,21.8709614747477,4.64233160564095));
#101986=CARTESIAN_POINT('Ctrl Pts',(-9.79533868790776,21.8635360269073,
4.66425041570765));
#101987=CARTESIAN_POINT('Ctrl Pts',(-9.95415924840633,21.8518392909558,
4.67829073224624));
#101988=CARTESIAN_POINT('Ctrl Pts',(-10.0123378697796,21.8476027582929,
4.67911823295361));
#101989=CARTESIAN_POINT('Ctrl Pts',(-10.0775621651369,21.8430541521517,
4.67521548465421));
#101990=CARTESIAN_POINT('Ctrl Pts',(-10.0847746276831,21.8425540039893,
4.6747172399784));
#101991=CARTESIAN_POINT('Ctrl Pts',(-10.0955053962565,21.8418145433738,
4.67387659930378));
#101992=CARTESIAN_POINT('Ctrl Pts',(-10.0990273227439,21.8415725954983,
4.67358473971121));
#101993=CARTESIAN_POINT('Ctrl Pts',(-10.1050618889919,21.8411593804347,
4.67305730047634));
#101994=CARTESIAN_POINT('Ctrl Pts',(-10.1075751374841,21.8409876892926,
4.67282949355771));
#101995=CARTESIAN_POINT('Ctrl Pts',(-10.1132808253094,21.8405988327509,
4.67229382109334));
#101996=CARTESIAN_POINT('Ctrl Pts',(-10.1164727512392,21.8403819455252,
4.67198099267715));
#101997=CARTESIAN_POINT('Ctrl Pts',(-10.1251505967325,21.8397939691701,
4.67109470750654));
#101998=CARTESIAN_POINT('Ctrl Pts',(-10.1306339149798,21.8394242602091,
4.67049573644395));
#101999=CARTESIAN_POINT('Ctrl Pts',(-10.1578046359435,21.8376004159884,
4.66733442426051));
#102000=CARTESIAN_POINT('Ctrl Pts',(-10.1794236259989,21.8361749103093,
4.66420757216516));
#102001=CARTESIAN_POINT('Ctrl Pts',(-10.222702197749,21.8333504808757,4.65671360904641));
#102002=CARTESIAN_POINT('Ctrl Pts',(-10.2443505002342,21.831952592415,4.65233483538477));
#102003=CARTESIAN_POINT('Ctrl Pts',(-10.3627757890489,21.8243265834302,
4.62489332615178));
#102004=CARTESIAN_POINT('Ctrl Pts',(-10.4564486897553,21.8183352226786,
4.59025059363022));
#102005=CARTESIAN_POINT('Ctrl Pts',(-10.5691322067729,21.8101904217924,
4.53147747594666));
#102006=CARTESIAN_POINT('Ctrl Pts',(-10.5931522809165,21.808397136702,4.51785432757466));
#102007=CARTESIAN_POINT('Ctrl Pts',(-10.6238724416345,21.8060155521596,
4.49897432634854));
#102008=CARTESIAN_POINT('Ctrl Pts',(-10.6310266925503,21.8054544839664,
4.49447063065251));
#102009=CARTESIAN_POINT('Ctrl Pts',(-10.64266020199,21.8045312049652,4.48697110243191));
#102010=CARTESIAN_POINT('Ctrl Pts',(-10.6471685645495,21.8041706750826,
4.48402080245969));
#102011=CARTESIAN_POINT('Ctrl Pts',(-10.6558652109445,21.8034698141119,
4.47824404771403));
#102012=CARTESIAN_POINT('Ctrl Pts',(-10.6600558685892,21.8031296290296,
4.47542136576162));
#102013=CARTESIAN_POINT('Ctrl Pts',(-10.6697185904393,21.8023394405889,
4.46882210816201));
#102014=CARTESIAN_POINT('Ctrl Pts',(-10.6751770520304,21.8018887095739,
4.46502601669752));
#102015=CARTESIAN_POINT('Ctrl Pts',(-10.6928687426397,21.8004133416613,
4.45249874025107));
#102016=CARTESIAN_POINT('Ctrl Pts',(-10.7049666077899,21.7993816065526,
4.44357988015936));
#102017=CARTESIAN_POINT('Ctrl Pts',(-10.7816628972542,21.7926886960074,
4.38473901599613));
#102018=CARTESIAN_POINT('Ctrl Pts',(-10.8410816839392,21.7867725861585,
4.32845458620045));
#102019=CARTESIAN_POINT('Ctrl Pts',(-10.9295621806644,21.7767945812469,
4.22523266426164));
#102020=CARTESIAN_POINT('Ctrl Pts',(-10.9620329983566,21.7727915361459,
4.18157270232591));
#102021=CARTESIAN_POINT('Ctrl Pts',(-11.0000593999272,21.7677416241228,
4.1222821666571));
#102022=CARTESIAN_POINT('Ctrl Pts',(-11.0084669995646,21.766598302739,4.10856245668405));
#102023=CARTESIAN_POINT('Ctrl Pts',(-11.0220193037739,21.7647142948109,
4.08539488592011));
#102024=CARTESIAN_POINT('Ctrl Pts',(-11.0273202899451,21.7639659951333,
4.0760413806091));
#102025=CARTESIAN_POINT('Ctrl Pts',(-11.0344862644481,21.7629396338561,
4.06298348298946));
#102026=CARTESIAN_POINT('Ctrl Pts',(-11.0364606939359,21.7626552166709,
4.05934020478251));
#102027=CARTESIAN_POINT('Ctrl Pts',(-11.0397735368128,21.7621753153193,
4.05314946844439));
#102028=CARTESIAN_POINT('Ctrl Pts',(-11.0411219062584,21.7619792181189,
4.0506074093977));
#102029=CARTESIAN_POINT('Ctrl Pts',(-11.0436922694824,21.7616039463091,
4.04571834340991));
#102030=CARTESIAN_POINT('Ctrl Pts',(-11.0449156833096,21.7614246792558,
4.04337213660475));
#102031=CARTESIAN_POINT('Ctrl Pts',(-11.0478327183914,21.7609956290836,
4.03773169584484));
#102032=CARTESIAN_POINT('Ctrl Pts',(-11.0495187396879,21.7607463132603,
4.03443353040128));
#102033=CARTESIAN_POINT('Ctrl Pts',(-11.055599397633,21.7598420704948,4.02239890020367));
#102034=CARTESIAN_POINT('Ctrl Pts',(-11.0599008853495,21.7591925826536,
4.01361544740916));
#102035=CARTESIAN_POINT('Ctrl Pts',(-11.0899349554065,21.7545782477769,
3.95030253735665));
#102036=CARTESIAN_POINT('Ctrl Pts',(-11.1115592611839,21.7508208994187,
3.8939143403414));
#102037=CARTESIAN_POINT('Ctrl Pts',(-11.1480598909885,21.7429008557308,
3.77133335846606));
#102038=CARTESIAN_POINT('Ctrl Pts',(-11.1617357242476,21.738754741515,3.70501902657362));
#102039=CARTESIAN_POINT('Ctrl Pts',(-11.1737361384073,21.7322404507094,
3.60323288527593));
#102040=CARTESIAN_POINT('Ctrl Pts',(-11.1762797282096,21.7299870019384,
3.56840456654972));
#102041=CARTESIAN_POINT('Ctrl Pts',(-11.1775328855013,21.7270831215993,
3.52438799562588));
#102042=CARTESIAN_POINT('Ctrl Pts',(-11.1776865905774,21.7264777052935,
3.51525638774523));
#102043=CARTESIAN_POINT('Ctrl Pts',(-11.1777628658049,21.7255000008533,
3.50058785196672));
#102044=CARTESIAN_POINT('Ctrl Pts',(-11.1777526159938,21.7251297994593,
3.49505152759654));
#102045=CARTESIAN_POINT('Ctrl Pts',(-11.1776587691406,21.7244225462642,
3.4845098335991));
#102046=CARTESIAN_POINT('Ctrl Pts',(-11.1775822923772,21.7240857230801,
3.47950450938479));
#102047=CARTESIAN_POINT('Ctrl Pts',(-11.1773345385335,21.7233135020717,
3.46806441387532));
#102048=CARTESIAN_POINT('Ctrl Pts',(-11.1771424130771,21.7228774669752,
3.46163030151686));
#102049=CARTESIAN_POINT('Ctrl Pts',(-11.1763846681915,21.7215229929797,
3.44172511825552));
#102050=CARTESIAN_POINT('Ctrl Pts',(-11.1756404777487,21.7205990670929,
3.4282623517072));
#102051=CARTESIAN_POINT('Ctrl Pts',(-11.1673054868669,21.712640992128,3.31332524974692));
#102052=CARTESIAN_POINT('Ctrl Pts',(-11.1468247047791,21.7051868421417,
3.21323517264621));
#102053=CARTESIAN_POINT('Ctrl Pts',(-11.0949534582972,21.6934844066775,
3.06237657518924));
#102054=CARTESIAN_POINT('Ctrl Pts',(-11.0721530844793,21.6892696002597,
3.00915716045355));
#102055=CARTESIAN_POINT('Ctrl Pts',(-11.0422085638946,21.684741537234,2.95141225303632));
#102056=CARTESIAN_POINT('Ctrl Pts',(-11.0388253390069,21.6842419624985,
2.94503231773434));
#102057=CARTESIAN_POINT('Ctrl Pts',(-11.0337000424018,21.6835031807407,
2.93557838272303));
#102058=CARTESIAN_POINT('Ctrl Pts',(-11.032002552061,21.6832613451691,2.93248059674107));
#102059=CARTESIAN_POINT('Ctrl Pts',(-11.0290685811872,21.6828482551897,
2.92718302660301));
#102060=CARTESIAN_POINT('Ctrl Pts',(-11.0278389432434,21.6826765775692,
2.92497953341313));
#102061=CARTESIAN_POINT('Ctrl Pts',(-11.0250298177703,21.6822876613856,
2.91998342431266));
#102062=CARTESIAN_POINT('Ctrl Pts',(-11.0234459957428,21.6820707015592,
2.91719329978942));
#102063=CARTESIAN_POINT('Ctrl Pts',(-11.0191059142591,21.6814823347117,
2.90961989028381));
#102064=CARTESIAN_POINT('Ctrl Pts',(-11.01632735048,21.6811123109142,2.90484938203497));
#102065=CARTESIAN_POINT('Ctrl Pts',(-11.0023628099584,21.6792843822694,
2.88125671805755));
#102066=CARTESIAN_POINT('Ctrl Pts',(-10.990686216488,21.6778552604976,2.86272814221592));
#102067=CARTESIAN_POINT('Ctrl Pts',(-10.96621566679,21.6750281030935,2.82619775654785));
#102068=CARTESIAN_POINT('Ctrl Pts',(-10.9534187904661,21.6736309723582,
2.80820892944009));
#102069=CARTESIAN_POINT('Ctrl Pts',(-10.8801490287803,21.6660004258613,
2.71111054368101));
#102070=CARTESIAN_POINT('Ctrl Pts',(-10.8103410218032,21.6600037390744,
2.63956011151695));
#102071=CARTESIAN_POINT('Ctrl Pts',(-10.710833322145,21.6518596486799,2.560549759865));
#102072=CARTESIAN_POINT('Ctrl Pts',(-10.6887140681461,21.6500738265903,
2.54421576256108));
#102073=CARTESIAN_POINT('Ctrl Pts',(-10.6590832186332,21.6477007717478,
2.52389773705692));
#102074=CARTESIAN_POINT('Ctrl Pts',(-10.6520705008869,21.6471405208899,
2.519199116786));
#102075=CARTESIAN_POINT('Ctrl Pts',(-10.6405022230419,21.6462182430471,
2.5116271122258));
#102076=CARTESIAN_POINT('Ctrl Pts',(-10.635976305133,21.6458578898257,2.50870882144673));
#102077=CARTESIAN_POINT('Ctrl Pts',(-10.6271645184658,21.6451571259854,
2.50311220786298));
#102078=CARTESIAN_POINT('Ctrl Pts',(-10.6228811040013,21.6448168597622,
2.5004302264277));
#102079=CARTESIAN_POINT('Ctrl Pts',(-10.6129169555056,21.6440261189539,
2.49428027520603));
#102080=CARTESIAN_POINT('Ctrl Pts',(-10.6072238673351,21.6435749135678,
2.49083275372079));
#102081=CARTESIAN_POINT('Ctrl Pts',(-10.588546741144,21.6420963723018,2.47973784719996));
#102082=CARTESIAN_POINT('Ctrl Pts',(-10.5754455657394,21.6410618957317,
2.4722916312653));
#102083=CARTESIAN_POINT('Ctrl Pts',(-10.4919220581323,21.6344803743921,
2.42691782964652));
#102084=CARTESIAN_POINT('Ctrl Pts',(-10.417944416415,21.6286896827707,2.39600237227468));
#102085=CARTESIAN_POINT('Ctrl Pts',(-10.2882084112286,21.6187433255133,
2.35670553029678));
#102086=CARTESIAN_POINT('Ctrl Pts',(-10.2339198405707,21.614645101014,2.34437531602081));
#102087=CARTESIAN_POINT('Ctrl Pts',(-10.1628597976156,21.6094887866822,
2.33345075892763));
#102088=CARTESIAN_POINT('Ctrl Pts',(-10.1467078797446,21.6083307151759,
2.33130957908645));
#102089=CARTESIAN_POINT('Ctrl Pts',(-10.1197322636978,21.606425073981,2.32830166828272));
#102090=CARTESIAN_POINT('Ctrl Pts',(-10.1089320173734,21.6056696792347,
2.32724826488207));
#102091=CARTESIAN_POINT('Ctrl Pts',(-10.0939738268989,21.6046352969177,
2.32599775173931));
#102092=CARTESIAN_POINT('Ctrl Pts',(-10.0898274850354,21.6043498258082,
2.32567322123748));
#102093=CARTESIAN_POINT('Ctrl Pts',(-10.0828066694807,21.6038686705337,
2.32516111118792));
#102094=CARTESIAN_POINT('Ctrl Pts',(-10.0799330934752,21.6036723659857,
2.32496210256212));
#102095=CARTESIAN_POINT('Ctrl Pts',(-10.0744218041311,21.6032971104566,
2.32460073125346));
#102096=CARTESIAN_POINT('Ctrl Pts',(-10.0717842465693,21.6031180646089,
2.3244367017482));
#102097=CARTESIAN_POINT('Ctrl Pts',(-10.0654611566832,21.6026900827338,
2.32406482940919));
#102098=CARTESIAN_POINT('Ctrl Pts',(-10.0617751268381,21.6024416088264,
2.32386543155666));
#102099=CARTESIAN_POINT('Ctrl Pts',(-10.0484195788042,21.60154480173,2.32320591593911));
#102100=CARTESIAN_POINT('Ctrl Pts',(-10.0387450939451,21.6009017880161,
2.32284767149286));
#102101=CARTESIAN_POINT('Ctrl Pts',(-9.96163517026617,21.595821520519,2.32094401604707));
#102102=CARTESIAN_POINT('Ctrl Pts',(-9.89417523585574,21.5916457831624,
2.32507510158336));
#102103=CARTESIAN_POINT('Ctrl Pts',(-9.82198378129026,21.5871330419721,
2.33576822427561));
#102104=CARTESIAN_POINT('Ctrl Pts',(-9.81654085550856,21.5867925610894,
2.33661350190372));
#102105=CARTESIAN_POINT('Ctrl Pts',(-9.81110406371016,21.5864520766487,
2.33749693000268));
#102106=CARTESIAN_POINT('Ctrl Pts',(-9.81110407243713,21.4868028556135,
2.33749692858463));
#102107=CARTESIAN_POINT('Ctrl Pts',(-9.81517067467535,21.4870722770751,
2.33683614357623));
#102108=CARTESIAN_POINT('Ctrl Pts',(-9.81924120982507,21.4873423546502,
2.33619662123157));
#102109=CARTESIAN_POINT('Ctrl Pts',(-9.83303428352159,21.4882589494198,
2.33410371765976));
#102110=CARTESIAN_POINT('Ctrl Pts',(-9.84277088387619,21.4889083879988,
2.33275080332901));
#102111=CARTESIAN_POINT('Ctrl Pts',(-9.8587378479823,21.4899778809616,2.33073557055172));
#102112=CARTESIAN_POINT('Ctrl Pts',(-9.86495870835362,21.4903956735842,
2.33000079121547));
#102113=CARTESIAN_POINT('Ctrl Pts',(-9.87614085585395,21.4911487887447,
2.32877037586977));
#102114=CARTESIAN_POINT('Ctrl Pts',(-9.88110002354407,21.4914835355677,
2.32825654927539));
#102115=CARTESIAN_POINT('Ctrl Pts',(-9.89167004103714,21.4921986798962,
2.32722916687655));
#102116=CARTESIAN_POINT('Ctrl Pts',(-9.8972815953929,21.4925793412509,2.32672435699143));
#102117=CARTESIAN_POINT('Ctrl Pts',(-9.91244938790626,21.4936110516241,
2.32546952546572));
#102118=CARTESIAN_POINT('Ctrl Pts',(-9.92201134098397,21.4942644542814,
2.32479588798927));
#102119=CARTESIAN_POINT('Ctrl Pts',(-9.97262803496219,21.4977399671803,
2.32185040525782));
#102120=CARTESIAN_POINT('Ctrl Pts',(-10.0137679521485,21.5006242779217,
2.32161320888497));
#102121=CARTESIAN_POINT('Ctrl Pts',(-10.1588035758424,21.511005580528,2.32837290664097));
#102122=CARTESIAN_POINT('Ctrl Pts',(-10.2616586579371,21.518802440347,2.34697807224981));
#102123=CARTESIAN_POINT('Ctrl Pts',(-10.3830147408723,21.5279392074216,
2.38602373832498));
#102124=CARTESIAN_POINT('Ctrl Pts',(-10.4050890730134,21.5295958415547,
2.3938596713672));
#102125=CARTESIAN_POINT('Ctrl Pts',(-10.4321713656941,21.5316097259848,
2.4043929715578));
#102126=CARTESIAN_POINT('Ctrl Pts',(-10.4374113586635,21.5319984981899,
2.40647443715146));
#102127=CARTESIAN_POINT('Ctrl Pts',(-10.4456337560816,21.5326069290953,
2.40980915418591));
#102128=CARTESIAN_POINT('Ctrl Pts',(-10.4486262053365,21.5328280218014,
2.41103716620755));
#102129=CARTESIAN_POINT('Ctrl Pts',(-10.4539394730286,21.533219932796,2.41324319208894));
#102130=CARTESIAN_POINT('Ctrl Pts',(-10.4562622058674,21.53339103251,2.41421631785437));
#102131=CARTESIAN_POINT('Ctrl Pts',(-10.4617984758005,21.5337983263239,
2.41655668087407));
#102132=CARTESIAN_POINT('Ctrl Pts',(-10.4650090696985,21.5340341059273,
2.41793076751005));
#102133=CARTESIAN_POINT('Ctrl Pts',(-10.4746577872373,21.5347415660773,
2.42211115092003));
#102134=CARTESIAN_POINT('Ctrl Pts',(-10.4810771105898,21.5352107312872,
2.42496083532509));
#102135=CARTESIAN_POINT('Ctrl Pts',(-10.4958657975622,21.5362889463584,
2.43168486873679));
#102136=CARTESIAN_POINT('Ctrl Pts',(-10.504216016322,21.5368957720601,2.43560048402255));
#102137=CARTESIAN_POINT('Ctrl Pts',(-10.610265072029,21.544588056823,2.48685750011809));
#102138=CARTESIAN_POINT('Ctrl Pts',(-10.7010211253718,21.5510541319297,
2.54739445712384));
#102139=CARTESIAN_POINT('Ctrl Pts',(-10.8175293886042,21.5608412143302,
2.65089858870542));
#102140=CARTESIAN_POINT('Ctrl Pts',(-10.8509281605442,21.5638591628275,
2.68437265775023));
#102141=CARTESIAN_POINT('Ctrl Pts',(-10.8889929303099,21.5676385469017,
2.72741276953132));
#102142=CARTESIAN_POINT('Ctrl Pts',(-10.895661765706,21.5683145195203,2.73515397008703));
#102143=CARTESIAN_POINT('Ctrl Pts',(-10.9059777810372,21.5693828140017,
2.74744877896466));
#102144=CARTESIAN_POINT('Ctrl Pts',(-10.9096933918586,21.569772357924,2.75194451358904));
#102145=CARTESIAN_POINT('Ctrl Pts',(-10.9161986784941,21.5704629701072,
2.75993578435973));
#102146=CARTESIAN_POINT('Ctrl Pts',(-10.91900214559,21.5707634784891,2.76341998588178));
#102147=CARTESIAN_POINT('Ctrl Pts',(-10.9253936401151,21.5714553237191,
2.77145674623781));
#102148=CARTESIAN_POINT('Ctrl Pts',(-10.928968013463,21.5718471905044,2.77601996598856));
#102149=CARTESIAN_POINT('Ctrl Pts',(-10.938820813771,21.5729414296021,2.7887916354707));
#102150=CARTESIAN_POINT('Ctrl Pts',(-10.9450249768115,21.5736466665227,
2.7970564464425));
#102151=CARTESIAN_POINT('Ctrl Pts',(-10.9839092432363,21.5781731378335,
2.85030099869168));
#102152=CARTESIAN_POINT('Ctrl Pts',(-11.0134735994954,21.5821113117776,
2.89745889831677));
#102153=CARTESIAN_POINT('Ctrl Pts',(-11.0782934478732,21.59209333158,3.01920956130157));
#102154=CARTESIAN_POINT('Ctrl Pts',(-11.1092601515494,21.5982219388943,
3.09575101075284));
#102155=CARTESIAN_POINT('Ctrl Pts',(-11.1398953365033,21.6062232699944,
3.20241999968618));
#102156=CARTESIAN_POINT('Ctrl Pts',(-11.1467948879311,21.6082599998995,
3.23022782064838));
#102157=CARTESIAN_POINT('Ctrl Pts',(-11.1537939556788,21.610625814954,3.2636013268679));
#102158=CARTESIAN_POINT('Ctrl Pts',(-11.1548766312647,21.6110024898336,
3.26894850305121));
#102159=CARTESIAN_POINT('Ctrl Pts',(-11.1565889857464,21.6116161724631,
3.2777184452769));
#102160=CARTESIAN_POINT('Ctrl Pts',(-11.1572407050726,21.6118543523878,
3.2811367485556));
#102161=CARTESIAN_POINT('Ctrl Pts',(-11.1583871701761,21.6122817857458,
3.28729833986086));
#102162=CARTESIAN_POINT('Ctrl Pts',(-11.1588873335337,21.6124713344613,
3.29004052555067));
#102163=CARTESIAN_POINT('Ctrl Pts',(-11.159968681859,21.6128880482592,3.29609070786868));
#102164=CARTESIAN_POINT('Ctrl Pts',(-11.1605454544756,21.6131149649992,
3.29939942393878));
#102165=CARTESIAN_POINT('Ctrl Pts',(-11.162175349159,21.6137701242357,3.30899185014391));
#102166=CARTESIAN_POINT('Ctrl Pts',(-11.163191666558,21.6141963706911,3.31528181774291));
#102167=CARTESIAN_POINT('Ctrl Pts',(-11.1708052012482,21.6175385550112,
3.36495866976929));
#102168=CARTESIAN_POINT('Ctrl Pts',(-11.1750245704109,21.6203351253198,
3.40868077583424));
#102169=CARTESIAN_POINT('Ctrl Pts',(-11.1810212841267,21.6296605105556,
3.5573764098261));
#102170=CARTESIAN_POINT('Ctrl Pts',(-11.1712224620157,21.6359739337432,
3.66230061828851));
#102171=CARTESIAN_POINT('Ctrl Pts',(-11.1427639967321,21.6441500726106,
3.78576171668288));
#102172=CARTESIAN_POINT('Ctrl Pts',(-11.1372851304337,21.6455712800106,
3.80684156451089));
#102173=CARTESIAN_POINT('Ctrl Pts',(-11.1289953473737,21.6475408609851,
3.83545309690688));
#102174=CARTESIAN_POINT('Ctrl Pts',(-11.1266868932461,21.6480731358535,
3.84312667327583));
#102175=CARTESIAN_POINT('Ctrl Pts',(-11.1228817617851,21.648925834145,3.85532280813239));
#102176=CARTESIAN_POINT('Ctrl Pts',(-11.1214356110884,21.6492446147442,
3.85986097034221));
#102177=CARTESIAN_POINT('Ctrl Pts',(-11.11840386614,21.6499023019012,3.86917911144047));
#102178=CARTESIAN_POINT('Ctrl Pts',(-11.1168150632454,21.6502413073615,
3.87395793516264));
#102179=CARTESIAN_POINT('Ctrl Pts',(-11.1130516254508,21.6510314954133,
3.88503973466421));
#102180=CARTESIAN_POINT('Ctrl Pts',(-11.1108540353886,21.6514834221491,
3.89133467399603));
#102181=CARTESIAN_POINT('Ctrl Pts',(-11.1036283972482,21.6529398350791,
3.91148093559938));
#102182=CARTESIAN_POINT('Ctrl Pts',(-11.0983939751393,21.6539510682763,
3.92525620591153));
#102183=CARTESIAN_POINT('Ctrl Pts',(-11.0854761480399,21.656349756588,3.95742068839113));
#102184=CARTESIAN_POINT('Ctrl Pts',(-11.0775819024816,21.6577438510636,
3.97571978771312));
#102185=CARTESIAN_POINT('Ctrl Pts',(-11.0282503144281,21.6660583343638,
4.08253579514326));
#102186=CARTESIAN_POINT('Ctrl Pts',(-10.9763910342186,21.6733139826275,
4.16580921944011));
#102187=CARTESIAN_POINT('Ctrl Pts',(-10.8890482099523,21.6834155845373,
4.27354262799605));
#102188=CARTESIAN_POINT('Ctrl Pts',(-10.8615892249823,21.686363070088,4.30401473160558));
#102189=CARTESIAN_POINT('Ctrl Pts',(-10.8283880077875,21.689625156212,4.33719993858729));
#102190=CARTESIAN_POINT('Ctrl Pts',(-10.8241499786093,21.690036280962,4.34137223929261));
#102191=CARTESIAN_POINT('Ctrl Pts',(-10.8173039659384,21.6906917487054,
4.34801071314387));
#102192=CARTESIAN_POINT('Ctrl Pts',(-10.8147160638966,21.6909375751822,
4.35049731242162));
#102193=CARTESIAN_POINT('Ctrl Pts',(-10.8100893005367,21.691373551303,4.35490246505053));
#102194=CARTESIAN_POINT('Ctrl Pts',(-10.8080549189143,21.6915640472247,
4.35682562300048));
#102195=CARTESIAN_POINT('Ctrl Pts',(-10.8036578351873,21.6919731877646,
4.36095271960525));
#102196=CARTESIAN_POINT('Ctrl Pts',(-10.8012929136054,21.6921916486279,
4.36315419751851));
#102197=CARTESIAN_POINT('Ctrl Pts',(-10.7946765873179,21.6927985207113,
4.36926263114877));
#102198=CARTESIAN_POINT('Ctrl Pts',(-10.790405395359,21.6931853643033,4.37314816309634));
#102199=CARTESIAN_POINT('Ctrl Pts',(-10.7648714480178,21.6954701744423,
4.39603565506007));
#102200=CARTESIAN_POINT('Ctrl Pts',(-10.7429508840491,21.6973182610938,
4.41429345348561));
#102201=CARTESIAN_POINT('Ctrl Pts',(-10.6598333726941,21.7040125223968,
4.47855692282397));
#102202=CARTESIAN_POINT('Ctrl Pts',(-10.5948562291706,21.7086610917834,
4.519363253048));
#102203=CARTESIAN_POINT('Ctrl Pts',(-10.4717687882584,21.7172236408201,
4.58085861958815));
#102204=CARTESIAN_POINT('Ctrl Pts',(-10.4151318874035,21.7210809082755,
4.60385015494241));
#102205=CARTESIAN_POINT('Ctrl Pts',(-10.3476362889929,21.7257346768253,
4.62531776545494));
#102206=CARTESIAN_POINT('Ctrl Pts',(-10.3382627663802,21.7263820325624,
4.62817080004644));
#102207=CARTESIAN_POINT('Ctrl Pts',(-10.3228493119951,21.7274487880799,
4.63265286029768));
#102208=CARTESIAN_POINT('Ctrl Pts',(-10.3168299435071,21.7278659459502,
4.63435134087523));
#102209=CARTESIAN_POINT('Ctrl Pts',(-10.3059892919184,21.7286183692001,
4.63731722238255));
#102210=CARTESIAN_POINT('Ctrl Pts',(-10.3011729165265,21.7289530633027,
4.63860211844908));
#102211=CARTESIAN_POINT('Ctrl Pts',(-10.2908895782006,21.7296685847242,
4.64127565950245));
#102212=CARTESIAN_POINT('Ctrl Pts',(-10.2854205228723,21.7300496790276,
4.64265567905805));
#102213=CARTESIAN_POINT('Ctrl Pts',(-10.270603132418,21.7310837896781,4.64628157147354));
#102214=CARTESIAN_POINT('Ctrl Pts',(-10.2612370354732,21.7317391784714,
4.64845230554885));
#102215=CARTESIAN_POINT('Ctrl Pts',(-10.2112493153471,21.7352470558314,
4.65939459278967));
#102216=CARTESIAN_POINT('Ctrl Pts',(-10.1702159203195,21.7381631471894,
4.66612516795698));
#102217=CARTESIAN_POINT('Ctrl Pts',(-10.0215775472286,21.748859530898,4.68249350971822));
#102218=CARTESIAN_POINT('Ctrl Pts',(-9.91313845917287,21.7569666946326,
4.67949465745268));
#102219=CARTESIAN_POINT('Ctrl Pts',(-9.78727160619767,21.7660655985922,
4.65854519447687));
#102220=CARTESIAN_POINT('Ctrl Pts',(-9.76799169907782,21.7674484957347,
4.65483877525444));
#102221=CARTESIAN_POINT('Ctrl Pts',(-9.74355635270306,21.7691800072668,
4.6495045271145));
#102222=CARTESIAN_POINT('Ctrl Pts',(-9.73830836911851,21.769550627205,4.6483211637927));
#102223=CARTESIAN_POINT('Ctrl Pts',(-9.73000585443508,21.7701347720265,
4.64638916250692));
#102224=CARTESIAN_POINT('Ctrl Pts',(-9.72694597658911,21.7703495845633,
4.64566419663078));
#102225=CARTESIAN_POINT('Ctrl Pts',(-9.72114922999216,21.770755588289,4.64426625110816));
#102226=CARTESIAN_POINT('Ctrl Pts',(-9.71841189973956,21.7709469039492,
4.64359570973499));
#102227=CARTESIAN_POINT('Ctrl Pts',(-9.71198796305757,21.7713949657094,
4.64199762681728));
#102228=CARTESIAN_POINT('Ctrl Pts',(-9.70830340620653,21.7716512529751,
4.64106205408025));
#102229=CARTESIAN_POINT('Ctrl Pts',(-9.69623647694154,21.7724884717113,
4.63793578290126));
#102230=CARTESIAN_POINT('Ctrl Pts',(-9.68787350053225,21.7730653395749,
4.63567036730967));
#102231=CARTESIAN_POINT('Ctrl Pts',(-9.64216108551712,21.7762038879674,
4.62274438232728));
#102232=CARTESIAN_POINT('Ctrl Pts',(-9.60532767950584,21.7786793262564,
4.61033240357154));
#102233=CARTESIAN_POINT('Ctrl Pts',(-9.48377213901692,21.7868737948191,
4.56255521807392));
#102234=CARTESIAN_POINT('Ctrl Pts',(-9.40258964468741,21.7924140098975,
4.51912522269836));
#102235=CARTESIAN_POINT('Ctrl Pts',(-9.29970956773928,21.8003863660617,
4.44753142954271));
#102236=CARTESIAN_POINT('Ctrl Pts',(-9.27298399161936,21.8025545923064,
4.42718385170613));
#102237=CARTESIAN_POINT('Ctrl Pts',(-9.23992868811659,21.805387415021,4.39970841119374));
#102238=CARTESIAN_POINT('Ctrl Pts',(-9.23276410357852,21.8060109662452,
4.39360656615301));
#102239=CARTESIAN_POINT('Ctrl Pts',(-9.22145705306379,21.8070108736661,
4.38374049225568));
#102240=CARTESIAN_POINT('Ctrl Pts',(-9.21726686606795,21.8073849667075,
4.38003137278449));
#102241=CARTESIAN_POINT('Ctrl Pts',(-9.20976067198723,21.8080616300315,
4.37329093106037));
#102242=CARTESIAN_POINT('Ctrl Pts',(-9.20643525465463,21.8083637542896,
4.37027021079243));
#102243=CARTESIAN_POINT('Ctrl Pts',(-9.1986493395123,21.8090767345027,4.3631159615435));
#102244=CARTESIAN_POINT('Ctrl Pts',(-9.19420344822566,21.8094882463053,
4.358966797307));
#102245=CARTESIAN_POINT('Ctrl Pts',(-9.18130597622644,21.810695095343,4.34674187503279));
#102246=CARTESIAN_POINT('Ctrl Pts',(-9.17294246221775,21.8114943316774,
4.33857469526382));
#102247=CARTESIAN_POINT('Ctrl Pts',(-9.1095662534862,21.817682511737,4.27481582433907));
#102248=CARTESIAN_POINT('Ctrl Pts',(-9.06010306459542,21.8233106859232,
4.21400368632121));
#102249=CARTESIAN_POINT('Ctrl Pts',(-8.97226763976339,21.8349916141909,
4.0809190027683));
#102250=CARTESIAN_POINT('Ctrl Pts',(-8.93463676396819,21.8410194355429,
4.00862942113423));
#102251=CARTESIAN_POINT('Ctrl Pts',(-8.90144387380693,21.8473341975225,
3.92467670187064));
#102252=CARTESIAN_POINT('Ctrl Pts',(-8.89823449662909,21.8479583939721,
3.91627953511174));
#102253=CARTESIAN_POINT('Ctrl Pts',(-8.8938860077113,21.8488229573773,3.90449922950167));
#102254=CARTESIAN_POINT('Ctrl Pts',(-8.89266575158476,21.8490677552318,
3.90114667358498));
#102255=CARTESIAN_POINT('Ctrl Pts',(-8.89057913328366,21.8494901282862,
3.89533177967653));
#102256=CARTESIAN_POINT('Ctrl Pts',(-8.88970569660362,21.8496681101149,
3.89287203478302));
#102257=CARTESIAN_POINT('Ctrl Pts',(-8.88787518624191,21.8500436081635,
3.88766214684093));
#102258=CARTESIAN_POINT('Ctrl Pts',(-8.88692012020401,21.8502410015256,
3.88491131839937));
#102259=CARTESIAN_POINT('Ctrl Pts',(-8.88457397826253,21.8507296778961,
3.87807208596694));
#102260=CARTESIAN_POINT('Ctrl Pts',(-8.88319515144265,21.8510202528708,
3.87397946983578));
#102261=CARTESIAN_POINT('Ctrl Pts',(-8.87808248896295,21.8521109793721,
3.85852366875419));
#102262=CARTESIAN_POINT('Ctrl Pts',(-8.87449915973305,21.8529029129152,
3.84711094567244));
#102263=CARTESIAN_POINT('Ctrl Pts',(-8.86579037159797,21.8549059325265,
3.81781977636356));
#102264=CARTESIAN_POINT('Ctrl Pts',(-8.86091321640439,21.8561055901371,
3.79987042147051));
#102265=CARTESIAN_POINT('Ctrl Pts',(-8.84014576814355,21.8616411204594,
3.71560027741768));
#102266=CARTESIAN_POINT('Ctrl Pts',(-8.82960884258752,21.8658049433229,
3.64809185660545));
#102267=CARTESIAN_POINT('Ctrl Pts',(-8.82021655868084,21.8743716551814,
3.5102204745359));
#102268=CARTESIAN_POINT('Ctrl Pts',(-8.82169371835029,21.8787637077503,
3.44011888749817));
#102269=CARTESIAN_POINT('Ctrl Pts',(-8.83047251192312,21.8840111599051,
3.36072085320286));
#102270=CARTESIAN_POINT('Ctrl Pts',(-8.83168553988959,21.8846656509144,
3.35088749681665));
#102271=CARTESIAN_POINT('Ctrl Pts',(-8.83387092222589,21.8857417822387,
3.3348407729421));
#102272=CARTESIAN_POINT('Ctrl Pts',(-8.83476925136269,21.8861611123166,
3.32861769007663));
#102273=CARTESIAN_POINT('Ctrl Pts',(-8.83646950996575,21.8869159084852,
3.31747125933727));
#102274=CARTESIAN_POINT('Ctrl Pts',(-8.83725297494085,21.8872507881111,
3.31254521395774));
#102275=CARTESIAN_POINT('Ctrl Pts',(-8.83898556986418,21.8879650437512,
3.30208048989017));
#102276=CARTESIAN_POINT('Ctrl Pts',(-8.83994309288268,21.8883446761303,
3.29654334658551));
#102277=CARTESIAN_POINT('Ctrl Pts',(-8.84254252260718,21.8893376479344,
3.28212666247222));
#102278=CARTESIAN_POINT('Ctrl Pts',(-8.84424696501407,21.8899529416023,
3.27325891994445));
#102279=CARTESIAN_POINT('Ctrl Pts',(-8.85269301864736,21.8928452054921,
3.23188885348993));
#102280=CARTESIAN_POINT('Ctrl Pts',(-8.86070420168162,21.8951617938466,
3.19966418467643));
#102281=CARTESIAN_POINT('Ctrl Pts',(-8.88870130724449,21.9022050723872,
3.10442895038725));
#102282=CARTESIAN_POINT('Ctrl Pts',(-8.91263795038509,21.9070402854017,
3.04272201003186));
#102283=CARTESIAN_POINT('Ctrl Pts',(-8.96938470451807,21.9165394902133,
2.92647254558138));
#102284=CARTESIAN_POINT('Ctrl Pts',(-9.00169479759932,21.9211851039395,
2.87191564100453));
#102285=CARTESIAN_POINT('Ctrl Pts',(-9.0438761486563,21.9263063678553,2.812237172837));
#102286=CARTESIAN_POINT('Ctrl Pts',(-9.04961488367065,21.9269857585909,
2.80432861797643));
#102287=CARTESIAN_POINT('Ctrl Pts',(-9.05766297932109,21.9279140265319,
2.79352303123261));
#102288=CARTESIAN_POINT('Ctrl Pts',(-9.05988837889258,21.9281681942064,
2.79056437308831));
#102289=CARTESIAN_POINT('Ctrl Pts',(-9.06372754037962,21.9286023272908,
2.78551001455653));
#102290=CARTESIAN_POINT('Ctrl Pts',(-9.06533446140725,21.928782752519,2.78340918979952));
#102291=CARTESIAN_POINT('Ctrl Pts',(-9.06870384169119,21.929158363504,2.77903481151096));
#102292=CARTESIAN_POINT('Ctrl Pts',(-9.07046757049206,21.929353451293,2.77676227958919));
#102293=CARTESIAN_POINT('Ctrl Pts',(-9.07479172303867,21.9298280969713,
2.77123263596257));
#102294=CARTESIAN_POINT('Ctrl Pts',(-9.07736107365033,21.9301070350908,
2.76798248687196));
#102295=CARTESIAN_POINT('Ctrl Pts',(-9.08644150371859,21.9310823360061,
2.75661978685024));
#102296=CARTESIAN_POINT('Ctrl Pts',(-9.09304308694545,21.9317726568497,
2.74857971568812));
#102297=CARTESIAN_POINT('Ctrl Pts',(-9.13127426651407,21.9356723478917,
2.70325596330276));
#102298=CARTESIAN_POINT('Ctrl Pts',(-9.16509833814906,21.9387493355969,
2.66787873877219));
#102299=CARTESIAN_POINT('Ctrl Pts',(-9.23675336229815,21.9448151996094,
2.60171600829347));
#102300=CARTESIAN_POINT('Ctrl Pts',(-9.27448774359679,21.9477991712231,
2.57097277677265));
#102301=CARTESIAN_POINT('Ctrl Pts',(-9.36390976967964,21.9546438464068,
2.5068977748864));
#102302=CARTESIAN_POINT('Ctrl Pts',(-9.41651685434449,21.9585215953546,
2.47510551062792));
#102303=CARTESIAN_POINT('Ctrl Pts',(-9.48011907270479,21.9631981330904,
2.44315799207569));
#102304=CARTESIAN_POINT('Ctrl Pts',(-9.48893559984864,21.9638459716114,
2.43886646567031));
#102305=CARTESIAN_POINT('Ctrl Pts',(-9.5034638314767,21.9649133616857,2.43201777090185));
#102306=CARTESIAN_POINT('Ctrl Pts',(-9.50914426702402,21.9653306667345,
2.42939509847233));
#102307=CARTESIAN_POINT('Ctrl Pts',(-9.51938767883757,21.9660832503043,
2.42476434680652));
#102308=CARTESIAN_POINT('Ctrl Pts',(-9.52394304996281,21.9664179565195,
2.42273972868125));
#102309=CARTESIAN_POINT('Ctrl Pts',(-9.53367852607802,21.967133389966,2.41848664170061));
#102310=CARTESIAN_POINT('Ctrl Pts',(-9.53886204128283,21.9675143834526,
2.41626634160683));
#102311=CARTESIAN_POINT('Ctrl Pts',(-9.54946689300735,21.9682940791329,
2.41181373166932));
#102312=CARTESIAN_POINT('Ctrl Pts',(-9.55488934683647,21.968692872576,2.40958451067744));
#102313=CARTESIAN_POINT('Ctrl Pts',(-9.56852944595827,21.9696964304524,
2.40409563520672));
#102314=CARTESIAN_POINT('Ctrl Pts',(-9.57676745552589,21.9703028971545,
2.4008878939507));
#102315=CARTESIAN_POINT('Ctrl Pts',(-9.65822383938616,21.9763040950047,
2.37022170619078));
#102316=CARTESIAN_POINT('Ctrl Pts',(-9.73394555776837,21.9819386115451,
2.350034469155));
#102317=CARTESIAN_POINT('Ctrl Pts',(-9.81110406961726,21.9876672748128,
2.33749692904284));
#102318=CARTESIAN_POINT('Origin',(-10.,12.3756328852638,3.5));
#102319=CARTESIAN_POINT('',(-9.81110404738689,22.5875279348072,2.33749693265506));
#102320=CARTESIAN_POINT('',(-9.81110406371112,22.4887934941609,2.33749693000253));
#102321=CARTESIAN_POINT('',(-9.81110406371068,12.3756328852638,2.3374969300026));
#102322=CARTESIAN_POINT('Ctrl Pts',(-9.81111389378217,22.5875286339524,
2.33749533275007));
#102323=CARTESIAN_POINT('Ctrl Pts',(-9.72555949551518,22.5814538128317,
2.35139712794946));
#102324=CARTESIAN_POINT('Ctrl Pts',(-9.64181293403421,22.5750945898088,
2.37469770477806));
#102325=CARTESIAN_POINT('Ctrl Pts',(-9.50651574673404,22.5643975402355,
2.42898871694999));
#102326=CARTESIAN_POINT('Ctrl Pts',(-9.45336513184311,22.5600820943743,
2.45511538686148));
#102327=CARTESIAN_POINT('Ctrl Pts',(-9.39614249259326,22.5554589601237,
2.4888106712376));
#102328=CARTESIAN_POINT('Ctrl Pts',(-9.38992182114609,22.5549567624739,
2.49255155457603));
#102329=CARTESIAN_POINT('Ctrl Pts',(-9.38071951120628,22.5542148761943,
2.49820198242319));
#102330=CARTESIAN_POINT('Ctrl Pts',(-9.37771139781822,22.5539725275117,
2.50006775817275));
#102331=CARTESIAN_POINT('Ctrl Pts',(-9.37257263360514,22.5535588655669,
2.50328723598973));
#102332=CARTESIAN_POINT('Ctrl Pts',(-9.37043787747973,22.5533871257053,
2.50463425396613));
#102333=CARTESIAN_POINT('Ctrl Pts',(-9.36560386870875,22.5529984797386,
2.50770625717497));
#102334=CARTESIAN_POINT('Ctrl Pts',(-9.36290731249977,22.5527818498101,
2.50943539756362));
#102335=CARTESIAN_POINT('Ctrl Pts',(-9.35560104202677,22.5521952569375,
2.51416264893798));
#102336=CARTESIAN_POINT('Ctrl Pts',(-9.35100514436171,22.551826663362,2.51718212262959));
#102337=CARTESIAN_POINT('Ctrl Pts',(-9.32843011714878,22.5500171932951,
2.5322411740018));
#102338=CARTESIAN_POINT('Ctrl Pts',(-9.31076270077627,22.5486044097237,
2.54474331094942));
#102339=CARTESIAN_POINT('Ctrl Pts',(-9.27575220616946,22.5457895456707,
2.57099546250814));
#102340=CARTESIAN_POINT('Ctrl Pts',(-9.25843229426695,22.5443889605833,
2.58476137869081));
#102341=CARTESIAN_POINT('Ctrl Pts',(-9.16563788696809,22.5367783291289,
2.66287931892294));
#102342=CARTESIAN_POINT('Ctrl Pts',(-9.09813992032658,22.5308051759434,
2.73607585946128));
#102343=CARTESIAN_POINT('Ctrl Pts',(-9.02981576249249,22.5232598586663,
2.8320298762372));
#102344=CARTESIAN_POINT('Ctrl Pts',(-9.0193805387261,22.5220566774688,2.84744582122026));
#102345=CARTESIAN_POINT('Ctrl Pts',(-9.00406702162296,22.5202064943524,
2.87126574924087));
#102346=CARTESIAN_POINT('Ctrl Pts',(-8.99891987268374,22.5195689635595,
2.87949389590779));
#102347=CARTESIAN_POINT('Ctrl Pts',(-8.98970894085492,22.5183983150926,
2.89463129119739));
#102348=CARTESIAN_POINT('Ctrl Pts',(-8.98561284684558,22.5178663823735,
2.90152026264539));
#102349=CARTESIAN_POINT('Ctrl Pts',(-8.97893653358354,22.5169799564346,
2.91301421125764));
#102350=CARTESIAN_POINT('Ctrl Pts',(-8.97631634759026,22.5166269036711,
2.91759576162104));
#102351=CARTESIAN_POINT('Ctrl Pts',(-8.9713586158957,22.5159487952961,2.92640147148972));
#102352=CARTESIAN_POINT('Ctrl Pts',(-8.96901607009313,22.5156239262654,
2.93062270498448));
#102353=CARTESIAN_POINT('Ctrl Pts',(-8.96360778275862,22.5148632997845,
2.94051117066737));
#102354=CARTESIAN_POINT('Ctrl Pts',(-8.96056248896243,22.5144268321504,
2.94618935014971));
#102355=CARTESIAN_POINT('Ctrl Pts',(-8.95127391195093,22.5130696588026,
2.96385511953369));
#102356=CARTESIAN_POINT('Ctrl Pts',(-8.94519046739396,22.5121434345011,
2.97592503967383));
#102357=CARTESIAN_POINT('Ctrl Pts',(-8.89519933581948,22.5042003059119,
3.07950859410976));
#102358=CARTESIAN_POINT('Ctrl Pts',(-8.86309288137422,22.4967658512563,
3.17622352672085));
#102359=CARTESIAN_POINT('Ctrl Pts',(-8.8327400315645,22.485067354181,3.33277516322405));
#102360=CARTESIAN_POINT('Ctrl Pts',(-8.82591983383854,22.4808376689838,
3.39046760746644));
#102361=CARTESIAN_POINT('Ctrl Pts',(-8.82306301311328,22.4762955362862,
3.45565344887865));
#102362=CARTESIAN_POINT('Ctrl Pts',(-8.82281304870948,22.4757955684185,
3.46287620746148));
#102363=CARTESIAN_POINT('Ctrl Pts',(-8.82253987534896,22.4750563212384,
3.47363330925202));
#102364=CARTESIAN_POINT('Ctrl Pts',(-8.82246606920406,22.4748144086654,
3.47716603026419));
#102365=CARTESIAN_POINT('Ctrl Pts',(-8.82236680724217,22.4744012329279,
3.48322222468937));
#102366=CARTESIAN_POINT('Ctrl Pts',(-8.82233356161298,22.4742295460422,
3.48574550000601));
#102367=CARTESIAN_POINT('Ctrl Pts',(-8.82227647693805,22.4738406707824,
3.4914762806554));
#102368=CARTESIAN_POINT('Ctrl Pts',(-8.82225763042966,22.4736237607589,
3.49468378844386));
#102369=CARTESIAN_POINT('Ctrl Pts',(-8.82224200968322,22.4730356617882,
3.5034086028157));
#102370=CARTESIAN_POINT('Ctrl Pts',(-8.82227090019157,22.4726658539685,
3.50892595983525));
#102371=CARTESIAN_POINT('Ctrl Pts',(-8.82260658671649,22.4708407285318,
3.53629727294185));
#102372=CARTESIAN_POINT('Ctrl Pts',(-8.82348291434856,22.4694140885965,
3.55814152245687));
#102373=CARTESIAN_POINT('Ctrl Pts',(-8.82646554322228,22.4665888039135,
3.60197732634387));
#102374=CARTESIAN_POINT('Ctrl Pts',(-8.82858343186148,22.4651911535401,
3.62395893556084));
#102375=CARTESIAN_POINT('Ctrl Pts',(-8.84364252023728,22.4575637294245,
3.74461019498027));
#102376=CARTESIAN_POINT('Ctrl Pts',(-8.86842959271848,22.451570705444,3.8413878645372));
#102377=CARTESIAN_POINT('Ctrl Pts',(-8.91524778213248,22.4434261306559,
3.95953002665625));
#102378=CARTESIAN_POINT('Ctrl Pts',(-8.92630147549828,22.441635180557,3.98479532497319));
#102379=CARTESIAN_POINT('Ctrl Pts',(-8.94188725538245,22.4392562645065,
4.01726577477724));
#102380=CARTESIAN_POINT('Ctrl Pts',(-8.94562554409381,22.438695451663,4.02484375067802));
#102381=CARTESIAN_POINT('Ctrl Pts',(-8.95188010281223,22.4377724854518,
4.03718596801832));
#102382=CARTESIAN_POINT('Ctrl Pts',(-8.95434814028535,22.4374120107708,
4.04197441798461));
#102383=CARTESIAN_POINT('Ctrl Pts',(-8.95919466099341,22.4367111802419,
4.05122122754505));
#102384=CARTESIAN_POINT('Ctrl Pts',(-8.96156916056801,22.4363709698971,
4.05568155066113));
#102385=CARTESIAN_POINT('Ctrl Pts',(-8.96713533219878,22.4355806092977,
4.06597692018125));
#102386=CARTESIAN_POINT('Ctrl Pts',(-8.97034784957455,22.4351297304064,
4.07180043908619));
#102387=CARTESIAN_POINT('Ctrl Pts',(-8.98098622415399,22.4336533737674,
4.09070486482942));
#102388=CARTESIAN_POINT('Ctrl Pts',(-8.98861311858687,22.4326207845875,
4.10367031759685));
#102389=CARTESIAN_POINT('Ctrl Pts',(-9.03897376584941,22.4259593845019,
4.18564727621822));
#102390=CARTESIAN_POINT('Ctrl Pts',(-9.08848988703125,22.4200788734109,
4.25021889189771));
#102391=CARTESIAN_POINT('Ctrl Pts',(-9.18181894980893,22.4101099413912,
4.34892088516813));
#102392=CARTESIAN_POINT('Ctrl Pts',(-9.22212393923692,22.4060800458334,
4.38600017319625));
#102393=CARTESIAN_POINT('Ctrl Pts',(-9.27747622969541,22.4010000842008,
4.43022317345313));
#102394=CARTESIAN_POINT('Ctrl Pts',(-9.29029715278954,22.3998525706572,
4.44004131549207));
#102395=CARTESIAN_POINT('Ctrl Pts',(-9.31200724324838,22.3979624104561,
4.45596925213839));
#102396=CARTESIAN_POINT('Ctrl Pts',(-9.32078543596382,22.3972120907018,
4.46222598234168));
#102397=CARTESIAN_POINT('Ctrl Pts',(-9.3330592981464,22.3961834447916,4.47072260171185));
#102398=CARTESIAN_POINT('Ctrl Pts',(-9.33648243869067,22.3958987267403,
4.47306562800808));
#102399=CARTESIAN_POINT('Ctrl Pts',(-9.34230170452359,22.3954184675781,
4.47700373552385));
#102400=CARTESIAN_POINT('Ctrl Pts',(-9.34469140782919,22.3952223113362,
4.4786081937138));
#102401=CARTESIAN_POINT('Ctrl Pts',(-9.34928838053649,22.3948470448317,
4.48167023326546));
#102402=CARTESIAN_POINT('Ctrl Pts',(-9.3514947004904,22.3946678414313,4.48312915501743));
#102403=CARTESIAN_POINT('Ctrl Pts',(-9.35679941576814,22.3942390982952,
4.48661125265021));
#102404=CARTESIAN_POINT('Ctrl Pts',(-9.35990249202658,22.3939900243667,
4.4886272991484));
#102405=CARTESIAN_POINT('Ctrl Pts',(-9.37121650887726,22.3930879398452,
4.49590233375147));
#102406=CARTESIAN_POINT('Ctrl Pts',(-9.37948345079794,22.3924403334364,
4.50107410538978));
#102407=CARTESIAN_POINT('Ctrl Pts',(-9.44008453232324,22.3877689425157,
4.53794673751422));
#102408=CARTESIAN_POINT('Ctrl Pts',(-9.49476130446408,22.3839591405728,
4.56563343118322));
#102409=CARTESIAN_POINT('Ctrl Pts',(-9.61324844901511,22.3760254775498,
4.6144506639708));
#102410=CARTESIAN_POINT('Ctrl Pts',(-9.67720627388599,22.3719166010519,
4.63462797072597));
#102411=CARTESIAN_POINT('Ctrl Pts',(-9.77641450351613,22.3654534218445,
4.65685365246097));
#102412=CARTESIAN_POINT('Ctrl Pts',(-9.81061522235923,22.3632114144455,
4.66294191221591));
#102413=CARTESIAN_POINT('Ctrl Pts',(-9.85407119560418,22.360320449151,4.66870996523399));
#102414=CARTESIAN_POINT('Ctrl Pts',(-9.86312324148109,22.3597160055256,
4.66980466062905));
#102415=CARTESIAN_POINT('Ctrl Pts',(-9.87768728091765,22.3587394961209,
4.67139458605251));
#102416=CARTESIAN_POINT('Ctrl Pts',(-9.88319176462538,22.3583695078131,
4.67195627557292));
#102417=CARTESIAN_POINT('Ctrl Pts',(-9.89368419471227,22.3576624144286,
4.67295229181495));
#102418=CARTESIAN_POINT('Ctrl Pts',(-9.89867136521094,22.3573255362428,
4.67339364058538));
#102419=CARTESIAN_POINT('Ctrl Pts',(-9.91008268752092,22.3565528383528,
4.67433021487081));
#102420=CARTESIAN_POINT('Ctrl Pts',(-9.91650834573871,22.3561163785527,
4.67480454435788));
#102421=CARTESIAN_POINT('Ctrl Pts',(-9.93642374858349,22.3547592541236,
4.67611044748734));
#102422=CARTESIAN_POINT('Ctrl Pts',(-9.94992374396886,22.3538330714803,
4.67676253616903));
#102423=CARTESIAN_POINT('Ctrl Pts',(-10.0648869280207,22.3458897644536,
4.68033380304585));
#102424=CARTESIAN_POINT('Ctrl Pts',(-10.1663054591593,22.3384550576385,
4.67035557181679));
#102425=CARTESIAN_POINT('Ctrl Pts',(-10.3216792027605,22.3267564904808,
4.63445238220202));
#102426=CARTESIAN_POINT('Ctrl Pts',(-10.3771606099677,22.3225269778226,
4.6172337234391));
#102427=CARTESIAN_POINT('Ctrl Pts',(-10.4378774894707,22.3179850082533,
4.59334833926638));
#102428=CARTESIAN_POINT('Ctrl Pts',(-10.4445781936335,22.3174850449339,
4.59064087722309));
#102429=CARTESIAN_POINT('Ctrl Pts',(-10.4545175154729,22.3167458031383,
4.58651800517167));
#102430=CARTESIAN_POINT('Ctrl Pts',(-10.457775217083,22.3165038914559,4.58514948227599));
#102431=CARTESIAN_POINT('Ctrl Pts',(-10.4633488664232,22.3160907167106,
4.58277848999989));
#102432=CARTESIAN_POINT('Ctrl Pts',(-10.4656677994781,22.3159190299324,
4.58178321829983));
#102433=CARTESIAN_POINT('Ctrl Pts',(-10.4709270063596,22.3155301542001,
4.57950595426882));
#102434=CARTESIAN_POINT('Ctrl Pts',(-10.4738652530577,22.3153132436011,
4.57821939937418));
#102435=CARTESIAN_POINT('Ctrl Pts',(-10.4818431766499,22.3147251415353,
4.57468723629766));
#102436=CARTESIAN_POINT('Ctrl Pts',(-10.4868724673683,22.3143553312203,
4.57241815829007));
#102437=CARTESIAN_POINT('Ctrl Pts',(-10.5117445920313,22.3125301734291,
4.56098550127302));
#102438=CARTESIAN_POINT('Ctrl Pts',(-10.5313470467539,22.3111035048499,
4.55130548609623));
#102439=CARTESIAN_POINT('Ctrl Pts',(-10.5701860929453,22.3082781985637,
4.53076200553939));
#102440=CARTESIAN_POINT('Ctrl Pts',(-10.5894089015904,22.306880554198,4.51989202215604));
#102441=CARTESIAN_POINT('Ctrl Pts',(-10.6935227010269,22.299253094247,4.45709099403719));
#102442=CARTESIAN_POINT('Ctrl Pts',(-10.7718699014231,22.2932600281749,
4.39510572286816));
#102443=CARTESIAN_POINT('Ctrl Pts',(-10.8607810826766,22.2851154590572,
4.30430783653869));
#102444=CARTESIAN_POINT('Ctrl Pts',(-10.8793713184431,22.2833245679962,
4.2839394502097));
#102445=CARTESIAN_POINT('Ctrl Pts',(-10.9027024312337,22.2809457194186,
4.2565016728679));
#102446=CARTESIAN_POINT('Ctrl Pts',(-10.9081065550702,22.2803849130357,
4.25000595921701));
#102447=CARTESIAN_POINT('Ctrl Pts',(-10.9168407726508,22.2794619547381,
4.23927469893849));
#102448=CARTESIAN_POINT('Ctrl Pts',(-10.9202125886999,22.2791014814536,
4.23507337922244));
#102449=CARTESIAN_POINT('Ctrl Pts',(-10.9266910506768,22.2784006516936,
4.22688671200349));
#102450=CARTESIAN_POINT('Ctrl Pts',(-10.9298011095357,22.2780604407084,
4.22290420584305));
#102451=CARTESIAN_POINT('Ctrl Pts',(-10.9369451270782,22.277270075748,4.21363374761644));
#102452=CARTESIAN_POINT('Ctrl Pts',(-10.9409600797858,22.2768191931112,
4.20833143512559));
#102453=CARTESIAN_POINT('Ctrl Pts',(-10.9539083181515,22.2753428114237,
4.19092708919635));
#102454=CARTESIAN_POINT('Ctrl Pts',(-10.9626543923604,22.2743102006057,
4.17868829843754));
#102455=CARTESIAN_POINT('Ctrl Pts',(-11.0170827983842,22.267648847812,4.09935467149147));
#102456=CARTESIAN_POINT('Ctrl Pts',(-11.0559518974809,22.2617684135024,
4.02786787465041));
#102457=CARTESIAN_POINT('Ctrl Pts',(-11.1081962309625,22.251799525032,3.90247740819524));
#102458=CARTESIAN_POINT('Ctrl Pts',(-11.125691408251,22.2477695946559,3.85058005713566));
#102459=CARTESIAN_POINT('Ctrl Pts',(-11.1435971408276,22.2426895940734,
3.7820307305509));
#102460=CARTESIAN_POINT('Ctrl Pts',(-11.1473562455867,22.2415420751095,
3.76632584231397));
#102461=CARTESIAN_POINT('Ctrl Pts',(-11.1530844231083,22.2396519069557,
3.74001574606053));
#102462=CARTESIAN_POINT('Ctrl Pts',(-11.1552328557163,22.2389015845913,
3.72945220626803));
#102463=CARTESIAN_POINT('Ctrl Pts',(-11.158006889313,22.2378729357296,3.71478434210418));
#102464=CARTESIAN_POINT('Ctrl Pts',(-11.1587562048868,22.2375882172899,
3.71070436222177));
#102465=CARTESIAN_POINT('Ctrl Pts',(-11.1599889217081,22.2371079576655,
3.70378677243828));
#102466=CARTESIAN_POINT('Ctrl Pts',(-11.160483500761,22.2369118013473,3.70095121856903));
#102467=CARTESIAN_POINT('Ctrl Pts',(-11.1614126174234,22.2365365348493,
3.69550649776286));
#102468=CARTESIAN_POINT('Ctrl Pts',(-11.1618487656391,22.2363573315308,
3.69289765346815));
#102469=CARTESIAN_POINT('Ctrl Pts',(-11.1628739931369,22.2359285887898,
3.68663555787491));
#102470=CARTESIAN_POINT('Ctrl Pts',(-11.1634546559265,22.2356795151727,
3.68298092770368));
#102471=CARTESIAN_POINT('Ctrl Pts',(-11.1655027123365,22.2347774334213,
3.66968666387292));
#102472=CARTESIAN_POINT('Ctrl Pts',(-11.1668676573237,22.2341298294264,
3.66003131533279));
#102473=CARTESIAN_POINT('Ctrl Pts',(-11.1759244496307,22.2294582006022,
3.5896710404321));
#102474=CARTESIAN_POINT('Ctrl Pts',(-11.1789959182013,22.2256481846331,
3.52845733912431));
#102475=CARTESIAN_POINT('Ctrl Pts',(-11.1754351561762,22.2177144705944,
3.4003562508788));
#102476=CARTESIAN_POINT('Ctrl Pts',(-11.1678730882563,22.2136057509646,
3.33372158964951));
#102477=CARTESIAN_POINT('Ctrl Pts',(-11.147854678902,22.20714278727,3.23404806842098));
#102478=CARTESIAN_POINT('Ctrl Pts',(-11.139515708418,22.204900828335,3.20032620765442));
#102479=CARTESIAN_POINT('Ctrl Pts',(-11.1271222322066,22.202009917753,3.15827837162324));
#102480=CARTESIAN_POINT('Ctrl Pts',(-11.1244430034573,22.2014054782605,
3.14956295590559));
#102481=CARTESIAN_POINT('Ctrl Pts',(-11.1199757669009,22.2004289739334,
3.13561015535049));
#102482=CARTESIAN_POINT('Ctrl Pts',(-11.1182515319567,22.2000589865309,
3.13035261825761));
#102483=CARTESIAN_POINT('Ctrl Pts',(-11.1148966498186,22.199351893824,3.1203612380389));
#102484=CARTESIAN_POINT('Ctrl Pts',(-11.1132727335552,22.199015015403,3.11562524959459));
#102485=CARTESIAN_POINT('Ctrl Pts',(-11.1094900218632,22.1982423154793,
3.10481843620123));
#102486=CARTESIAN_POINT('Ctrl Pts',(-11.1073115218441,22.1978058538687,
3.09875472874456));
#102487=CARTESIAN_POINT('Ctrl Pts',(-11.1004095095312,22.1964487181342,
3.08002781103546));
#102488=CARTESIAN_POINT('Ctrl Pts',(-11.0955178379286,22.1955225258633,
3.06742819270565));
#102489=CARTESIAN_POINT('Ctrl Pts',(-11.0520514506142,22.1875792821989,
2.96093996121632));
#102490=CARTESIAN_POINT('Ctrl Pts',(-11.0017112746471,22.1801446587205,
2.87233450560586));
#102491=CARTESIAN_POINT('Ctrl Pts',(-10.9057528400591,22.1684461080741,
2.74496913577792));
#102492=CARTESIAN_POINT('Ctrl Pts',(-10.8674685214916,22.1642165322775,
2.70127615598767));
#102493=CARTESIAN_POINT('Ctrl Pts',(-10.8209648769333,22.1596745030138,
2.65550964603116));
#102494=CARTESIAN_POINT('Ctrl Pts',(-10.8157674885821,22.1591745380301,
2.65048796462936));
#102495=CARTESIAN_POINT('Ctrl Pts',(-10.8079604742552,22.1584352942642,
2.64308260636843));
#102496=CARTESIAN_POINT('Ctrl Pts',(-10.8053859303956,22.158193382256,2.6406624345386));
#102497=CARTESIAN_POINT('Ctrl Pts',(-10.8009540939124,22.1577802071477,
2.63653374711593));
#102498=CARTESIAN_POINT('Ctrl Pts',(-10.7991021641032,22.1576085203302,
2.63481957824148));
#102499=CARTESIAN_POINT('Ctrl Pts',(-10.7948837821957,22.1572196447708,
2.6309400921671));
#102500=CARTESIAN_POINT('Ctrl Pts',(-10.7925139854522,22.1570027343824,
2.62877848162224));
#102501=CARTESIAN_POINT('Ctrl Pts',(-10.7860439712692,22.1564146334494,
2.62292510136028));
#102502=CARTESIAN_POINT('Ctrl Pts',(-10.7819265321687,22.1560448240476,
2.61925236086059));
#102503=CARTESIAN_POINT('Ctrl Pts',(-10.7613711949434,22.1542196780974,
2.60117484588003));
#102504=CARTESIAN_POINT('Ctrl Pts',(-10.7445591625958,22.1527930200011,
2.58719960814795));
#102505=CARTESIAN_POINT('Ctrl Pts',(-10.7100023957452,22.1499677216212,
2.56006431494759));
#102506=CARTESIAN_POINT('Ctrl Pts',(-10.6922573015275,22.1485700750568,
2.54691951023992));
#102507=CARTESIAN_POINT('Ctrl Pts',(-10.5925589793672,22.1409426282226,
2.47732179414901));
#102508=CARTESIAN_POINT('Ctrl Pts',(-10.5040795022807,22.1349495775568,
2.43093442470316));
#102509=CARTESIAN_POINT('Ctrl Pts',(-10.384980745302,22.1268050063642,2.38660653282203));
#102510=CARTESIAN_POINT('Ctrl Pts',(-10.3588141458205,22.1250140936948,
2.37790044789053));
#102511=CARTESIAN_POINT('Ctrl Pts',(-10.3242614242211,22.1226352204215,
2.36773634263888));
#102512=CARTESIAN_POINT('Ctrl Pts',(-10.3161298633127,22.1220744116739,
2.36543913148922));
#102513=CARTESIAN_POINT('Ctrl Pts',(-10.3027748378282,22.1211514504798,
2.36182098044806));
#102514=CARTESIAN_POINT('Ctrl Pts',(-10.297565686207,22.1207909766841,2.36044800745204));
#102515=CARTESIAN_POINT('Ctrl Pts',(-10.2874525042433,22.1200901466426,
2.35785655311483));
#102516=CARTESIAN_POINT('Ctrl Pts',(-10.2825496826949,22.1197499358918,
2.35663379842887));
#102517=CARTESIAN_POINT('Ctrl Pts',(-10.2711757775239,22.1189595725276,
2.35387479117138));
#102518=CARTESIAN_POINT('Ctrl Pts',(-10.2646992988388,22.1185086912616,
2.35236174050038));
#102519=CARTESIAN_POINT('Ctrl Pts',(-10.2435346084948,22.1170323187422,
2.34760587771566));
#102520=CARTESIAN_POINT('Ctrl Pts',(-10.2287975443728,22.1159997158441,
2.34458969805409));
#102521=CARTESIAN_POINT('Ctrl Pts',(-10.1341854029018,22.1093380645483,
2.3271068079901));
#102522=CARTESIAN_POINT('Ctrl Pts',(-10.0530668290272,22.1034572933146,
2.32065122416567));
#102523=CARTESIAN_POINT('Ctrl Pts',(-9.91805451334948,22.0935462558775,
2.32386829630545));
#102524=CARTESIAN_POINT('Ctrl Pts',(-9.86431471500832,22.089575070732,2.32885069407818));
#102525=CARTESIAN_POINT('Ctrl Pts',(-9.81110406355273,22.0857064764352,
2.33749693002826));
#102526=CARTESIAN_POINT('Ctrl Pts',(-9.8111040696154,21.9876672748127,2.33749692904314));
#102527=CARTESIAN_POINT('Ctrl Pts',(-9.87819815585959,21.9926487009463,
2.32659476442867));
#102528=CARTESIAN_POINT('Ctrl Pts',(-9.94610318052165,21.9976751846187,
2.32152147714435));
#102529=CARTESIAN_POINT('Ctrl Pts',(-10.0297196451487,22.00362504353,2.32252114418055));
#102530=CARTESIAN_POINT('Ctrl Pts',(-10.0453554859209,22.0047268891869,
2.32301969032066));
#102531=CARTESIAN_POINT('Ctrl Pts',(-10.0657045114906,22.0061430931441,
2.32407466935722));
#102532=CARTESIAN_POINT('Ctrl Pts',(-10.0704299822049,22.0064707135964,
2.32434822948283));
#102533=CARTESIAN_POINT('Ctrl Pts',(-10.0792908738116,22.0070825405063,
2.32491480928958));
#102534=CARTESIAN_POINT('Ctrl Pts',(-10.0834266303263,22.0073670813893,
2.32520118881562));
#102535=CARTESIAN_POINT('Ctrl Pts',(-10.0904299953181,22.0078470813904,
2.32572330513678));
#102536=CARTESIAN_POINT('Ctrl Pts',(-10.0932983845497,22.008043154678,2.32594772166279));
#102537=CARTESIAN_POINT('Ctrl Pts',(-10.0988014649904,22.0084182906247,
2.32639856621338));
#102538=CARTESIAN_POINT('Ctrl Pts',(-10.1014362429372,22.0085974461927,
2.32662335806366));
#102539=CARTESIAN_POINT('Ctrl Pts',(-10.1077556991021,22.009026108058,2.3271839611209));
#102540=CARTESIAN_POINT('Ctrl Pts',(-10.1114396246146,22.0092751485481,
2.32752826783353));
#102541=CARTESIAN_POINT('Ctrl Pts',(-10.1248284910324,22.0101773777237,
2.32884329119695));
#102542=CARTESIAN_POINT('Ctrl Pts',(-10.1345232268833,22.0108251585374,
2.32991722283237));
#102543=CARTESIAN_POINT('Ctrl Pts',(-10.2036744343364,22.0154134420393,
2.33844829569929));
#102544=CARTESIAN_POINT('Ctrl Pts',(-10.2625065764362,22.0191489360262,
2.3503140327401));
#102545=CARTESIAN_POINT('Ctrl Pts',(-10.3641372597904,22.0256893678699,
2.37902499041741));
#102546=CARTESIAN_POINT('Ctrl Pts',(-10.4073284980213,22.0284982663367,
2.39398719840255));
#102547=CARTESIAN_POINT('Ctrl Pts',(-10.4986206969682,22.034668816066,2.4316872714663));
#102548=CARTESIAN_POINT('Ctrl Pts',(-10.5462678604914,22.0380401343023,
2.45524881100488));
#102549=CARTESIAN_POINT('Ctrl Pts',(-10.6017886737427,22.04225582356,2.4875428173464));
#102550=CARTESIAN_POINT('Ctrl Pts',(-10.6113376715883,22.0429915644591,
2.49327988400616));
#102551=CARTESIAN_POINT('Ctrl Pts',(-10.626009712147,22.0441394877179,2.50238061645066));
#102552=CARTESIAN_POINT('Ctrl Pts',(-10.6311904698151,22.0445482590806,
2.50565037207584));
#102553=CARTESIAN_POINT('Ctrl Pts',(-10.6405315712947,22.0452916676645,
2.5116482823902));
#102554=CARTESIAN_POINT('Ctrl Pts',(-10.6447006135056,22.0456257922874,
2.51436267868494));
#102555=CARTESIAN_POINT('Ctrl Pts',(-10.6536345911874,22.0463469084196,
2.52026038105914));
#102556=CARTESIAN_POINT('Ctrl Pts',(-10.6583937240264,22.0467342110984,
2.52345220195346));
#102557=CARTESIAN_POINT('Ctrl Pts',(-10.671201771032,22.0477852557383,2.5321783956718));
#102558=CARTESIAN_POINT('Ctrl Pts',(-10.6792052866337,22.0484514461455,
2.53777827719809));
#102559=CARTESIAN_POINT('Ctrl Pts',(-10.7195987911834,22.0518628586171,
2.56679578148276));
#102560=CARTESIAN_POINT('Ctrl Pts',(-10.7508478065048,22.0546664204829,
2.59174923253043));
#102561=CARTESIAN_POINT('Ctrl Pts',(-10.8527462201602,22.0643928472976,
2.68197645400811));
#102562=CARTESIAN_POINT('Ctrl Pts',(-10.9166419077113,22.0715637869243,
2.75427696612489));
#102563=CARTESIAN_POINT('Ctrl Pts',(-10.9887476401344,22.0807726416558,
2.85933425571479));
#102564=CARTESIAN_POINT('Ctrl Pts',(-11.0054237510702,22.0830033183512,
2.88583555632829));
#102565=CARTESIAN_POINT('Ctrl Pts',(-11.0239520512199,22.0855824663701,
2.91806209146585));
#102566=CARTESIAN_POINT('Ctrl Pts',(-11.0268403802859,22.0859877026338,
2.92317388271512));
#102567=CARTESIAN_POINT('Ctrl Pts',(-11.0313173133216,22.0866206321607,
2.93123740048873));
#102568=CARTESIAN_POINT('Ctrl Pts',(-11.0329317010754,22.0868498784648,
2.93417458789679));
#102569=CARTESIAN_POINT('Ctrl Pts',(-11.0358658954976,22.0872683514378,
2.93956741660968));
#102570=CARTESIAN_POINT('Ctrl Pts',(-11.0371895229283,22.0874578102384,
2.94202085356191));
#102571=CARTESIAN_POINT('Ctrl Pts',(-11.0401496061393,22.0878830685177,
2.94755450564967));
#102572=CARTESIAN_POINT('Ctrl Pts',(-11.0417810969789,22.0881185570915,
2.95063730182402));
#102573=CARTESIAN_POINT('Ctrl Pts',(-11.0459415238944,22.0887220465344,
2.95858385534162));
#102574=CARTESIAN_POINT('Ctrl Pts',(-11.0484502753889,22.0890888349177,
2.96345816937408));
#102575=CARTESIAN_POINT('Ctrl Pts',(-11.0640833448657,22.0913940325237,
2.99436041902814));
#102576=CARTESIAN_POINT('Ctrl Pts',(-11.0762728323061,22.0932803930998,
3.02085298167945));
#102577=CARTESIAN_POINT('Ctrl Pts',(-11.1252789594728,22.1014009318217,
3.13869773644542));
#102578=CARTESIAN_POINT('Ctrl Pts',(-11.1515394416143,22.107306956937,3.23400843240098));
#102579=CARTESIAN_POINT('Ctrl Pts',(-11.1714099394503,22.1160854191793,
3.37145117272148));
#102580=CARTESIAN_POINT('Ctrl Pts',(-11.1751282813674,22.1186810026192,
3.41168791042498));
#102581=CARTESIAN_POINT('Ctrl Pts',(-11.1771612229977,22.1219698142552,
3.46156212338712));
#102582=CARTESIAN_POINT('Ctrl Pts',(-11.1774338716598,22.1226015970142,
3.47109525427539));
#102583=CARTESIAN_POINT('Ctrl Pts',(-11.1776831979547,22.1236116194228,
3.48625326532252));
#102584=CARTESIAN_POINT('Ctrl Pts',(-11.1777354101229,22.1239875141372,
3.49187661778551));
#102585=CARTESIAN_POINT('Ctrl Pts',(-11.1777579330679,22.12469914187,3.50248735174402));
#102586=CARTESIAN_POINT('Ctrl Pts',(-11.1777368402003,22.1250346004664,
3.50747460639836));
#102587=CARTESIAN_POINT('Ctrl Pts',(-11.1776176162082,22.1257947622752,
3.51874195529776));
#102588=CARTESIAN_POINT('Ctrl Pts',(-11.177500923489,22.1262200319672,3.52502165902602));
#102589=CARTESIAN_POINT('Ctrl Pts',(-11.1770712985442,22.1273186830036,
3.54118177586455));
#102590=CARTESIAN_POINT('Ctrl Pts',(-11.1766841937867,22.1279943379136,
3.55105955574499));
#102591=CARTESIAN_POINT('Ctrl Pts',(-11.1726344980923,22.1333752858914,
3.6292322286402));
#102592=CARTESIAN_POINT('Ctrl Pts',(-11.1631542810495,22.1382619715537,
3.69708313900837));
#102593=CARTESIAN_POINT('Ctrl Pts',(-11.1322712700033,22.1483228748747,
3.83150288229873));
#102594=CARTESIAN_POINT('Ctrl Pts',(-11.1107240715515,22.1534802595565,
3.89777451699018));
#102595=CARTESIAN_POINT('Ctrl Pts',(-11.0724600960666,22.160508964899,3.98755598380316));
#102596=CARTESIAN_POINT('Ctrl Pts',(-11.0605461906433,22.1625009499129,
4.01295571691674));
#102597=CARTESIAN_POINT('Ctrl Pts',(-11.0451105398646,22.1648435047048,
4.04302123169852));
#102598=CARTESIAN_POINT('Ctrl Pts',(-11.0424479555176,22.1652398562807,
4.04811528169876));
#102599=CARTESIAN_POINT('Ctrl Pts',(-11.0382332184573,22.1658551284276,
4.05603709300212));
#102600=CARTESIAN_POINT('Ctrl Pts',(-11.0367066066577,22.1660755718294,
4.05887823096716));
#102601=CARTESIAN_POINT('Ctrl Pts',(-11.0338326788969,22.1664860438734,
4.06417452714636));
#102602=CARTESIAN_POINT('Ctrl Pts',(-11.0324882879326,22.1666762401404,
4.0666311327001));
#102603=CARTESIAN_POINT('Ctrl Pts',(-11.0293968325784,22.1671095033239,
4.07223261461879));
#102604=CARTESIAN_POINT('Ctrl Pts',(-11.0276441111894,22.1673522097884,
4.0753743005698));
#102605=CARTESIAN_POINT('Ctrl Pts',(-11.0229414022039,22.1679958006365,
4.08371368619543));
#102606=CARTESIAN_POINT('Ctrl Pts',(-11.019966154278,22.1683951495066,4.08889712820039));
#102607=CARTESIAN_POINT('Ctrl Pts',(-10.9958700737207,22.1715695117732,
4.13014655554927));
#102608=CARTESIAN_POINT('Ctrl Pts',(-10.9728799150741,22.1742368813648,
4.16509202016769));
#102609=CARTESIAN_POINT('Ctrl Pts',(-10.8894099110891,22.1830652620182,
4.27834659497096));
#102610=CARTESIAN_POINT('Ctrl Pts',(-10.8209534468426,22.1890210331115,
4.35024078738506));
#102611=CARTESIAN_POINT('Ctrl Pts',(-10.7223325159853,22.1971690141051,
4.43066401105529));
#102612=CARTESIAN_POINT('Ctrl Pts',(-10.6997094050158,22.1990104191988,
4.44779022300222));
#102613=CARTESIAN_POINT('Ctrl Pts',(-10.6695079570304,22.2014468301798,
4.4689824256468));
#102614=CARTESIAN_POINT('Ctrl Pts',(-10.6624715201355,22.2020129663741,
4.47380661549748));
#102615=CARTESIAN_POINT('Ctrl Pts',(-10.6508937936291,22.2029423739758,
4.48156076251719));
#102616=CARTESIAN_POINT('Ctrl Pts',(-10.6463835665918,22.2033039192836,
4.48453671555779));
#102617=CARTESIAN_POINT('Ctrl Pts',(-10.6376240831623,22.2040051846983,
4.49023029213341));
#102618=CARTESIAN_POINT('Ctrl Pts',(-10.633377526254,22.2043447486263,4.49295186729208));
#102619=CARTESIAN_POINT('Ctrl Pts',(-10.6235315483333,22.2051311940205,
4.49917319402068));
#102620=CARTESIAN_POINT('Ctrl Pts',(-10.6179199592271,22.2055787829027,
4.50265327223217));
#102621=CARTESIAN_POINT('Ctrl Pts',(-10.5996551740386,22.2070337597525,
4.51376877773323));
#102622=CARTESIAN_POINT('Ctrl Pts',(-10.5868878861677,22.2080479780482,
4.521213022314));
#102623=CARTESIAN_POINT('Ctrl Pts',(-10.4972929581787,22.2151490589301,
4.57121822607051));
#102624=CARTESIAN_POINT('Ctrl Pts',(-10.4160683329059,22.2215359757464,
4.60530098705531));
#102625=CARTESIAN_POINT('Ctrl Pts',(-10.2648545038587,22.2331084453963,
4.64970413056364));
#102626=CARTESIAN_POINT('Ctrl Pts',(-10.1962561672777,22.2382401029016,
4.66338006127205));
#102627=CARTESIAN_POINT('Ctrl Pts',(-10.1196963622983,22.2436002962789,
4.67167381637525));
#102628=CARTESIAN_POINT('Ctrl Pts',(-10.1125415343706,22.2440976516662,
4.67238268523291));
#102629=CARTESIAN_POINT('Ctrl Pts',(-10.1018692408524,22.2448337560238,
4.67334144574814));
#102630=CARTESIAN_POINT('Ctrl Pts',(-10.0983565815229,22.2450751073661,
4.67364111815887));
#102631=CARTESIAN_POINT('Ctrl Pts',(-10.0923289282043,22.2454876089015,
4.67412809827691));
#102632=CARTESIAN_POINT('Ctrl Pts',(-10.0898146275256,22.2456591793799,
4.67432310514116));
#102633=CARTESIAN_POINT('Ctrl Pts',(-10.084097475031,22.2460481710457,4.67474805287377));
#102634=CARTESIAN_POINT('Ctrl Pts',(-10.0808942975097,22.2462653117054,
4.67497297257901));
#102635=CARTESIAN_POINT('Ctrl Pts',(-10.072166906762,22.2468548490445,4.67554993091432));
#102636=CARTESIAN_POINT('Ctrl Pts',(-10.0666409811312,22.2472258526874,
4.67587613511491));
#102637=CARTESIAN_POINT('Ctrl Pts',(-10.0390549149078,22.2490675228593,
4.67730949252029));
#102638=CARTESIAN_POINT('Ctrl Pts',(-10.0169673805789,22.2505088823298,
4.67783495775458));
#102639=CARTESIAN_POINT('Ctrl Pts',(-9.88946870907654,22.2587044625537,
4.67728029977967));
#102640=CARTESIAN_POINT('Ctrl Pts',(-9.7845925480739,22.264994905042,4.66267366183043));
#102641=CARTESIAN_POINT('Ctrl Pts',(-9.64330073198281,22.2742607490217,
4.62319378677043));
#102642=CARTESIAN_POINT('Ctrl Pts',(-9.6041642032603,22.2769115890524,4.61000544851472));
#102643=CARTESIAN_POINT('Ctrl Pts',(-9.55688348055992,22.2802624258923,
4.59125381733467));
#102644=CARTESIAN_POINT('Ctrl Pts',(-9.54800729939772,22.2808980551269,
4.58760734332668));
#102645=CARTESIAN_POINT('Ctrl Pts',(-9.5339897647633,22.2819128038305,4.58164749024288));
#102646=CARTESIAN_POINT('Ctrl Pts',(-9.52881862772023,22.2822895397315,
4.57940490319199));
#102647=CARTESIAN_POINT('Ctrl Pts',(-9.51910439997351,22.2830018712729,
4.5751089891964));
#102648=CARTESIAN_POINT('Ctrl Pts',(-9.51455784723318,22.2833371860097,
4.57306375941842));
#102649=CARTESIAN_POINT('Ctrl Pts',(-9.50433138319463,22.2840958210331,
4.56838517396512));
#102650=CARTESIAN_POINT('Ctrl Pts',(-9.49865924618378,22.2845196985873,
4.56573528775604));
#102651=CARTESIAN_POINT('Ctrl Pts',(-9.48414646467492,22.2856123594336,
4.55881376738984));
#102652=CARTESIAN_POINT('Ctrl Pts',(-9.47533777135234,22.2862833748265,
4.5544766472432));
#102653=CARTESIAN_POINT('Ctrl Pts',(-9.41127134674679,22.2912223968423,
4.52193089179353));
#102654=CARTESIAN_POINT('Ctrl Pts',(-9.35827411487587,22.2956380339668,
4.4895098733112));
#102655=CARTESIAN_POINT('Ctrl Pts',(-9.24684884324462,22.3056486156696,
4.40861671049233));
#102656=CARTESIAN_POINT('Ctrl Pts',(-9.19004305398253,22.3112703110453,
4.3583650252624));
#102657=CARTESIAN_POINT('Ctrl Pts',(-9.11910618930527,22.3187658104108,
4.28225708113894));
#102658=CARTESIAN_POINT('Ctrl Pts',(-9.10051586444404,22.3207818004421,
4.26080788694628));
#102659=CARTESIAN_POINT('Ctrl Pts',(-9.07910038322968,22.3231485600952,
4.23421536687438));
#102660=CARTESIAN_POINT('Ctrl Pts',(-9.07551678478683,22.3235461902141,
4.2296979493774));
#102661=CARTESIAN_POINT('Ctrl Pts',(-9.06997814901695,22.3241630059763,
4.22260974741094));
#102662=CARTESIAN_POINT('Ctrl Pts',(-9.06800032426337,22.3243837265553,
4.22005700845329));
#102663=CARTESIAN_POINT('Ctrl Pts',(-9.06432732872563,22.3247944338049,
4.21527585840877));
#102664=CARTESIAN_POINT('Ctrl Pts',(-9.06262961694608,22.3249845901798,
4.21304955409555));
#102665=CARTESIAN_POINT('Ctrl Pts',(-9.05877223844409,22.325417411436,4.20795357316349));
#102666=CARTESIAN_POINT('Ctrl Pts',(-9.05661774594752,22.3256597186396,
4.2050800553665));
#102667=CARTESIAN_POINT('Ctrl Pts',(-9.05092545067806,22.3263015403717,
4.19741525190562));
#102668=CARTESIAN_POINT('Ctrl Pts',(-9.04741073412138,22.326699532731,4.19260683503569));
#102669=CARTESIAN_POINT('Ctrl Pts',(-9.01985583148657,22.3298351551966,
4.15430293275221));
#102670=CARTESIAN_POINT('Ctrl Pts',(-8.99755020494375,22.3324680383166,
4.11958868418623));
#102671=CARTESIAN_POINT('Ctrl Pts',(-8.92850905273416,22.3412130264482,
3.99861413492556));
#102672=CARTESIAN_POINT('Ctrl Pts',(-8.89073396578147,22.34711846511,3.90772344497099));
#102673=CARTESIAN_POINT('Ctrl Pts',(-8.85679760744793,22.3552778360896,
3.7847053408878));
#102674=CARTESIAN_POINT('Ctrl Pts',(-8.85001288766764,22.3571946755338,
3.75592626053806));
#102675=CARTESIAN_POINT('Ctrl Pts',(-8.84265125391466,22.3597170408715,
3.7184348657173));
#102676=CARTESIAN_POINT('Ctrl Pts',(-8.84107795065384,22.3602910276958,
3.70992757688324));
#102677=CARTESIAN_POINT('Ctrl Pts',(-8.83867001929862,22.3612300615691,
3.69605412718506));
#102678=CARTESIAN_POINT('Ctrl Pts',(-8.83777850998507,22.3615933124716,
3.69069806325441));
#102679=CARTESIAN_POINT('Ctrl Pts',(-8.83613188361129,22.3622956058562,
3.68036466643513));
#102680=CARTESIAN_POINT('Ctrl Pts',(-8.83537157930525,22.362634477094,3.6753882709818));
#102681=CARTESIAN_POINT('Ctrl Pts',(-8.83369670316043,22.3634160242503,
3.66393436495275));
#102682=CARTESIAN_POINT('Ctrl Pts',(-8.83280415631846,22.363859379701,3.65745385267506));
#102683=CARTESIAN_POINT('Ctrl Pts',(-8.83018421592774,22.3652499822013,
3.63718324080177));
#102684=CARTESIAN_POINT('Ctrl Pts',(-8.82864694847033,22.3662031046965,
3.62337021566095));
#102685=CARTESIAN_POINT('Ctrl Pts',(-8.8183640135199,22.3738462357418,3.51328323041129));
#102686=CARTESIAN_POINT('Ctrl Pts',(-8.82125974652214,22.3809095118362,
3.41630972939003));
#102687=CARTESIAN_POINT('Ctrl Pts',(-8.84264457109023,22.3912267462604,
3.27739654090259));
#102688=CARTESIAN_POINT('Ctrl Pts',(-8.85175001851315,22.3944414350054,
3.23439434465437));
#102689=CARTESIAN_POINT('Ctrl Pts',(-8.86695993121961,22.398596404737,3.17825796113221));
#102690=CARTESIAN_POINT('Ctrl Pts',(-8.87093200633344,22.3996049338589,
3.16458497021061));
#102691=CARTESIAN_POINT('Ctrl Pts',(-8.87805783415036,22.4012893910498,
3.14161885600952));
#102692=CARTESIAN_POINT('Ctrl Pts',(-8.88108148860042,22.4019711203979,
3.13228727443923));
#102693=CARTESIAN_POINT('Ctrl Pts',(-8.88550042505872,22.4029217137968,
3.11920908282922));
#102694=CARTESIAN_POINT('Ctrl Pts',(-8.88679863271106,22.4031957912578,
3.11543044557834));
#102695=CARTESIAN_POINT('Ctrl Pts',(-8.88905557216204,22.4036634280102,
3.10896846769012));
#102696=CARTESIAN_POINT('Ctrl Pts',(-8.89000485197604,22.4038575290419,
3.10628188626637));
#102697=CARTESIAN_POINT('Ctrl Pts',(-8.89186651707134,22.4042331822237,
3.10107339215072));
#102698=CARTESIAN_POINT('Ctrl Pts',(-8.89277777120447,22.4044148020431,
3.09855113542854));
#102699=CARTESIAN_POINT('Ctrl Pts',(-8.89528419671721,22.4049083189378,
3.09168706619551));
#102700=CARTESIAN_POINT('Ctrl Pts',(-8.89689636493688,22.405219231528,3.08735144489524));
#102701=CARTESIAN_POINT('Ctrl Pts',(-8.90318530934593,22.4064078314259,
3.0707387853088));
#102702=CARTESIAN_POINT('Ctrl Pts',(-8.90804204615833,22.4072756124512,
3.05853027428557));
#102703=CARTESIAN_POINT('Ctrl Pts',(-8.94394057383233,22.41336652772,2.9725107534463));
#102704=CARTESIAN_POINT('Ctrl Pts',(-8.9822382188358,22.4182504608339,2.90194420114871));
#102705=CARTESIAN_POINT('Ctrl Pts',(-9.06913293459486,22.4277886920449,
2.77470281899041));
#102706=CARTESIAN_POINT('Ctrl Pts',(-9.11651815016022,22.4324132483565,
2.71767835181147));
#102707=CARTESIAN_POINT('Ctrl Pts',(-9.17711537741943,22.4380252383403,
2.6573320613409));
#102708=CARTESIAN_POINT('Ctrl Pts',(-9.18541517538,22.4387877941195,2.64930622140219));
#102709=CARTESIAN_POINT('Ctrl Pts',(-9.19824309327323,22.4399580432492,
2.63726159990147));
#102710=CARTESIAN_POINT('Ctrl Pts',(-9.20268659102756,22.4403619255146,
2.63315341031463));
#102711=CARTESIAN_POINT('Ctrl Pts',(-9.21048138048688,22.4410679653809,
2.62605745744712));
#102712=CARTESIAN_POINT('Ctrl Pts',(-9.21381849180469,22.4413694665255,
2.62305424714222));
#102713=CARTESIAN_POINT('Ctrl Pts',(-9.22136893488262,22.4420499645926,
2.61633701413857));
#102714=CARTESIAN_POINT('Ctrl Pts',(-9.22559180334325,22.4424294043394,
2.61263392491907));
#102715=CARTESIAN_POINT('Ctrl Pts',(-9.23703176328023,22.4434543471603,
2.60274592765321));
#102716=CARTESIAN_POINT('Ctrl Pts',(-9.24429737593586,22.4441021511866,
2.59661805677827));
#102717=CARTESIAN_POINT('Ctrl Pts',(-9.27856563252399,22.4471437077546,
2.56841866178803));
#102718=CARTESIAN_POINT('Ctrl Pts',(-9.30646339627353,22.4495811603724,
2.54746764940007));
#102719=CARTESIAN_POINT('Ctrl Pts',(-9.40999842638136,22.4584982259682,
2.47667534578905));
#102720=CARTESIAN_POINT('Ctrl Pts',(-9.4903902305523,22.4652167075591,2.43435964630283));
#102721=CARTESIAN_POINT('Ctrl Pts',(-9.61082865842582,22.4746275634346,
2.38773574905088));
#102722=CARTESIAN_POINT('Ctrl Pts',(-9.6475061800053,22.4774088148649,2.3755735609717));
#102723=CARTESIAN_POINT('Ctrl Pts',(-9.69304183976916,22.4807105504651,
2.36292200037025));
#102724=CARTESIAN_POINT('Ctrl Pts',(-9.70139073836647,22.4813097909009,
2.36070100095704));
#102725=CARTESIAN_POINT('Ctrl Pts',(-9.71344346741404,22.4821653503904,
2.35763629569006));
#102726=CARTESIAN_POINT('Ctrl Pts',(-9.71712788269938,22.4824256132387,
2.35671838746412));
#102727=CARTESIAN_POINT('Ctrl Pts',(-9.72355404630266,22.4828772566101,
2.35515038710305));
#102728=CARTESIAN_POINT('Ctrl Pts',(-9.72629377945689,22.4830690842414,
2.35449229291434));
#102729=CARTESIAN_POINT('Ctrl Pts',(-9.73209828245168,22.4834739386758,
2.3531200436102));
#102730=CARTESIAN_POINT('Ctrl Pts',(-9.7351635684767,22.4836868271169,2.35240833492023));
#102731=CARTESIAN_POINT('Ctrl Pts',(-9.74348659928192,22.4842624983586,
2.35051098893096));
#102732=CARTESIAN_POINT('Ctrl Pts',(-9.74874976963892,22.4846239652978,
2.34934912513089));
#102733=CARTESIAN_POINT('Ctrl Pts',(-9.77295624102721,22.4862754463977,
2.34417947057636));
#102734=CARTESIAN_POINT('Ctrl Pts',(-9.79198976176031,22.487543193226,2.34060282628503));
#102735=CARTESIAN_POINT('Ctrl Pts',(-9.81110406371156,22.4887934941609,
2.33749693000246));
#102736=CARTESIAN_POINT('Origin',(-10.,12.3756328852638,3.5));
#102737=CARTESIAN_POINT('',(-9.81110406371069,23.0867835801461,2.3374969300026));
#102738=CARTESIAN_POINT('',(-9.81110406371074,22.9869701371802,2.33749693000259));
#102739=CARTESIAN_POINT('',(-9.81110406371068,12.3756328852638,2.3374969300026));
#102740=CARTESIAN_POINT('Ctrl Pts',(-9.8111040637107,23.0867835801461,2.3374969300026));
#102741=CARTESIAN_POINT('Ctrl Pts',(-9.751178490704,23.0830160202839,2.347234278241));
#102742=CARTESIAN_POINT('Ctrl Pts',(-9.69207037239346,23.079201471488,2.36159457127933));
#102743=CARTESIAN_POINT('Ctrl Pts',(-9.62000848223303,23.0742571631329,
2.38513328343377));
#102744=CARTESIAN_POINT('Ctrl Pts',(-9.60580053016976,23.0732679368808,
2.39007743795704));
#102745=CARTESIAN_POINT('Ctrl Pts',(-9.585453107092,23.0718285213703,2.39759799862038));
#102746=CARTESIAN_POINT('Ctrl Pts',(-9.57923429217758,23.0713854916472,
2.39995658488689));
#102747=CARTESIAN_POINT('Ctrl Pts',(-9.56832658723452,23.070602795237,2.40419953436903));
#102748=CARTESIAN_POINT('Ctrl Pts',(-9.56362918267486,23.0702638746225,
2.40606165430127));
#102749=CARTESIAN_POINT('Ctrl Pts',(-9.55394898344562,23.0695615340065,
2.40997129725149));
#102750=CARTESIAN_POINT('Ctrl Pts',(-9.54896797150063,23.0691979842158,
2.4120228909651));
#102751=CARTESIAN_POINT('Ctrl Pts',(-9.53621086116104,23.0682612326462,
2.41737998813079));
#102752=CARTESIAN_POINT('Ctrl Pts',(-9.52845605483273,23.0676863731341,
2.42073508502336));
#102753=CARTESIAN_POINT('Ctrl Pts',(-9.49555648831778,23.065223823561,2.43539126066882));
#102754=CARTESIAN_POINT('Ctrl Pts',(-9.47077840523181,23.0633093565331,
2.44748904607397));
#102755=CARTESIAN_POINT('Ctrl Pts',(-9.35860417055929,23.0543551047048,
2.50722045017388));
#102756=CARTESIAN_POINT('Ctrl Pts',(-9.27705128891861,23.0469716630282,
2.56493900388996));
#102757=CARTESIAN_POINT('Ctrl Pts',(-9.18745916098188,23.0381091525356,
2.647145485005));
#102758=CARTESIAN_POINT('Ctrl Pts',(-9.17159883438843,23.0365088076013,
2.66254251359347));
#102759=CARTESIAN_POINT('Ctrl Pts',(-9.14094518393495,23.0333659222212,
2.69402430286012));
#102760=CARTESIAN_POINT('Ctrl Pts',(-9.12614682421654,23.0318234942734,
2.71009318411981));
#102761=CARTESIAN_POINT('Ctrl Pts',(-9.10818058185257,23.0299282155362,
2.73072526878453));
#102762=CARTESIAN_POINT('Ctrl Pts',(-9.10458749754778,23.0295479903052,
2.73491050188852));
#102763=CARTESIAN_POINT('Ctrl Pts',(-9.09895188363171,23.0289499392386,
2.74156896130162));
#102764=CARTESIAN_POINT('Ctrl Pts',(-9.09688988196361,23.0287307571406,
2.74402548733671));
#102765=CARTESIAN_POINT('Ctrl Pts',(-9.09322336460718,23.0283404178905,
2.74842993381425));
#102766=CARTESIAN_POINT('Ctrl Pts',(-9.09161508295561,23.0281689936773,
2.75037457784156));
#102767=CARTESIAN_POINT('Ctrl Pts',(-9.0877695791583,23.0277585909487,2.75505489449824));
#102768=CARTESIAN_POINT('Ctrl Pts',(-9.08553840627414,23.0275200455541,
2.75779548280745));
#102769=CARTESIAN_POINT('Ctrl Pts',(-9.07878073130715,23.0267960916564,
2.76617278471099));
#102770=CARTESIAN_POINT('Ctrl Pts',(-9.07429365720912,23.0263133736313,
2.77184129730732));
#102771=CARTESIAN_POINT('Ctrl Pts',(-9.03422461456419,23.0219806289653,
2.82342951931208));
#102772=CARTESIAN_POINT('Ctrl Pts',(-9.00202823893325,23.0183372044505,
2.87188855632511));
#102773=CARTESIAN_POINT('Ctrl Pts',(-8.92383010259879,23.0084392756755,
3.01088770814555));
#102774=CARTESIAN_POINT('Ctrl Pts',(-8.88574396555258,23.0022659856779,
3.10527994350012));
#102775=CARTESIAN_POINT('Ctrl Pts',(-8.85680672798537,22.9947532088867,
3.21647352985328));
#102776=CARTESIAN_POINT('Ctrl Pts',(-8.8536252171123,22.993861882147,3.22962442973756));
#102777=CARTESIAN_POINT('Ctrl Pts',(-8.84926353835541,22.9925352883519,
3.24911714285368));
#102778=CARTESIAN_POINT('Ctrl Pts',(-8.84790770158202,22.9921055911176,
3.25541883696982));
#102779=CARTESIAN_POINT('Ctrl Pts',(-8.84559072287574,22.9913391912972,
3.26663472064089));
#102780=CARTESIAN_POINT('Ctrl Pts',(-8.84460905456937,22.9910031472258,
3.27154454567591));
#102781=CARTESIAN_POINT('Ctrl Pts',(-8.84260882160657,22.9902937479081,
3.28189149129765));
#102782=CARTESIAN_POINT('Ctrl Pts',(-8.8415971981809,22.9899201823506,3.28732981327721));
#102783=CARTESIAN_POINT('Ctrl Pts',(-8.8390208088264,22.9889280705859,3.30174411591937));
#102784=CARTESIAN_POINT('Ctrl Pts',(-8.83752185456827,22.9883074731128,
3.31073132542408));
#102785=CARTESIAN_POINT('Ctrl Pts',(-8.83082479147894,22.9853112918499,
3.3539705572244));
#102786=CARTESIAN_POINT('Ctrl Pts',(-8.82703589878992,22.9828922857979,
3.38842018872435));
#102787=CARTESIAN_POINT('Ctrl Pts',(-8.8204111533025,22.9756962939875,3.4895105468395));
#102788=CARTESIAN_POINT('Ctrl Pts',(-8.82170864262925,22.9708127131509,
3.55628058586012));
#102789=CARTESIAN_POINT('Ctrl Pts',(-8.83505326406694,22.9613976441742,
3.68380563593608));
#102790=CARTESIAN_POINT('Ctrl Pts',(-8.84625276007084,22.9568842466013,
3.74444685178082));
#102791=CARTESIAN_POINT('Ctrl Pts',(-8.86466004880756,22.9518860704531,
3.81335810222273));
#102792=CARTESIAN_POINT('Ctrl Pts',(-8.86729289943504,22.9512081985965,
3.82274563483428));
#102793=CARTESIAN_POINT('Ctrl Pts',(-8.87108549214189,22.9502815568797,
3.835649799364));
#102794=CARTESIAN_POINT('Ctrl Pts',(-8.87214560527832,22.9500275223116,
3.83919495736716));
#102795=CARTESIAN_POINT('Ctrl Pts',(-8.87399213090569,22.9495935184387,
3.84526560359985));
#102796=CARTESIAN_POINT('Ctrl Pts',(-8.87477036713728,22.9494130902777,
3.847793519165));
#102797=CARTESIAN_POINT('Ctrl Pts',(-8.87641329078853,22.9490373587804,
3.85306692634283));
#102798=CARTESIAN_POINT('Ctrl Pts',(-8.87727953529114,22.9488421540607,
3.85581189687584));
#102799=CARTESIAN_POINT('Ctrl Pts',(-8.87941876427522,22.9483670312179,
3.86250512474029));
#102800=CARTESIAN_POINT('Ctrl Pts',(-8.88070257873264,22.9480877352461,
3.8664499356919));
#102801=CARTESIAN_POINT('Ctrl Pts',(-8.88539754270523,22.9470867324137,
3.88062138938491));
#102802=CARTESIAN_POINT('Ctrl Pts',(-8.8889283470235,22.946371595946,3.89080824224801));
#102803=CARTESIAN_POINT('Ctrl Pts',(-8.8980964020739,22.9446016289321,3.91613017065139));
#102804=CARTESIAN_POINT('Ctrl Pts',(-8.90390614235746,22.9435551365598,
3.93120084378869));
#102805=CARTESIAN_POINT('Ctrl Pts',(-8.9307515929507,22.9390117608701,3.99678645093033));
#102806=CARTESIAN_POINT('Ctrl Pts',(-8.95498424295203,22.9356341429664,
4.04592302664047));
#102807=CARTESIAN_POINT('Ctrl Pts',(-9.02341368975843,22.9272357802339,
4.16329278718968));
#102808=CARTESIAN_POINT('Ctrl Pts',(-9.07140770928212,22.9222185825489,
4.2289666633575));
#102809=CARTESIAN_POINT('Ctrl Pts',(-9.13584619806587,22.9159465830941,
4.30034964010879));
#102810=CARTESIAN_POINT('Ctrl Pts',(-9.14613844965934,22.9149573771656,
4.31132099636075));
#102811=CARTESIAN_POINT('Ctrl Pts',(-9.16128015955294,22.9135179859253,
4.32685447786994));
#102812=CARTESIAN_POINT('Ctrl Pts',(-9.16596286344667,22.913074959806,4.33157762724275));
#102813=CARTESIAN_POINT('Ctrl Pts',(-9.17427314705011,22.912292267597,4.33981888523157));
#102814=CARTESIAN_POINT('Ctrl Pts',(-9.17788386543568,22.9119533475543,
4.34335381400726));
#102815=CARTESIAN_POINT('Ctrl Pts',(-9.18539072392015,22.9112510060069,
4.35060908162623));
#102816=CARTESIAN_POINT('Ctrl Pts',(-9.18928985891481,22.9108874547001,
4.35432613672612));
#102817=CARTESIAN_POINT('Ctrl Pts',(-9.19936996860191,22.9099506947303,
4.36380438174757));
#102818=CARTESIAN_POINT('Ctrl Pts',(-9.20558760151119,22.9093758282771,
4.36952595806485));
#102819=CARTESIAN_POINT('Ctrl Pts',(-9.23235202199716,22.9069132065865,
4.39362836702318));
#102820=CARTESIAN_POINT('Ctrl Pts',(-9.25347772717576,22.9049986724255,
4.41135029094205));
#102821=CARTESIAN_POINT('Ctrl Pts',(-9.35364843628494,22.8960443939538,
4.48956018440189));
#102822=CARTESIAN_POINT('Ctrl Pts',(-9.43953234870287,22.8886610032355,
4.54061028983103));
#102823=CARTESIAN_POINT('Ctrl Pts',(-9.55105769518797,22.8797985408336,
4.5890519957481));
#102824=CARTESIAN_POINT('Ctrl Pts',(-9.57157228371355,22.8781981904997,
4.59728447921133));
#102825=CARTESIAN_POINT('Ctrl Pts',(-9.61279560933652,22.8750553330705,
4.61249482770354));
#102826=CARTESIAN_POINT('Ctrl Pts',(-9.63349187484446,22.8735129375136,
4.61948377621964));
#102827=CARTESIAN_POINT('Ctrl Pts',(-9.65964498676793,22.8716176926594,
4.62751228428989));
#102828=CARTESIAN_POINT('Ctrl Pts',(-9.66492933730371,22.8712374700557,
4.62909394660222));
#102829=CARTESIAN_POINT('Ctrl Pts',(-9.67330360897312,22.8706394221968,
4.63153648483219));
#102830=CARTESIAN_POINT('Ctrl Pts',(-9.67638618673021,22.8704202407028,
4.63242193942965));
#102831=CARTESIAN_POINT('Ctrl Pts',(-9.68190070177898,22.8700299019667,
4.63398159921538));
#102832=CARTESIAN_POINT('Ctrl Pts',(-9.68433117632398,22.869858477668,4.63466057692419));
#102833=CARTESIAN_POINT('Ctrl Pts',(-9.69017051742674,22.8694480740127,
4.63627164126254));
#102834=CARTESIAN_POINT('Ctrl Pts',(-9.69358141641125,22.8692095277826,
4.63719620271137));
#102835=CARTESIAN_POINT('Ctrl Pts',(-9.70398233724887,22.8684855687757,
4.63996529209301));
#102836=CARTESIAN_POINT('Ctrl Pts',(-9.71098538643763,22.8680028465326,
4.64176086965066));
#102837=CARTESIAN_POINT('Ctrl Pts',(-9.77440889144461,22.8636699489553,
4.65740166925768));
#102838=CARTESIAN_POINT('Ctrl Pts',(-9.83177334691347,22.8600263916886,
4.66712110628741));
#102839=CARTESIAN_POINT('Ctrl Pts',(-9.99055656767438,22.8501285153288,
4.68206713353976));
#102840=CARTESIAN_POINT('Ctrl Pts',(-10.0922772414015,22.8439553906687,
4.67849681731113));
#102841=CARTESIAN_POINT('Ctrl Pts',(-10.2056303536822,22.8364427864322,
4.65973888621556));
#102842=CARTESIAN_POINT('Ctrl Pts',(-10.2189394052176,22.8355514355074,
4.65730015068657));
#102843=CARTESIAN_POINT('Ctrl Pts',(-10.2385225069046,22.8342248125344,
4.65336188023546));
#102844=CARTESIAN_POINT('Ctrl Pts',(-10.2448313088402,22.8337951106678,
4.65203916622086));
#102845=CARTESIAN_POINT('Ctrl Pts',(-10.2560207076755,22.8330287056575,
4.64959711640558));
#102846=CARTESIAN_POINT('Ctrl Pts',(-10.2609056605451,22.8326926610611,
4.64849830987026));
#102847=CARTESIAN_POINT('Ctrl Pts',(-10.2711722887196,22.8319832637974,
4.64612008568311));
#102848=CARTESIAN_POINT('Ctrl Pts',(-10.2765522404055,22.8316097008387,
4.6448338383775));
#102849=CARTESIAN_POINT('Ctrl Pts',(-10.2907690779143,22.8306176033824,
4.64132879492533));
#102850=CARTESIAN_POINT('Ctrl Pts',(-10.2995894732042,22.8299970177244,
4.6390453082358));
#102851=CARTESIAN_POINT('Ctrl Pts',(-10.3418155454092,22.8270009915379,
4.627589134115));
#102852=CARTESIAN_POINT('Ctrl Pts',(-10.3748290111891,22.8245821342223,
4.61704874805799));
#102853=CARTESIAN_POINT('Ctrl Pts',(-10.4698757177248,22.8173868189739,
4.58201465924872));
#102854=CARTESIAN_POINT('Ctrl Pts',(-10.5303474313801,22.8125037917916,
4.55369287113804));
#102855=CARTESIAN_POINT('Ctrl Pts',(-10.6414416516414,22.8030885404692,
4.48966620873711));
#102856=CARTESIAN_POINT('Ctrl Pts',(-10.6923033371855,22.7985744075567,
4.45477967851165));
#102857=CARTESIAN_POINT('Ctrl Pts',(-10.7477903296272,22.7935755563251,
4.40994490365898));
#102858=CARTESIAN_POINT('Ctrl Pts',(-10.7552971661018,22.7928976852761,
4.40372358115197));
#102859=CARTESIAN_POINT('Ctrl Pts',(-10.7655456090146,22.7919710444605,
4.39501322580882));
#102860=CARTESIAN_POINT('Ctrl Pts',(-10.7683537751204,22.7917170099989,
4.39260362482078));
#102861=CARTESIAN_POINT('Ctrl Pts',(-10.773149726938,22.7912830062645,4.38844896196955));
#102862=CARTESIAN_POINT('Ctrl Pts',(-10.7751430538494,22.791102578136,4.38671038378503));
#102863=CARTESIAN_POINT('Ctrl Pts',(-10.779293359031,22.79072684665,4.38306580058673));
#102864=CARTESIAN_POINT('Ctrl Pts',(-10.7814492282923,22.7905316419095,
4.38115858472673));
#102865=CARTESIAN_POINT('Ctrl Pts',(-10.7866950358297,22.7900565189346,
4.3764834236517));
#102866=CARTESIAN_POINT('Ctrl Pts',(-10.7897774231587,22.7897772228524,
4.37370698435284));
#102867=CARTESIAN_POINT('Ctrl Pts',(-10.8008169682858,22.7887762191819,
4.36365702880626));
#102868=CARTESIAN_POINT('Ctrl Pts',(-10.8086891347469,22.7880610820009,
4.35629036187227));
#102869=CARTESIAN_POINT('Ctrl Pts',(-10.8280982614162,22.7862911128643,
4.33762111255625));
#102870=CARTESIAN_POINT('Ctrl Pts',(-10.8395062665342,22.7852446191083,
4.32618711053092));
#102871=CARTESIAN_POINT('Ctrl Pts',(-10.8885174577236,22.780701233503,4.27500043614223));
#102872=CARTESIAN_POINT('Ctrl Pts',(-10.9235618016018,22.7773236075959,
4.23288709704573));
#102873=CARTESIAN_POINT('Ctrl Pts',(-11.0029831913953,22.7689252475592,
4.12265787682346));
#102874=CARTESIAN_POINT('Ctrl Pts',(-11.0434784642931,22.7639080602669,
4.05211294508536));
#102875=CARTESIAN_POINT('Ctrl Pts',(-11.0825057016338,22.7576360722458,
3.96422273306177));
#102876=CARTESIAN_POINT('Ctrl Pts',(-11.088346276408,22.756646866013,3.95035951089803));
#102877=CARTESIAN_POINT('Ctrl Pts',(-11.0963839103617,22.7552074744053,
3.93021113356674));
#102878=CARTESIAN_POINT('Ctrl Pts',(-11.0987958727566,22.7547644482282,
3.92401288341935));
#102879=CARTESIAN_POINT('Ctrl Pts',(-11.1029476784655,22.7539817559477,
3.91307022919081));
#102880=CARTESIAN_POINT('Ctrl Pts',(-11.1047097434336,22.7536428358918,
3.90833439369775));
#102881=CARTESIAN_POINT('Ctrl Pts',(-11.1082872586754,22.752940494347,3.89852657963515));
#102882=CARTESIAN_POINT('Ctrl Pts',(-11.1100984913735,22.7525769430562,
3.89345319950344));
#102883=CARTESIAN_POINT('Ctrl Pts',(-11.1146610949147,22.7516401831913,
3.88039072092305));
#102884=CARTESIAN_POINT('Ctrl Pts',(-11.1173613716986,22.7510653168277,
3.87238423118512));
#102885=CARTESIAN_POINT('Ctrl Pts',(-11.1285037661965,22.7486026961152,
3.83813359112886));
#102886=CARTESIAN_POINT('Ctrl Pts',(-11.1361085495252,22.7466881628699,
3.81162833569484));
#102887=CARTESIAN_POINT('Ctrl Pts',(-11.1668491146724,22.737733884525,3.68831582163793));
#102888=CARTESIAN_POINT('Ctrl Pts',(-11.1785820311721,22.7303504928557,
3.58909636281973));
#102889=CARTESIAN_POINT('Ctrl Pts',(-11.1775091561932,22.7214880295139,
3.46750954637182));
#102890=CARTESIAN_POINT('Ctrl Pts',(-11.1766922042522,22.7198876791792,
3.44541984925432));
#102891=CARTESIAN_POINT('Ctrl Pts',(-11.1738330866712,22.7167448218033,
3.40157304017101));
#102892=CARTESIAN_POINT('Ctrl Pts',(-11.1718061170206,22.7152024262992,
3.37982281786415));
#102893=CARTESIAN_POINT('Ctrl Pts',(-11.1685108839151,22.7133071814942,
3.35266432737117));
#102894=CARTESIAN_POINT('Ctrl Pts',(-11.1678080343469,22.7129269588897,
3.3471933111132));
#102895=CARTESIAN_POINT('Ctrl Pts',(-11.1666357598958,22.7123289110269,
3.33854922685531));
#102896=CARTESIAN_POINT('Ctrl Pts',(-11.1661917765163,22.7121097295298,
3.33537287760948));
#102897=CARTESIAN_POINT('Ctrl Pts',(-11.1653752680284,22.7117193907882,
3.32970051216835));
#102898=CARTESIAN_POINT('Ctrl Pts',(-11.1650076979605,22.7115479664872,
3.32720389252114));
#102899=CARTESIAN_POINT('Ctrl Pts',(-11.1641061223085,22.7111375628252,
3.32121385117013));
#102900=CARTESIAN_POINT('Ctrl Pts',(-11.1635644151219,22.7108990165907,
3.3177216313102));
#102901=CARTESIAN_POINT('Ctrl Pts',(-11.1618667165516,22.7101750575611,
3.30709313954435));
#102902=CARTESIAN_POINT('Ctrl Pts',(-11.160660705781,22.7096923352997,3.2999648621416));
#102903=CARTESIAN_POINT('Ctrl Pts',(-11.1491710637265,22.7053594371209,
3.23565961416983));
#102904=CARTESIAN_POINT('Ctrl Pts',(-11.1347341459828,22.7017158793319,
3.17929717413292));
#102905=CARTESIAN_POINT('Ctrl Pts',(-11.0838485488928,22.6918180300698,
3.02814820180221));
#102906=CARTESIAN_POINT('Ctrl Pts',(-11.0392398600315,22.6856449322495,
2.93666150420985));
#102907=CARTESIAN_POINT('Ctrl Pts',(-10.9760264812506,22.6781323423325,
2.84071975452016));
#102908=CARTESIAN_POINT('Ctrl Pts',(-10.9683883585278,22.6772409731502,
2.82955082472361));
#102909=CARTESIAN_POINT('Ctrl Pts',(-10.9568298884922,22.6759143281443,
2.8132590166168));
#102910=CARTESIAN_POINT('Ctrl Pts',(-10.95305697729,22.6754846227743,2.80803250869444));
#102911=CARTESIAN_POINT('Ctrl Pts',(-10.9463828327682,22.6747301183026,
2.79894513986962));
#102912=CARTESIAN_POINT('Ctrl Pts',(-10.943500376574,22.6744060461559,2.79507062673994));
#102913=CARTESIAN_POINT('Ctrl Pts',(-10.9404984449235,22.6740703401572,
2.79108691441192));
#102914=CARTESIAN_POINT('Ctrl Pts',(-10.9404026542334,22.6740596297606,
2.79095984899853));
#102915=CARTESIAN_POINT('Ctrl Pts',(-10.9401945068614,22.6740363607883,
2.79068385992561));
#102916=CARTESIAN_POINT('Ctrl Pts',(-10.9400821405552,22.6740238018383,
2.79053494355861));
#102917=CARTESIAN_POINT('Ctrl Pts',(-10.9366849798909,22.6736441859637,
2.78603499222511));
#102918=CARTESIAN_POINT('Ctrl Pts',(-10.9333700980759,22.6732759603372,
2.78170685499116));
#102919=CARTESIAN_POINT('Ctrl Pts',(-10.9244908013384,22.6722953019204,
2.7702786883632));
#102920=CARTESIAN_POINT('Ctrl Pts',(-10.9188747522893,22.6716808474911,
2.76321942470442));
#102921=CARTESIAN_POINT('Ctrl Pts',(-10.9063397076008,22.6703216620176,
2.74782936847711));
#102922=CARTESIAN_POINT('Ctrl Pts',(-10.8993858476592,22.6695755755493,
2.7395281675355));
#102923=CARTESIAN_POINT('Ctrl Pts',(-10.8781144460172,22.6673163496157,
2.71483521988049));
#102924=CARTESIAN_POINT('Ctrl Pts',(-10.86345670748,22.6657898444177,2.69874403466731));
#102925=CARTESIAN_POINT('Ctrl Pts',(-10.8043753815629,22.65975128346,2.63738955702079));
#102926=CARTESIAN_POINT('Ctrl Pts',(-10.7567755782989,22.6551196603724,
2.59534229879862));
#102927=CARTESIAN_POINT('Ctrl Pts',(-10.6524475488982,22.6455488522504,
2.51720360213104));
#102928=CARTESIAN_POINT('Ctrl Pts',(-10.595536589942,22.640624500551,2.48171002477099));
#102929=CARTESIAN_POINT('Ctrl Pts',(-10.5272797096882,22.6352538046754,
2.44683089371647));
#102930=CARTESIAN_POINT('Ctrl Pts',(-10.5185919055761,22.6345797294726,
2.44252588240749));
#102931=CARTESIAN_POINT('Ctrl Pts',(-10.5065223244178,22.633657303694,2.43672964980951));
#102932=CARTESIAN_POINT('Ctrl Pts',(-10.5031855043475,22.633403751244,2.43514646459337));
#102933=CARTESIAN_POINT('Ctrl Pts',(-10.4974479587568,22.6329703555232,
2.43245722477787));
#102934=CARTESIAN_POINT('Ctrl Pts',(-10.4950508818725,22.6327900561641,
2.43134351950177));
#102935=CARTESIAN_POINT('Ctrl Pts',(-10.4900341296499,22.6324143479675,
2.42903318978926));
#102936=CARTESIAN_POINT('Ctrl Pts',(-10.4874137881076,22.6322190389804,
2.42783809235608));
#102937=CARTESIAN_POINT('Ctrl Pts',(-10.4810009339065,22.631743261178,2.42494165675585));
#102938=CARTESIAN_POINT('Ctrl Pts',(-10.4772036990365,22.6314634185973,
2.42325073915324));
#102939=CARTESIAN_POINT('Ctrl Pts',(-10.4634762491885,22.6304582349115,
2.41722475643673));
#102940=CARTESIAN_POINT('Ctrl Pts',(-10.4534949120126,22.6297395365565,
2.41300651009185));
#102941=CARTESIAN_POINT('Ctrl Pts',(-10.428393497874,22.6279589537935,2.40280428198749));
#102942=CARTESIAN_POINT('Ctrl Pts',(-10.4132046846674,22.6269055364922,
2.39699438958741));
#102943=CARTESIAN_POINT('Ctrl Pts',(-10.3457550286884,22.6223122430691,
2.37278310438681));
#102944=CARTESIAN_POINT('Ctrl Pts',(-10.2923504182,22.6188943098857,2.35776680383763));
#102945=CARTESIAN_POINT('Ctrl Pts',(-10.1803869570358,22.6118273598725,
2.33465613649588));
#102946=CARTESIAN_POINT('Ctrl Pts',(-10.1218823962121,22.6081858122779,
2.32709345723607));
#102947=CARTESIAN_POINT('Ctrl Pts',(-10.0320757670174,22.6024488935694,
2.32227804859184));
#102948=CARTESIAN_POINT('Ctrl Pts',(-10.0010403120032,22.6004408014835,
2.3218419022633));
#102949=CARTESIAN_POINT('Ctrl Pts',(-9.96089153893417,22.5977923301093,
2.32286403517224));
#102950=CARTESIAN_POINT('Ctrl Pts',(-9.95176050739249,22.5971866256816,
2.32320286583241));
#102951=CARTESIAN_POINT('Ctrl Pts',(-9.93710380885206,22.5962085672495,
2.32391760769405));
#102952=CARTESIAN_POINT('Ctrl Pts',(-9.93157511943903,22.5958383027342,
2.3242263150194));
#102953=CARTESIAN_POINT('Ctrl Pts',(-9.92120640916872,22.5951413099788,
2.32487865520179));
#102954=CARTESIAN_POINT('Ctrl Pts',(-9.91636591902299,22.5948148702439,
2.32521323456465));
#102955=CARTESIAN_POINT('Ctrl Pts',(-9.90670274303069,22.5941610195652,
2.32594118689477));
#102956=CARTESIAN_POINT('Ctrl Pts',(-9.90188013924116,22.593833620134,2.32633438897631));
#102957=CARTESIAN_POINT('Ctrl Pts',(-9.89089078943258,22.5930850443722,
2.32729859010483));
#102958=CARTESIAN_POINT('Ctrl Pts',(-9.88472589228886,22.5926632863752,
2.32788853169215));
#102959=CARTESIAN_POINT('Ctrl Pts',(-9.85599229840556,22.5906888598805,
2.33086703344397));
#102960=CARTESIAN_POINT('Ctrl Pts',(-9.83350225220027,22.5891183274746,
2.33385743237855));
#102961=CARTESIAN_POINT('Ctrl Pts',(-9.81110404738658,22.5875279348072,
2.33749693265511));
#102962=CARTESIAN_POINT('Ctrl Pts',(-9.81110406371156,22.4887934941609,
2.33749693000246));
#102963=CARTESIAN_POINT('Ctrl Pts',(-9.81147112136522,22.4888175040634,
2.33743728654779));
#102964=CARTESIAN_POINT('Ctrl Pts',(-9.81183820880857,22.488841507528,2.33737781668908));
#102965=CARTESIAN_POINT('Ctrl Pts',(-9.85155032860022,22.4914373403487,
2.33096357106418));
#102966=CARTESIAN_POINT('Ctrl Pts',(-9.89119577716716,22.493933679374,2.32660934983867));
#102967=CARTESIAN_POINT('Ctrl Pts',(-10.0285358260178,22.502478031877,2.31854791086634));
#102968=CARTESIAN_POINT('Ctrl Pts',(-10.1264065581075,22.5084226337522,
2.32498376589142));
#102969=CARTESIAN_POINT('Ctrl Pts',(-10.2388190935285,22.5158639769365,
2.34659567678142));
#102970=CARTESIAN_POINT('Ctrl Pts',(-10.2552113863922,22.5169636356785,
2.35011165989876));
#102971=CARTESIAN_POINT('Ctrl Pts',(-10.2778488043926,22.5185050531027,
2.35547504427309));
#102972=CARTESIAN_POINT('Ctrl Pts',(-10.2841625673003,22.5189374467861,
2.35702626237878));
#102973=CARTESIAN_POINT('Ctrl Pts',(-10.2950356665279,22.5196865205771,
2.3597933166146));
#102974=CARTESIAN_POINT('Ctrl Pts',(-10.2996011824306,22.5200024067507,
2.36098443568946));
#102975=CARTESIAN_POINT('Ctrl Pts',(-10.3090487474681,22.5206589572948,
2.36350998743947));
#102976=CARTESIAN_POINT('Ctrl Pts',(-10.3139295904058,22.520999747303,2.36484851766386));
#102977=CARTESIAN_POINT('Ctrl Pts',(-10.325373120717,22.5218025968335,2.36806625889796));
#102978=CARTESIAN_POINT('Ctrl Pts',(-10.3319283392438,22.5222654748031,
2.36997113482653));
#102979=CARTESIAN_POINT('Ctrl Pts',(-10.3534428339781,22.523794708362,2.37642636754206));
#102980=CARTESIAN_POINT('Ctrl Pts',(-10.3683275266647,22.5248687923098,
2.38121747572462));
#102981=CARTESIAN_POINT('Ctrl Pts',(-10.4034658004634,22.5274440870409,
2.39330504689871));
#102982=CARTESIAN_POINT('Ctrl Pts',(-10.4236228055717,22.5289533353942,
2.40086307101975));
#102983=CARTESIAN_POINT('Ctrl Pts',(-10.5011617362671,22.5348849452216,
2.43238663638491));
#102984=CARTESIAN_POINT('Ctrl Pts',(-10.5568119147752,22.5394222443518,
2.46032685739353));
#102985=CARTESIAN_POINT('Ctrl Pts',(-10.6687350402838,22.5490281612899,
2.52809236099422));
#102986=CARTESIAN_POINT('Ctrl Pts',(-10.724261561519,22.5540849841267,2.56873312236311));
#102987=CARTESIAN_POINT('Ctrl Pts',(-10.7831945367248,22.5595732580376,
2.62034408004894));
#102988=CARTESIAN_POINT('Ctrl Pts',(-10.7903773918459,22.5602442731153,
2.62679222784452));
#102989=CARTESIAN_POINT('Ctrl Pts',(-10.8001934207664,22.5611632350731,
2.63582458724426));
#102990=CARTESIAN_POINT('Ctrl Pts',(-10.8028947041331,22.5614163340016,
2.63833373650506));
#102991=CARTESIAN_POINT('Ctrl Pts',(-10.8075106366579,22.5618491190787,
2.6426619055685));
#102992=CARTESIAN_POINT('Ctrl Pts',(-10.8094310108728,22.5620292589124,
2.64447473709484));
#102993=CARTESIAN_POINT('Ctrl Pts',(-10.8134330263759,22.5624048188505,
2.64827817362354));
#102994=CARTESIAN_POINT('Ctrl Pts',(-10.8155134846138,22.562600138252,2.65026997547042));
#102995=CARTESIAN_POINT('Ctrl Pts',(-10.8205818650077,22.5630762380493,
2.65515813227322));
#102996=CARTESIAN_POINT('Ctrl Pts',(-10.823561822078,22.5633563896119,2.65806276648798));
#102997=CARTESIAN_POINT('Ctrl Pts',(-10.8342713546468,22.5643643261544,
2.66861286637392));
#102998=CARTESIAN_POINT('Ctrl Pts',(-10.8419106591018,22.5650854190019,
2.67634975740693));
#102999=CARTESIAN_POINT('Ctrl Pts',(-10.8607572041319,22.5668732444412,
2.69597329809755));
#103000=CARTESIAN_POINT('Ctrl Pts',(-10.8718266082196,22.5679314196791,
2.70798969507191));
#103001=CARTESIAN_POINT('Ctrl Pts',(-10.9196437305343,22.5725597724467,
2.76211541975835));
#103002=CARTESIAN_POINT('Ctrl Pts',(-10.9536195014925,22.5760060963925,
2.80658159902901));
#103003=CARTESIAN_POINT('Ctrl Pts',(-11.0280257184825,22.5843824230875,
2.91983096405164));
#103004=CARTESIAN_POINT('Ctrl Pts',(-11.0648762191173,22.5893111180967,
2.99061845228588));
#103005=CARTESIAN_POINT('Ctrl Pts',(-11.09987716372,22.5954853845657,3.07858273864619));
#103006=CARTESIAN_POINT('Ctrl Pts',(-11.1051804603674,22.5964766165181,
3.09269372736918));
#103007=CARTESIAN_POINT('Ctrl Pts',(-11.1124325760055,22.5979183380969,
3.11317559901439));
#103008=CARTESIAN_POINT('Ctrl Pts',(-11.114600609015,22.5983616336624,3.1194676982417));
#103009=CARTESIAN_POINT('Ctrl Pts',(-11.1183205163343,22.5991445485932,
3.1305682585376));
#103010=CARTESIAN_POINT('Ctrl Pts',(-11.1198950063468,22.5994834194811,
3.13536900536065));
#103011=CARTESIAN_POINT('Ctrl Pts',(-11.1230830053116,22.6001854109187,
3.14530492228476));
#103012=CARTESIAN_POINT('Ctrl Pts',(-11.1246922942466,22.6005486596762,
3.15044131169001));
#103013=CARTESIAN_POINT('Ctrl Pts',(-11.128732911939,22.6014841112113,3.16365460811502));
#103014=CARTESIAN_POINT('Ctrl Pts',(-11.131112747975,22.6020579639269,3.17174681409444));
#103015=CARTESIAN_POINT('Ctrl Pts',(-11.140866077134,22.6045112069916,3.20627734420504));
#103016=CARTESIAN_POINT('Ctrl Pts',(-11.1474005465787,22.6064171272024,
3.23294162966112));
#103017=CARTESIAN_POINT('Ctrl Pts',(-11.1733054455582,22.6153654662514,
3.35729330379808));
#103018=CARTESIAN_POINT('Ctrl Pts',(-11.1811654032006,22.6227525912476,
3.45695127777926));
#103019=CARTESIAN_POINT('Ctrl Pts',(-11.1753423374674,22.6316183019501,
3.57844129287645));
#103020=CARTESIAN_POINT('Ctrl Pts',(-11.1736650577098,22.6332174831642,
3.60046428410857));
#103021=CARTESIAN_POINT('Ctrl Pts',(-11.1690890239858,22.6363665548424,
3.6442469414909));
#103022=CARTESIAN_POINT('Ctrl Pts',(-11.1661992143519,22.6379161220559,
3.6659996073744));
#103023=CARTESIAN_POINT('Ctrl Pts',(-11.161823143084,22.6398187828371,3.69311278846275));
#103024=CARTESIAN_POINT('Ctrl Pts',(-11.1609047724736,22.640199503536,3.69855900163287));
#103025=CARTESIAN_POINT('Ctrl Pts',(-11.1593924178605,22.6407981139688,
3.70715833577478));
#103026=CARTESIAN_POINT('Ctrl Pts',(-11.1588238176981,22.6410173646873,
3.71031575032225));
#103027=CARTESIAN_POINT('Ctrl Pts',(-11.157785133408,22.6414076902399,3.71595140548517));
#103028=CARTESIAN_POINT('Ctrl Pts',(-11.1573199923684,22.6415790330228,
3.71843044686254));
#103029=CARTESIAN_POINT('Ctrl Pts',(-11.1561848530464,22.6419890611733,
3.72437492187632));
#103030=CARTESIAN_POINT('Ctrl Pts',(-11.1555072373839,22.6422273151463,
3.72783885786239));
#103031=CARTESIAN_POINT('Ctrl Pts',(-11.1533979532726,22.6429497423578,
3.73836991508846));
#103032=CARTESIAN_POINT('Ctrl Pts',(-11.1519169148759,22.6434312407912,
3.74542714334026));
#103033=CARTESIAN_POINT('Ctrl Pts',(-11.1356474007692,22.6484656539802,
3.81955848126425));
#103034=CARTESIAN_POINT('Ctrl Pts',(-11.1150807901605,22.6527284782774,
3.88524064942433));
#103035=CARTESIAN_POINT('Ctrl Pts',(-11.0549897510122,22.6624843743005,
4.03104857018291));
#103036=CARTESIAN_POINT('Ctrl Pts',(-11.0118651569389,22.6679546790693,
4.10921477243793));
#103037=CARTESIAN_POINT('Ctrl Pts',(-10.9518351398395,22.674721762686,4.19377331474239));
#103038=CARTESIAN_POINT('Ctrl Pts',(-10.9430941193624,22.6756896939809,
4.20560966281997));
#103039=CARTESIAN_POINT('Ctrl Pts',(-10.9301195407496,22.6771035646855,
4.22250685198628));
#103040=CARTESIAN_POINT('Ctrl Pts',(-10.9260613649033,22.6775426982204,
4.22770107648143));
#103041=CARTESIAN_POINT('Ctrl Pts',(-10.9188224618674,22.6783207678073,
4.23680782283906));
#103042=CARTESIAN_POINT('Ctrl Pts',(-10.915659783461,22.6786589844663,4.2407345299276));
#103043=CARTESIAN_POINT('Ctrl Pts',(-10.9090525515149,22.6793620923168,
4.2488309365469));
#103044=CARTESIAN_POINT('Ctrl Pts',(-10.9056043008041,22.679727126805,4.25299745127169));
#103045=CARTESIAN_POINT('Ctrl Pts',(-10.8966288395546,22.6806724810337,
4.26369165649639));
#103046=CARTESIAN_POINT('Ctrl Pts',(-10.8910590770366,22.6812545187207,
4.27018305397498));
#103047=CARTESIAN_POINT('Ctrl Pts',(-10.8665720213626,22.6837941794013,
4.29810083052737));
#103048=CARTESIAN_POINT('Ctrl Pts',(-10.8469504026008,22.6857807215146,
4.31889362858558));
#103049=CARTESIAN_POINT('Ctrl Pts',(-10.7562549315112,22.6947625412879,
4.40825319477484));
#103050=CARTESIAN_POINT('Ctrl Pts',(-10.6774860835743,22.7020901661018,
4.46842776188902));
#103051=CARTESIAN_POINT('Ctrl Pts',(-10.5561125603031,22.7123216985217,
4.53902478374099));
#103052=CARTESIAN_POINT('Ctrl Pts',(-10.5189771668227,22.7153221249059,
4.5580629363984));
#103053=CARTESIAN_POINT('Ctrl Pts',(-10.4754543869269,22.7186356473081,
4.5775313718774));
#103054=CARTESIAN_POINT('Ctrl Pts',(-10.4699839989109,22.7190485542376,
4.57992859760193));
#103055=CARTESIAN_POINT('Ctrl Pts',(-10.4611907064019,22.7197063048984,
4.5837025089888));
#103056=CARTESIAN_POINT('Ctrl Pts',(-10.4578794071982,22.7199526480885,
4.58510572986747));
#103057=CARTESIAN_POINT('Ctrl Pts',(-10.4519783754874,22.7203891969778,
4.58757457314159));
#103058=CARTESIAN_POINT('Ctrl Pts',(-10.4493912094941,22.7205797524303,
4.58864615256977));
#103059=CARTESIAN_POINT('Ctrl Pts',(-10.4438152979682,22.7209886243323,
4.5909323769148));
#103060=CARTESIAN_POINT('Ctrl Pts',(-10.4408253736641,22.7212067596026,
4.59214397415234));
#103061=CARTESIAN_POINT('Ctrl Pts',(-10.4324913688708,22.7218117976014,
4.59548133508704));
#103062=CARTESIAN_POINT('Ctrl Pts',(-10.4271365496538,22.7221971480358,
4.5975802981885));
#103063=CARTESIAN_POINT('Ctrl Pts',(-10.3955233433343,22.7244533815988,
4.60970552942141));
#103064=CARTESIAN_POINT('Ctrl Pts',(-10.3689258232112,22.7262758287322,
4.61882934819671));
#103065=CARTESIAN_POINT('Ctrl Pts',(-10.2711367320055,22.7327908019953,
4.64850681129185));
#103066=CARTESIAN_POINT('Ctrl Pts',(-10.1983723437466,22.7372971067394,
4.66328543607542));
#103067=CARTESIAN_POINT('Ctrl Pts',(-10.0611977866984,22.7458699248212,
4.67789125675449));
#103068=CARTESIAN_POINT('Ctrl Pts',(-9.9972620587247,22.7498964281365,4.67947608504159));
#103069=CARTESIAN_POINT('Ctrl Pts',(-9.92368738043517,22.7547379207235,
4.67531629802573));
#103070=CARTESIAN_POINT('Ctrl Pts',(-9.91386417754612,22.7553884316813,
4.67463723199335));
#103071=CARTESIAN_POINT('Ctrl Pts',(-9.89780262305695,22.7564593338705,
4.67332436275405));
#103072=CARTESIAN_POINT('Ctrl Pts',(-9.89155864602184,22.7568774530901,
4.67276375893351));
#103073=CARTESIAN_POINT('Ctrl Pts',(-9.88035703657543,22.757630924742,4.67166782237895));
#103074=CARTESIAN_POINT('Ctrl Pts',(-9.87539773048635,22.7579656991762,
4.6711508006296));
#103075=CARTESIAN_POINT('Ctrl Pts',(-9.86484506401242,22.7586806518238,
4.66998286923371));
#103076=CARTESIAN_POINT('Ctrl Pts',(-9.85925280675639,22.7590610922839,
4.66932330717715));
#103077=CARTESIAN_POINT('Ctrl Pts',(-9.84416883004046,22.7600915783859,
4.66743449979983));
#103078=CARTESIAN_POINT('Ctrl Pts',(-9.83468718398015,22.7607439680981,
4.66612963614303));
#103079=CARTESIAN_POINT('Ctrl Pts',(-9.78478032163743,22.7642031489257,
4.65864057056181));
#103080=CARTESIAN_POINT('Ctrl Pts',(-9.74468618091658,22.7670714394813,
4.65047018230721));
#103081=CARTESIAN_POINT('Ctrl Pts',(-9.60607438152136,22.7773060954421,
4.61462104282906));
#103082=CARTESIAN_POINT('Ctrl Pts',(-9.51081960894664,22.7849604029738,
4.57622314853734));
#103083=CARTESIAN_POINT('Ctrl Pts',(-9.39975463853945,22.7941176434468,
4.51362555992845));
#103084=CARTESIAN_POINT('Ctrl Pts',(-9.37818275575029,22.795905411481,4.50053725811511));
#103085=CARTESIAN_POINT('Ctrl Pts',(-9.35221351847893,22.7980544293897,
4.48361629021532));
#103086=CARTESIAN_POINT('Ctrl Pts',(-9.34740395648211,22.7984522887774,
4.48043191472639));
#103087=CARTESIAN_POINT('Ctrl Pts',(-9.33990946392472,22.799071789127,4.47539028172277));
#103088=CARTESIAN_POINT('Ctrl Pts',(-9.33720861065951,22.7992949483867,
4.47355703087602));
#103089=CARTESIAN_POINT('Ctrl Pts',(-9.3322094522975,22.7997077771441,4.47013331976912));
#103090=CARTESIAN_POINT('Ctrl Pts',(-9.3299091990891,22.7998976344894,4.46854591658023));
#103091=CARTESIAN_POINT('Ctrl Pts',(-9.3246590072643,22.8003307751176,4.46489510568789));
#103092=CARTESIAN_POINT('Ctrl Pts',(-9.32171286228271,22.8005736944037,
4.46282635045081));
#103093=CARTESIAN_POINT('Ctrl Pts',(-9.31259984992687,22.8013248211682,
4.45636469119734));
#103094=CARTESIAN_POINT('Ctrl Pts',(-9.30646567458109,22.8018300342972,
4.45192569865471));
#103095=CARTESIAN_POINT('Ctrl Pts',(-9.29220492865885,22.8030047461393,
4.44139488898275));
#103096=CARTESIAN_POINT('Ctrl Pts',(-9.284113383506,22.8036714259412,4.43525641821857));
#103097=CARTESIAN_POINT('Ctrl Pts',(-9.25571858082127,22.8060154802308,
4.41313086780707));
#103098=CARTESIAN_POINT('Ctrl Pts',(-9.23586203184508,22.8076631339968,
4.39658025857982));
#103099=CARTESIAN_POINT('Ctrl Pts',(-9.15638711174995,22.8143683300938,
4.32577715628847));
#103100=CARTESIAN_POINT('Ctrl Pts',(-9.10187025245824,22.8192506808579,
4.26612956147161));
#103101=CARTESIAN_POINT('Ctrl Pts',(-9.02559758672961,22.8272924998202,
4.16324122388732));
#103102=CARTESIAN_POINT('Ctrl Pts',(-8.99965975655842,22.8303243938388,
4.1234320808522));
#103103=CARTESIAN_POINT('Ctrl Pts',(-8.97114041427299,22.8341193452375,
4.07327798138237));
#103104=CARTESIAN_POINT('Ctrl Pts',(-8.96620043261456,22.8347960576015,
4.0643209500944));
#103105=CARTESIAN_POINT('Ctrl Pts',(-8.9586266981879,22.8358652675289,4.05015521102481));
#103106=CARTESIAN_POINT('Ctrl Pts',(-8.95591384902843,22.8362549792115,
4.04498919000041));
#103107=CARTESIAN_POINT('Ctrl Pts',(-8.95118988026336,22.8369457530302,
4.03582869820003));
#103108=CARTESIAN_POINT('Ctrl Pts',(-8.94916289856311,22.8372462540806,
4.03184250147239));
#103109=CARTESIAN_POINT('Ctrl Pts',(-8.94456195012644,22.8379379187112,
4.02266543348808));
#103110=CARTESIAN_POINT('Ctrl Pts',(-8.94200350538437,22.8383296111018,
4.01746695332625));
#103111=CARTESIAN_POINT('Ctrl Pts',(-8.93499392710419,22.8394228693472,
4.00295494817141));
#103112=CARTESIAN_POINT('Ctrl Pts',(-8.93062681457883,22.8401272914525,
3.99360165485661));
#103113=CARTESIAN_POINT('Ctrl Pts',(-8.90364757695215,22.8446325630852,
3.93377965412974));
#103114=CARTESIAN_POINT('Ctrl Pts',(-8.88449423721458,22.8485490531958,
3.88183591636507));
#103115=CARTESIAN_POINT('Ctrl Pts',(-8.8557918886302,22.8559891120865,3.78309526674766));
#103116=CARTESIAN_POINT('Ctrl Pts',(-8.84529877326061,22.8594830575908,
3.7366850180096));
#103117=CARTESIAN_POINT('Ctrl Pts',(-8.8325443485864,22.8652935166092,3.65856298320422));
#103118=CARTESIAN_POINT('Ctrl Pts',(-8.82870802096962,22.8676096905187,
3.62716196305031));
#103119=CARTESIAN_POINT('Ctrl Pts',(-8.82355938170878,22.8721946861261,
3.56397130282093));
#103120=CARTESIAN_POINT('Ctrl Pts',(-8.82226142586907,22.8744614045507,
3.53220422301078));
#103121=CARTESIAN_POINT('Ctrl Pts',(-8.82224806909126,22.8770576580766,
3.49480350695868));
#103122=CARTESIAN_POINT('Ctrl Pts',(-8.82228624790393,22.8774456561934,
3.48918632619435));
#103123=CARTESIAN_POINT('Ctrl Pts',(-8.82241384376095,22.87807397988,3.48004105586985));
#103124=CARTESIAN_POINT('Ctrl Pts',(-8.8224789314498,22.8783155708503,3.47651279583978));
#103125=CARTESIAN_POINT('Ctrl Pts',(-8.82262386715468,22.8787465846121,
3.47019586076069));
#103126=CARTESIAN_POINT('Ctrl Pts',(-8.82269776581589,22.8789363264076,
3.46740713543066));
#103127=CARTESIAN_POINT('Ctrl Pts',(-8.82288123665371,22.8793504891829,
3.46130264916024));
#103128=CARTESIAN_POINT('Ctrl Pts',(-8.8229949094535,22.8795746822134,3.45798707941662));
#103129=CARTESIAN_POINT('Ctrl Pts',(-8.82336030858917,22.8802141367617,
3.44850001127749));
#103130=CARTESIAN_POINT('Ctrl Pts',(-8.82364657995732,22.8806275468544,
3.44232983863344));
#103131=CARTESIAN_POINT('Ctrl Pts',(-8.82601751710285,22.8835382509326,
3.39865259496866));
#103132=CARTESIAN_POINT('Ctrl Pts',(-8.82984729060606,22.8859483410634,
3.36125762952449));
#103133=CARTESIAN_POINT('Ctrl Pts',(-8.84745744154454,22.8933813108197,
3.24466624471591));
#103134=CARTESIAN_POINT('Ctrl Pts',(-8.86755307733356,22.8982484577425,
3.16666139223133));
#103135=CARTESIAN_POINT('Ctrl Pts',(-8.91220979989904,22.9063233148052,
3.04596854063539));
#103136=CARTESIAN_POINT('Ctrl Pts',(-8.9317589192599,22.9094085207859,3.00171070797751));
#103137=CARTESIAN_POINT('Ctrl Pts',(-8.95827015169717,22.9132028776575,
2.95047152081461));
#103138=CARTESIAN_POINT('Ctrl Pts',(-8.96266906716406,22.913821594004,2.94221226816856));
#103139=CARTESIAN_POINT('Ctrl Pts',(-8.97010706456577,22.9148506639582,
2.92863928918754));
#103140=CARTESIAN_POINT('Ctrl Pts',(-8.97309004253927,22.9152590407653,
2.92329517325145));
#103141=CARTESIAN_POINT('Ctrl Pts',(-8.97841651523805,22.9159808540324,
2.91392496616363));
#103142=CARTESIAN_POINT('Ctrl Pts',(-8.98074251626196,22.9162936614842,
2.90988904229916));
#103143=CARTESIAN_POINT('Ctrl Pts',(-8.985823708183,22.9169719190666,2.90119216220076));
#103144=CARTESIAN_POINT('Ctrl Pts',(-8.98858721028807,22.917337663036,2.89653621102473));
#103145=CARTESIAN_POINT('Ctrl Pts',(-8.99604882947459,22.9183170101244,
2.88416010059939));
#103146=CARTESIAN_POINT('Ctrl Pts',(-9.0008037896631,22.918932662821,2.87647481220961));
#103147=CARTESIAN_POINT('Ctrl Pts',(-9.01149180577035,22.9202985213205,
2.85963636804076));
#103148=CARTESIAN_POINT('Ctrl Pts',(-9.01746446930144,22.9210501367655,
2.85050947023202));
#103149=CARTESIAN_POINT('Ctrl Pts',(-9.03585962436427,22.9233311021802,
2.82323412441864));
#103150=CARTESIAN_POINT('Ctrl Pts',(-9.0486639307353,22.924874119586,2.80535023943774));
#103151=CARTESIAN_POINT('Ctrl Pts',(-9.10104472787236,22.9310177963152,
2.73635593017204));
#103152=CARTESIAN_POINT('Ctrl Pts',(-9.14429621338611,22.9357427072336,
2.68818591587217));
#103153=CARTESIAN_POINT('Ctrl Pts',(-9.23873658953856,22.9452821294783,
2.59898082414551));
#103154=CARTESIAN_POINT('Ctrl Pts',(-9.28984902514721,22.9500796862204,
2.55816943488881));
#103155=CARTESIAN_POINT('Ctrl Pts',(-9.35215524594312,22.9553360154291,
2.51639101222574));
#103156=CARTESIAN_POINT('Ctrl Pts',(-9.36029212843856,22.9560115706129,
2.51107971980795));
#103157=CARTESIAN_POINT('Ctrl Pts',(-9.37161318720491,22.9569355835336,
2.50388819393825));
#103158=CARTESIAN_POINT('Ctrl Pts',(-9.37474160194837,22.9571892680886,
2.50192151948692));
#103159=CARTESIAN_POINT('Ctrl Pts',(-9.38012349529984,22.9576227916385,
2.49857343397411));
#103160=CARTESIAN_POINT('Ctrl Pts',(-9.38237243874137,22.9578030876769,
2.49718484048716));
#103161=CARTESIAN_POINT('Ctrl Pts',(-9.38708014967686,22.958178674492,2.49429994345847));
#103162=CARTESIAN_POINT('Ctrl Pts',(-9.38953975204667,22.9583738660677,
2.49280506724892));
#103163=CARTESIAN_POINT('Ctrl Pts',(-9.39556010488616,22.9588491648408,
2.48917622304701));
#103164=CARTESIAN_POINT('Ctrl Pts',(-9.39912675074334,22.9591286481999,
2.48705200800242));
#103165=CARTESIAN_POINT('Ctrl Pts',(-9.41201685023571,22.9601314629707,
2.47946699101358));
#103166=CARTESIAN_POINT('Ctrl Pts',(-9.42140445621274,22.9608481911866,
2.47411549184541));
#103167=CARTESIAN_POINT('Ctrl Pts',(-9.4450475607895,22.9626229951323,2.4610653111875));
#103168=CARTESIAN_POINT('Ctrl Pts',(-9.45939109288218,22.9636726724585,
2.45352995178986));
#103169=CARTESIAN_POINT('Ctrl Pts',(-9.52312743210442,22.9682394075834,
2.42170654196351));
#103170=CARTESIAN_POINT('Ctrl Pts',(-9.57403546410357,22.971635936793,2.40060043569637));
#103171=CARTESIAN_POINT('Ctrl Pts',(-9.68653025503974,22.9789689096178,
2.3629537187566));
#103172=CARTESIAN_POINT('Ctrl Pts',(-9.74835386439087,22.9828982796882,
2.34769325374467));
#103173=CARTESIAN_POINT('Ctrl Pts',(-9.8111040637108,22.9869701371802,2.33749693000258));
#103174=CARTESIAN_POINT('Origin',(-10.,12.3756328852638,3.5));
#103175=CARTESIAN_POINT('',(-9.81110406371025,23.5855117083725,2.33749693000267));
#103176=CARTESIAN_POINT('',(-9.81110406371068,23.4873487054734,2.3374969300026));
#103177=CARTESIAN_POINT('',(-9.81110406371068,12.3756328852638,2.3374969300026));
#103178=CARTESIAN_POINT('Ctrl Pts',(-9.81110406370983,23.5855117083725,
2.33749693000274));
#103179=CARTESIAN_POINT('Ctrl Pts',(-9.81101707518383,23.5855055469538,
2.33751106482912));
#103180=CARTESIAN_POINT('Ctrl Pts',(-9.81093008809885,23.5854993859672,
2.337525209443));
#103181=CARTESIAN_POINT('Ctrl Pts',(-9.80226865091188,23.5848859600242,
2.33893460820937));
#103182=CARTESIAN_POINT('Ctrl Pts',(-9.7937095796167,23.5842829952613,2.34042473120738));
#103183=CARTESIAN_POINT('Ctrl Pts',(-9.78169619421968,23.5834419290962,
2.34265347653336));
#103184=CARTESIAN_POINT('Ctrl Pts',(-9.7782277735032,23.5831997197652,2.34331309017284));
#103185=CARTESIAN_POINT('Ctrl Pts',(-9.77195496188742,23.5827628541751,
2.34453528677058));
#103186=CARTESIAN_POINT('Ctrl Pts',(-9.76914955961378,23.5825679030302,
2.34509250685753));
#103187=CARTESIAN_POINT('Ctrl Pts',(-9.76341917038147,23.5821706056214,
2.34625241415772));
#103188=CARTESIAN_POINT('Ctrl Pts',(-9.76049440301973,23.58196831198,2.34685601493027));
#103189=CARTESIAN_POINT('Ctrl Pts',(-9.75301012025541,23.5814518260193,
2.34843029191857));
#103190=CARTESIAN_POINT('Ctrl Pts',(-9.74845396022,23.5811385219708,2.34941693695617));
#103191=CARTESIAN_POINT('Ctrl Pts',(-9.72960140501996,23.5798462921623,
2.35361683134307));
#103192=CARTESIAN_POINT('Ctrl Pts',(-9.71535901643465,23.5788800036326,
2.35706984956996));
#103193=CARTESIAN_POINT('Ctrl Pts',(-9.67728282427724,23.5763143591768,
2.36705725797825));
#103194=CARTESIAN_POINT('Ctrl Pts',(-9.65358324299116,23.5747361805619,
2.37407761130642));
#103195=CARTESIAN_POINT('Ctrl Pts',(-9.5790534432492,23.5697826789619,2.39873151520884));
#103196=CARTESIAN_POINT('Ctrl Pts',(-9.52920128349297,23.5664813304822,
2.41910344002792));
#103197=CARTESIAN_POINT('Ctrl Pts',(-9.41368706332256,23.5585149651967,
2.47582163609594));
#103198=CARTESIAN_POINT('Ctrl Pts',(-9.34977113351562,23.5538328158559,
2.51516277653947));
#103199=CARTESIAN_POINT('Ctrl Pts',(-9.28214195159639,23.5482645163903,
2.56625884324312));
#103200=CARTESIAN_POINT('Ctrl Pts',(-9.2743324726514,23.5476116694787,2.57231505589825));
#103201=CARTESIAN_POINT('Ctrl Pts',(-9.26168569481117,23.546537624221,2.5823799800188));
#103202=CARTESIAN_POINT('Ctrl Pts',(-9.25680251856624,23.5461187197544,
2.58633046711241));
#103203=CARTESIAN_POINT('Ctrl Pts',(-9.24809792827701,23.54536428793,2.5934884305085));
#103204=CARTESIAN_POINT('Ctrl Pts',(-9.24426482642995,23.5450293434679,
2.59668150843771));
#103205=CARTESIAN_POINT('Ctrl Pts',(-9.23615191040966,23.5443145164667,
2.60352756942573));
#103206=CARTESIAN_POINT('Ctrl Pts',(-9.23187776968723,23.5439343746302,
2.60718705198356));
#103207=CARTESIAN_POINT('Ctrl Pts',(-9.22042365434018,23.5429059099274,
2.61713709695367));
#103208=CARTESIAN_POINT('Ctrl Pts',(-9.2132937954423,23.5422552599191,2.6234844424371));
#103209=CARTESIAN_POINT('Ctrl Pts',(-9.1763319139982,23.5388259976685,2.65720399215282));
#103210=CARTESIAN_POINT('Ctrl Pts',(-9.14785211353399,23.5359871673753,
2.68601134459554));
#103211=CARTESIAN_POINT('Ctrl Pts',(-9.05490272319349,23.5260066887844,
2.79026376700387));
#103212=CARTESIAN_POINT('Ctrl Pts',(-8.99851808058813,23.518596891733,2.87233390778798));
#103213=CARTESIAN_POINT('Ctrl Pts',(-8.94007636325438,23.5094011561515,
2.98573965111557));
#103214=CARTESIAN_POINT('Ctrl Pts',(-8.92798151386329,23.5073816021219,
3.01145267386354));
#103215=CARTESIAN_POINT('Ctrl Pts',(-8.91468974465211,23.5050329677426,
3.04258732744809));
#103216=CARTESIAN_POINT('Ctrl Pts',(-8.9125868264393,23.5046570733917,3.04760935444201));
#103217=CARTESIAN_POINT('Ctrl Pts',(-8.90919805317204,23.5040443589991,
3.05586233553087));
#103218=CARTESIAN_POINT('Ctrl Pts',(-8.90789157570977,23.5038063733817,
3.05908465371917));
#103219=CARTESIAN_POINT('Ctrl Pts',(-8.90556316458353,23.5033790790681,
3.06490133280638));
#103220=CARTESIAN_POINT('Ctrl Pts',(-8.90453616203801,23.5031894768288,
3.06749356408747));
#103221=CARTESIAN_POINT('Ctrl Pts',(-8.90229064064518,23.5027723904805,
3.07322074002767));
#103222=CARTESIAN_POINT('Ctrl Pts',(-8.90107634080789,23.5025451566556,
3.07635726568556));
#103223=CARTESIAN_POINT('Ctrl Pts',(-8.89759375199082,23.5018883845145,
3.08546849577285));
#103224=CARTESIAN_POINT('Ctrl Pts',(-8.89536059101781,23.5014608566283,
3.09145663105133));
#103225=CARTESIAN_POINT('Ctrl Pts',(-8.87794080178847,23.4980716490016,
3.13935440930605));
#103226=CARTESIAN_POINT('Ctrl Pts',(-8.86509398194838,23.4952331498113,
3.18208268762178));
#103227=CARTESIAN_POINT('Ctrl Pts',(-8.82882610413601,23.4854898947136,
3.3333714158876));
#103228=CARTESIAN_POINT('Ctrl Pts',(-8.81833889267637,23.47881866449,3.44440884737529));
#103229=CARTESIAN_POINT('Ctrl Pts',(-8.82433587244591,23.4705125533034,
3.57204786151172));
#103230=CARTESIAN_POINT('Ctrl Pts',(-8.82548256202627,23.4694110868983,
3.58880189767733));
#103231=CARTESIAN_POINT('Ctrl Pts',(-8.82757002399933,23.4678674561839,
3.61200606003856));
#103232=CARTESIAN_POINT('Ctrl Pts',(-8.8282067537677,23.4674346908718,3.6184820296495));
#103233=CARTESIAN_POINT('Ctrl Pts',(-8.82939796104694,23.4666850778343,
3.62964650186105));
#103234=CARTESIAN_POINT('Ctrl Pts',(-8.82992702998382,23.4663690260153,
3.63433760745525));
#103235=CARTESIAN_POINT('Ctrl Pts',(-8.83108184921524,23.4657122299756,
3.64405223334209));
#103236=CARTESIAN_POINT('Ctrl Pts',(-8.83171181254191,23.4653713605783,
3.64907514491255));
#103237=CARTESIAN_POINT('Ctrl Pts',(-8.83326715052518,23.4645684979268,
3.6608605197483));
#103238=CARTESIAN_POINT('Ctrl Pts',(-8.83421896024185,23.4641056872272,
3.66761924945302));
#103239=CARTESIAN_POINT('Ctrl Pts',(-8.83754237941596,23.4625774508508,
3.68981938995061));
#103240=CARTESIAN_POINT('Ctrl Pts',(-8.84016239109484,23.4615043128495,
3.70522134540036));
#103241=CARTESIAN_POINT('Ctrl Pts',(-8.84711403406541,23.4589318240004,
3.74168408097576));
#103242=CARTESIAN_POINT('Ctrl Pts',(-8.85171744156,23.4574244609459,3.7626867154389));
#103243=CARTESIAN_POINT('Ctrl Pts',(-8.8718286822172,23.451505029933,3.84376329162419));
#103244=CARTESIAN_POINT('Ctrl Pts',(-8.89149714874639,23.446978559522,3.90269533367618));
#103245=CARTESIAN_POINT('Ctrl Pts',(-8.94259832125502,23.4373688546333,
4.02320134496668));
#103246=CARTESIAN_POINT('Ctrl Pts',(-8.97499687617051,23.4322970140959,
4.08413042525668));
#103247=CARTESIAN_POINT('Ctrl Pts',(-9.01779411951237,23.426795631612,4.14996898455672));
#103248=CARTESIAN_POINT('Ctrl Pts',(-9.02314960528399,23.4261251540622,
4.15799042082109));
#103249=CARTESIAN_POINT('Ctrl Pts',(-9.03068775447707,23.425206734713,4.16898611634926));
#103250=CARTESIAN_POINT('Ctrl Pts',(-9.03278657611005,23.4249536501735,
4.17201699885985));
#103251=CARTESIAN_POINT('Ctrl Pts',(-9.03641354496114,23.424520844159,4.17720246817957));
#103252=CARTESIAN_POINT('Ctrl Pts',(-9.03793475616552,23.4243406692806,
4.17936183746314));
#103253=CARTESIAN_POINT('Ctrl Pts',(-9.04113067826038,23.4239649815283,
4.18386620745407));
#103254=CARTESIAN_POINT('Ctrl Pts',(-9.0428067477167,23.4237695697075,4.18621020387677));
#103255=CARTESIAN_POINT('Ctrl Pts',(-9.04692622004022,23.423293148642,4.19192685818933));
#103256=CARTESIAN_POINT('Ctrl Pts',(-9.04937897316487,23.4230127696446,
4.19529279572514));
#103257=CARTESIAN_POINT('Ctrl Pts',(-9.05830894144836,23.422003469309,4.20741188989303));
#103258=CARTESIAN_POINT('Ctrl Pts',(-9.06488985544988,23.4212812623764,
4.21608845142274));
#103259=CARTESIAN_POINT('Ctrl Pts',(-9.08166197307433,23.4194902052022,
4.23757593195497));
#103260=CARTESIAN_POINT('Ctrl Pts',(-9.09200193049313,23.4184299503672,
4.25026831816613));
#103261=CARTESIAN_POINT('Ctrl Pts',(-9.13892737746803,23.4137868753006,
4.30547799986115));
#103262=CARTESIAN_POINT('Ctrl Pts',(-9.17826047041481,23.4103286950745,
4.34556845318698));
#103263=CARTESIAN_POINT('Ctrl Pts',(-9.27976876738372,23.4019565318056,
4.43523101264957));
#103264=CARTESIAN_POINT('Ctrl Pts',(-9.34438121545476,23.3970435419503,
4.48160685996782));
#103265=CARTESIAN_POINT('Ctrl Pts',(-9.42623512297582,23.3908865465204,
4.52864781979968));
#103266=CARTESIAN_POINT('Ctrl Pts',(-9.43945246130103,23.3898949133534,
4.53590969411713));
#103267=CARTESIAN_POINT('Ctrl Pts',(-9.45870049499698,23.3884526234533,
4.54600871493575));
#103268=CARTESIAN_POINT('Ctrl Pts',(-9.46462189843755,23.3880091668679,
4.54905179621608));
#103269=CARTESIAN_POINT('Ctrl Pts',(-9.47508336334705,23.3872259723091,
4.554316428426));
#103270=CARTESIAN_POINT('Ctrl Pts',(-9.47961256013503,23.3868869833996,
4.55655928264882));
#103271=CARTESIAN_POINT('Ctrl Pts',(-9.48899647778078,23.3861847511278,
4.56113121468938));
#103272=CARTESIAN_POINT('Ctrl Pts',(-9.49385300727551,23.3858213794986,
4.56345628711216));
#103273=CARTESIAN_POINT('Ctrl Pts',(-9.50636043651531,23.3848856167639,
4.56933915897361));
#103274=CARTESIAN_POINT('Ctrl Pts',(-9.51403382576969,23.3843115746743,
4.57284813771647));
#103275=CARTESIAN_POINT('Ctrl Pts',(-9.5468346251224,23.3818575075611,4.58742358237182));
#103276=CARTESIAN_POINT('Ctrl Pts',(-9.57230538530207,23.3799509352076,
4.59769121514611));
#103277=CARTESIAN_POINT('Ctrl Pts',(-9.69173773467153,23.370999836015,4.64104815204983));
#103278=CARTESIAN_POINT('Ctrl Pts',(-9.7892904225141,23.3636104223965,4.66301849242003));
#103279=CARTESIAN_POINT('Ctrl Pts',(-9.91040892687715,23.3547422802659,
4.67454520474798));
#103280=CARTESIAN_POINT('Ctrl Pts',(-9.93245445787871,23.3531425821469,
4.67601900143798));
#103281=CARTESIAN_POINT('Ctrl Pts',(-9.97640594384946,23.3499963265144,
4.67771714839619));
#103282=CARTESIAN_POINT('Ctrl Pts',(-9.99830359624389,23.3484499969593,
4.67795230529546));
#103283=CARTESIAN_POINT('Ctrl Pts',(-10.0257162109439,23.3465506379679,
4.67748214975646));
#103284=CARTESIAN_POINT('Ctrl Pts',(-10.0312351284897,23.3461700970871,
4.67734867658333));
#103285=CARTESIAN_POINT('Ctrl Pts',(-10.0399596876264,23.3455716608668,
4.67707628405724));
#103286=CARTESIAN_POINT('Ctrl Pts',(-10.0431659636651,23.3453524064341,
4.67696306455678));
#103287=CARTESIAN_POINT('Ctrl Pts',(-10.0488932192871,23.3449620061932,
4.67673738918582));
#103288=CARTESIAN_POINT('Ctrl Pts',(-10.0514142872176,23.3447905927912,
4.67662993385771));
#103289=CARTESIAN_POINT('Ctrl Pts',(-10.0574637255756,23.3443803030669,
4.67635260885028));
#103290=CARTESIAN_POINT('Ctrl Pts',(-10.0609916974175,23.3441418591729,
4.6761749673291));
#103291=CARTESIAN_POINT('Ctrl Pts',(-10.0717294179682,23.3434185229589,
4.67558585459938));
#103292=CARTESIAN_POINT('Ctrl Pts',(-10.0789363941969,23.3429363144214,
4.67512393519489));
#103293=CARTESIAN_POINT('Ctrl Pts',(-10.1438050908159,23.3386219393218,
4.67036679437135));
#103294=CARTESIAN_POINT('Ctrl Pts',(-10.2010901683696,23.3349944654803,
4.66189628246485));
#103295=CARTESIAN_POINT('Ctrl Pts',(-10.3567973717927,23.3250901826691,
4.62700485358089));
#103296=CARTESIAN_POINT('Ctrl Pts',(-10.4527548543426,23.3188969946901,
4.59199602132031));
#103297=CARTESIAN_POINT('Ctrl Pts',(-10.5549845392699,23.311363458729,4.53887874889231));
#103298=CARTESIAN_POINT('Ctrl Pts',(-10.5668421380572,23.3104750643262,
4.53245671089563));
#103299=CARTESIAN_POINT('Ctrl Pts',(-10.5841934336795,23.3091520097465,
4.52267029554523));
#103300=CARTESIAN_POINT('Ctrl Pts',(-10.5897742731672,23.3087228757776,
4.5194620175764));
#103301=CARTESIAN_POINT('Ctrl Pts',(-10.5996477774832,23.3079571078968,
4.51367779157077));
#103302=CARTESIAN_POINT('Ctrl Pts',(-10.6039508804681,23.3076211285435,
4.51111990130719));
#103303=CARTESIAN_POINT('Ctrl Pts',(-10.6129782463306,23.3069114815719,
4.50567558451094));
#103304=CARTESIAN_POINT('Ctrl Pts',(-10.6176987134544,23.306537601241,4.50278313175881));
#103305=CARTESIAN_POINT('Ctrl Pts',(-10.6301512448122,23.3055437517526,
4.49503159015562));
#103306=CARTESIAN_POINT('Ctrl Pts',(-10.6378473581646,23.3049217184631,
4.49011574891226));
#103307=CARTESIAN_POINT('Ctrl Pts',(-10.6746750834727,23.3019065936442,
4.46598470553752));
#103308=CARTESIAN_POINT('Ctrl Pts',(-10.7029973879467,23.2994694078982,
4.44557239465249));
#103309=CARTESIAN_POINT('Ctrl Pts',(-10.7833690607167,23.2921902110997,
4.38203867004065));
#103310=CARTESIAN_POINT('Ctrl Pts',(-10.8326601002508,23.2872383952941,
4.33566414290791));
#103311=CARTESIAN_POINT('Ctrl Pts',(-10.9179362468099,23.2778484491652,
4.24035760511454));
#103312=CARTESIAN_POINT('Ctrl Pts',(-10.9546618017348,23.2734280958764,
4.19235733427934));
#103313=CARTESIAN_POINT('Ctrl Pts',(-10.9928773672048,23.268513240034,4.13354969517362));
#103314=CARTESIAN_POINT('Ctrl Pts',(-10.9981035402641,23.267833281333,4.12528395236271));
#103315=CARTESIAN_POINT('Ctrl Pts',(-11.0051666385238,23.2669043259113,
4.11379867257014));
#103316=CARTESIAN_POINT('Ctrl Pts',(-11.0070920513212,23.2666500297705,
4.1106344100599));
#103317=CARTESIAN_POINT('Ctrl Pts',(-11.0103672681286,23.266215695865,4.1051942225876));
#103318=CARTESIAN_POINT('Ctrl Pts',(-11.0117243739554,23.2660351977404,
4.10292276044115));
#103319=CARTESIAN_POINT('Ctrl Pts',(-11.0145413547174,23.2656594528853,
4.09817153244428));
#103320=CARTESIAN_POINT('Ctrl Pts',(-11.015999811051,23.2654643041044,4.09569096588834));
#103321=CARTESIAN_POINT('Ctrl Pts',(-11.0195363656332,23.2649895337436,
4.08962516368918));
#103322=CARTESIAN_POINT('Ctrl Pts',(-11.0216046879249,23.2647105321189,
4.08603421181082));
#103323=CARTESIAN_POINT('Ctrl Pts',(-11.0289707722116,23.2637117749175,
4.07308794941716));
#103324=CARTESIAN_POINT('Ctrl Pts',(-11.0341595256549,23.2629985510409,
4.06367077586474));
#103325=CARTESIAN_POINT('Ctrl Pts',(-11.0467899046986,23.261234276896,4.03998597022747));
#103326=CARTESIAN_POINT('Ctrl Pts',(-11.0540696520248,23.2601914961133,
4.02563406964567));
#103327=CARTESIAN_POINT('Ctrl Pts',(-11.0846417881746,23.2556746723774,
3.96217029645215));
#103328=CARTESIAN_POINT('Ctrl Pts',(-11.1048142069596,23.2523184816334,
3.91162567659839));
#103329=CARTESIAN_POINT('Ctrl Pts',(-11.1463631698139,23.2439127004305,
3.78214928450594));
#103330=CARTESIAN_POINT('Ctrl Pts',(-11.1631533058807,23.2388675161486,
3.70206188922571));
#103331=CARTESIAN_POINT('Ctrl Pts',(-11.1730722110978,23.2325647266658,
3.60593649631977));
#103332=CARTESIAN_POINT('Ctrl Pts',(-11.1743285096681,23.2315763504572,
3.59095862594046));
#103333=CARTESIAN_POINT('Ctrl Pts',(-11.1757266318038,23.2301379501857,
3.56932644287678));
#103334=CARTESIAN_POINT('Ctrl Pts',(-11.1760992571527,23.2296950713407,
3.56268813835158));
#103335=CARTESIAN_POINT('Ctrl Pts',(-11.1766560970862,23.2289125508986,
3.55100020698347));
#103336=CARTESIAN_POINT('Ctrl Pts',(-11.1768640613717,23.2285736543167,
3.54595184013623));
#103337=CARTESIAN_POINT('Ctrl Pts',(-11.177226649725,23.2278712749456,3.53551770266875));
#103338=CARTESIAN_POINT('Ctrl Pts',(-11.1773768125007,23.2275076618275,
3.53013190571305));
#103339=CARTESIAN_POINT('Ctrl Pts',(-11.1776676296243,23.2265705590003,
3.51629357507749));
#103340=CARTESIAN_POINT('Ctrl Pts',(-11.1777542396828,23.2259954091592,
3.50784033621611));
#103341=CARTESIAN_POINT('Ctrl Pts',(-11.1777354735185,23.2235298395984,
3.47178007639624));
#103342=CARTESIAN_POINT('Ctrl Pts',(-11.17675043923,23.2216125609006,3.44418429720845));
#103343=CARTESIAN_POINT('Ctrl Pts',(-11.1677558339711,23.2126571793346,
3.31740688234046));
#103344=CARTESIAN_POINT('Ctrl Pts',(-11.1481673106871,23.2052758565925,
3.21946509557233));
#103345=CARTESIAN_POINT('Ctrl Pts',(-11.1094781170695,23.1964153424189,
3.10421987858845));
#103346=CARTESIAN_POINT('Ctrl Pts',(-11.101854943103,23.1948147655459,3.08346743809587));
#103347=CARTESIAN_POINT('Ctrl Pts',(-11.0855546728982,23.1916730829631,
3.04267931151401));
#103348=CARTESIAN_POINT('Ctrl Pts',(-11.0768953121776,23.1901320484666,
3.02264500061779));
#103349=CARTESIAN_POINT('Ctrl Pts',(-11.0653560135108,23.1882382272865,
2.99786253542938));
#103350=CARTESIAN_POINT('Ctrl Pts',(-11.0629932875171,23.187858115015,2.99287995253891));
#103351=CARTESIAN_POINT('Ctrl Pts',(-11.0592012769998,23.1872602017794,
2.9850262133917));
#103352=CARTESIAN_POINT('Ctrl Pts',(-11.057795147973,23.1870410455657,2.98214406285108));
#103353=CARTESIAN_POINT('Ctrl Pts',(-11.0552614423572,23.1866507281333,
2.9770040923002));
#103354=CARTESIAN_POINT('Ctrl Pts',(-11.0541383869982,23.1864793000443,
2.97474416478042));
#103355=CARTESIAN_POINT('Ctrl Pts',(-11.0514249711527,23.1860688568256,
2.969327704857));
#103356=CARTESIAN_POINT('Ctrl Pts',(-11.0498276564678,23.1858302750649,
2.96617470336081));
#103357=CARTESIAN_POINT('Ctrl Pts',(-11.0449189014065,23.1851060996829,
2.9565923697817));
#103358=CARTESIAN_POINT('Ctrl Pts',(-11.0415623399643,23.1846231989432,
2.95018615736621));
#103359=CARTESIAN_POINT('Ctrl Pts',(-11.010667187408,23.1802838372059,2.89251923053103));
#103360=CARTESIAN_POINT('Ctrl Pts',(-10.9794198699957,23.1766346683611,
2.84332680414146));
#103361=CARTESIAN_POINT('Ctrl Pts',(-10.8841916339141,23.1667390022392,
2.71542884769285));
#103362=CARTESIAN_POINT('Ctrl Pts',(-10.8135123263704,23.1605728638889,
2.64236232592251));
#103363=CARTESIAN_POINT('Ctrl Pts',(-10.72377249514,23.1530675523117,2.57078962122851));
#103364=CARTESIAN_POINT('Ctrl Pts',(-10.7130378007323,23.152175181706,2.5625270015829));
#103365=CARTESIAN_POINT('Ctrl Pts',(-10.696985833039,23.150847328269,2.55060682531489));
#103366=CARTESIAN_POINT('Ctrl Pts',(-10.6917769267933,23.1504174308258,
2.54680467250241));
#103367=CARTESIAN_POINT('Ctrl Pts',(-10.6824684976073,23.1496508062632,
2.54012663008854));
#103368=CARTESIAN_POINT('Ctrl Pts',(-10.6783813325898,23.1493147390655,
2.53723372371194));
#103369=CARTESIAN_POINT('Ctrl Pts',(-10.6697418558365,23.1486054270809,
2.53120100633172));
#103370=CARTESIAN_POINT('Ctrl Pts',(-10.6651856405615,23.148231972833,2.52806702629443));
#103371=CARTESIAN_POINT('Ctrl Pts',(-10.6530706276395,23.1472404753333,
2.51985883693834));
#103372=CARTESIAN_POINT('Ctrl Pts',(-10.645474900742,23.1466203853548,2.51484006952346));
#103373=CARTESIAN_POINT('Ctrl Pts',(-10.6087730332824,23.1436308618374,
2.49119650600975));
#103374=CARTESIAN_POINT('Ctrl Pts',(-10.5789175299784,23.141218240841,2.47377236303456));
#103375=CARTESIAN_POINT('Ctrl Pts',(-10.4896128637742,23.1340512337476,
2.42679080178953));
#103376=CARTESIAN_POINT('Ctrl Pts',(-10.4283836229475,23.1291913554873,
2.40091657292208));
#103377=CARTESIAN_POINT('Ctrl Pts',(-10.3063869741341,23.1197684535021,
2.36111303167791));
#103378=CARTESIAN_POINT('Ctrl Pts',(-10.2460326994818,23.1152235226079,
2.34656773979351));
#103379=CARTESIAN_POINT('Ctrl Pts',(-10.1751812292,23.110196423447,2.33531050179874));
#103380=CARTESIAN_POINT('Ctrl Pts',(-10.1655347545678,23.1095186048482,
2.33390036841459));
#103381=CARTESIAN_POINT('Ctrl Pts',(-10.1522039590012,23.1085920222282,
2.3321204222968));
#103382=CARTESIAN_POINT('Ctrl Pts',(-10.1485340689348,23.1083379943824,
2.33164800490259));
#103383=CARTESIAN_POINT('Ctrl Pts',(-10.1422371049742,23.1079039990078,
2.33086755920325));
#103384=CARTESIAN_POINT('Ctrl Pts',(-10.1396111366587,23.1077235726613,
2.33055107463824));
#103385=CARTESIAN_POINT('Ctrl Pts',(-10.1341252215403,23.1073478415379,
2.32990864772608));
#103386=CARTESIAN_POINT('Ctrl Pts',(-10.131265117865,23.1071526353949,2.32958434016285));
#103387=CARTESIAN_POINT('Ctrl Pts',(-10.1242800923387,23.1066775035493,
2.32881823318869));
#103388=CARTESIAN_POINT('Ctrl Pts',(-10.120153917095,23.1063982000543,2.32838773061533));
#103389=CARTESIAN_POINT('Ctrl Pts',(-10.1052967516266,23.1053971397262,
2.32691692955242));
#103390=CARTESIAN_POINT('Ctrl Pts',(-10.094553477483,23.1046819542787,2.32600214805739));
#103391=CARTESIAN_POINT('Ctrl Pts',(-10.0676889442456,23.1029118413972,
2.32408583909969));
#103392=CARTESIAN_POINT('Ctrl Pts',(-10.051556412582,23.1018652539019,2.32326812836946));
#103393=CARTESIAN_POINT('Ctrl Pts',(-9.98071044339814,23.0973211958324,
2.32113704265959));
#103394=CARTESIAN_POINT('Ctrl Pts',(-9.92595690401097,23.0939430271003,
2.32330610220372));
#103395=CARTESIAN_POINT('Ctrl Pts',(-9.85132243203161,23.0893017531441,
2.33149493546198));
#103396=CARTESIAN_POINT('Ctrl Pts',(-9.83116744989325,23.088044978322,2.33423681635998));
#103397=CARTESIAN_POINT('Ctrl Pts',(-9.8111040637107,23.0867835801461,2.3374969300026));
#103398=CARTESIAN_POINT('',(-9.81115948034543,22.9869737331824,2.33748792667061));
#103399=CARTESIAN_POINT('Ctrl Pts',(-9.8111040637108,22.9869701371802,2.33749693000258));
#103400=CARTESIAN_POINT('Ctrl Pts',(-9.81112581929086,22.9869715488987,
2.33749339492317));
#103401=CARTESIAN_POINT('Ctrl Pts',(-9.81113772457216,22.986972321436,2.33749146071695));
#103402=CARTESIAN_POINT('Ctrl Pts',(-9.81115948034541,22.9869737331824,
2.33748792667061));
#103403=CARTESIAN_POINT('Ctrl Pts',(-9.81115948034545,22.9869737331824,
2.33748792667061));
#103404=CARTESIAN_POINT('Ctrl Pts',(-9.82933045015929,22.9881528593244,
2.33453620215867));
#103405=CARTESIAN_POINT('Ctrl Pts',(-9.84755744172139,22.9893419534045,
2.33201234132762));
#103406=CARTESIAN_POINT('Ctrl Pts',(-9.87752473866595,22.9913121344289,
2.32857647474011));
#103407=CARTESIAN_POINT('Ctrl Pts',(-9.88922322805877,22.992084996478,2.32741236746751));
#103408=CARTESIAN_POINT('Ctrl Pts',(-9.90664980367938,22.9932427720667,
2.32594136700875));
#103409=CARTESIAN_POINT('Ctrl Pts',(-9.9123661130932,22.9936235825559,2.32550085875634));
#103410=CARTESIAN_POINT('Ctrl Pts',(-9.92278582165,22.9943197186435,2.32477438965723));
#103411=CARTESIAN_POINT('Ctrl Pts',(-9.9274881808665,22.9946346197485,2.32447488349496));
#103412=CARTESIAN_POINT('Ctrl Pts',(-9.93667333437253,22.9952512190345,
2.32394517828075));
#103413=CARTESIAN_POINT('Ctrl Pts',(-9.94115590195987,22.995552830928,2.32371237299893));
#103414=CARTESIAN_POINT('Ctrl Pts',(-9.95142206249744,22.9962452442893,
2.32323802138882));
#103415=CARTESIAN_POINT('Ctrl Pts',(-9.95720628667639,22.9966365661914,
2.32301348081542));
#103416=CARTESIAN_POINT('Ctrl Pts',(-9.97301063543375,22.9977091739265,
2.32251661917644));
#103417=CARTESIAN_POINT('Ctrl Pts',(-9.98303276112712,22.9983930800217,
2.32232957076422));
#103418=CARTESIAN_POINT('Ctrl Pts',(-10.0273602127523,23.0014352152979,
2.32206820417229));
#103419=CARTESIAN_POINT('Ctrl Pts',(-10.0616537382153,23.0038351055056,
2.32336484021042));
#103420=CARTESIAN_POINT('Ctrl Pts',(-10.1454009295848,23.009812264309,2.33020241317789));
#103421=CARTESIAN_POINT('Ctrl Pts',(-10.1946523792398,23.0134293086955,
2.33738336818735));
#103422=CARTESIAN_POINT('Ctrl Pts',(-10.3162493957474,23.0225409881098,
2.36305652239483));
#103423=CARTESIAN_POINT('Ctrl Pts',(-10.3875780628195,23.028057242111,2.38535249724469));
#103424=CARTESIAN_POINT('Ctrl Pts',(-10.4671228361506,23.0341257659899,
2.41878376866579));
#103425=CARTESIAN_POINT('Ctrl Pts',(-10.477854160598,23.0349423355658,2.42348352988791));
#103426=CARTESIAN_POINT('Ctrl Pts',(-10.4924121273541,23.0360454522139,
2.43011976763798));
#103427=CARTESIAN_POINT('Ctrl Pts',(-10.4963005318373,23.0363396355962,
2.43191798147123));
#103428=CARTESIAN_POINT('Ctrl Pts',(-10.5028088618272,23.0368311599454,
2.43497101057247));
#103429=CARTESIAN_POINT('Ctrl Pts',(-10.5054340833018,23.0370291827564,
2.43621435998972));
#103430=CARTESIAN_POINT('Ctrl Pts',(-10.5104150897067,23.0374044106437,
2.43859605060154));
#103431=CARTESIAN_POINT('Ctrl Pts',(-10.5127717160224,23.0375817299307,
2.43973254544482));
#103432=CARTESIAN_POINT('Ctrl Pts',(-10.5183548048173,23.0380013657455,
2.44244798634289));
#103433=CARTESIAN_POINT('Ctrl Pts',(-10.5215778931791,23.0382432599517,
2.44403387011638));
#103434=CARTESIAN_POINT('Ctrl Pts',(-10.5328959441981,23.0390915942668,
2.44966725075774));
#103435=CARTESIAN_POINT('Ctrl Pts',(-10.5409517118907,23.0396934361345,
2.4537934098937));
#103436=CARTESIAN_POINT('Ctrl Pts',(-10.6206501318649,23.0456359398445,
2.4957816144695));
#103437=CARTESIAN_POINT('Ctrl Pts',(-10.6882627972059,23.0505922381058,
2.54085482699908));
#103438=CARTESIAN_POINT('Ctrl Pts',(-10.7849351010806,23.0583519991997,
2.62082765707672));
#103439=CARTESIAN_POINT('Ctrl Pts',(-10.8175223657971,23.0611071263157,
2.65104536660552));
#103440=CARTESIAN_POINT('Ctrl Pts',(-10.8657156269797,23.0655092936261,
2.70108817750477));
#103441=CARTESIAN_POINT('Ctrl Pts',(-10.8825250043757,23.0671149856522,
2.71969676622847));
#103442=CARTESIAN_POINT('Ctrl Pts',(-10.906451667302,23.0695200132337,2.74794728007398));
#103443=CARTESIAN_POINT('Ctrl Pts',(-10.9140368210976,23.0703014909455,
2.75718468510322));
#103444=CARTESIAN_POINT('Ctrl Pts',(-10.9275612562168,23.0717313780518,
2.77417596086155));
#103445=CARTESIAN_POINT('Ctrl Pts',(-10.9335472333948,23.0723779169368,
2.78189139164954));
#103446=CARTESIAN_POINT('Ctrl Pts',(-10.9428226510478,23.0734021040643,
2.79415863382085));
#103447=CARTESIAN_POINT('Ctrl Pts',(-10.9461767501791,23.0737772316565,
2.79866117952385));
#103448=CARTESIAN_POINT('Ctrl Pts',(-10.9495588799937,23.0741604490122,
2.80326977505809));
#103449=CARTESIAN_POINT('Ctrl Pts',(-10.9496192707213,23.0741672932999,
2.80335208778239));
#103450=CARTESIAN_POINT('Ctrl Pts',(-10.9497446767683,23.0741815093713,
2.80352306316844));
#103451=CARTESIAN_POINT('Ctrl Pts',(-10.9498096903923,23.0741888812225,
2.80361172710556));
#103452=CARTESIAN_POINT('Ctrl Pts',(-10.9499146882163,23.0742007899018,
2.80375496253993));
#103453=CARTESIAN_POINT('Ctrl Pts',(-10.9499546801361,23.0742053264332,
2.8038095283873));
#103454=CARTESIAN_POINT('Ctrl Pts',(-10.9500515661709,23.0742163185477,
2.80394174569729));
#103455=CARTESIAN_POINT('Ctrl Pts',(-10.9501084554518,23.0742227743144,
2.80401940066855));
#103456=CARTESIAN_POINT('Ctrl Pts',(-10.9502461107579,23.0742383988704,
2.80420735116147));
#103457=CARTESIAN_POINT('Ctrl Pts',(-10.9503268670896,23.0742475680309,
2.80431765375577));
#103458=CARTESIAN_POINT('Ctrl Pts',(-10.9507991597674,23.0743012097293,
2.80496297952106));
#103459=CARTESIAN_POINT('Ctrl Pts',(-10.9511902628288,23.0743456988309,
2.80549831825458));
#103460=CARTESIAN_POINT('Ctrl Pts',(-10.9545578418995,23.0747293642029,
2.81011601408111));
#103461=CARTESIAN_POINT('Ctrl Pts',(-10.9575084330614,23.0750695258186,
2.81421709936473));
#103462=CARTESIAN_POINT('Ctrl Pts',(-10.9642839489682,23.075860080017,2.82376349635286));
#103463=CARTESIAN_POINT('Ctrl Pts',(-10.9680892613445,23.0763112033964,
2.82922244968103));
#103464=CARTESIAN_POINT('Ctrl Pts',(-10.9803604777621,23.0777897166042,
2.84714819049596));
#103465=CARTESIAN_POINT('Ctrl Pts',(-10.9886331075552,23.0788242487294,
2.85974482155988));
#103466=CARTESIAN_POINT('Ctrl Pts',(-11.0401538772754,23.0855197383915,
2.94157502954212));
#103467=CARTESIAN_POINT('Ctrl Pts',(-11.0763389402264,23.0914354698669,
3.01497586133421));
#103468=CARTESIAN_POINT('Ctrl Pts',(-11.1234775660357,23.1014102870791,
3.14244919016272));
#103469=CARTESIAN_POINT('Ctrl Pts',(-11.1387687755876,23.1054106472644,
3.19463026933931));
#103470=CARTESIAN_POINT('Ctrl Pts',(-11.1538499245659,23.1104574535629,
3.26339056072969));
#103471=CARTESIAN_POINT('Ctrl Pts',(-11.1569732609394,23.1116002663262,
3.27916838279357));
#103472=CARTESIAN_POINT('Ctrl Pts',(-11.161643031155,23.1134834758004,3.30558804476212));
#103473=CARTESIAN_POINT('Ctrl Pts',(-11.1633686095288,23.1142314795262,
3.31619565002432));
#103474=CARTESIAN_POINT('Ctrl Pts',(-11.1655579064777,23.1152574471973,
3.33092313036986));
#103475=CARTESIAN_POINT('Ctrl Pts',(-11.1661453747261,23.1155417619797,
3.33502367591212));
#103476=CARTESIAN_POINT('Ctrl Pts',(-11.1671041127655,23.1160214930971,
3.34197681654123));
#103477=CARTESIAN_POINT('Ctrl Pts',(-11.1674865852185,23.1162175220266,
3.34482780353112));
#103478=CARTESIAN_POINT('Ctrl Pts',(-11.1682007026767,23.1165926620113,
3.35030304949369));
#103479=CARTESIAN_POINT('Ctrl Pts',(-11.1685339561704,23.116771865454,3.35292705090696));
#103480=CARTESIAN_POINT('Ctrl Pts',(-11.1693124900505,23.1172007582149,
3.35922687515752));
#103481=CARTESIAN_POINT('Ctrl Pts',(-11.1697492853397,23.1174499806069,
3.36290374754294));
#103482=CARTESIAN_POINT('Ctrl Pts',(-11.1712760585983,23.1183538333206,
3.37629468020565));
#103483=CARTESIAN_POINT('Ctrl Pts',(-11.1722624688999,23.1190030295047,
3.38602048015204));
#103484=CARTESIAN_POINT('Ctrl Pts',(-11.1784705570504,23.1236216894576,
3.45588548354031));
#103485=CARTESIAN_POINT('Ctrl Pts',(-11.1791835156877,23.1273831383303,
3.51634328370099));
#103486=CARTESIAN_POINT('Ctrl Pts',(-11.1708637312362,23.1353046675188,
3.64399862292482));
#103487=CARTESIAN_POINT('Ctrl Pts',(-11.1606809909735,23.1394482905764,
3.7108945379637));
#103488=CARTESIAN_POINT('Ctrl Pts',(-11.1366284329172,23.1459590772207,
3.81046480039585));
#103489=CARTESIAN_POINT('Ctrl Pts',(-11.1269326789683,23.1482116676388,
3.84399848368288));
#103490=CARTESIAN_POINT('Ctrl Pts',(-11.1128407269703,23.1511144503027,
3.88569927459808));
#103491=CARTESIAN_POINT('Ctrl Pts',(-11.1098175015094,23.1517196634186,
3.89431398606395));
#103492=CARTESIAN_POINT('Ctrl Pts',(-11.1048012336015,23.1526970374537,
3.90809303711878));
#103493=CARTESIAN_POINT('Ctrl Pts',(-11.1028713642119,23.1530671130495,
3.91328010469405));
#103494=CARTESIAN_POINT('Ctrl Pts',(-11.0991270511796,23.1537741234056,
3.92313098420012));
#103495=CARTESIAN_POINT('Ctrl Pts',(-11.0973192969696,23.1541108296978,
3.92779722251508));
#103496=CARTESIAN_POINT('Ctrl Pts',(-11.0931191626544,23.1548827778113,
3.93843695559237));
#103497=CARTESIAN_POINT('Ctrl Pts',(-11.0907074721916,23.1553186564355,
3.94440260467422));
#103498=CARTESIAN_POINT('Ctrl Pts',(-11.0830934677002,23.1566726173322,
3.96280152357305));
#103499=CARTESIAN_POINT('Ctrl Pts',(-11.0777266850735,23.157596182324,3.9751651039506));
#103500=CARTESIAN_POINT('Ctrl Pts',(-11.0300216796261,23.1655560583394,
4.08009610726531));
#103501=CARTESIAN_POINT('Ctrl Pts',(-10.9760667377985,23.1730126849874,
4.16688925384512));
#103502=CARTESIAN_POINT('Ctrl Pts',(-10.8750602016379,23.1847159812735,
4.29038261986591));
#103503=CARTESIAN_POINT('Ctrl Pts',(-10.8352233383987,23.1889292672099,
4.33236927401729));
#103504=CARTESIAN_POINT('Ctrl Pts',(-10.7871195674739,23.1934557690624,
4.37612211592631));
#103505=CARTESIAN_POINT('Ctrl Pts',(-10.7817344968149,23.1939551916662,
4.38093039370179));
#103506=CARTESIAN_POINT('Ctrl Pts',(-10.7736498893391,23.1946937439817,
4.38801654283783));
#103507=CARTESIAN_POINT('Ctrl Pts',(-10.770983891727,23.1949355007695,4.39033216899616));
#103508=CARTESIAN_POINT('Ctrl Pts',(-10.7663956429986,23.1953484534316,
4.39428135607766));
#103509=CARTESIAN_POINT('Ctrl Pts',(-10.7644785193549,23.1955200722671,
4.39592076620813));
#103510=CARTESIAN_POINT('Ctrl Pts',(-10.7601120430664,23.1959088463342,
4.3996304960616));
#103511=CARTESIAN_POINT('Ctrl Pts',(-10.7576594925098,23.1961257230802,
4.40169697875158));
#103512=CARTESIAN_POINT('Ctrl Pts',(-10.7509642206263,23.1967138405205,
4.40729171175524));
#103513=CARTESIAN_POINT('Ctrl Pts',(-10.7467050294985,23.1970836993063,
4.41080025953542));
#103514=CARTESIAN_POINT('Ctrl Pts',(-10.7254365992137,23.1989104231113,
4.42807084894456));
#103515=CARTESIAN_POINT('Ctrl Pts',(-10.7080696048275,23.2003385461329,
4.44138798754538));
#103516=CARTESIAN_POINT('Ctrl Pts',(-10.6724560469037,23.2031649719364,
4.46715313371203));
#103517=CARTESIAN_POINT('Ctrl Pts',(-10.6542106184531,23.2045623330808,
4.47958709829406));
#103518=CARTESIAN_POINT('Ctrl Pts',(-10.5519067878126,23.2121854605729,
4.54517140559674));
#103519=CARTESIAN_POINT('Ctrl Pts',(-10.4617311208844,23.2181749113842,
4.58802078615555));
#103520=CARTESIAN_POINT('Ctrl Pts',(-10.3410113574056,23.2263174644757,
4.62763844376149));
#103521=CARTESIAN_POINT('Ctrl Pts',(-10.3144881075835,23.2281107016962,
4.63532120753413));
#103522=CARTESIAN_POINT('Ctrl Pts',(-10.2795252391042,23.2304921148332,
4.64412942324497));
#103523=CARTESIAN_POINT('Ctrl Pts',(-10.2713076620247,23.2310530598692,
4.64610586019299));
#103524=CARTESIAN_POINT('Ctrl Pts',(-10.2578194845839,23.2319761064925,
4.64919675779049));
#103525=CARTESIAN_POINT('Ctrl Pts',(-10.2525611540561,23.232336527722,4.65036382791168));
#103526=CARTESIAN_POINT('Ctrl Pts',(-10.2423568635783,23.2330371552342,
4.65255530186122));
#103527=CARTESIAN_POINT('Ctrl Pts',(-10.2374119472146,23.2333772154745,
4.65358404077084));
#103528=CARTESIAN_POINT('Ctrl Pts',(-10.2259455980152,23.2341670796585,
4.65589264878858));
#103529=CARTESIAN_POINT('Ctrl Pts',(-10.219419696762,23.2346176104722,4.65714917893545));
#103530=CARTESIAN_POINT('Ctrl Pts',(-10.1981106318597,23.2360921595994,
4.66106539550293));
#103531=CARTESIAN_POINT('Ctrl Pts',(-10.1832876786367,23.2371232671596,
4.66349742829467));
#103532=CARTESIAN_POINT('Ctrl Pts',(-10.0873648709804,23.2438334923351,
4.67735721332051));
#103533=CARTESIAN_POINT('Ctrl Pts',(-10.0053209671194,23.24976935697,4.68058022344533));
#103534=CARTESIAN_POINT('Ctrl Pts',(-9.86958271485929,23.2597528662967,
4.67175892140751));
#103535=CARTESIAN_POINT('Ctrl Pts',(-9.81584746281155,23.2637415001055,
4.66452396072934));
#103536=CARTESIAN_POINT('Ctrl Pts',(-9.74707148462057,23.268775173617,4.65038255837818));
#103537=CARTESIAN_POINT('Ctrl Pts',(-9.73141120675879,23.2699161468259,
4.64682735359267));
#103538=CARTESIAN_POINT('Ctrl Pts',(-9.70541135519511,23.271796655567,4.64036301286977));
#103539=CARTESIAN_POINT('Ctrl Pts',(-9.69503039103909,23.2725437718774,
4.63763079636926));
#103540=CARTESIAN_POINT('Ctrl Pts',(-9.68069851937139,23.2735687356609,
4.63364843312371));
#103541=CARTESIAN_POINT('Ctrl Pts',(-9.67671505394268,23.2738529180562,
4.63251889627262));
#103542=CARTESIAN_POINT('Ctrl Pts',(-9.66997472093026,23.2743324917589,
4.63056917064355));
#103543=CARTESIAN_POINT('Ctrl Pts',(-9.66721477364654,23.2745284947388,
4.6297598542318));
#103544=CARTESIAN_POINT('Ctrl Pts',(-9.66192192844809,23.2749036371779,
4.62818672148005));
#103545=CARTESIAN_POINT('Ctrl Pts',(-9.65938861374635,23.2750828687189,
4.62742447414259));
#103546=CARTESIAN_POINT('Ctrl Pts',(-9.65331431013368,23.2755118970093,
4.62557443842932));
#103547=CARTESIAN_POINT('Ctrl Pts',(-9.64977581489861,23.2757612261753,
4.62447845915314));
#103548=CARTESIAN_POINT('Ctrl Pts',(-9.63690677944093,23.2766660344139,
4.62042588963239));
#103549=CARTESIAN_POINT('Ctrl Pts',(-9.62760770321934,23.2773160638543,
4.61736961372478));
#103550=CARTESIAN_POINT('Ctrl Pts',(-9.56146693430513,23.2819196437725,
4.59471403376653));
#103551=CARTESIAN_POINT('Ctrl Pts',(-9.50615404050545,23.2856669362543,
4.57090061935014));
#103552=CARTESIAN_POINT('Ctrl Pts',(-9.39293194450838,23.2935845140801,
4.51150806525642));
#103553=CARTESIAN_POINT('Ctrl Pts',(-9.33579561405133,23.2977378838956,
4.47494210889107));
#103554=CARTESIAN_POINT('Ctrl Pts',(-9.25441931212821,23.3042620349929,
4.41237346487831));
#103555=CARTESIAN_POINT('Ctrl Pts',(-9.22768379963132,23.3065176016736,
4.38985572972593));
#103556=CARTESIAN_POINT('Ctrl Pts',(-9.19527308581868,23.3094237434334,
4.35999597565929));
#103557=CARTESIAN_POINT('Ctrl Pts',(-9.18862811796076,23.3100292086062,
4.35372955074626));
#103558=CARTESIAN_POINT('Ctrl Pts',(-9.17807422803848,23.311006892302,4.34354236850563));
#103559=CARTESIAN_POINT('Ctrl Pts',(-9.1741188085816,23.3113770230975,4.33967014830915));
#103560=CARTESIAN_POINT('Ctrl Pts',(-9.16663988786045,23.3120840749315,
4.33224457101203));
#103561=CARTESIAN_POINT('Ctrl Pts',(-9.16311144050307,23.3124207670553,
4.32869634977843));
#103562=CARTESIAN_POINT('Ctrl Pts',(-9.15509875806343,23.3131925920681,
4.32053539758769));
#103563=CARTESIAN_POINT('Ctrl Pts',(-9.15062952340823,23.3136283610314,
4.31590822888441));
#103564=CARTESIAN_POINT('Ctrl Pts',(-9.13692071714168,23.314981638236,4.30148027813739));
#103565=CARTESIAN_POINT('Ctrl Pts',(-9.12781147823395,23.3159046212112,
4.29155773069694));
#103566=CARTESIAN_POINT('Ctrl Pts',(-9.05129066452536,23.3238682733305,
4.20528003479912));
#103567=CARTESIAN_POINT('Ctrl Pts',(-8.99388978077641,23.331329879206,4.12064719507611));
#103568=CARTESIAN_POINT('Ctrl Pts',(-8.92212701591141,23.3430341715243,
3.97814136760841));
#103569=CARTESIAN_POINT('Ctrl Pts',(-8.89998073013925,23.3472436999236,
3.92472171097933));
#103570=CARTESIAN_POINT('Ctrl Pts',(-8.87957469040795,23.3517666476949,
3.86303482016365));
#103571=CARTESIAN_POINT('Ctrl Pts',(-8.87737090427838,23.3522659706824,
3.85616158552503));
#103572=CARTESIAN_POINT('Ctrl Pts',(-8.87418327210011,23.3530044050559,
3.845896263104));
#103573=CARTESIAN_POINT('Ctrl Pts',(-8.87315132052637,23.353246142325,3.84251946519972));
#103574=CARTESIAN_POINT('Ctrl Pts',(-8.87140820260761,23.3536590732679,
3.83672240812784));
#103575=CARTESIAN_POINT('Ctrl Pts',(-8.87068961010261,23.3538306897738,
3.83430445553303));
#103576=CARTESIAN_POINT('Ctrl Pts',(-8.86907499450222,23.3542194743091,
3.82880690477619));
#103577=CARTESIAN_POINT('Ctrl Pts',(-8.86818377872898,23.3544363637547,
3.82572594397406));
#103578=CARTESIAN_POINT('Ctrl Pts',(-8.86579327630545,23.3550245493437,
3.81733362252417));
#103579=CARTESIAN_POINT('Ctrl Pts',(-8.86431869541627,23.3553944630465,
3.812015219895));
#103580=CARTESIAN_POINT('Ctrl Pts',(-8.85718159024956,23.3572218993939,
3.78555258239075));
#103581=CARTESIAN_POINT('Ctrl Pts',(-8.8520715005743,23.3586506532497,3.76426218723496));
#103582=CARTESIAN_POINT('Ctrl Pts',(-8.84300645704952,23.3614775551634,
3.72124235529943));
#103583=CARTESIAN_POINT('Ctrl Pts',(-8.83906323058472,23.3628747843244,
3.69951980591548));
#103584=CARTESIAN_POINT('Ctrl Pts',(-8.8207261347638,23.3704987079885,3.57937635004485));
#103585=CARTESIAN_POINT('Ctrl Pts',(-8.81823442504374,23.3764890921039,
3.4795532868496));
#103586=CARTESIAN_POINT('Ctrl Pts',(-8.83111435099077,23.3846315207775,
3.35315856518573));
#103587=CARTESIAN_POINT('Ctrl Pts',(-8.83487414616044,23.3864234507394,
3.32582301841254));
#103588=CARTESIAN_POINT('Ctrl Pts',(-8.84103443793159,23.3888033700423,
3.29032099429569));
#103589=CARTESIAN_POINT('Ctrl Pts',(-8.84256855366958,23.3893641722794,
3.28201169674781));
#103590=CARTESIAN_POINT('Ctrl Pts',(-8.84522668774398,23.3902870440368,
3.26843431396956));
#103591=CARTESIAN_POINT('Ctrl Pts',(-8.84629769129515,23.3906474344519,
3.26315606215587));
#103592=CARTESIAN_POINT('Ctrl Pts',(-8.84844320053769,23.3913480450722,
3.25294228852423));
#103593=CARTESIAN_POINT('Ctrl Pts',(-8.84951333011119,23.3916881195162,
3.24800595994144));
#103594=CARTESIAN_POINT('Ctrl Pts',(-8.85206518646545,23.3924780801647,
3.23658984714381));
#103595=CARTESIAN_POINT('Ctrl Pts',(-8.85357007075657,23.3929286937872,
3.23011547110349));
#103596=CARTESIAN_POINT('Ctrl Pts',(-8.85865562653411,23.3944037960693,
3.20904656398069));
#103597=CARTESIAN_POINT('Ctrl Pts',(-8.8624607037958,23.3954353813628,3.19450827504879));
#103598=CARTESIAN_POINT('Ctrl Pts',(-8.8887266483475,23.4021295051825,3.10145911988546));
#103599=CARTESIAN_POINT('Ctrl Pts',(-8.91901963041153,23.4080471221999,
3.02540530811363));
#103600=CARTESIAN_POINT('Ctrl Pts',(-8.98924242682943,23.4191460779312,
2.8914707554874));
#103601=CARTESIAN_POINT('Ctrl Pts',(-9.02696224635812,23.4242793743449,
2.83281345055004));
#103602=CARTESIAN_POINT('Ctrl Pts',(-9.07662172037985,23.4299714584954,
2.76883853567892));
#103603=CARTESIAN_POINT('Ctrl Pts',(-9.08372905434086,23.430764245782,2.75995127693934));
#103604=CARTESIAN_POINT('Ctrl Pts',(-9.09365768594777,23.4318406940891,
2.74789853372323));
#103605=CARTESIAN_POINT('Ctrl Pts',(-9.0963686448159,23.4321315331021,2.74464354034595));
#103606=CARTESIAN_POINT('Ctrl Pts',(-9.10096181598024,23.4326190485995,
2.73918873108227));
#103607=CARTESIAN_POINT('Ctrl Pts',(-9.10283466559849,23.4328163833394,
2.73698112302647));
#103608=CARTESIAN_POINT('Ctrl Pts',(-9.10642145665841,23.4331915239221,
2.73278468344091));
#103609=CARTESIAN_POINT('Ctrl Pts',(-9.10813393017699,23.4333694367857,
2.73079465100173));
#103610=CARTESIAN_POINT('Ctrl Pts',(-9.11222835799636,23.4337920308252,
2.72606865097102));
#103611=CARTESIAN_POINT('Ctrl Pts',(-9.1146163441647,23.4340362754754,2.72333790860702));
#103612=CARTESIAN_POINT('Ctrl Pts',(-9.12314542351985,23.4349009582636,
2.71367508032983));
#103613=CARTESIAN_POINT('Ctrl Pts',(-9.12935581397608,23.4355165638523,
2.70680422210237));
#103614=CARTESIAN_POINT('Ctrl Pts',(-9.18792819945987,23.4412018654453,
2.64351962941284));
#103615=CARTESIAN_POINT('Ctrl Pts',(-9.24562909126624,23.4459266187752,
2.59228458586582));
#103616=CARTESIAN_POINT('Ctrl Pts',(-9.37417809794799,23.4557485472166,
2.49892732677693));
#103617=CARTESIAN_POINT('Ctrl Pts',(-9.44525788318716,23.4608319106327,
2.45785880602235));
#103618=CARTESIAN_POINT('Ctrl Pts',(-9.530797020055,23.4669757749784,2.41968384768958));
#103619=CARTESIAN_POINT('Ctrl Pts',(-9.54164876213505,23.4677552195766,
2.41503523026823));
#103620=CARTESIAN_POINT('Ctrl Pts',(-9.5582154395472,23.4689460590446,2.40823137312488));
#103621=CARTESIAN_POINT('Ctrl Pts',(-9.56388050004409,23.4693534301441,
2.405956074068));
#103622=CARTESIAN_POINT('Ctrl Pts',(-9.57374709562373,23.4700633211342,
2.40208209302186));
#103623=CARTESIAN_POINT('Ctrl Pts',(-9.5779406068059,23.4703651610101,2.40046321725575));
#103624=CARTESIAN_POINT('Ctrl Pts',(-9.5873603871918,23.471043501198,2.39688860455902));
#103625=CARTESIAN_POINT('Ctrl Pts',(-9.59259146604538,23.4714204262742,
2.39494593552422));
#103626=CARTESIAN_POINT('Ctrl Pts',(-9.60661313880329,23.4724314587763,
2.38985179146799));
#103627=CARTESIAN_POINT('Ctrl Pts',(-9.61542758890321,23.4730677604288,
2.38676762563264));
#103628=CARTESIAN_POINT('Ctrl Pts',(-9.65570011603182,23.475978981281,2.37321168722426));
#103629=CARTESIAN_POINT('Ctrl Pts',(-9.68755228883306,23.4782931822013,
2.36396727032804));
#103630=CARTESIAN_POINT('Ctrl Pts',(-9.74996777618204,23.4828532652028,
2.34867601877673));
#103631=CARTESIAN_POINT('Ctrl Pts',(-9.78044374222133,23.4850911448363,
2.34247894706917));
#103632=CARTESIAN_POINT('Ctrl Pts',(-9.81110406371068,23.4873487054734,
2.3374969300026));
#103633=CARTESIAN_POINT('Origin',(-10.,12.3756328852638,3.5));
#103634=CARTESIAN_POINT('',(-9.81110406371068,24.0873412831715,2.3374969300026));
#103635=CARTESIAN_POINT('',(-9.81110406371069,23.9889087884094,2.3374969300026));
#103636=CARTESIAN_POINT('',(-9.81110406371068,12.3756328852638,2.3374969300026));
#103637=CARTESIAN_POINT('Ctrl Pts',(-9.81110406371069,24.0873412831715,
2.3374969300026));
#103638=CARTESIAN_POINT('Ctrl Pts',(-9.74357372492119,24.0824554593664,
2.34846998194783));
#103639=CARTESIAN_POINT('Ctrl Pts',(-9.67707560096892,24.0774182711905,
2.3653149679055));
#103640=CARTESIAN_POINT('Ctrl Pts',(-9.55774576776678,24.0681478523538,
2.40690680585405));
#103641=CARTESIAN_POINT('Ctrl Pts',(-9.50459022776225,24.063930227775,2.42994752981934));
#103642=CARTESIAN_POINT('Ctrl Pts',(-9.44694158882869,24.0593995462754,
2.46015692936817));
#103643=CARTESIAN_POINT('Ctrl Pts',(-9.44057557513891,24.0588999157289,
2.46356788108037));
#103644=CARTESIAN_POINT('Ctrl Pts',(-9.43114311266536,24.058161080565,2.46873408803481));
#103645=CARTESIAN_POINT('Ctrl Pts',(-9.4280526795725,24.057919246332,2.47044485192393));
#103646=CARTESIAN_POINT('Ctrl Pts',(-9.42276799924539,24.0575061730287,
2.4734014192899));
#103647=CARTESIAN_POINT('Ctrl Pts',(-9.42057001289399,24.057334510611,2.47464039522845));
#103648=CARTESIAN_POINT('Ctrl Pts',(-9.41558679633419,24.0569456536593,
2.47747050970815));
#103649=CARTESIAN_POINT('Ctrl Pts',(-9.41280407413561,24.0567287376857,
2.47906596863196));
#103650=CARTESIAN_POINT('Ctrl Pts',(-9.40525148582439,24.0561405330082,
2.48343729971027));
#103651=CARTESIAN_POINT('Ctrl Pts',(-9.40049448221763,24.0557706267073,
2.48623540412376));
#103652=CARTESIAN_POINT('Ctrl Pts',(-9.37697719181959,24.0539438723636,
2.50029187668128));
#103653=CARTESIAN_POINT('Ctrl Pts',(-9.35851213514121,24.0525157692467,
2.51203885762965));
#103654=CARTESIAN_POINT('Ctrl Pts',(-9.32209675321034,24.0496893842896,
2.53665712168377));
#103655=CARTESIAN_POINT('Ctrl Pts',(-9.30416001060986,24.0482920442572,
2.5495321574285));
#103656=CARTESIAN_POINT('Ctrl Pts',(-9.20742490449701,24.0406654568903,
2.62317599148236));
#103657=CARTESIAN_POINT('Ctrl Pts',(-9.13621433393267,24.0346728069635,
2.69323458384475));
#103658=CARTESIAN_POINT('Ctrl Pts',(-9.05760909087374,24.0265292441198,
2.79306718509312));
#103659=CARTESIAN_POINT('Ctrl Pts',(-9.04132611092989,24.0247389821614,
2.81531115529514));
#103660=CARTESIAN_POINT('Ctrl Pts',(-9.02109139216019,24.0223608932655,
2.8450920909953));
#103661=CARTESIAN_POINT('Ctrl Pts',(-9.01641902406435,24.0218002003561,
2.85213049973338));
#103662=CARTESIAN_POINT('Ctrl Pts',(-9.0088923746425,24.0208774118868,2.86373767280989));
#103663=CARTESIAN_POINT('Ctrl Pts',(-9.00599294943121,24.0205169943684,
2.86827691523815));
#103664=CARTESIAN_POINT('Ctrl Pts',(-9.00043433634345,24.0198162614892,
2.87711231068603));
#103665=CARTESIAN_POINT('Ctrl Pts',(-8.99777145246276,24.019476091521,2.88140600828212));
#103666=CARTESIAN_POINT('Ctrl Pts',(-8.99166766671436,24.0186858055833,
2.89139076962594));
#103667=CARTESIAN_POINT('Ctrl Pts',(-8.98824720512307,24.0182349609094,
2.89709406326543));
#103668=CARTESIAN_POINT('Ctrl Pts',(-8.97724846161348,24.0167586368137,
2.91579061538641));
#103669=CARTESIAN_POINT('Ctrl Pts',(-8.96987102631648,24.0157260447666,
2.92889968003823));
#103670=CARTESIAN_POINT('Ctrl Pts',(-8.92429944104744,24.0090645634159,
3.01363378462953));
#103671=CARTESIAN_POINT('Ctrl Pts',(-8.89335218272255,24.0031839340262,
3.08889191535067));
#103672=CARTESIAN_POINT('Ctrl Pts',(-8.85491027822392,23.9932144415457,
3.21918512241161));
#103673=CARTESIAN_POINT('Ctrl Pts',(-8.84310383763222,23.9891841142858,
3.27266916464562));
#103674=CARTESIAN_POINT('Ctrl Pts',(-8.83268291164885,23.9841037123425,
3.34275311502857));
#103675=CARTESIAN_POINT('Ctrl Pts',(-8.83063673390186,23.982956156826,3.35877190580605));
#103676=CARTESIAN_POINT('Ctrl Pts',(-8.82777494406594,23.9810659550975,
3.38554624212253));
#103677=CARTESIAN_POINT('Ctrl Pts',(-8.82677650935534,23.9803156338232,
3.39627967330447));
#103678=CARTESIAN_POINT('Ctrl Pts',(-8.82559809730526,23.9792870091483,
3.41116060795672));
#103679=CARTESIAN_POINT('Ctrl Pts',(-8.82529250078572,23.9790023128278,
3.41529723006494));
#103680=CARTESIAN_POINT('Ctrl Pts',(-8.82481188669995,23.9785220947086,
3.42230673240159));
#103681=CARTESIAN_POINT('Ctrl Pts',(-8.82462553624673,23.9783259577827,
3.42517877234607));
#103682=CARTESIAN_POINT('Ctrl Pts',(-8.82428812759596,23.9779507093295,
3.43069161837056));
#103683=CARTESIAN_POINT('Ctrl Pts',(-8.82413543563939,23.9777715047626,
3.43333227685037));
#103684=CARTESIAN_POINT('Ctrl Pts',(-8.82379047927197,23.9773427681755,
3.43966826776755));
#103685=CARTESIAN_POINT('Ctrl Pts',(-8.82360672973643,23.9770937018829,
3.44336406470333));
#103686=CARTESIAN_POINT('Ctrl Pts',(-8.82300216036569,23.9761916952841,
3.45680043955325));
#103687=CARTESIAN_POINT('Ctrl Pts',(-8.82268486146288,23.9755441576955,
3.46654560823821));
#103688=CARTESIAN_POINT('Ctrl Pts',(-8.82125301953222,23.970859658916,3.53766721136896));
#103689=CARTESIAN_POINT('Ctrl Pts',(-8.82481745000881,23.9670381129837,
3.59905170948979));
#103690=CARTESIAN_POINT('Ctrl Pts',(-8.84222150143454,23.9591015964265,
3.72606693842428));
#103691=CARTESIAN_POINT('Ctrl Pts',(-8.85690332902964,23.9550012799187,
3.79135320048569));
#103692=CARTESIAN_POINT('Ctrl Pts',(-8.88749465769506,23.9485498270871,
3.88811057869496));
#103693=CARTESIAN_POINT('Ctrl Pts',(-8.89940476417073,23.9463104259834,
3.92069908932711));
#103694=CARTESIAN_POINT('Ctrl Pts',(-8.91623804203854,23.9434223797439,
3.96112705635159));
#103695=CARTESIAN_POINT('Ctrl Pts',(-8.91983917181495,23.9428181325545,
3.96950050175579));
#103696=CARTESIAN_POINT('Ctrl Pts',(-8.92578172920347,23.9418418486449,
3.98288795744225));
#103697=CARTESIAN_POINT('Ctrl Pts',(-8.92806198282407,23.9414718873023,
3.987928845543));
#103698=CARTESIAN_POINT('Ctrl Pts',(-8.93247342755905,23.9407647846526,
3.99750090624318));
#103699=CARTESIAN_POINT('Ctrl Pts',(-8.9345981692479,23.9404278698307,4.00203493133102));
#103700=CARTESIAN_POINT('Ctrl Pts',(-8.93952379797838,23.9396550011608,
4.01237371794138));
#103701=CARTESIAN_POINT('Ctrl Pts',(-8.9423435310397,23.9392184064738,4.01816927030507));
#103702=CARTESIAN_POINT('Ctrl Pts',(-8.95122711733754,23.9378605300416,
4.03605354949671));
#103703=CARTESIAN_POINT('Ctrl Pts',(-8.95745154596989,23.9369337221889,
4.04806081943611));
#103704=CARTESIAN_POINT('Ctrl Pts',(-9.0121022850983,23.9289953170451,4.14918390318014));
#103705=CARTESIAN_POINT('Ctrl Pts',(-9.07163837185019,23.9215669463448,
4.23179082672774));
#103706=CARTESIAN_POINT('Ctrl Pts',(-9.18071481933319,23.9098705686517,
4.34807872319119));
#103707=CARTESIAN_POINT('Ctrl Pts',(-9.22351534095563,23.9056371468017,
4.38743388824816));
#103708=CARTESIAN_POINT('Ctrl Pts',(-9.27471694161216,23.9010914306633,
4.42796109787714));
#103709=CARTESIAN_POINT('Ctrl Pts',(-9.28042619009648,23.9005913363944,
4.43239522340341));
#103710=CARTESIAN_POINT('Ctrl Pts',(-9.28898698730006,23.8998519253699,
4.43891855198856));
#103711=CARTESIAN_POINT('Ctrl Pts',(-9.29180756887576,23.8996099742054,
4.44104783768997));
#103712=CARTESIAN_POINT('Ctrl Pts',(-9.29665874937702,23.8991967460305,
4.44467587914371));
#103713=CARTESIAN_POINT('Ctrl Pts',(-9.29868462319215,23.8990250451092,
4.44618083586683));
#103714=CARTESIAN_POINT('Ctrl Pts',(-9.30329625533382,23.8986361598701,
4.44958372055939));
#103715=CARTESIAN_POINT('Ctrl Pts',(-9.30588493877044,23.8984192537893,
4.45147760487521));
#103716=CARTESIAN_POINT('Ctrl Pts',(-9.31294709335089,23.8978311868983,
4.45660012604585));
#103717=CARTESIAN_POINT('Ctrl Pts',(-9.3174356340809,23.8974614068988,4.45980799487661));
#103718=CARTESIAN_POINT('Ctrl Pts',(-9.33981231433111,23.8956366935544,
4.47556378972595));
#103719=CARTESIAN_POINT('Ctrl Pts',(-9.35802598237196,23.8942104215255,
4.48764467117932));
#103720=CARTESIAN_POINT('Ctrl Pts',(-9.3952985797548,23.8913854147618,4.51089996266216));
#103721=CARTESIAN_POINT('Ctrl Pts',(-9.41435644041523,23.889987687607,4.52205883430514));
#103722=CARTESIAN_POINT('Ctrl Pts',(-9.52096836402355,23.8823601062256,
4.58052098527914));
#103723=CARTESIAN_POINT('Ctrl Pts',(-9.61392727158488,23.8763670395781,
4.61711469826957));
#103724=CARTESIAN_POINT('Ctrl Pts',(-9.73710838056421,23.8682223059457,
4.64836550184109));
#103725=CARTESIAN_POINT('Ctrl Pts',(-9.76406263940538,23.8664312287492,
4.65420479131426));
#103726=CARTESIAN_POINT('Ctrl Pts',(-9.79951152840016,23.8640521687142,
4.66059072806934));
#103727=CARTESIAN_POINT('Ctrl Pts',(-9.80784338234675,23.8634913431225,
4.66199926567614));
#103728=CARTESIAN_POINT('Ctrl Pts',(-9.82151059006454,23.8625683620116,
4.66415875806456));
#103729=CARTESIAN_POINT('Ctrl Pts',(-9.82683731468442,23.862207885294,4.66496298920162));
#103730=CARTESIAN_POINT('Ctrl Pts',(-9.83717069919895,23.8615070551732,
4.66645069069539));
#103731=CARTESIAN_POINT('Ctrl Pts',(-9.84217661719173,23.861166847301,4.66713854082958));
#103732=CARTESIAN_POINT('Ctrl Pts',(-9.85378121420336,23.8603764989538,
4.66865707584187));
#103733=CARTESIAN_POINT('Ctrl Pts',(-9.86038275892182,23.8599256299,4.66946411534257));
#103734=CARTESIAN_POINT('Ctrl Pts',(-9.88193529603711,23.8584493350579,
4.671913825944));
#103735=CARTESIAN_POINT('Ctrl Pts',(-9.89691045647981,23.857416798602,4.67332595612959));
#103736=CARTESIAN_POINT('Ctrl Pts',(-9.9929054765429,23.850751635935,4.68052625416412));
#103737=CARTESIAN_POINT('Ctrl Pts',(-10.0742996007773,23.8448669287615,
4.67820524163744));
#103738=CARTESIAN_POINT('Ctrl Pts',(-10.2089777164519,23.8348966307027,
4.66034953611414));
#103739=CARTESIAN_POINT('Ctrl Pts',(-10.262599784569,23.8308696100445,4.64940186962942));
#103740=CARTESIAN_POINT('Ctrl Pts',(-10.3308203454896,23.8257928676023,
4.6304483410427));
#103741=CARTESIAN_POINT('Ctrl Pts',(-10.3462814384368,23.8246458002523,
4.62580849756253));
#103742=CARTESIAN_POINT('Ctrl Pts',(-10.3718981639098,23.8227562969774,
4.617543258122));
#103743=CARTESIAN_POINT('Ctrl Pts',(-10.382107847746,23.8220061940752,4.61409370857377));
#103744=CARTESIAN_POINT('Ctrl Pts',(-10.3961799668054,23.8209777969046,
4.60912294129082));
#103745=CARTESIAN_POINT('Ctrl Pts',(-10.4000834927303,23.8206931144513,
4.60772084261028));
#103746=CARTESIAN_POINT('Ctrl Pts',(-10.4066831482057,23.8202129004431,
4.6053108898631));
#103747=CARTESIAN_POINT('Ctrl Pts',(-10.4093831152979,23.8200167539753,
4.60431372891498));
#103748=CARTESIAN_POINT('Ctrl Pts',(-10.4145573232763,23.8196414944539,
4.60238118839328));
#103749=CARTESIAN_POINT('Ctrl Pts',(-10.4170320940141,23.8194622883326,
4.60144736221059));
#103750=CARTESIAN_POINT('Ctrl Pts',(-10.4229616827652,23.8190335240828,
4.59918705067032));
#103751=CARTESIAN_POINT('Ctrl Pts',(-10.4264134629599,23.8187844318948,
4.59785259346538));
#103752=CARTESIAN_POINT('Ctrl Pts',(-10.4389392675885,23.8178821609235,
4.59294213280805));
#103753=CARTESIAN_POINT('Ctrl Pts',(-10.4479753778139,23.8172343895273,
4.58926960042853));
#103754=CARTESIAN_POINT('Ctrl Pts',(-10.5131930964369,23.8125746184801,
4.56181438548205));
#103755=CARTESIAN_POINT('Ctrl Pts',(-10.5675046499917,23.8087753158279,
4.53380723042979));
#103756=CARTESIAN_POINT('Ctrl Pts',(-10.6764604641247,23.8008441738512,
4.46643468616136));
#103757=CARTESIAN_POINT('Ctrl Pts',(-10.7303923847933,23.7967276251116,
4.42634826377169));
#103758=CARTESIAN_POINT('Ctrl Pts',(-10.8066474358408,23.7902539068963,
4.3588500362639));
#103759=CARTESIAN_POINT('Ctrl Pts',(-10.8316420103137,23.7880095338998,
4.3346703983474));
#103760=CARTESIAN_POINT('Ctrl Pts',(-10.8617975793566,23.7851159035078,
4.30279710120222));
#103761=CARTESIAN_POINT('Ctrl Pts',(-10.8679887042022,23.7845112645562,
4.29609914904853));
#103762=CARTESIAN_POINT('Ctrl Pts',(-10.8778099514203,23.7835345190767,
4.28522313599939));
#103763=CARTESIAN_POINT('Ctrl Pts',(-10.8814895878258,23.7831644919395,
4.28109012853766));
#103764=CARTESIAN_POINT('Ctrl Pts',(-10.8884425259255,23.7824573767328,
4.27316880758897));
#103765=CARTESIAN_POINT('Ctrl Pts',(-10.8917210734431,23.7821205159151,
4.26938524338956));
#103766=CARTESIAN_POINT('Ctrl Pts',(-10.8991627192592,23.7813479322799,
4.26068585021914));
#103767=CARTESIAN_POINT('Ctrl Pts',(-10.9033097783901,23.7809115699771,
4.25575657445314));
#103768=CARTESIAN_POINT('Ctrl Pts',(-10.9160273047438,23.7795550318081,
4.24038605414415));
#103769=CARTESIAN_POINT('Ctrl Pts',(-10.9244584706811,23.7786293446285,
4.22983151600253));
#103770=CARTESIAN_POINT('Ctrl Pts',(-10.9947184730083,23.7706827911356,
4.1387054387195));
#103771=CARTESIAN_POINT('Ctrl Pts',(-11.0460555946995,23.7632438051067,
4.05060750729996));
#103772=CARTESIAN_POINT('Ctrl Pts',(-11.1079450174856,23.7515443441016,
3.90362442750183));
#103773=CARTESIAN_POINT('Ctrl Pts',(-11.126467130191,23.7473180290309,3.84860901352965));
#103774=CARTESIAN_POINT('Ctrl Pts',(-11.1426576443109,23.7427790904938,
3.785448377643));
#103775=CARTESIAN_POINT('Ctrl Pts',(-11.1443873879626,23.7422792162987,
3.77843272299209));
#103776=CARTESIAN_POINT('Ctrl Pts',(-11.1468666841089,23.7415400822145,
3.76796334510997));
#103777=CARTESIAN_POINT('Ctrl Pts',(-11.1476653972407,23.7412981901362,
3.7645216101626));
#103778=CARTESIAN_POINT('Ctrl Pts',(-11.1490080011032,23.7408850381905,
3.75861562905306));
#103779=CARTESIAN_POINT('Ctrl Pts',(-11.1495594720713,23.7407133547336,
3.75615317839993));
#103780=CARTESIAN_POINT('Ctrl Pts',(-11.1507939795114,23.7403244708959,
3.75055651745531));
#103781=CARTESIAN_POINT('Ctrl Pts',(-11.1514721289393,23.7401075489643,
3.7474212776147));
#103782=CARTESIAN_POINT('Ctrl Pts',(-11.1532819811434,23.739519388985,3.73888529136071));
#103783=CARTESIAN_POINT('Ctrl Pts',(-11.1543885694944,23.7391495325236,
3.73347921544909));
#103784=CARTESIAN_POINT('Ctrl Pts',(-11.1596910903611,23.7373237908082,
3.70661483876489));
#103785=CARTESIAN_POINT('Ctrl Pts',(-11.1633272106256,23.7358966061409,
3.68504881959785));
#103786=CARTESIAN_POINT('Ctrl Pts',(-11.1694237019178,23.7330709102144,
3.64152961432118));
#103787=CARTESIAN_POINT('Ctrl Pts',(-11.1718712487657,23.7316733736831,
3.61958386217328));
#103788=CARTESIAN_POINT('Ctrl Pts',(-11.1819462968778,23.7240452066313,
3.49840187809117));
#103789=CARTESIAN_POINT('Ctrl Pts',(-11.1775883343904,23.7180513238473,
3.39858102613226));
#103790=CARTESIAN_POINT('Ctrl Pts',(-11.1560622003909,23.7099068222259,
3.27334077835033));
#103791=CARTESIAN_POINT('Ctrl Pts',(-11.1504437949019,23.7081170279694,
3.24636029860222));
#103792=CARTESIAN_POINT('Ctrl Pts',(-11.1418736435704,23.7057394296445,
3.21139817680151));
#103793=CARTESIAN_POINT('Ctrl Pts',(-11.1397741930354,23.7051787397776,
3.20321520769412));
#103794=CARTESIAN_POINT('Ctrl Pts',(-11.1361922057639,23.704255921768,3.18985269522415));
#103795=CARTESIAN_POINT('Ctrl Pts',(-11.1347618149761,23.7038954712035,
3.1846593893443));
#103796=CARTESIAN_POINT('Ctrl Pts',(-11.1319206323133,23.7031946487214,
3.17461364521116));
#103797=CARTESIAN_POINT('Ctrl Pts',(-11.1305141349725,23.7028544220548,
3.16976010690089));
#103798=CARTESIAN_POINT('Ctrl Pts',(-11.1271838925165,23.7020639661097,
3.15853875187798));
#103799=CARTESIAN_POINT('Ctrl Pts',(-11.1252373610865,23.7016130076908,
3.15217793402919));
#103800=CARTESIAN_POINT('Ctrl Pts',(-11.1187119476671,23.7001361345097,
3.13148258902579));
#103801=CARTESIAN_POINT('Ctrl Pts',(-11.1139123688111,23.699103101537,3.11721977303774));
#103802=CARTESIAN_POINT('Ctrl Pts',(-11.0815667270918,23.6924582498196,
3.02686461374704));
#103803=CARTESIAN_POINT('Ctrl Pts',(-11.0465176558544,23.6865964223549,
2.95370340063427));
#103804=CARTESIAN_POINT('Ctrl Pts',(-10.975584889035,23.6766323653871,2.83792652717423));
#103805=CARTESIAN_POINT('Ctrl Pts',(-10.9436759959894,23.6725884644744,
2.79318789922231));
#103806=CARTESIAN_POINT('Ctrl Pts',(-10.8984726641327,23.6674928353562,
2.738354683249));
#103807=CARTESIAN_POINT('Ctrl Pts',(-10.8879267174741,23.6663431433701,
2.72608597604728));
#103808=CARTESIAN_POINT('Ctrl Pts',(-10.8699277940507,23.6644497853856,
2.7059992457024));
#103809=CARTESIAN_POINT('Ctrl Pts',(-10.8626142665421,23.6636984152081,
2.69805972002774));
#103810=CARTESIAN_POINT('Ctrl Pts',(-10.8523386489115,23.6626685791219,
2.68720782746603));
#103811=CARTESIAN_POINT('Ctrl Pts',(-10.8494690314039,23.6623837025155,
2.68420918480168));
#103812=CARTESIAN_POINT('Ctrl Pts',(-10.8445822445138,23.6619032529932,
2.67915642048078));
#103813=CARTESIAN_POINT('Ctrl Pts',(-10.8425733033742,23.6617070638589,
2.67709442892734));
#103814=CARTESIAN_POINT('Ctrl Pts',(-10.83870441001,23.6613317969085,2.67315239092663));
#103815=CARTESIAN_POINT('Ctrl Pts',(-10.8368456672802,23.6611526255885,
2.67127122319315));
#103816=CARTESIAN_POINT('Ctrl Pts',(-10.8323722001315,23.6607240381542,
2.66677418298574));
#103817=CARTESIAN_POINT('Ctrl Pts',(-10.829751438581,23.660475087089,2.66416431472123));
#103818=CARTESIAN_POINT('Ctrl Pts',(-10.8201873739642,23.6595740980788,
2.65472931909697));
#103819=CARTESIAN_POINT('Ctrl Pts',(-10.813171570096,23.6589274466233,2.64797777895053));
#103820=CARTESIAN_POINT('Ctrl Pts',(-10.7591421904687,23.6540472672213,
2.59725890354204));
#103821=CARTESIAN_POINT('Ctrl Pts',(-10.7086724273206,23.6500511697405,
2.55711931092429));
#103822=CARTESIAN_POINT('Ctrl Pts',(-10.6009091200361,23.6420284569847,
2.48497945380869));
#103823=CARTESIAN_POINT('Ctrl Pts',(-10.5437267541401,23.6380135668804,
2.45323402321985));
#103824=CARTESIAN_POINT('Ctrl Pts',(-10.4640496196473,23.6324492750353,
2.41729868158648));
#103825=CARTESIAN_POINT('Ctrl Pts',(-10.4436378104736,23.6310270875745,
2.4087761015558));
#103826=CARTESIAN_POINT('Ctrl Pts',(-10.4080996547845,23.6285472439129,
2.3950997311493));
#103827=CARTESIAN_POINT('Ctrl Pts',(-10.3930858020622,23.6274984933614,
2.38966966866181));
#103828=CARTESIAN_POINT('Ctrl Pts',(-10.371446705681,23.6259831872884,2.3823373497377));
#103829=CARTESIAN_POINT('Ctrl Pts',(-10.3649075000058,23.6255247898507,
2.38018529746614));
#103830=CARTESIAN_POINT('Ctrl Pts',(-10.3535183347448,23.6247254028659,
2.37654747525841));
#103831=CARTESIAN_POINT('Ctrl Pts',(-10.3486768984253,23.6243852764271,
2.37503546390294));
#103832=CARTESIAN_POINT('Ctrl Pts',(-10.3393249206759,23.6237275980221,
2.37218095110167));
#103833=CARTESIAN_POINT('Ctrl Pts',(-10.3348157944247,23.6234101940062,
2.37083411690671));
#103834=CARTESIAN_POINT('Ctrl Pts',(-10.3241084695806,23.6226557221821,
2.36770571249692));
#103835=CARTESIAN_POINT('Ctrl Pts',(-10.3179035242519,23.6222178947171,
2.36594797299477));
#103836=CARTESIAN_POINT('Ctrl Pts',(-10.2958414568409,23.6206588294125,
2.35989351276056));
#103837=CARTESIAN_POINT('Ctrl Pts',(-10.2799098501674,23.6195286770676,
2.35587789191278));
#103838=CARTESIAN_POINT('Ctrl Pts',(-10.1553293300501,23.6106534633178,
2.32723463508429));
#103839=CARTESIAN_POINT('Ctrl Pts',(-10.0437812076379,23.6024058353221,
2.31780765211192));
#103840=CARTESIAN_POINT('Ctrl Pts',(-9.89190655802231,23.5913047374816,
2.326512558362));
#103841=CARTESIAN_POINT('Ctrl Pts',(-9.85135104491018,23.5883624119763,
2.33095716989985));
#103842=CARTESIAN_POINT('Ctrl Pts',(-9.81110406370983,23.5855117083725,
2.33749693000274));
#103843=CARTESIAN_POINT('Ctrl Pts',(-9.81110406371068,23.4873487054734,
2.3374969300026));
#103844=CARTESIAN_POINT('Ctrl Pts',(-9.87134046747871,23.4917839927589,
2.32770907465656));
#103845=CARTESIAN_POINT('Ctrl Pts',(-9.93228809589294,23.4963001685831,
2.32261115923266));
#103846=CARTESIAN_POINT('Ctrl Pts',(-10.0359488392081,23.5038554906571,
2.32202991350013));
#103847=CARTESIAN_POINT('Ctrl Pts',(-10.0784883483419,23.5069180100853,
2.32409767893046));
#103848=CARTESIAN_POINT('Ctrl Pts',(-10.1271285556948,23.5103134273303,
2.32911421347605));
#103849=CARTESIAN_POINT('Ctrl Pts',(-10.1334249632994,23.5107508777757,
2.32981498112066));
#103850=CARTESIAN_POINT('Ctrl Pts',(-10.1430428503261,23.5114155996187,
2.33096405778238));
#103851=CARTESIAN_POINT('Ctrl Pts',(-10.1463684582694,23.5116448029577,
2.33137578051879));
#103852=CARTESIAN_POINT('Ctrl Pts',(-10.1524574703399,23.5120632344828,
2.33215602332165));
#103853=CARTESIAN_POINT('Ctrl Pts',(-10.1552213248156,23.512252694493,2.33252016085938));
#103854=CARTESIAN_POINT('Ctrl Pts',(-10.1614409551899,23.5126780013161,
2.33336207403037));
#103855=CARTESIAN_POINT('Ctrl Pts',(-10.1648959143414,23.5129135368851,
2.33384539166219));
#103856=CARTESIAN_POINT('Ctrl Pts',(-10.1737765937301,23.5135172285843,
2.33512797518922));
#103857=CARTESIAN_POINT('Ctrl Pts',(-10.1791990445895,23.5138841708593,
2.33594981035684));
#103858=CARTESIAN_POINT('Ctrl Pts',(-10.2134500495516,23.51619255771,2.34138595588647));
#103859=CARTESIAN_POINT('Ctrl Pts',(-10.2421070925027,23.5180817877162,
2.3470334315056));
#103860=CARTESIAN_POINT('Ctrl Pts',(-10.3663252610318,23.5262019958568,
2.37635000323533));
#103861=CARTESIAN_POINT('Ctrl Pts',(-10.4589145078455,23.532105600726,2.41087947671889));
#103862=CARTESIAN_POINT('Ctrl Pts',(-10.5819091289109,23.5408809782114,
2.47525255903733));
#103863=CARTESIAN_POINT('Ctrl Pts',(-10.6166945891777,23.543476180306,2.49580241408152));
#103864=CARTESIAN_POINT('Ctrl Pts',(-10.6583043722647,23.5467645636923,
2.52336221615197));
#103865=CARTESIAN_POINT('Ctrl Pts',(-10.6661906113755,23.547396319413,2.52872451494545));
#103866=CARTESIAN_POINT('Ctrl Pts',(-10.6786222594177,23.5484063085265,
2.53740012702518));
#103867=CARTESIAN_POINT('Ctrl Pts',(-10.6832106654075,23.5487821972534,
2.54065132968317));
#103868=CARTESIAN_POINT('Ctrl Pts',(-10.6918241198066,23.5494938198819,
2.54684769150019));
#103869=CARTESIAN_POINT('Ctrl Pts',(-10.6958540994004,23.5498292794069,
2.54978580994863));
#103870=CARTESIAN_POINT('Ctrl Pts',(-10.7049169270239,23.5505894517735,
2.55648177619441));
#103871=CARTESIAN_POINT('Ctrl Pts',(-10.7099385858221,23.5510147311593,
2.56025444168942));
#103872=CARTESIAN_POINT('Ctrl Pts',(-10.7227857101931,23.5521134241664,
2.57006795574444));
#103873=CARTESIAN_POINT('Ctrl Pts',(-10.7305655930084,23.5527891116465,
2.5761673886878));
#103874=CARTESIAN_POINT('Ctrl Pts',(-10.7915963671532,23.5581737158395,
2.62526859577035));
#103875=CARTESIAN_POINT('Ctrl Pts',(-10.8410740402208,23.5630643210913,
2.6727326305068));
#103876=CARTESIAN_POINT('Ctrl Pts',(-10.9319287784207,23.5731260847822,
2.77651193159085));
#103877=CARTESIAN_POINT('Ctrl Pts',(-10.9729931741445,23.5782801102099,
2.83275892035766));
#103878=CARTESIAN_POINT('Ctrl Pts',(-11.0233236648928,23.5853049567174,
2.9163136988242));
#103879=CARTESIAN_POINT('Ctrl Pts',(-11.0369286076875,23.5872963252596,
2.94083957700686));
#103880=CARTESIAN_POINT('Ctrl Pts',(-11.052252950371,23.5896382580722,2.97095196663099));
#103881=CARTESIAN_POINT('Ctrl Pts',(-11.0548221551108,23.5900345765803,
2.97609321664473));
#103882=CARTESIAN_POINT('Ctrl Pts',(-11.0587742187887,23.5906498088235,
2.98414864770004));
#103883=CARTESIAN_POINT('Ctrl Pts',(-11.0601828736926,23.5908702450764,
2.98704996441718));
#103884=CARTESIAN_POINT('Ctrl Pts',(-11.0627924028258,23.5912807113445,
2.99248131694517));
#103885=CARTESIAN_POINT('Ctrl Pts',(-11.0639961624295,23.591470908929,2.99500983007957));
#103886=CARTESIAN_POINT('Ctrl Pts',(-11.0667257632721,23.5919041844397,
3.00079648307236));
#103887=CARTESIAN_POINT('Ctrl Pts',(-11.0682457040757,23.5921469018397,
3.00405734008063));
#103888=CARTESIAN_POINT('Ctrl Pts',(-11.072250972955,23.5927905403267,3.01275402783155));
#103889=CARTESIAN_POINT('Ctrl Pts',(-11.074709943605,23.5931899255471,3.01820198506493));
#103890=CARTESIAN_POINT('Ctrl Pts',(-11.0940369721877,23.5963652920292,
3.06190615923066));
#103891=CARTESIAN_POINT('Ctrl Pts',(-11.1089005251343,23.5990335542725,
3.10102183620292));
#103892=CARTESIAN_POINT('Ctrl Pts',(-11.1518154039672,23.6078642520082,
3.23504819676));
#103893=CARTESIAN_POINT('Ctrl Pts',(-11.1699908605694,23.6138214759154,
3.33266765648044));
#103894=CARTESIAN_POINT('Ctrl Pts',(-11.1774012379728,23.6219692105759,
3.4596983953908));
#103895=CARTESIAN_POINT('Ctrl Pts',(-11.1780299134458,23.6238085269764,
3.48803290434519));
#103896=CARTESIAN_POINT('Ctrl Pts',(-11.1775178892408,23.6262425554278,
3.52488791624394));
#103897=CARTESIAN_POINT('Ctrl Pts',(-11.177306813993,23.626808469969,3.53341327921837));
#103898=CARTESIAN_POINT('Ctrl Pts',(-11.1768108034502,23.6277376062525,
3.54733482924011));
#103899=CARTESIAN_POINT('Ctrl Pts',(-11.1765812788508,23.6280991038632,
3.5527327770721));
#103900=CARTESIAN_POINT('Ctrl Pts',(-11.1760656664596,23.6288003423067,
3.56316687467385));
#103901=CARTESIAN_POINT('Ctrl Pts',(-11.1757843487723,23.629139927392,3.56820315020917));
#103902=CARTESIAN_POINT('Ctrl Pts',(-11.1750599709616,23.6299265175479,
3.57982951770778));
#103903=CARTESIAN_POINT('Ctrl Pts',(-11.1745938116968,23.6303742308522,
3.58641794771668));
#103904=CARTESIAN_POINT('Ctrl Pts',(-11.1729044815384,23.6318300295772,
3.60774432600491));
#103905=CARTESIAN_POINT('Ctrl Pts',(-11.1714591777559,23.6328449560789,
3.62246274043899));
#103906=CARTESIAN_POINT('Ctrl Pts',(-11.1595324485788,23.6399332840094,
3.72418488387559));
#103907=CARTESIAN_POINT('Ctrl Pts',(-11.1396476297149,23.6463052383613,
3.80979353133322));
#103908=CARTESIAN_POINT('Ctrl Pts',(-11.0871584061359,23.657873777436,3.95833846699633));
#103909=CARTESIAN_POINT('Ctrl Pts',(-11.0580231272876,23.6630166067964,
4.02208885143681));
#103910=CARTESIAN_POINT('Ctrl Pts',(-11.0198284152148,23.6683887776524,
4.08914946789466));
#103911=CARTESIAN_POINT('Ctrl Pts',(-11.0162009289422,23.6688877940868,
4.0953845568575));
#103912=CARTESIAN_POINT('Ctrl Pts',(-11.0107131638716,23.669625865636,4.10462089274858));
#103913=CARTESIAN_POINT('Ctrl Pts',(-11.0088963883889,23.6698675429621,
4.10764759679456));
#103914=CARTESIAN_POINT('Ctrl Pts',(-11.0057581540402,23.6702804071296,
4.11282294373398));
#103915=CARTESIAN_POINT('Ctrl Pts',(-11.0044433745845,23.6704520164085,
4.11497555437633));
#103916=CARTESIAN_POINT('Ctrl Pts',(-11.0014408134876,23.6708408325963,
4.11985615227144));
#103917=CARTESIAN_POINT('Ctrl Pts',(-10.999748796384,23.6710577606218,4.12258147834475));
#103918=CARTESIAN_POINT('Ctrl Pts',(-10.9951141837021,23.6716461548264,
4.12997881679343));
#103919=CARTESIAN_POINT('Ctrl Pts',(-10.9921497894248,23.6720162369256,
4.13463717707898));
#103920=CARTESIAN_POINT('Ctrl Pts',(-10.9772548048278,23.6738458679861,
4.15768425749344));
#103921=CARTESIAN_POINT('Ctrl Pts',(-10.9648443727188,23.6752765654319,
4.17575958856746));
#103922=CARTESIAN_POINT('Ctrl Pts',(-10.9389425843052,23.6781049348365,
4.21131484808431));
#103923=CARTESIAN_POINT('Ctrl Pts',(-10.9254501415301,23.6795017579289,
4.22878263044846));
#103924=CARTESIAN_POINT('Ctrl Pts',(-10.8484566912129,23.6871280880367,
4.32287183720304));
#103925=CARTESIAN_POINT('Ctrl Pts',(-10.7759365424521,23.693121303182,4.39158274027145));
#103926=CARTESIAN_POINT('Ctrl Pts',(-10.6734298073257,23.7012633380182,
4.46661517569012));
#103927=CARTESIAN_POINT('Ctrl Pts',(-10.6506588927732,23.703051283036,4.48208727642169));
#103928=CARTESIAN_POINT('Ctrl Pts',(-10.6202228946633,23.7054266472887,
4.50124417974429));
#103929=CARTESIAN_POINT('Ctrl Pts',(-10.6130294778427,23.7059870125333,
4.50566455623247));
#103930=CARTESIAN_POINT('Ctrl Pts',(-10.6011718177693,23.7069093484708,
4.51277662860465));
#103931=CARTESIAN_POINT('Ctrl Pts',(-10.5965354547339,23.7072696438798,
4.51551440341017));
#103932=CARTESIAN_POINT('Ctrl Pts',(-10.5875131972473,23.707970201043,4.52075894522764));
#103933=CARTESIAN_POINT('Ctrl Pts',(-10.5831296196806,23.7083103178941,
4.52326947891647));
#103934=CARTESIAN_POINT('Ctrl Pts',(-10.5729377798476,23.709100570855,4.52901972464193));
#103935=CARTESIAN_POINT('Ctrl Pts',(-10.5671180032987,23.709551436055,4.53223856760855));
#103936=CARTESIAN_POINT('Ctrl Pts',(-10.5480419593723,23.7110282242833,
4.5425792628818));
#103937=CARTESIAN_POINT('Ctrl Pts',(-10.5346768741699,23.712061266526,4.54949612307497));
#103938=CARTESIAN_POINT('Ctrl Pts',(-10.4486770725449,23.7187013132352,
4.59193467093531));
#103939=CARTESIAN_POINT('Ctrl Pts',(-10.3726920097259,23.7245578603293,
4.62014669435456));
#103940=CARTESIAN_POINT('Ctrl Pts',(-10.2263599942347,23.7356484619345,
4.65792873298871));
#103941=CARTESIAN_POINT('Ctrl Pts',(-10.1568452198501,23.7408363276891,
4.66937548710646));
#103942=CARTESIAN_POINT('Ctrl Pts',(-10.0753228561955,23.7465822273821,
4.67539445579665));
#103943=CARTESIAN_POINT('Ctrl Pts',(-10.0639137914941,23.7473785104806,
4.67607002815331));
#103944=CARTESIAN_POINT('Ctrl Pts',(-10.0482573202014,23.7484588842655,
4.6767685827087));
#103945=CARTESIAN_POINT('Ctrl Pts',(-10.044017386127,23.7487502195074,4.67693480589384));
#103946=CARTESIAN_POINT('Ctrl Pts',(-10.0368818352359,23.7492383287049,
4.6771759349204));
#103947=CARTESIAN_POINT('Ctrl Pts',(-10.0339867027271,23.7494357644113,
4.67726307858167));
#103948=CARTESIAN_POINT('Ctrl Pts',(-10.0284681619974,23.749810913207,4.67740881239099));
#103949=CARTESIAN_POINT('Ctrl Pts',(-10.0258448446948,23.7499887343987,
4.6774693168365));
#103950=CARTESIAN_POINT('Ctrl Pts',(-10.0195999155633,23.7504108760665,
4.67759247001611));
#103951=CARTESIAN_POINT('Ctrl Pts',(-10.0159781468086,23.7506547621857,
4.6776471805346));
#103952=CARTESIAN_POINT('Ctrl Pts',(-10.0031271562201,23.7515169953,4.67778201149794));
#103953=CARTESIAN_POINT('Ctrl Pts',(-9.99389701604686,23.7521305450048,
4.67777035635863));
#103954=CARTESIAN_POINT('Ctrl Pts',(-9.90687749016525,23.7578688342754,
4.67663740819367));
#103955=CARTESIAN_POINT('Ctrl Pts',(-9.82936708318603,23.7626408666315,
4.66791926106481));
#103956=CARTESIAN_POINT('Ctrl Pts',(-9.67322522867196,23.7725136538506,
4.63446693743941));
#103957=CARTESIAN_POINT('Ctrl Pts',(-9.59519432679469,23.7775998045525,
4.60902066409386));
#103958=CARTESIAN_POINT('Ctrl Pts',(-9.51007537320035,23.783717745883,4.57107311953033));
#103959=CARTESIAN_POINT('Ctrl Pts',(-9.49978123401993,23.7844672664242,
4.56630433684951));
#103960=CARTESIAN_POINT('Ctrl Pts',(-9.48414156363063,23.785621604239,4.55878291335345));
#103961=CARTESIAN_POINT('Ctrl Pts',(-9.47874535580714,23.7860227708797,
4.5561367229787));
#103962=CARTESIAN_POINT('Ctrl Pts',(-9.46896687076106,23.7867551038512,
4.55124835685043));
#103963=CARTESIAN_POINT('Ctrl Pts',(-9.46457792052002,23.7870857929138,
4.54901977468096));
#103964=CARTESIAN_POINT('Ctrl Pts',(-9.45504217813098,23.7878086913508,
4.54410236727641));
#103965=CARTESIAN_POINT('Ctrl Pts',(-9.44990106511162,23.7882012672329,
4.54140287147131));
#103966=CARTESIAN_POINT('Ctrl Pts',(-9.43586951722983,23.7892806263323,
4.53390229203741));
#103967=CARTESIAN_POINT('Ctrl Pts',(-9.42702074589338,23.7899700846695,
4.52902473942494));
#103968=CARTESIAN_POINT('Ctrl Pts',(-9.37908291821461,23.793754401468,4.50179078274726));
#103969=CARTESIAN_POINT('Ctrl Pts',(-9.34124265455703,23.7969241584934,
4.47732320150947));
#103970=CARTESIAN_POINT('Ctrl Pts',(-9.23816336621629,23.8060923969847,
4.40196136775153));
#103971=CARTESIAN_POINT('Ctrl Pts',(-9.17675224219001,23.81223090797,4.34628039263864));
#103972=CARTESIAN_POINT('Ctrl Pts',(-9.09584475789561,23.8210602396578,
4.25571334230284));
#103973=CARTESIAN_POINT('Ctrl Pts',(-9.0714468650037,23.8238425884907,4.22552678071012));
#103974=CARTESIAN_POINT('Ctrl Pts',(-9.04491545927201,23.8269671319655,
4.18916417264557));
#103975=CARTESIAN_POINT('Ctrl Pts',(-9.04128968936591,23.827396450313,4.18411130770517));
#103976=CARTESIAN_POINT('Ctrl Pts',(-9.03578616780716,23.8280514172476,
4.17631192022765));
#103977=CARTESIAN_POINT('Ctrl Pts',(-9.03387981337412,23.8282789135404,
4.17358586187757));
#103978=CARTESIAN_POINT('Ctrl Pts',(-9.03039630128335,23.8286957204143,
4.168559278751));
#103979=CARTESIAN_POINT('Ctrl Pts',(-9.02881576758655,23.8288852505089,
4.16626123165446));
#103980=CARTESIAN_POINT('Ctrl Pts',(-9.02526022860582,23.8293125788578,
4.16105205170739));
#103981=CARTESIAN_POINT('Ctrl Pts',(-9.02329009378911,23.8295500519712,
4.15813767322915));
#103982=CARTESIAN_POINT('Ctrl Pts',(-9.01822845273933,23.8301620811689,
4.15057730748148));
#103983=CARTESIAN_POINT('Ctrl Pts',(-9.01515681301003,23.8305353664732,
4.14591803201631));
#103984=CARTESIAN_POINT('Ctrl Pts',(-8.99514757186776,23.8329807594324,
4.11509204584473));
#103985=CARTESIAN_POINT('Ctrl Pts',(-8.97921967928989,23.83499326539,4.08828101444889));
#103986=CARTESIAN_POINT('Ctrl Pts',(-8.91838477902032,23.8431004152923,
3.97595087849477));
#103987=CARTESIAN_POINT('Ctrl Pts',(-8.88301341057005,23.8489002221996,
3.88569912404111));
#103988=CARTESIAN_POINT('Ctrl Pts',(-8.84910802691948,23.8575430177518,
3.75328139299766));
#103989=CARTESIAN_POINT('Ctrl Pts',(-8.8411514169592,23.8601214088915,3.71394678024683));
#103990=CARTESIAN_POINT('Ctrl Pts',(-8.83380844873831,23.8633909176912,
3.66487245297488));
#103991=CARTESIAN_POINT('Ctrl Pts',(-8.83251411780653,23.8640214844554,
3.6554424848073));
#103992=CARTESIAN_POINT('Ctrl Pts',(-8.8306376344257,23.86503001508,3.64042186449809));
#103993=CARTESIAN_POINT('Ctrl Pts',(-8.82998094201227,23.8654056462074,
3.63484081035416));
#103994=CARTESIAN_POINT('Ctrl Pts',(-8.82881680387449,23.8661170593123,
3.62429748091954));
#103995=CARTESIAN_POINT('Ctrl Pts',(-8.82830089151082,23.8664525689335,
3.61933624972127));
#103996=CARTESIAN_POINT('Ctrl Pts',(-8.82720594563834,23.8672132328656,
3.608114290138));
#103997=CARTESIAN_POINT('Ctrl Pts',(-8.82664550426155,23.867638956637,3.60185194325914));
#103998=CARTESIAN_POINT('Ctrl Pts',(-8.82533119818919,23.8687395560514,
3.58571123814033));
#103999=CARTESIAN_POINT('Ctrl Pts',(-8.82465179942531,23.8694167187662,
3.57582748346809));
#104000=CARTESIAN_POINT('Ctrl Pts',(-8.82006612960381,23.8750475378317,
3.49404736808586));
#104001=CARTESIAN_POINT('Ctrl Pts',(-8.82263657538866,23.880203516386,3.42195330452403));
#104002=CARTESIAN_POINT('Ctrl Pts',(-8.84021428314793,23.8903249666973,
3.28454439463232));
#104003=CARTESIAN_POINT('Ctrl Pts',(-8.85423871760985,23.8952546929784,
3.21936607815493));
#104004=CARTESIAN_POINT('Ctrl Pts',(-8.88171902826667,23.9020207411904,
3.12946455934411));
#104005=CARTESIAN_POINT('Ctrl Pts',(-8.89066111072591,23.9039698103572,
3.10349482708682));
#104006=CARTESIAN_POINT('Ctrl Pts',(-8.90255182315797,23.9062690118763,
3.07252460352686));
#104007=CARTESIAN_POINT('Ctrl Pts',(-8.90463883975899,23.9066630258453,
3.0672048435975));
#104008=CARTESIAN_POINT('Ctrl Pts',(-8.90796156923046,23.9072754756593,
3.05891329241829));
#104009=CARTESIAN_POINT('Ctrl Pts',(-8.90917084888182,23.9074954122955,
3.05593110716472));
#104010=CARTESIAN_POINT('Ctrl Pts',(-8.91145580316724,23.9079054561983,
3.05036187505279));
#104011=CARTESIAN_POINT('Ctrl Pts',(-8.91252847711631,23.9080957272876,
3.04777373030479));
#104012=CARTESIAN_POINT('Ctrl Pts',(-8.91500393915851,23.9085298093984,
3.04186068449079));
#104013=CARTESIAN_POINT('Ctrl Pts',(-8.91641278129487,23.9087732548243,
3.03853838210982));
#104014=CARTESIAN_POINT('Ctrl Pts',(-8.92021049494198,23.9094201307703,
3.02969598751237));
#104015=CARTESIAN_POINT('Ctrl Pts',(-8.92262645785426,23.9098220007971,
3.02418754342833));
#104016=CARTESIAN_POINT('Ctrl Pts',(-8.94389196619759,23.9132793238638,
2.97669426681406));
#104017=CARTESIAN_POINT('Ctrl Pts',(-8.96514769616483,23.91620383488,2.93582373661358));
#104018=CARTESIAN_POINT('Ctrl Pts',(-9.04679997268813,23.9261652960619,
2.79904875727945));
#104019=CARTESIAN_POINT('Ctrl Pts',(-9.11857375832019,23.9329792984337,
2.71069002717898));
#104020=CARTESIAN_POINT('Ctrl Pts',(-9.21235095020103,23.9413073693433,
2.62426737635624));
#104021=CARTESIAN_POINT('Ctrl Pts',(-9.22301784118901,23.9422465285172,
2.61478965782006));
#104022=CARTESIAN_POINT('Ctrl Pts',(-9.23879946104927,23.9436259298127,
2.60127245310413));
#104023=CARTESIAN_POINT('Ctrl Pts',(-9.24377996373205,23.9440598305615,
2.59707767890721));
#104024=CARTESIAN_POINT('Ctrl Pts',(-9.25266851812704,23.9448318456982,
2.58971651964758));
#104025=CARTESIAN_POINT('Ctrl Pts',(-9.25656258072849,23.9451692770237,
2.58653343756683));
#104026=CARTESIAN_POINT('Ctrl Pts',(-9.26471310577264,23.9458739828845,
2.57995767895249));
#104027=CARTESIAN_POINT('Ctrl Pts',(-9.26897293000333,23.9462414205239,
2.57656937967643));
#104028=CARTESIAN_POINT('Ctrl Pts',(-9.28011209737974,23.9472000875652,
2.56783457507285));
#104029=CARTESIAN_POINT('Ctrl Pts',(-9.28702744792748,23.947793127955,2.56253474482892));
#104030=CARTESIAN_POINT('Ctrl Pts',(-9.31816369053002,23.9504544824182,
2.53921614096332));
#104031=CARTESIAN_POINT('Ctrl Pts',(-9.34301129544578,23.9525552717841,
2.52205729629554));
#104032=CARTESIAN_POINT('Ctrl Pts',(-9.45090600407031,23.9615896100804,
2.45351803230599));
#104033=CARTESIAN_POINT('Ctrl Pts',(-9.53950756581154,23.9688387292814,
2.41162038657657));
#104034=CARTESIAN_POINT('Ctrl Pts',(-9.67111414646436,23.9789284319097,
2.36836242325051));
#104035=CARTESIAN_POINT('Ctrl Pts',(-9.71063223727229,23.9818710067288,
2.35761802839803));
#104036=CARTESIAN_POINT('Ctrl Pts',(-9.75644342183527,23.9851283194583,
2.34769335938745));
#104037=CARTESIAN_POINT('Ctrl Pts',(-9.76226284372576,23.9855392802199,
2.34647867424707));
#104038=CARTESIAN_POINT('Ctrl Pts',(-9.77160924513654,23.9861945355241,
2.3446015404726));
#104039=CARTESIAN_POINT('Ctrl Pts',(-9.77513039715869,23.9864403121219,
2.34391107618617));
#104040=CARTESIAN_POINT('Ctrl Pts',(-9.78140418235259,23.986876229845,2.34271059479256));
#104041=CARTESIAN_POINT('Ctrl Pts',(-9.7841555412148,23.9870667169374,2.34219428696871));
#104042=CARTESIAN_POINT('Ctrl Pts',(-9.79008677168292,23.9874758726541,
2.3411031364476));
#104043=CARTESIAN_POINT('Ctrl Pts',(-9.79326717875975,23.9876943573053,
2.34053156790238));
#104044=CARTESIAN_POINT('Ctrl Pts',(-9.80132929731045,23.9882459899798,
2.33911690704655));
#104045=CARTESIAN_POINT('Ctrl Pts',(-9.80621410020899,23.9885781716899,
2.33829150358947));
#104046=CARTESIAN_POINT('Ctrl Pts',(-9.8111040637107,23.9889087884094,2.3374969300026));
#104047=CARTESIAN_POINT('Origin',(-10.,12.3756328852638,3.5));
#104048=CARTESIAN_POINT('',(-9.81111852688625,24.5869833862071,2.3377666957199));
#104049=CARTESIAN_POINT('',(-9.81110406371068,24.4872084044306,2.3374969300026));
#104050=CARTESIAN_POINT('',(-9.81110406371068,12.3756328852638,2.3374969300026));
#104051=CARTESIAN_POINT('Ctrl Pts',(-9.81106550641579,24.5871379729677,
2.3375031958607));
#104052=CARTESIAN_POINT('Ctrl Pts',(-9.778173526296,24.5850437659178,2.3428489564553));
#104053=CARTESIAN_POINT('Ctrl Pts',(-9.74552537487917,24.5829249747512,
2.34958792665165));
#104054=CARTESIAN_POINT('Ctrl Pts',(-9.69640028524721,24.5796436570711,
2.36192153158769));
#104055=CARTESIAN_POINT('Ctrl Pts',(-9.67968798209671,24.578510716744,2.36651177816805));
#104056=CARTESIAN_POINT('Ctrl Pts',(-9.65696427979307,24.576944422228,2.37329580545251));
#104057=CARTESIAN_POINT('Ctrl Pts',(-9.65085992780051,24.5765210873338,
2.37517243335176));
#104058=CARTESIAN_POINT('Ctrl Pts',(-9.64008411827752,24.5757690635254,
2.37858135013507));
#104059=CARTESIAN_POINT('Ctrl Pts',(-9.6354063896023,24.5754410275816,2.38009342880476));
#104060=CARTESIAN_POINT('Ctrl Pts',(-9.62616119321268,24.5747894698107,
2.38314600635575));
#104061=CARTESIAN_POINT('Ctrl Pts',(-9.62159344271248,24.5744659908854,
2.38468534807298));
#104062=CARTESIAN_POINT('Ctrl Pts',(-9.61187893550175,24.5737746212577,
2.38802570450796));
#104063=CARTESIAN_POINT('Ctrl Pts',(-9.60673499493011,24.5734064826443,
2.38983450395624));
#104064=CARTESIAN_POINT('Ctrl Pts',(-9.59344754898872,24.5724501115701,
2.39461079770613));
#104065=CARTESIAN_POINT('Ctrl Pts',(-9.58532403193604,24.5718601108319,
2.39763253925453));
#104066=CARTESIAN_POINT('Ctrl Pts',(-9.55243902486903,24.5694495494772,
2.41027984960885));
#104067=CARTESIAN_POINT('Ctrl Pts',(-9.52797490025081,24.5676045735673,
2.42065161258633));
#104068=CARTESIAN_POINT('Ctrl Pts',(-9.47288282225408,24.5633266875081,
2.4462396207243));
#104069=CARTESIAN_POINT('Ctrl Pts',(-9.44252575845392,24.5608786715716,
2.46197997257215));
#104070=CARTESIAN_POINT('Ctrl Pts',(-9.35966027936587,24.553950521184,2.50963058102462));
#104071=CARTESIAN_POINT('Ctrl Pts',(-9.30889970784357,24.5494111218619,
2.54436077492083));
#104072=CARTESIAN_POINT('Ctrl Pts',(-9.22869765334448,24.5418804429928,
2.60897964518787));
#104073=CARTESIAN_POINT('Ctrl Pts',(-9.19771488896222,24.5388692792818,
2.63677125413567));
#104074=CARTESIAN_POINT('Ctrl Pts',(-9.16068629150373,24.5351978929914,
2.67370577889197));
#104075=CARTESIAN_POINT('Ctrl Pts',(-9.15321076810281,24.5344527322241,
2.6813684234149));
#104076=CARTESIAN_POINT('Ctrl Pts',(-9.1429902628072,24.5334296931726,2.69213459637554));
#104077=CARTESIAN_POINT('Ctrl Pts',(-9.14015588710096,24.5331455160698,
2.69515200016651));
#104078=CARTESIAN_POINT('Ctrl Pts',(-9.13537820777708,24.5326658032224,
2.70029224045094));
#104079=CARTESIAN_POINT('Ctrl Pts',(-9.13342669187868,24.5324696570292,
2.70240734305236));
#104080=CARTESIAN_POINT('Ctrl Pts',(-9.12970488291039,24.5320952308081,
2.70647091939302));
#104081=CARTESIAN_POINT('Ctrl Pts',(-9.12793333795856,24.531916854214,2.70841821022375));
#104082=CARTESIAN_POINT('Ctrl Pts',(-9.1236959602389,24.5314897758885,2.713107446587));
#104083=CARTESIAN_POINT('Ctrl Pts',(-9.12123642734107,24.5312415412185,
2.71585508673062));
#104084=CARTESIAN_POINT('Ctrl Pts',(-9.11232467045768,24.5303406457329,
2.72590534856023));
#104085=CARTESIAN_POINT('Ctrl Pts',(-9.10595001833896,24.5296934264287,
2.73327666940665));
#104086=CARTESIAN_POINT('Ctrl Pts',(-9.06068387280957,24.5250697928318,
2.78695244278102));
#104087=CARTESIAN_POINT('Ctrl Pts',(-9.02531292741572,24.5213037480345,
2.83611848664304));
#104088=CARTESIAN_POINT('Ctrl Pts',(-8.96681235378847,24.5143387984332,
2.9322604603614));
#104089=CARTESIAN_POINT('Ctrl Pts',(-8.9427314072081,24.5111414827707,2.97847547796598));
#104090=CARTESIAN_POINT('Ctrl Pts',(-8.90881892498954,24.5058541984097,
3.05563777050059));
#104091=CARTESIAN_POINT('Ctrl Pts',(-8.89706814976645,24.5038092040746,
3.08566315361815));
#104092=CARTESIAN_POINT('Ctrl Pts',(-8.881940128703,24.500810441796,3.12954292168344));
#104093=CARTESIAN_POINT('Ctrl Pts',(-8.87755909375188,24.4998869983706,
3.14303682556338));
#104094=CARTESIAN_POINT('Ctrl Pts',(-8.87016269936401,24.4982219540112,
3.16730227886122));
#104095=CARTESIAN_POINT('Ctrl Pts',(-8.86705498124146,24.4974833440926,
3.17804399389608));
#104096=CARTESIAN_POINT('Ctrl Pts',(-8.86253687891457,24.4963461876596,
3.1945368323374));
#104097=CARTESIAN_POINT('Ctrl Pts',(-8.86101607572831,24.4959512104584,
3.20025724912627));
#104098=CARTESIAN_POINT('Ctrl Pts',(-8.85952930082603,24.495552378179,3.20602440887385));
#104099=CARTESIAN_POINT('Ctrl Pts',(-8.85952012227789,24.495549915502,3.20606001911393));
#104100=CARTESIAN_POINT('Ctrl Pts',(-8.85950107683156,24.495544804418,3.2061339245243));
#104101=CARTESIAN_POINT('Ctrl Pts',(-8.85949121019862,24.4955421560037,
3.20617221974486));
#104102=CARTESIAN_POINT('Ctrl Pts',(-8.85947073554607,24.4955366589677,
3.20625170428873));
#104103=CARTESIAN_POINT('Ctrl Pts',(-8.85946012782387,24.4955338103348,
3.20629289370946));
#104104=CARTESIAN_POINT('Ctrl Pts',(-8.85943811365089,24.4955278971827,
3.20637839316351));
#104105=CARTESIAN_POINT('Ctrl Pts',(-8.85942670755547,24.4955248326535,
3.20642270326927));
#104106=CARTESIAN_POINT('Ctrl Pts',(-8.8594030346878,24.49551847074,3.20651468921928));
#104107=CARTESIAN_POINT('Ctrl Pts',(-8.85939076831832,24.4955151733415,
3.20656236518473));
#104108=CARTESIAN_POINT('Ctrl Pts',(-8.85936530789049,24.4955083272984,
3.20666134850182));
#104109=CARTESIAN_POINT('Ctrl Pts',(-8.85935211431048,24.4955047786402,
3.2067126559523));
#104110=CARTESIAN_POINT('Ctrl Pts',(-8.85932472701947,24.4954974101549,
3.206819189983));
#104111=CARTESIAN_POINT('Ctrl Pts',(-8.85931053385455,24.4954935903094,
3.20687441671485));
#104112=CARTESIAN_POINT('Ctrl Pts',(-8.8592810689919,24.49548565784,3.20698910138323));
#104113=CARTESIAN_POINT('Ctrl Pts',(-8.85926579793959,24.4954815451975,
3.20704855945387));
#104114=CARTESIAN_POINT('Ctrl Pts',(-8.85923409251358,24.4954730037076,
3.20717204507373));
#104115=CARTESIAN_POINT('Ctrl Pts',(-8.85921765887455,24.4954685748343,
3.20723607284032));
#104116=CARTESIAN_POINT('Ctrl Pts',(-8.85918353647414,24.4954593754534,
3.2073690650028));
#104117=CARTESIAN_POINT('Ctrl Pts',(-8.85916584858057,24.4954546049193,
3.20743802960041));
#104118=CARTESIAN_POINT('Ctrl Pts',(-8.85912911834146,24.4954446946245,
3.20758129374695));
#104119=CARTESIAN_POINT('Ctrl Pts',(-8.85911007699933,24.4954395548312,
3.20765559355693));
#104120=CARTESIAN_POINT('Ctrl Pts',(-8.85907053235528,24.495428876064,3.2078099604862));
#104121=CARTESIAN_POINT('Ctrl Pts',(-8.85905003021955,24.4954233370515,
3.20789002791908));
#104122=CARTESIAN_POINT('Ctrl Pts',(-8.85900744762761,24.4954118273193,
3.20805639951062));
#104123=CARTESIAN_POINT('Ctrl Pts',(-8.85898536853677,24.4954058565562,
3.20814270400968));
#104124=CARTESIAN_POINT('Ctrl Pts',(-8.85893950615215,24.49539344801,3.20832205927806));
#104125=CARTESIAN_POINT('Ctrl Pts',(-8.85891572444684,24.4953870101754,
3.20841511045768));
#104126=CARTESIAN_POINT('Ctrl Pts',(-8.8588663206733,24.495373629143,3.20860851225019));
#104127=CARTESIAN_POINT('Ctrl Pts',(-8.85884070046377,24.4953666858868,
3.20870886331933));
#104128=CARTESIAN_POINT('Ctrl Pts',(-8.85878747251416,24.4953522523952,
3.2089174651584));
#104129=CARTESIAN_POINT('Ctrl Pts',(-8.85875986694311,24.4953447620914,
3.20902571646158));
#104130=CARTESIAN_POINT('Ctrl Pts',(-8.85871160224477,24.4953316581035,
3.20921509210886));
#104131=CARTESIAN_POINT('Ctrl Pts',(-8.85869093635798,24.4953260446358,
3.20929621475369));
#104132=CARTESIAN_POINT('Ctrl Pts',(-8.85744766898421,24.4949881781523,
3.21417875902125));
#104133=CARTESIAN_POINT('Ctrl Pts',(-8.85625538587042,24.4946549557038,
3.21898778095268));
#104134=CARTESIAN_POINT('Ctrl Pts',(-8.85362777611421,24.4938991545359,
3.22987993290495));
#104135=CARTESIAN_POINT('Ctrl Pts',(-8.85221046756938,24.4934760076995,
3.23596721235092));
#104136=CARTESIAN_POINT('Ctrl Pts',(-8.84868319001925,24.492381542043,3.25168204862117));
#104137=CARTESIAN_POINT('Ctrl Pts',(-8.84664553828063,24.4917079410663,
3.26132516430873));
#104138=CARTESIAN_POINT('Ctrl Pts',(-8.83008356101068,24.4858530889064,
3.34487511716343));
#104139=CARTESIAN_POINT('Ctrl Pts',(-8.8225617934004,24.4804473462329,3.41997802999067));
#104140=CARTESIAN_POINT('Ctrl Pts',(-8.82204275818911,24.4709838669453,
3.54925293191191));
#104141=CARTESIAN_POINT('Ctrl Pts',(-8.82553758840936,24.4669933287691,
3.60318553001316));
#104142=CARTESIAN_POINT('Ctrl Pts',(-8.83761037549097,24.4604019906188,
3.69312403347695));
#104143=CARTESIAN_POINT('Ctrl Pts',(-8.84420510662729,24.4577684582247,
3.72931483947473));
#104144=CARTESIAN_POINT('Ctrl Pts',(-8.85385975541533,24.4547920040582,
3.77109960806783));
#104145=CARTESIAN_POINT('Ctrl Pts',(-8.85528285600135,24.4543698941246,
3.77704714773884));
#104146=CARTESIAN_POINT('Ctrl Pts',(-8.85754245877454,24.4537246759209,
3.78617589847587));
#104147=CARTESIAN_POINT('Ctrl Pts',(-8.85834604254963,24.4534997717774,
3.7893650298247));
#104148=CARTESIAN_POINT('Ctrl Pts',(-8.85985428385718,24.4530859739321,
3.79524659805779));
#104149=CARTESIAN_POINT('Ctrl Pts',(-8.86055512015956,24.4528968753134,
3.79793988269276));
#104150=CARTESIAN_POINT('Ctrl Pts',(-8.86216722315777,24.45246898817,3.80404623514055));
#104151=CARTESIAN_POINT('Ctrl Pts',(-8.86308430442793,24.4522305354783,
3.80745770951602));
#104152=CARTESIAN_POINT('Ctrl Pts',(-8.86550146617423,24.4516145638811,
3.81629065868477));
#104153=CARTESIAN_POINT('Ctrl Pts',(-8.86702508342782,24.4512383413307,
3.82170568153532));
#104154=CARTESIAN_POINT('Ctrl Pts',(-8.87743453692639,24.4487448876755,
3.85771007281686));
#104155=CARTESIAN_POINT('Ctrl Pts',(-8.88752031353462,24.4466898726167,
3.88794210014765));
#104156=CARTESIAN_POINT('Ctrl Pts',(-8.90988361725549,24.4426918637017,
3.94689396370194));
#104157=CARTESIAN_POINT('Ctrl Pts',(-8.92210130103532,24.4407489850332,
3.97560752330536));
#104158=CARTESIAN_POINT('Ctrl Pts',(-8.96534164812484,24.4344837771879,
4.06697596633123));
#104159=CARTESIAN_POINT('Ctrl Pts',(-9.00080025394839,24.4302040522692,
4.12735871889088));
#104160=CARTESIAN_POINT('Ctrl Pts',(-9.05506728485749,24.4242709184256,
4.2033850162583));
#104161=CARTESIAN_POINT('Ctrl Pts',(-9.06930227533093,24.422761251279,4.22211491838378));
#104162=CARTESIAN_POINT('Ctrl Pts',(-9.09461263305664,24.4201423493734,
4.25342488786535));
#104163=CARTESIAN_POINT('Ctrl Pts',(-9.10541341805402,24.4190434348606,
4.26621808095122));
#104164=CARTESIAN_POINT('Ctrl Pts',(-9.12112824306675,24.4174677930225,
4.28404646106886));
#104165=CARTESIAN_POINT('Ctrl Pts',(-9.12582067659058,24.4170001276418,
4.2892749363753));
#104166=CARTESIAN_POINT('Ctrl Pts',(-9.13400433839749,24.4161891490678,
4.29823095386762));
#104167=CARTESIAN_POINT('Ctrl Pts',(-9.13747359043889,24.4158467605432,
4.3019783868873));
#104168=CARTESIAN_POINT('Ctrl Pts',(-9.14417562802156,24.4151879279886,
4.30912403537428));
#104169=CARTESIAN_POINT('Ctrl Pts',(-9.14740456327196,24.4148716513653,
4.31252574141736));
#104170=CARTESIAN_POINT('Ctrl Pts',(-9.1550555144395,24.4141248407655,4.3204902507853));
#104171=CARTESIAN_POINT('Ctrl Pts',(-9.15949427059681,24.4136935910788,
4.3250366970065));
#104172=CARTESIAN_POINT('Ctrl Pts',(-9.17280307358579,24.4124063638712,
4.33844951855604));
#104173=CARTESIAN_POINT('Ctrl Pts',(-9.18177795118553,24.4115458360644,
4.34721013213532));
#104174=CARTESIAN_POINT('Ctrl Pts',(-9.26170169013972,24.4039450928261,
4.42277114416103));
#104175=CARTESIAN_POINT('Ctrl Pts',(-9.34053466081499,24.3968245810713,
4.48065739024635));
#104176=CARTESIAN_POINT('Ctrl Pts',(-9.47848218459731,24.3852336643963,
4.55772757507243));
#104177=CARTESIAN_POINT('Ctrl Pts',(-9.53360231003288,24.3808074611513,
4.58316358829024));
#104178=CARTESIAN_POINT('Ctrl Pts',(-9.59730119746411,24.3760775846879,
4.60678917022509));
#104179=CARTESIAN_POINT('Ctrl Pts',(-9.60418479230835,24.3755713750257,
4.6092695438965));
#104180=CARTESIAN_POINT('Ctrl Pts',(-9.61445181787299,24.3748241033848,
4.61286132882159));
#104181=CARTESIAN_POINT('Ctrl Pts',(-9.61781773621291,24.3745803499737,
4.61402174844764));
#104182=CARTESIAN_POINT('Ctrl Pts',(-9.62358785230638,24.3741646535518,
4.61598179935642));
#104183=CARTESIAN_POINT('Ctrl Pts',(-9.62598942904145,24.3739922780917,
4.61678895710871));
#104184=CARTESIAN_POINT('Ctrl Pts',(-9.63143555399285,24.3736028428096,
4.61859983362698));
#104185=CARTESIAN_POINT('Ctrl Pts',(-9.63448161013199,24.373386056207,4.61959887724968));
#104186=CARTESIAN_POINT('Ctrl Pts',(-9.64276246156687,24.3727993996682,
4.62227742854087));
#104187=CARTESIAN_POINT('Ctrl Pts',(-9.64800507924434,24.3724308948974,
4.62393276674868));
#104188=CARTESIAN_POINT('Ctrl Pts',(-9.67387049230317,24.3706262073116,
4.63190094452035));
#104189=CARTESIAN_POINT('Ctrl Pts',(-9.69465388351345,24.3692178779321,
4.63768365346537));
#104190=CARTESIAN_POINT('Ctrl Pts',(-9.73706102257202,24.3664063569308,
4.64823686467416));
#104191=CARTESIAN_POINT('Ctrl Pts',(-9.75868360882956,24.3650048173268,
4.65297497861202));
#104192=CARTESIAN_POINT('Ctrl Pts',(-9.87832533580387,24.357362894595,4.67567825337601));
#104193=CARTESIAN_POINT('Ctrl Pts',(-9.97818090239306,24.3513614706143,
4.68175654317401));
#104194=CARTESIAN_POINT('Ctrl Pts',(-10.1051429738336,24.3432064532232,
4.67337177083322));
#104195=CARTESIAN_POINT('Ctrl Pts',(-10.132600255881,24.3414141115809,4.67058674967412));
#104196=CARTESIAN_POINT('Ctrl Pts',(-10.1683087617237,24.3390334699319,
4.66569236838154));
#104197=CARTESIAN_POINT('Ctrl Pts',(-10.1766719156577,24.3384723469898,
4.6644541918869));
#104198=CARTESIAN_POINT('Ctrl Pts',(-10.190343552091,24.3375488883831,4.66227941686375));
#104199=CARTESIAN_POINT('Ctrl Pts',(-10.1956603155959,24.3371882323909,
4.66139620713384));
#104200=CARTESIAN_POINT('Ctrl Pts',(-10.2059518599833,24.3364870601956,
4.65961392255995));
#104201=CARTESIAN_POINT('Ctrl Pts',(-10.210927290817,24.3361466896402,4.65871924754895));
#104202=CARTESIAN_POINT('Ctrl Pts',(-10.2224375582474,24.3353559716996,
4.65657289657576));
#104203=CARTESIAN_POINT('Ctrl Pts',(-10.2289678023463,24.3349048954224,
4.65529782945498));
#104204=CARTESIAN_POINT('Ctrl Pts',(-10.2502297358889,24.3334279581042,
4.65095896885672));
#104205=CARTESIAN_POINT('Ctrl Pts',(-10.2649130588474,24.3323949828224,
4.64766828982858));
#104206=CARTESIAN_POINT('Ctrl Pts',(-10.3587882224366,24.3257038638226,
4.62473247398366));
#104207=CARTESIAN_POINT('Ctrl Pts',(-10.4358065826944,24.3197911702094,
4.59718737828363));
#104208=CARTESIAN_POINT('Ctrl Pts',(-10.5584952957335,24.3098035278222,
4.53833970052955));
#104209=CARTESIAN_POINT('Ctrl Pts',(-10.6059498155291,24.3057875353895,
4.51138109818273));
#104210=CARTESIAN_POINT('Ctrl Pts',(-10.6647965237534,24.3007230571944,
4.47231704075621));
#104211=CARTESIAN_POINT('Ctrl Pts',(-10.6780412340188,24.2995775363267,
4.46312770991178));
#104212=CARTESIAN_POINT('Ctrl Pts',(-10.6998105800994,24.2976902994671,
4.44735215117807));
#104213=CARTESIAN_POINT('Ctrl Pts',(-10.7084407374898,24.2969409341223,
4.44091587747201));
#104214=CARTESIAN_POINT('Ctrl Pts',(-10.7202705833178,24.2959134049267,
4.43183825534769));
#104215=CARTESIAN_POINT('Ctrl Pts',(-10.7235460771481,24.2956288631527,
4.42929721988055));
#104216=CARTESIAN_POINT('Ctrl Pts',(-10.7290720604629,24.2951488572233,
4.4249633889364));
#104217=CARTESIAN_POINT('Ctrl Pts',(-10.7313295018371,24.2949527786357,
4.42317956033893));
#104218=CARTESIAN_POINT('Ctrl Pts',(-10.7356480371724,24.2945777307675,
4.41974127489869));
#104219=CARTESIAN_POINT('Ctrl Pts',(-10.7377101217449,24.2943986680624,
4.41808813518947));
#104220=CARTESIAN_POINT('Ctrl Pts',(-10.7426440921362,24.2939702259037,
4.41410529468319));
#104221=CARTESIAN_POINT('Ctrl Pts',(-10.7455106271219,24.2937213122776,
4.4117689636762));
#104222=CARTESIAN_POINT('Ctrl Pts',(-10.7558922725725,24.2928196379011,
4.40322584877651));
#104223=CARTESIAN_POINT('Ctrl Pts',(-10.7633415182733,24.2921722834478,
4.39693913023562));
#104224=CARTESIAN_POINT('Ctrl Pts',(-10.8170872479234,24.2874916293172,
4.35042629776266));
#104225=CARTESIAN_POINT('Ctrl Pts',(-10.8602630555789,24.2836735960284,
4.30672544048429));
#104226=CARTESIAN_POINT('Ctrl Pts',(-10.9429776746966,24.2757374633022,
4.20877233243274));
#104227=CARTESIAN_POINT('Ctrl Pts',(-10.9816825631639,24.2716341345672,
4.15411301328122));
#104228=CARTESIAN_POINT('Ctrl Pts',(-11.0331112299902,24.265178722192,4.06655092375093));
#104229=CARTESIAN_POINT('Ctrl Pts',(-11.0493500838197,24.2629387020381,
4.03587573431201));
#104230=CARTESIAN_POINT('Ctrl Pts',(-11.0681129690451,24.260050307342,3.99629904144079));
#104231=CARTESIAN_POINT('Ctrl Pts',(-11.0719197916083,24.2594464064131,
3.98802254641771));
#104232=CARTESIAN_POINT('Ctrl Pts',(-11.0778816794069,24.258470794376,3.9746543011807));
#104233=CARTESIAN_POINT('Ctrl Pts',(-11.0800976217184,24.2581011590103,
3.96958997669834));
#104234=CARTESIAN_POINT('Ctrl Pts',(-11.0842505095648,24.25739475823,3.95991402722388));
#104235=CARTESIAN_POINT('Ctrl Pts',(-11.0861938946848,24.2570582195747,
3.95530528411999));
#104236=CARTESIAN_POINT('Ctrl Pts',(-11.0905708013905,24.2562863318043,
3.94473791837185));
#104237=CARTESIAN_POINT('Ctrl Pts',(-11.0929849340541,24.2558503434936,
3.93877148944935));
#104238=CARTESIAN_POINT('Ctrl Pts',(-11.1003103474507,24.2544948382353,
3.92023138508594));
#104239=CARTESIAN_POINT('Ctrl Pts',(-11.1050543047041,24.2535698120514,
3.90759322241757));
#104240=CARTESIAN_POINT('Ctrl Pts',(-11.1436710583243,24.2456157496913,
3.79908247855799));
#104241=CARTESIAN_POINT('Ctrl Pts',(-11.1652068601323,24.2381670520375,
3.69929427076204));
#104242=CARTESIAN_POINT('Ctrl Pts',(-11.1784864565149,24.2264595884829,
3.54027072943912));
#104243=CARTESIAN_POINT('Ctrl Pts',(-11.1790413562769,24.2222348213543,
3.4822477865585));
#104244=CARTESIAN_POINT('Ctrl Pts',(-11.174858617989,24.2176978845472,3.41720856954971));
#104245=CARTESIAN_POINT('Ctrl Pts',(-11.1743289768438,24.2171983687719,
3.41000747855053));
#104246=CARTESIAN_POINT('Ctrl Pts',(-11.1734418367923,24.2164598111208,
3.39929360219905));
#104247=CARTESIAN_POINT('Ctrl Pts',(-11.1731347264072,24.2162181376278,
3.39577698232172));
#104248=CARTESIAN_POINT('Ctrl Pts',(-11.1725811076617,24.2158053088983,
3.38975042692776));
#104249=CARTESIAN_POINT('Ctrl Pts',(-11.1723423443561,24.2156337310799,
3.38723985426329));
#104250=CARTESIAN_POINT('Ctrl Pts',(-11.1717815771572,24.215244960192,3.3815378271182));
#104251=CARTESIAN_POINT('Ctrl Pts',(-11.1714545989229,24.2150280461342,
3.37834691022124));
#104252=CARTESIAN_POINT('Ctrl Pts',(-11.1705298386934,24.2144399985982,
3.36967199072267));
#104253=CARTESIAN_POINT('Ctrl Pts',(-11.1699065480027,24.2140702453971,
3.3641907028999));
#104254=CARTESIAN_POINT('Ctrl Pts',(-11.1666246857412,24.212246184056,3.33703092392216));
#104255=CARTESIAN_POINT('Ctrl Pts',(-11.1634017743239,24.2108205077062,
3.31542335974056));
#104256=CARTESIAN_POINT('Ctrl Pts',(-11.1557157619461,24.2079959327418,
3.27217615644928));
#104257=CARTESIAN_POINT('Ctrl Pts',(-11.151241214385,24.2065980635236,3.25054782031563));
#104258=CARTESIAN_POINT('Ctrl Pts',(-11.1232762191888,24.1989722249328,
3.1322484195828));
#104259=CARTESIAN_POINT('Ctrl Pts',(-11.088220324039,24.1929809626272,3.03873249527051));
#104260=CARTESIAN_POINT('Ctrl Pts',(-11.028941951065,24.1848351983103,2.92629557063618));
#104261=CARTESIAN_POINT('Ctrl Pts',(-11.0152026045046,24.1830406777031,
2.90231965838381));
#104262=CARTESIAN_POINT('Ctrl Pts',(-10.9961731016209,24.1806575421282,
2.87166430001134));
#104263=CARTESIAN_POINT('Ctrl Pts',(-10.9916351406955,24.1800961895335,
2.86452667891526));
#104264=CARTESIAN_POINT('Ctrl Pts',(-10.9840798939414,24.1791724601592,
2.85292127145348));
#104265=CARTESIAN_POINT('Ctrl Pts',(-10.9811080588686,24.1788117655393,
2.84842414580067));
#104266=CARTESIAN_POINT('Ctrl Pts',(-10.9752897878399,24.1781105950015,
2.83974971178937));
#104267=CARTESIAN_POINT('Ctrl Pts',(-10.9724471191786,24.1777702652364,
2.83557000942539));
#104268=CARTESIAN_POINT('Ctrl Pts',(-10.9658018196126,24.1769797533639,
2.82593312819351));
#104269=CARTESIAN_POINT('Ctrl Pts',(-10.9619797204256,24.1765288433951,
2.82048964925511));
#104270=CARTESIAN_POINT('Ctrl Pts',(-10.9493682636117,24.1750529204122,
2.80284792968513));
#104271=CARTESIAN_POINT('Ctrl Pts',(-10.9403917085939,24.1740208074746,
2.79078599342776));
#104272=CARTESIAN_POINT('Ctrl Pts',(-10.8814272828743,24.1673529998721,
2.7146427605901));
#104273=CARTESIAN_POINT('Ctrl Pts',(-10.8251590871369,24.1614650438022,
2.65572043733789));
#104274=CARTESIAN_POINT('Ctrl Pts',(-10.721744802459,24.1515002652096,2.56771512893189));
#104275=CARTESIAN_POINT('Ctrl Pts',(-10.6777945409312,24.1474819509128,
2.53528979877945));
#104276=CARTESIAN_POINT('Ctrl Pts',(-10.6181464308509,24.1424147791954,
2.49737844406073));
#104277=CARTESIAN_POINT('Ctrl Pts',(-10.6043628919056,24.1412690152447,
2.48901011670976));
#104278=CARTESIAN_POINT('Ctrl Pts',(-10.5810937382364,24.1393813318692,
2.47552887568332));
#104279=CARTESIAN_POINT('Ctrl Pts',(-10.5717022884101,24.1386317721532,
2.47025851242008));
#104280=CARTESIAN_POINT('Ctrl Pts',(-10.5585945231385,24.1376038693147,
2.46313721822583));
#104281=CARTESIAN_POINT('Ctrl Pts',(-10.5549390746922,24.1373191535429,
2.4611761967489));
#104282=CARTESIAN_POINT('Ctrl Pts',(-10.5487286491935,24.1368388131403,
2.45788665499965));
#104283=CARTESIAN_POINT('Ctrl Pts',(-10.5461790436348,24.1366425742519,
2.45654812893116));
#104284=CARTESIAN_POINT('Ctrl Pts',(-10.541277090975,24.1362671492125,2.45399752607333));
#104285=CARTESIAN_POINT('Ctrl Pts',(-10.5389255431997,24.1360878699456,
2.45278401276746));
#104286=CARTESIAN_POINT('Ctrl Pts',(-10.5332729265085,24.135658833079,2.4498910696929));
#104287=CARTESIAN_POINT('Ctrl Pts',(-10.52996796064,24.1354095424291,2.44821925227834));
#104288=CARTESIAN_POINT('Ctrl Pts',(-10.5179145463092,24.1345058191473,
2.44219327030303));
#104289=CARTESIAN_POINT('Ctrl Pts',(-10.5091195866238,24.1338568152216,
2.43793229193465));
#104290=CARTESIAN_POINT('Ctrl Pts',(-10.4455584040963,24.1292335402041,
2.40810924459237));
#104291=CARTESIAN_POINT('Ctrl Pts',(-10.3889420389112,24.1254677652967,
2.38668345425721));
#104292=CARTESIAN_POINT('Ctrl Pts',(-10.2661655423819,24.1175459860524,
2.35073756470135));
#104293=CARTESIAN_POINT('Ctrl Pts',(-10.1999009423255,24.1134062802498,
2.33737914950645));
#104294=CARTESIAN_POINT('Ctrl Pts',(-10.0982076998485,24.1069008963359,
2.32583370260708));
#104295=CARTESIAN_POINT('Ctrl Pts',(-10.063401842772,24.1046495063003,2.32344099761911));
#104296=CARTESIAN_POINT('Ctrl Pts',(-10.0194159832921,24.1017479459793,
2.32237465938294));
#104297=CARTESIAN_POINT('Ctrl Pts',(-10.0102864085954,24.1011426970592,
2.32225953398003));
#104298=CARTESIAN_POINT('Ctrl Pts',(-9.99562078069965,24.1001651928335,
2.32224513138096));
#104299=CARTESIAN_POINT('Ctrl Pts',(-9.99008504743967,24.0997950225358,
2.32227872565096));
#104300=CARTESIAN_POINT('Ctrl Pts',(-9.97954409971858,24.0990877825575,
2.32241701763618));
#104301=CARTESIAN_POINT('Ctrl Pts',(-9.9745389007896,24.0987509411749,2.32251460505739));
#104302=CARTESIAN_POINT('Ctrl Pts',(-9.96309843183033,24.0979786130508,
2.32281064054415));
#104303=CARTESIAN_POINT('Ctrl Pts',(-9.9566639092263,24.097542488493,2.32302995189951));
#104304=CARTESIAN_POINT('Ctrl Pts',(-9.93675454604167,24.0961874904716,
2.32387201741309));
#104305=CARTESIAN_POINT('Ctrl Pts',(-9.92328877352544,24.0952631240218,
2.3246735005663));
#104306=CARTESIAN_POINT('Ctrl Pts',(-9.87674450865754,24.0920394019108,
2.32824707018164));
#104307=CARTESIAN_POINT('Ctrl Pts',(-9.8438033470503,24.0897070781581,2.3321836006));
#104308=CARTESIAN_POINT('Ctrl Pts',(-9.81110406371069,24.0873412831715,
2.3374969300026));
#104309=CARTESIAN_POINT('Ctrl Pts',(-9.8111040637107,23.9889087884094,2.3374969300026));
#104310=CARTESIAN_POINT('Ctrl Pts',(-9.81191529024896,23.9889636364787,
2.33736511323545));
#104311=CARTESIAN_POINT('Ctrl Pts',(-9.81272665881509,23.9890184414769,
2.33723414495445));
#104312=CARTESIAN_POINT('Ctrl Pts',(-9.84172904331265,23.9909755864873,
2.33258382552641));
#104313=CARTESIAN_POINT('Ctrl Pts',(-9.87007769787267,23.9928258615754,
2.32908978796103));
#104314=CARTESIAN_POINT('Ctrl Pts',(-9.97499901218653,23.9995357008595,
2.32001627997921));
#104315=CARTESIAN_POINT('Ctrl Pts',(-10.0519381221756,24.0041966484075,
2.32089410523933));
#104316=CARTESIAN_POINT('Ctrl Pts',(-10.1886920676342,24.0127588545096,
2.33587475697394));
#104317=CARTESIAN_POINT('Ctrl Pts',(-10.2485237563857,24.0166018568367,
2.34716578101397));
#104318=CARTESIAN_POINT('Ctrl Pts',(-10.3166652259444,24.0212397627773,
2.36557763965318));
#104319=CARTESIAN_POINT('Ctrl Pts',(-10.3260863158081,24.0218867679212,
2.36824973507468));
#104320=CARTESIAN_POINT('Ctrl Pts',(-10.3414665093096,24.0229530620515,
2.37281998657419));
#104321=CARTESIAN_POINT('Ctrl Pts',(-10.3474458774571,24.023370112437,2.3746487129173));
#104322=CARTESIAN_POINT('Ctrl Pts',(-10.3581652644104,24.0241224177185,
2.3780206985772));
#104323=CARTESIAN_POINT('Ctrl Pts',(-10.3629106168192,24.0244571020804,
2.37954661304432));
#104324=CARTESIAN_POINT('Ctrl Pts',(-10.3730056981297,24.025172684895,2.38286364372141));
#104325=CARTESIAN_POINT('Ctrl Pts',(-10.3783525134138,24.0255538508584,
2.38466316162746));
#104326=CARTESIAN_POINT('Ctrl Pts',(-10.3927804073928,24.026588362199,2.38963468164101));
#104327=CARTESIAN_POINT('Ctrl Pts',(-10.4018357254085,24.0272440831808,
2.39287957797434));
#104328=CARTESIAN_POINT('Ctrl Pts',(-10.4498670089184,24.0307574448773,
2.41075807055968));
#104329=CARTESIAN_POINT('Ctrl Pts',(-10.4880818226941,24.0336789275895,
2.42733802668741));
#104330=CARTESIAN_POINT('Ctrl Pts',(-10.6226302890315,24.0444329518062,
2.49439363666767));
#104331=CARTESIAN_POINT('Ctrl Pts',(-10.7127299581438,24.0525975143552,
2.5561119203801));
#104332=CARTESIAN_POINT('Ctrl Pts',(-10.8070925010526,24.0616903809206,
2.64206304080867));
#104333=CARTESIAN_POINT('Ctrl Pts',(-10.8207923809904,24.063024375184,2.65516031133632));
#104334=CARTESIAN_POINT('Ctrl Pts',(-10.8379217989654,24.0647038632244,
2.67234647965151));
#104335=CARTESIAN_POINT('Ctrl Pts',(-10.8416470526713,24.0650698367928,
2.67613500356579));
#104336=CARTESIAN_POINT('Ctrl Pts',(-10.8475259149516,24.0656483527517,
2.68219520539779));
#104337=CARTESIAN_POINT('Ctrl Pts',(-10.8496962698398,24.0658621420012,
2.68445042566917));
#104338=CARTESIAN_POINT('Ctrl Pts',(-10.8538069716921,24.0662674239749,
2.6887560870136));
#104339=CARTESIAN_POINT('Ctrl Pts',(-10.8557489187102,24.0664590330245,
2.69080483221791));
#104340=CARTESIAN_POINT('Ctrl Pts',(-10.8603095886263,24.066909422426,2.695651097327));
#104341=CARTESIAN_POINT('Ctrl Pts',(-10.8629220511306,24.0671677296809,
2.69845444282798));
#104342=CARTESIAN_POINT('Ctrl Pts',(-10.8715131306733,24.0680184160729,
2.7077639257757));
#104343=CARTESIAN_POINT('Ctrl Pts',(-10.8774323894889,24.0686065498161,
2.7143247823347));
#104344=CARTESIAN_POINT('Ctrl Pts',(-10.9100096679501,24.0718589289608,
2.75126059547338));
#104345=CARTESIAN_POINT('Ctrl Pts',(-10.9351671856618,24.0744299334073,
2.7829286334952));
#104346=CARTESIAN_POINT('Ctrl Pts',(-11.0235730783276,24.0839638950252,
2.90680182008208));
#104347=CARTESIAN_POINT('Ctrl Pts',(-11.0752147353238,24.0906787363243,
3.00654358945951));
#104348=CARTESIAN_POINT('Ctrl Pts',(-11.1174671347088,24.0990208610115,
3.12766277933815));
#104349=CARTESIAN_POINT('Ctrl Pts',(-11.1225780280356,24.1001044803195,
3.14336807468007));
#104350=CARTESIAN_POINT('Ctrl Pts',(-11.1292268821546,24.1016269788217,
3.16536068582546));
#104351=CARTESIAN_POINT('Ctrl Pts',(-11.1310459698255,24.1020567983486,
3.17156152276821));
#104352=CARTESIAN_POINT('Ctrl Pts',(-11.1341021067961,24.1028026432653,
3.18230573883432));
#104353=CARTESIAN_POINT('Ctrl Pts',(-11.1353631215619,24.1031178911798,
3.1868421910346));
#104354=CARTESIAN_POINT('Ctrl Pts',(-11.1379249104958,24.1037742936354,
3.19627702412192));
#104355=CARTESIAN_POINT('Ctrl Pts',(-11.1392213338658,24.1041155802914,
3.20117647501722));
#104356=CARTESIAN_POINT('Ctrl Pts',(-11.142199783399,24.104921707053,3.21273379444466));
#104357=CARTESIAN_POINT('Ctrl Pts',(-11.1438552669073,24.105387384604,3.21939824849787));
#104358=CARTESIAN_POINT('Ctrl Pts',(-11.1491435059492,24.1069355322548,
3.24151183037535));
#104359=CARTESIAN_POINT('Ctrl Pts',(-11.1525221377801,24.1080259960737,
3.25701932123866));
#104360=CARTESIAN_POINT('Ctrl Pts',(-11.1598239857355,24.1106477872416,
3.29412368946212));
#104361=CARTESIAN_POINT('Ctrl Pts',(-11.1634587080319,24.1121875447555,
3.31577063013765));
#104362=CARTESIAN_POINT('Ctrl Pts',(-11.1753706476987,24.1183102831794,
3.40128183167365));
#104363=CARTESIAN_POINT('Ctrl Pts',(-11.1790086177185,24.1230165690624,
3.46567274180069));
#104364=CARTESIAN_POINT('Ctrl Pts',(-11.1756942409554,24.1325613930551,
3.59561513165207));
#104365=CARTESIAN_POINT('Ctrl Pts',(-11.1685441374264,24.1373833301956,
3.66095184226147));
#104366=CARTESIAN_POINT('Ctrl Pts',(-11.1541277724144,24.1426625009959,
3.7349014289201));
#104367=CARTESIAN_POINT('Ctrl Pts',(-11.1521491590677,24.1433385277543,
3.74442161725159));
#104368=CARTESIAN_POINT('Ctrl Pts',(-11.149255948915,24.144263065487,3.75752570171869));
#104369=CARTESIAN_POINT('Ctrl Pts',(-11.1484421054994,24.144516810971,3.76113110578009));
#104370=CARTESIAN_POINT('Ctrl Pts',(-11.1470171253302,24.1449504145443,
3.76730836856232));
#104371=CARTESIAN_POINT('Ctrl Pts',(-11.1464142844339,24.1451307300009,
3.76988208259098));
#104372=CARTESIAN_POINT('Ctrl Pts',(-11.1451370641186,24.1455063015767,
3.77525342519396));
#104373=CARTESIAN_POINT('Ctrl Pts',(-11.1444610897819,24.1457014587139,
3.77805063911787));
#104374=CARTESIAN_POINT('Ctrl Pts',(-11.1427853326147,24.1461766221915,
3.78487535163241));
#104375=CARTESIAN_POINT('Ctrl Pts',(-11.1417744905766,24.1464560052845,
3.78890014949772));
#104376=CARTESIAN_POINT('Ctrl Pts',(-11.1380570442915,24.1474581975698,
3.8033773253675));
#104377=CARTESIAN_POINT('Ctrl Pts',(-11.1352279128659,24.1481744128238,
3.81379809423215));
#104378=CARTESIAN_POINT('Ctrl Pts',(-11.1278009076869,24.1499477201924,
3.83973830325954));
#104379=CARTESIAN_POINT('Ctrl Pts',(-11.1230255800533,24.1509964301968,
3.85520501594267));
#104380=CARTESIAN_POINT('Ctrl Pts',(-11.1006447766295,24.1555563401294,
3.92272340332944));
#104381=CARTESIAN_POINT('Ctrl Pts',(-11.0797269337279,24.1589473524532,
3.97360817774133));
#104382=CARTESIAN_POINT('Ctrl Pts',(-11.0194381504682,24.167342000269,4.09529633153584));
#104383=CARTESIAN_POINT('Ctrl Pts',(-10.9761859717322,24.1723425770645,
4.16384540049577));
#104384=CARTESIAN_POINT('Ctrl Pts',(-10.9169637275359,24.1785961981693,
4.23925572066521));
#104385=CARTESIAN_POINT('Ctrl Pts',(-10.907444081569,24.1795857399449,4.25091058282987));
#104386=CARTESIAN_POINT('Ctrl Pts',(-10.893399380992,24.1810254102074,4.2674482601571));
#104387=CARTESIAN_POINT('Ctrl Pts',(-10.8890518873859,24.1814683718461,
4.27248043629549));
#104388=CARTESIAN_POINT('Ctrl Pts',(-10.8813277272416,24.1822508620973,
4.28126948771694));
#104389=CARTESIAN_POINT('Ctrl Pts',(-10.8779690424634,24.182589644258,4.28504199528249));
#104390=CARTESIAN_POINT('Ctrl Pts',(-10.8709806206956,24.1832916125095,
4.29279051687329));
#104391=CARTESIAN_POINT('Ctrl Pts',(-10.8673476865037,24.1836549277722,
4.29676347451588));
#104392=CARTESIAN_POINT('Ctrl Pts',(-10.8579487165592,24.184590889867,4.30690167835532));
#104393=CARTESIAN_POINT('Ctrl Pts',(-10.8521434878504,24.1851651907578,
4.3130300046301));
#104394=CARTESIAN_POINT('Ctrl Pts',(-10.8271375366571,24.1876235091398,
4.33886565849901));
#104395=CARTESIAN_POINT('Ctrl Pts',(-10.8073166493765,24.189534199184,4.35795786992865));
#104396=CARTESIAN_POINT('Ctrl Pts',(-10.7128009902719,24.198483481559,4.44282170940828));
#104397=CARTESIAN_POINT('Ctrl Pts',(-10.6306340208212,24.2058659765903,
4.49964634278999));
#104398=CARTESIAN_POINT('Ctrl Pts',(-10.5227216164905,24.2147272092718,
4.55562535048993));
#104399=CARTESIAN_POINT('Ctrl Pts',(-10.5028350691704,24.2163265857171,
4.5652416419023));
#104400=CARTESIAN_POINT('Ctrl Pts',(-10.4626914948827,24.2194747874122,
4.58327848382458));
#104401=CARTESIAN_POINT('Ctrl Pts',(-10.4424454050007,24.2210233204887,
4.59170412995736));
#104402=CARTESIAN_POINT('Ctrl Pts',(-10.4168196816447,24.2229248666298,
4.60153842403963));
#104403=CARTESIAN_POINT('Ctrl Pts',(-10.411651012751,24.2233054738132,4.60348040007461));
#104404=CARTESIAN_POINT('Ctrl Pts',(-10.4034583209276,24.2239039286604,
4.60649298863004));
#104405=CARTESIAN_POINT('Ctrl Pts',(-10.4004433342001,24.2241231365364,
4.60758768832645));
#104406=CARTESIAN_POINT('Ctrl Pts',(-10.395049705165,24.2245134033883,4.60952113720498));
#104407=CARTESIAN_POINT('Ctrl Pts',(-10.3926728531371,24.2246847301414,
4.6103645590727));
#104408=CARTESIAN_POINT('Ctrl Pts',(-10.3869632402317,24.2250947371436,
4.61236997896257));
#104409=CARTESIAN_POINT('Ctrl Pts',(-10.3836279463389,24.2253329859171,
4.61352463780255));
#104410=CARTESIAN_POINT('Ctrl Pts',(-10.373462612011,24.2260554437884,4.61699272153963));
#104411=CARTESIAN_POINT('Ctrl Pts',(-10.3666163143677,24.2265369773123,
4.61925848087774));
#104412=CARTESIAN_POINT('Ctrl Pts',(-10.2940548524148,24.2315918070207,
4.64253520452934));
#104413=CARTESIAN_POINT('Ctrl Pts',(-10.2266249458674,24.2358723645131,
4.65779920550411));
#104414=CARTESIAN_POINT('Ctrl Pts',(-10.0703481299661,24.2456276582886,
4.67898802644893));
#104415=CARTESIAN_POINT('Ctrl Pts',(-9.98140506213337,24.2510804180271,
4.68093760653492));
#104416=CARTESIAN_POINT('Ctrl Pts',(-9.87841685996031,24.2578286773854,
4.67155012466697));
#104417=CARTESIAN_POINT('Ctrl Pts',(-9.86377060047379,24.2587979480084,
4.66993746571443));
#104418=CARTESIAN_POINT('Ctrl Pts',(-9.84261795209693,24.260213427659,4.66720583096438));
#104419=CARTESIAN_POINT('Ctrl Pts',(-9.83608426693785,24.2606528087374,
4.66630621635849));
#104420=CARTESIAN_POINT('Ctrl Pts',(-9.82456899746088,24.2614311719526,
4.66462202214448));
#104421=CARTESIAN_POINT('Ctrl Pts',(-9.81958420850442,24.2617694330122,
4.66386022869601));
#104422=CARTESIAN_POINT('Ctrl Pts',(-9.80926497968736,24.2624724895564,
4.66221531988234));
#104423=CARTESIAN_POINT('Ctrl Pts',(-9.80393143145864,24.2628374274638,
4.66132743551747));
#104424=CARTESIAN_POINT('Ctrl Pts',(-9.79018358906478,24.2637822218593,
4.65894140482426));
#104425=CARTESIAN_POINT('Ctrl Pts',(-9.78177927292031,24.2643637922863,
4.65738835905638));
#104426=CARTESIAN_POINT('Ctrl Pts',(-9.74541060061829,24.2668983584304,
4.65025753844924));
#104427=CARTESIAN_POINT('Ctrl Pts',(-9.7176391828448,24.2688801271902,4.64375709536075));
#104428=CARTESIAN_POINT('Ctrl Pts',(-9.5948034139582,24.2778612078305,4.61025869106878));
#104429=CARTESIAN_POINT('Ctrl Pts',(-9.503133469902,24.2851936833931,4.57236962114452));
#104430=CARTESIAN_POINT('Ctrl Pts',(-9.38105678563893,24.2954296788097,
4.50286723195353));
#104431=CARTESIAN_POINT('Ctrl Pts',(-9.34594086655984,24.2984298107287,
4.48032690123639));
#104432=CARTESIAN_POINT('Ctrl Pts',(-9.30724293608549,24.3017431118799,
4.45248012518211));
#104433=CARTESIAN_POINT('Ctrl Pts',(-9.30242124055299,24.3021560575304,
4.4489544860329));
#104434=CARTESIAN_POINT('Ctrl Pts',(-9.29473930253434,24.3028138786995,
4.44324723573708));
#104435=CARTESIAN_POINT('Ctrl Pts',(-9.29186194567442,24.3030602536743,
4.44108899472839));
#104436=CARTESIAN_POINT('Ctrl Pts',(-9.28676129659575,24.3034968983908,
4.43722647281982));
#104437=CARTESIAN_POINT('Ctrl Pts',(-9.28453414621374,24.3036875174806,
4.43552740316397));
#104438=CARTESIAN_POINT('Ctrl Pts',(-9.27975323057566,24.3040966156015,
4.43185303369437));
#104439=CARTESIAN_POINT('Ctrl Pts',(-9.2772015164985,24.3043149128093,4.42987517342508));
#104440=CARTESIAN_POINT('Ctrl Pts',(-9.27012279949983,24.3049204527922,
4.42434164157424));
#104441=CARTESIAN_POINT('Ctrl Pts',(-9.26561360709267,24.3053061414466,
4.4207631766241));
#104442=CARTESIAN_POINT('Ctrl Pts',(-9.2392060405879,24.3075658400765,4.39948889934357));
#104443=CARTESIAN_POINT('Ctrl Pts',(-9.21791966020004,24.3093912876951,
4.38104390819895));
#104444=CARTESIAN_POINT('Ctrl Pts',(-9.14289506408989,24.3159271951498,
4.31116965183271));
#104445=CARTESIAN_POINT('Ctrl Pts',(-9.09339600043173,24.3204503386145,
4.25544413312255));
#104446=CARTESIAN_POINT('Ctrl Pts',(-9.01202441224111,24.3290167748111,
4.14422301126975));
#104447=CARTESIAN_POINT('Ctrl Pts',(-8.97877066676186,24.3330180236281,
4.09009158106499));
#104448=CARTESIAN_POINT('Ctrl Pts',(-8.94558002571878,24.3378315387344,
4.02477657225738));
#104449=CARTESIAN_POINT('Ctrl Pts',(-8.94123149980395,24.3384817836427,
4.01594688326271));
#104450=CARTESIAN_POINT('Ctrl Pts',(-8.93429513935819,24.3395524271792,
4.00140553972513));
#104451=CARTESIAN_POINT('Ctrl Pts',(-8.93164129360405,24.3399705582732,
3.99572576810771));
#104452=CARTESIAN_POINT('Ctrl Pts',(-8.92695756794208,24.3407241724259,
3.98548932293499));
#104453=CARTESIAN_POINT('Ctrl Pts',(-8.9249110376468,24.3410590784532,3.98094039692475));
#104454=CARTESIAN_POINT('Ctrl Pts',(-8.92061417091324,24.3417744453672,
3.97122505188383));
#104455=CARTESIAN_POINT('Ctrl Pts',(-8.91837190116292,24.342155169453,3.966055223606));
#104456=CARTESIAN_POINT('Ctrl Pts',(-8.91241692689779,24.3431867626496,
3.95205083106616));
#104457=CARTESIAN_POINT('Ctrl Pts',(-8.90877487370587,24.343839982006,3.94318687825367));
#104458=CARTESIAN_POINT('Ctrl Pts',(-8.890109885129,24.3473097340914,3.89613504604175));
#104459=CARTESIAN_POINT('Ctrl Pts',(-8.87698397865023,24.3501881860563,
3.85723011591546));
#104460=CARTESIAN_POINT('Ctrl Pts',(-8.83803160479263,24.3605111905588,
3.71819327413174));
#104461=CARTESIAN_POINT('Ctrl Pts',(-8.82337406762189,24.3682506968201,
3.61544043113425));
#104462=CARTESIAN_POINT('Ctrl Pts',(-8.82206404542765,24.3773963265622,
3.48795472708509));
#104463=CARTESIAN_POINT('Ctrl Pts',(-8.82255861041381,24.3791060169908,
3.46380370478829));
#104464=CARTESIAN_POINT('Ctrl Pts',(-8.82408714899806,24.381174854874,3.43399658779826));
#104465=CARTESIAN_POINT('Ctrl Pts',(-8.82441999866294,24.3815675345662,
3.42831215364252));
#104466=CARTESIAN_POINT('Ctrl Pts',(-8.8250074128629,24.3821807442675,3.41938964404949));
#104467=CARTESIAN_POINT('Ctrl Pts',(-8.82523416205303,24.3824027440407,
3.41614991977712));
#104468=CARTESIAN_POINT('Ctrl Pts',(-8.82567904546122,24.3828126220791,
3.41014999161365));
#104469=CARTESIAN_POINT('Ctrl Pts',(-8.82589351054565,24.3830006912897,
3.40738963363798));
#104470=CARTESIAN_POINT('Ctrl Pts',(-8.82640968761386,24.3834324359487,
3.40103615878903));
#104471=CARTESIAN_POINT('Ctrl Pts',(-8.82671816705856,24.3836757339303,
3.39744365181161));
#104472=CARTESIAN_POINT('Ctrl Pts',(-8.82772930759005,24.3844300184669,
3.38627028580868));
#104473=CARTESIAN_POINT('Ctrl Pts',(-8.8284889965435,24.384937968062,3.37869459828809));
#104474=CARTESIAN_POINT('Ctrl Pts',(-8.83044156344638,24.3861202274647,
3.36095760769738));
#104475=CARTESIAN_POINT('Ctrl Pts',(-8.83169349994172,24.3867916629658,
3.35080328051745));
#104476=CARTESIAN_POINT('Ctrl Pts',(-8.83661329461588,24.3891590559477,
3.31477189462154));
#104477=CARTESIAN_POINT('Ctrl Pts',(-8.84101012210147,24.3908245986558,
3.28900064600185));
#104478=CARTESIAN_POINT('Ctrl Pts',(-8.86277904510676,24.3976472359572,
3.18285033400713));
#104479=CARTESIAN_POINT('Ctrl Pts',(-8.88768594380953,24.4026239926642,
3.10425542019625));
#104480=CARTESIAN_POINT('Ctrl Pts',(-8.93884366034744,24.4106652551332,
2.98704032478918));
#104481=CARTESIAN_POINT('Ctrl Pts',(-8.95952683311905,24.4135854895129,
2.94628956197865));
#104482=CARTESIAN_POINT('Ctrl Pts',(-8.98762379648753,24.4172555736018,
2.89809292741013));
#104483=CARTESIAN_POINT('Ctrl Pts',(-8.99283873979115,24.4179258958574,
2.88940693841259));
#104484=CARTESIAN_POINT('Ctrl Pts',(-9.00121937018993,24.4189869698737,
2.8758477214116));
#104485=CARTESIAN_POINT('Ctrl Pts',(-9.00431025744655,24.4193749994365,
2.87092866233433));
#104486=CARTESIAN_POINT('Ctrl Pts',(-9.01008422527972,24.4200939320146,
2.86188872424522));
#104487=CARTESIAN_POINT('Ctrl Pts',(-9.01275697642874,24.4204244490011,
2.85776137422834));
#104488=CARTESIAN_POINT('Ctrl Pts',(-9.01874523034053,24.4211600364058,
2.84863982828143));
#104489=CARTESIAN_POINT('Ctrl Pts',(-9.02207315595482,24.4215655630385,
2.84365399241824));
#104490=CARTESIAN_POINT('Ctrl Pts',(-9.03177626224032,24.4227387606132,
2.8293546098887));
#104491=CARTESIAN_POINT('Ctrl Pts',(-9.03824729854296,24.4235100134031,
2.82010723535407));
#104492=CARTESIAN_POINT('Ctrl Pts',(-9.09326260967914,24.4299779948076,
2.74384539671418));
#104493=CARTESIAN_POINT('Ctrl Pts',(-9.14860328150742,24.4359460769373,
2.68203848534737));
#104494=CARTESIAN_POINT('Ctrl Pts',(-9.26704529509314,24.4476577550002,
2.57490567406071));
#104495=CARTESIAN_POINT('Ctrl Pts',(-9.32907179068441,24.4533545926746,
2.52898020952262));
#104496=CARTESIAN_POINT('Ctrl Pts',(-9.40308516353879,24.4593926849135,
2.4846806186782));
#104497=CARTESIAN_POINT('Ctrl Pts',(-9.41108482824211,24.4600359119414,
2.48001975416346));
#104498=CARTESIAN_POINT('Ctrl Pts',(-9.42229269438758,24.4609232531667,
2.47366551515474));
#104499=CARTESIAN_POINT('Ctrl Pts',(-9.42545475454424,24.4611720819424,
2.47189204480144));
#104500=CARTESIAN_POINT('Ctrl Pts',(-9.43091896944154,24.4615994006953,
2.468860472488));
#104501=CARTESIAN_POINT('Ctrl Pts',(-9.43321720788587,24.4617783208176,
2.46759542259409));
#104502=CARTESIAN_POINT('Ctrl Pts',(-9.43805940247676,24.4621535608969,
2.46495111172499));
#104503=CARTESIAN_POINT('Ctrl Pts',(-9.44060424744939,24.4623497694241,
2.46357352957027));
#104504=CARTESIAN_POINT('Ctrl Pts',(-9.4468840481462,24.4628315472717,2.46020399903846));
#104505=CARTESIAN_POINT('Ctrl Pts',(-9.45062476116366,24.463116451531,2.458222755026));
#104506=CARTESIAN_POINT('Ctrl Pts',(-9.46444467316649,24.464161687603,2.45099826826977));
#104507=CARTESIAN_POINT('Ctrl Pts',(-9.47458929777979,24.4649146582012,
2.44588057652014));
#104508=CARTESIAN_POINT('Ctrl Pts',(-9.54715197539782,24.4702110383263,
2.41058253436047));
#104509=CARTESIAN_POINT('Ctrl Pts',(-9.61206200005963,24.4744881663096,
2.38581490445392));
#104510=CARTESIAN_POINT('Ctrl Pts',(-9.72232003540705,24.4815720685054,
2.35455823863656));
#104511=CARTESIAN_POINT('Ctrl Pts',(-9.76650114682695,24.4843643460958,
2.34474448913894));
#104512=CARTESIAN_POINT('Ctrl Pts',(-9.81110406371068,24.4872084044306,
2.3374969300026));
#104513=CARTESIAN_POINT('Origin',(-10.,12.3756328852638,3.5));
#104514=CARTESIAN_POINT('',(-8.88740821192766,24.85,3.88630891215967));
#104515=CARTESIAN_POINT('Ctrl Pts',(-9.81110406371068,24.4872084044306,
2.3374969300026));
#104516=CARTESIAN_POINT('Ctrl Pts',(-9.84744767330581,24.4895258166764,
2.33159143147981));
#104517=CARTESIAN_POINT('Ctrl Pts',(-9.88407135600494,24.4918772584382,
2.32738971255254));
#104518=CARTESIAN_POINT('Ctrl Pts',(-9.93585211116218,24.4952622625889,
2.32390221340624));
#104519=CARTESIAN_POINT('Ctrl Pts',(-9.9508652393094,24.4962506731116,2.32317941167113));
#104520=CARTESIAN_POINT('Ctrl Pts',(-9.97253398679687,24.4976891501419,
2.32255153283919));
#104521=CARTESIAN_POINT('Ctrl Pts',(-9.97918181701203,24.4981320730973,
2.32241523663539));
#104522=CARTESIAN_POINT('Ctrl Pts',(-9.9908831335633,24.4989146801423,2.32227444633923));
#104523=CARTESIAN_POINT('Ctrl Pts',(-9.9959362053581,24.4992536194162,2.32224617121823));
#104524=CARTESIAN_POINT('Ctrl Pts',(-10.006377803737,24.4999560951491,2.32225494150819));
#104525=CARTESIAN_POINT('Ctrl Pts',(-10.0117661979241,24.5003197619567,
2.3222964489739));
#104526=CARTESIAN_POINT('Ctrl Pts',(-10.025608102459,24.5012570208635,2.32249807902151));
#104527=CARTESIAN_POINT('Ctrl Pts',(-10.0340603947914,24.5018322727855,
2.3227122561429));
#104528=CARTESIAN_POINT('Ctrl Pts',(-10.0701066742898,24.5042985381159,
2.32401415126517));
#104529=CARTESIAN_POINT('Ctrl Pts',(-10.0976581075266,24.5062164080555,
2.32598111791656));
#104530=CARTESIAN_POINT('Ctrl Pts',(-10.2241537223738,24.5151801732983,
2.33949529173965));
#104531=CARTESIAN_POINT('Ctrl Pts',(-10.3214424889142,24.5225696808515,
2.3625973129843));
#104532=CARTESIAN_POINT('Ctrl Pts',(-10.435370567593,24.5314392822114,2.40545077646408));
#104533=CARTESIAN_POINT('Ctrl Pts',(-10.4558762463951,24.5330425250445,
2.4138312852233));
#104534=CARTESIAN_POINT('Ctrl Pts',(-10.495869957306,24.5361687506067,2.43150870911483));
#104535=CARTESIAN_POINT('Ctrl Pts',(-10.5153637212961,24.537692178363,2.44077338014174));
#104536=CARTESIAN_POINT('Ctrl Pts',(-10.5394916397183,24.53956783786,2.45306444652941));
#104537=CARTESIAN_POINT('Ctrl Pts',(-10.5443725547072,24.5399467473109,
2.45559404104909));
#104538=CARTESIAN_POINT('Ctrl Pts',(-10.5520707813183,24.5405433270755,
2.45965237231793));
#104539=CARTESIAN_POINT('Ctrl Pts',(-10.5548997961721,24.5407623395513,
2.46115855356095));
#104540=CARTESIAN_POINT('Ctrl Pts',(-10.5599533487098,24.5411531187626,
2.46387562324609));
#104541=CARTESIAN_POINT('Ctrl Pts',(-10.562180114459,24.5413251477094,2.46508213084928));
#104542=CARTESIAN_POINT('Ctrl Pts',(-10.5675261852479,24.5417377956757,
2.46800108843247));
#104543=CARTESIAN_POINT('Ctrl Pts',(-10.5706416429414,24.5419779743059,
2.46972050365281));
#104544=CARTESIAN_POINT('Ctrl Pts',(-10.5801336042773,24.5427089811739,
2.4750153630886));
#104545=CARTESIAN_POINT('Ctrl Pts',(-10.5864848000015,24.5431970647081,
2.47863616142687));
#104546=CARTESIAN_POINT('Ctrl Pts',(-10.6450295576518,24.547690392334,2.51273854727147));
#104547=CARTESIAN_POINT('Ctrl Pts',(-10.6948454971311,24.5514732908712,
2.54714107492292));
#104548=CARTESIAN_POINT('Ctrl Pts',(-10.8176511937564,24.5612818958166,
2.64672573467748));
#104549=CARTESIAN_POINT('Ctrl Pts',(-10.8855451811361,24.5672476308877,
2.71741578046518));
#104550=CARTESIAN_POINT('Ctrl Pts',(-10.9522485518537,24.57453703089,2.80681101364116));
#104551=CARTESIAN_POINT('Ctrl Pts',(-10.9603630488586,24.5754524221367,
2.81809746798643));
#104552=CARTESIAN_POINT('Ctrl Pts',(-10.9719499482024,24.5768039345743,
2.83483083477734));
#104553=CARTESIAN_POINT('Ctrl Pts',(-10.9755805266181,24.5772341123044,
2.84016717763361));
#104554=CARTESIAN_POINT('Ctrl Pts',(-10.981963221781,24.5780025971655,2.84971651246152));
#104555=CARTESIAN_POINT('Ctrl Pts',(-10.9847325658078,24.5783402534562,
2.85391784145478));
#104556=CARTESIAN_POINT('Ctrl Pts',(-10.9904685240862,24.5790486096619,
2.86274232934819));
#104557=CARTESIAN_POINT('Ctrl Pts',(-10.9934298809175,24.5794194926574,
2.86736874409735));
#104558=CARTESIAN_POINT('Ctrl Pts',(-11.0011033812624,24.5803943313984,
2.87954350429007));
#104559=CARTESIAN_POINT('Ctrl Pts',(-11.0057624567711,24.5810001998471,
2.88712471412224));
#104560=CARTESIAN_POINT('Ctrl Pts',(-11.0267906901765,24.5838007984269,
2.92222729309866));
#104561=CARTESIAN_POINT('Ctrl Pts',(-11.0421176833835,24.5860322226038,
2.95035391782175));
#104562=CARTESIAN_POINT('Ctrl Pts',(-11.1006501734712,24.5954044951267,
3.06903849499745));
#104563=CARTESIAN_POINT('Ctrl Pts',(-11.133340926597,24.6028720028285,3.16430418967029));
#104564=CARTESIAN_POINT('Ctrl Pts',(-11.1551715559829,24.6107333941226,
3.27035363368577));
#104565=CARTESIAN_POINT('Ctrl Pts',(-11.1567014679258,24.6113112850736,
3.27818815235943));
#104566=CARTESIAN_POINT('Ctrl Pts',(-11.1634462987685,24.6139893387851,
3.31469710120222));
#104567=CARTESIAN_POINT('Ctrl Pts',(-11.1676758582834,24.6160630055586,
3.34354595595367));
#104568=CARTESIAN_POINT('Ctrl Pts',(-11.1714244154802,24.6184660213716,
3.37797554935323));
#104569=CARTESIAN_POINT('Ctrl Pts',(-11.1719798354967,24.618844630165,3.38343072517334));
#104570=CARTESIAN_POINT('Ctrl Pts',(-11.1728262985415,24.6194608623473,
3.3923630708616));
#104571=CARTESIAN_POINT('Ctrl Pts',(-11.1731400170512,24.6196996730503,
3.39583793275172));
#104572=CARTESIAN_POINT('Ctrl Pts',(-11.1736758913255,24.6201271783819,
3.40208325588426));
#104573=CARTESIAN_POINT('Ctrl Pts',(-11.1739036878909,24.6203161796981,
3.40485317222141));
#104574=CARTESIAN_POINT('Ctrl Pts',(-11.1743822722149,24.6207298953925,
3.41093609399126));
#104575=CARTESIAN_POINT('Ctrl Pts',(-11.1746288480315,24.620954374219,3.4142493690343));
#104576=CARTESIAN_POINT('Ctrl Pts',(-11.1753007899725,24.6216007991028,
3.42382571591282));
#104577=CARTESIAN_POINT('Ctrl Pts',(-11.1756901163328,24.6220207953815,
3.43009132261101));
#104578=CARTESIAN_POINT('Ctrl Pts',(-11.1782855297841,24.6252152931303,
3.47805295471361));
#104579=CARTESIAN_POINT('Ctrl Pts',(-11.1783232241898,24.627880759095,3.519841793099));
#104580=CARTESIAN_POINT('Ctrl Pts',(-11.1715019384844,24.6360688363326,
3.65018982671148));
#104581=CARTESIAN_POINT('Ctrl Pts',(-11.1568579807933,24.6414247655147,
3.73802116742698));
#104582=CARTESIAN_POINT('Ctrl Pts',(-11.1221808252907,24.6494204005243,
3.85946314593704));
#104583=CARTESIAN_POINT('Ctrl Pts',(-11.110158144781,24.6518351000848,3.89503417950717));
#104584=CARTESIAN_POINT('Ctrl Pts',(-11.0929674978348,24.6549356787997,
3.93887194002238));
#104585=CARTESIAN_POINT('Ctrl Pts',(-11.0893677045515,24.6555688947879,
3.94773265056259));
#104586=CARTESIAN_POINT('Ctrl Pts',(-11.0834667544391,24.6565825742762,
3.96176496215947));
#104587=CARTESIAN_POINT('Ctrl Pts',(-11.0812354864862,24.6569606712743,
3.96696564017513));
#104588=CARTESIAN_POINT('Ctrl Pts',(-11.0769856110184,24.6576713587674,
3.97667754354162));
#104589=CARTESIAN_POINT('Ctrl Pts',(-11.0749759131138,24.6580036391707,
3.98119255167981));
#104590=CARTESIAN_POINT('Ctrl Pts',(-11.0704128130022,24.6587497940021,
3.99127279919678));
#104591=CARTESIAN_POINT('Ctrl Pts',(-11.0678443232913,24.6591641795745,
3.99683100970883));
#104592=CARTESIAN_POINT('Ctrl Pts',(-11.0601045360422,24.6603966729942,
4.01324260471443));
#104593=CARTESIAN_POINT('Ctrl Pts',(-11.0548103987138,24.6612189993113,
4.02403683324936));
#104594=CARTESIAN_POINT('Ctrl Pts',(-11.0175125867451,24.6668771620815,
4.09722748314501));
#104595=CARTESIAN_POINT('Ctrl Pts',(-10.9801624161662,24.6719029745937,
4.15672747834859));
#104596=CARTESIAN_POINT('Ctrl Pts',(-10.8924717794376,24.6824965971428,
4.27213356121441));
#104597=CARTESIAN_POINT('Ctrl Pts',(-10.8416157609093,24.6880543584961,
4.32727242856068));
#104598=CARTESIAN_POINT('Ctrl Pts',(-10.7710390506492,24.6948163454437,
4.39050004775844));
#104599=CARTESIAN_POINT('Ctrl Pts',(-10.7558724303697,24.6962200674192,
4.40340939677099));
#104600=CARTESIAN_POINT('Ctrl Pts',(-10.7361950044635,24.6979722378829,
4.41931550669535));
#104601=CARTESIAN_POINT('Ctrl Pts',(-10.7319820484678,24.69834348231,4.42267348991208));
#104602=CARTESIAN_POINT('Ctrl Pts',(-10.7252814219442,24.6989276109887,
4.42793951744813));
#104603=CARTESIAN_POINT('Ctrl Pts',(-10.7228089856875,24.6991417990795,
4.4298666892926));
#104604=CARTESIAN_POINT('Ctrl Pts',(-10.7181023376188,24.6995469419265,
4.43350523041063));
#104605=CARTESIAN_POINT('Ctrl Pts',(-10.715869662876,24.6997380240306,4.43521848166122));
#104606=CARTESIAN_POINT('Ctrl Pts',(-10.710618964948,24.7001848684021,4.43921780400885));
#104607=CARTESIAN_POINT('Ctrl Pts',(-10.707595985527,24.7004401819263,4.4414973812903));
#104608=CARTESIAN_POINT('Ctrl Pts',(-10.6977004217185,24.7012697984553,
4.44888487469039));
#104609=CARTESIAN_POINT('Ctrl Pts',(-10.690782922766,24.7018401504645,4.45393256996105));
#104610=CARTESIAN_POINT('Ctrl Pts',(-10.6333959288998,24.7064989980139,
4.49485618716958));
#104611=CARTESIAN_POINT('Ctrl Pts',(-10.5802169131868,24.7103604762319,
4.52678123939741));
#104612=CARTESIAN_POINT('Ctrl Pts',(-10.439462011152,24.7200974689023,4.5968353116984));
#104613=CARTESIAN_POINT('Ctrl Pts',(-10.349330878844,24.7259281099295,4.62877821214286));
#104614=CARTESIAN_POINT('Ctrl Pts',(-10.2423306590079,24.7330885267044,
4.65263912210892));
#104615=CARTESIAN_POINT('Ctrl Pts',(-10.2282655523376,24.7340334742023,
4.65550677304565));
#104616=CARTESIAN_POINT('Ctrl Pts',(-10.2077139414109,24.7354211779157,
4.65930705481101));
#104617=CARTESIAN_POINT('Ctrl Pts',(-10.201266146849,24.735857540156,4.66044382200123));
#104618=CARTESIAN_POINT('Ctrl Pts',(-10.1898230547305,24.7366338640599,
4.66236303820255));
#104619=CARTESIAN_POINT('Ctrl Pts',(-10.1848315267483,24.7369731378763,
4.66316719780408));
#104620=CARTESIAN_POINT('Ctrl Pts',(-10.1744284135187,24.7376816342498,
4.66477453633613));
#104621=CARTESIAN_POINT('Ctrl Pts',(-10.1690161110633,24.7380510203235,
4.66557219613443));
#104622=CARTESIAN_POINT('Ctrl Pts',(-10.1549275179755,24.7390146948843,
4.6675483683054));
#104623=CARTESIAN_POINT('Ctrl Pts',(-10.1462434261853,24.739610801227,4.66866786611394));
#104624=CARTESIAN_POINT('Ctrl Pts',(-10.1073997039169,24.7422871092663,
4.67323563103416));
#104625=CARTESIAN_POINT('Ctrl Pts',(-10.0771283640713,24.7443999204743,
4.67561365615504));
#104626=CARTESIAN_POINT('Ctrl Pts',(-9.94814003051134,24.7535243028678,
4.68074342291793));
#104627=CARTESIAN_POINT('Ctrl Pts',(-9.84938454656352,24.7608553383744,
4.67224325478121));
#104628=CARTESIAN_POINT('Ctrl Pts',(-9.71478833380063,24.7708602454614,
4.64335748139481));
#104629=CARTESIAN_POINT('Ctrl Pts',(-9.67713166219693,24.7736544798527,
4.63329992910002));
#104630=CARTESIAN_POINT('Ctrl Pts',(-9.63439214308377,24.7767721707989,
4.6195807832112));
#104631=CARTESIAN_POINT('Ctrl Pts',(-9.62875890158339,24.7771819827859,
4.61772549654814));
#104632=CARTESIAN_POINT('Ctrl Pts',(-9.61968878589105,24.7778397617332,
4.61466215092699));
#104633=CARTESIAN_POINT('Ctrl Pts',(-9.61624316678565,24.7780891603604,
4.6134805899254));
#104634=CARTESIAN_POINT('Ctrl Pts',(-9.61018203740412,24.7785269536142,
4.61137064950751));
#104635=CARTESIAN_POINT('Ctrl Pts',(-9.6075643216126,24.7787157210086,4.61044900969929));
#104636=CARTESIAN_POINT('Ctrl Pts',(-9.60491925481046,24.7789061574666,
4.60950721869302));
#104637=CARTESIAN_POINT('Ctrl Pts',(-9.60488870787621,24.7789083567089,
4.6094963408627));
#104638=CARTESIAN_POINT('Ctrl Pts',(-9.60482845106778,24.7789126948493,
4.60947488047688));
#104639=CARTESIAN_POINT('Ctrl Pts',(-9.60479874117483,24.7789148337508,
4.60946429799146));
#104640=CARTESIAN_POINT('Ctrl Pts',(-9.60474012446376,24.7789190536628,
4.60944341641778));
#104641=CARTESIAN_POINT('Ctrl Pts',(-9.60471121765258,24.7789211346748,
4.60943311740364));
#104642=CARTESIAN_POINT('Ctrl Pts',(-9.60465417506417,24.7789252411204,
4.60941279156947));
#104643=CARTESIAN_POINT('Ctrl Pts',(-9.60462603923627,24.7789272665595,
4.60940276479833));
#104644=CARTESIAN_POINT('Ctrl Pts',(-9.60457050807002,24.778931264064,4.60938297276363));
#104645=CARTESIAN_POINT('Ctrl Pts',(-9.60454311273798,24.7789332361307,
4.60937320756493));
#104646=CARTESIAN_POINT('Ctrl Pts',(-9.60448903373301,24.7789371289709,
4.60935392858415));
#104647=CARTESIAN_POINT('Ctrl Pts',(-9.60446235003137,24.7789390497481,
4.60934441485042));
#104648=CARTESIAN_POINT('Ctrl Pts',(-9.60440966684827,24.7789428419896,
4.60932562919048));
#104649=CARTESIAN_POINT('Ctrl Pts',(-9.60438366735648,24.7789447134561,
4.60931635731546));
#104650=CARTESIAN_POINT('Ctrl Pts',(-9.60433232661003,24.778948408951,4.60929804626983));
#104651=CARTESIAN_POINT('Ctrl Pts',(-9.60430698532761,24.7789502329829,
4.60928900714078));
#104652=CARTESIAN_POINT('Ctrl Pts',(-9.60425693616873,24.7789538354003,
4.60927115288266));
#104653=CARTESIAN_POINT('Ctrl Pts',(-9.60423222832188,24.7789556137851,
4.60926233781244));
#104654=CARTESIAN_POINT('Ctrl Pts',(-9.60418342265416,24.778959126595,4.60924492347402));
#104655=CARTESIAN_POINT('Ctrl Pts',(-9.60415932478083,24.7789608610253,
4.60923632423244));
#104656=CARTESIAN_POINT('Ctrl Pts',(-9.60411171661651,24.7789642875457,
4.60921933367699));
#104657=CARTESIAN_POINT('Ctrl Pts',(-9.60408820632863,24.7789659796366,
4.60921094240684));
#104658=CARTESIAN_POINT('Ctrl Pts',(-9.60404175207241,24.7789693230123,
4.60919436033169));
#104659=CARTESIAN_POINT('Ctrl Pts',(-9.60401880808486,24.7789709742994,
4.60918616955991));
#104660=CARTESIAN_POINT('Ctrl Pts',(-9.60397346620513,24.7789742375263,
4.60916998138069));
#104661=CARTESIAN_POINT('Ctrl Pts',(-9.60395106826876,24.7789758494703,
4.6091619839952));
#104662=CARTESIAN_POINT('Ctrl Pts',(-9.60390679912848,24.7789790354076,
4.6091461757869));
#104663=CARTESIAN_POINT('Ctrl Pts',(-9.60388492791828,24.7789806094023,
4.60913836499738));
#104664=CARTESIAN_POINT('Ctrl Pts',(-9.60384169381251,24.7789837207695,
4.60912292350905));
#104665=CARTESIAN_POINT('Ctrl Pts',(-9.60382033091821,24.7789852581429,
4.60911529284419));
#104666=CARTESIAN_POINT('Ctrl Pts',(-9.6037780958261,24.7789882975381,4.6091002054116));
#104667=CARTESIAN_POINT('Ctrl Pts',(-9.60375722365093,24.7789897995591,
4.60909274868355));
#104668=CARTESIAN_POINT('Ctrl Pts',(-9.60371595334081,24.778992769451,4.60907800326786));
#104669=CARTESIAN_POINT('Ctrl Pts',(-9.60369555515816,24.7789942373262,
4.60907071459299));
#104670=CARTESIAN_POINT('Ctrl Pts',(-9.60365521676299,24.7789971400851,
4.6090562996301));
#104671=CARTESIAN_POINT('Ctrl Pts',(-9.60363527654893,24.7789985749698,
4.60904917336967));
#104672=CARTESIAN_POINT('Ctrl Pts',(-9.60359583877762,24.7790014128522,
4.60903507784664));
#104673=CARTESIAN_POINT('Ctrl Pts',(-9.6035763412221,24.7790028158506,4.60902810861126));
#104674=CARTESIAN_POINT('Ctrl Pts',(-9.60027553212759,24.7792403315723,
4.60784816430784));
#104675=CARTESIAN_POINT('Ctrl Pts',(-9.59699939059866,24.779475611179,4.60666061417405));
#104676=CARTESIAN_POINT('Ctrl Pts',(-9.59013873376859,24.7799674441173,
4.60413922673925));
#104677=CARTESIAN_POINT('Ctrl Pts',(-9.58655533969737,24.7802238318712,
4.60280243171948));
#104678=CARTESIAN_POINT('Ctrl Pts',(-9.57717070350627,24.7808941319978,
4.5992492955189));
#104679=CARTESIAN_POINT('Ctrl Pts',(-9.57138028382695,24.7813065467064,
4.5970044532125));
#104680=CARTESIAN_POINT('Ctrl Pts',(-9.52772179376773,24.7844091653559,
4.57968037391898));
#104681=CARTESIAN_POINT('Ctrl Pts',(-9.49063763219807,24.7870056159933,
4.56268861581218));
#104682=CARTESIAN_POINT('Ctrl Pts',(-9.35961276667372,24.7962913842629,
4.49421488816823));
#104683=CARTESIAN_POINT('Ctrl Pts',(-9.27193149659004,24.8027742899929,
4.43192005708362));
#104684=CARTESIAN_POINT('Ctrl Pts',(-9.18215429882838,24.810794602548,4.34763309535276));
#104685=CARTESIAN_POINT('Ctrl Pts',(-9.17066210892228,24.8118504202317,
4.33639229921493));
#104686=CARTESIAN_POINT('Ctrl Pts',(-9.15488697911064,24.8133436908852,
4.32031739833469));
#104687=CARTESIAN_POINT('Ctrl Pts',(-9.1504079253251,24.8137728288019,4.31567760544476));
#104688=CARTESIAN_POINT('Ctrl Pts',(-9.14269129747648,24.8145213380263,
4.30755153657204));
#104689=CARTESIAN_POINT('Ctrl Pts',(-9.13943629395877,24.8148399713782,
4.30408196247375));
#104690=CARTESIAN_POINT('Ctrl Pts',(-9.13268243933127,24.815507268165,4.29679490829198));
#104691=CARTESIAN_POINT('Ctrl Pts',(-9.12918757255436,24.8158560866118,
4.29297389091868));
#104692=CARTESIAN_POINT('Ctrl Pts',(-9.12094573429126,24.8166871949752,
4.28384270810267));
#104693=CARTESIAN_POINT('Ctrl Pts',(-9.11622155757175,24.8171704022077,
4.27851233387102));
#104694=CARTESIAN_POINT('Ctrl Pts',(-9.10040013098923,24.8188122601994,
4.26033112934403));
#104695=CARTESIAN_POINT('Ctrl Pts',(-9.08953296617723,24.8199800456983,
4.24728380099273));
#104696=CARTESIAN_POINT('Ctrl Pts',(-9.0640900145919,24.8228145551844,4.21535742015004));
#104697=CARTESIAN_POINT('Ctrl Pts',(-9.04979871954204,24.8244913992758,
4.19626225746629));
#104698=CARTESIAN_POINT('Ctrl Pts',(-8.97328829329972,24.8339608209114,
4.08728723908584));
#104699=CARTESIAN_POINT('Ctrl Pts',(-8.92325344280207,24.8421525464417,
3.98954522966905));
#104700=CARTESIAN_POINT('Ctrl Pts',(-8.88740821192768,24.85,3.88630891215973));
#104701=CARTESIAN_POINT('',(-9.99063336962939,24.85,4.67771275306651));
#104702=CARTESIAN_POINT('Origin',(-10.,24.85,3.5));
#104703=CARTESIAN_POINT('',(-11.1772880725875,24.7251753227386,3.4996108612957));
#104704=CARTESIAN_POINT('Ctrl Pts',(-11.1777499294838,24.7254411208432,
3.49959244531692));
#104705=CARTESIAN_POINT('Ctrl Pts',(-11.177755138959,24.7264977516175,3.51464676629648));
#104706=CARTESIAN_POINT('Ctrl Pts',(-11.1774717063853,24.7275454784774,
3.52970041717589));
#104707=CARTESIAN_POINT('Ctrl Pts',(-11.176514931794,24.7292825855865,3.5548657671731));
#104708=CARTESIAN_POINT('Ctrl Pts',(-11.1759996106182,24.7299769475529,
3.56498126463823));
#104709=CARTESIAN_POINT('Ctrl Pts',(-11.1750130228752,24.7310313066549,
3.58042410351479));
#104710=CARTESIAN_POINT('Ctrl Pts',(-11.1746358678129,24.7313943558125,
3.58575674975724));
#104711=CARTESIAN_POINT('Ctrl Pts',(-11.1738818741506,24.7320542601341,
3.59547667609124));
#104712=CARTESIAN_POINT('Ctrl Pts',(-11.1735167171838,24.7323514918127,
3.59986473645066));
#104713=CARTESIAN_POINT('Ctrl Pts',(-11.1727548552257,24.7329309160681,
3.60843792390885));
#104714=CARTESIAN_POINT('Ctrl Pts',(-11.1723603351763,24.7332131755401,
3.61262317314638));
#104715=CARTESIAN_POINT('Ctrl Pts',(-11.1714052847838,24.7338580797188,
3.62220540717993));
#104716=CARTESIAN_POINT('Ctrl Pts',(-11.1708298467939,24.7342202311984,
3.6276008400157));
#104717=CARTESIAN_POINT('Ctrl Pts',(-11.1691539993501,24.7352074834157,
3.64234685982795));
#104718=CARTESIAN_POINT('Ctrl Pts',(-11.1679787057468,24.7358301342547,
3.65168867624558));
#104719=CARTESIAN_POINT('Ctrl Pts',(-11.1627134868986,24.7383627554835,
3.68983954298161));
#104720=CARTESIAN_POINT('Ctrl Pts',(-11.1576684580273,24.7402416619903,
3.71850783311194));
#104721=CARTESIAN_POINT('Ctrl Pts',(-11.1292884404647,24.7488563029863,
3.850841905454));
#104722=CARTESIAN_POINT('Ctrl Pts',(-11.0930608022952,24.7551722476283,
3.95121806583432));
#104723=CARTESIAN_POINT('Ctrl Pts',(-11.0287903288429,24.7639539015492,
4.07423517106098));
#104724=CARTESIAN_POINT('Ctrl Pts',(-11.0125214477603,24.766052892499,4.1024578178727));
#104725=CARTESIAN_POINT('Ctrl Pts',(-10.9920344070001,24.7686064114546,
4.13481948699576));
#104726=CARTESIAN_POINT('Ctrl Pts',(-10.9889271063245,24.7689914956883,
4.13964929499859));
#104727=CARTESIAN_POINT('Ctrl Pts',(-10.9840731037844,24.7695900030116,
4.14707416339296));
#104728=CARTESIAN_POINT('Ctrl Pts',(-10.9823511581631,24.7698017482794,
4.14968534558134));
#104729=CARTESIAN_POINT('Ctrl Pts',(-10.9790877091956,24.7702020135359,
4.15459144700913));
#104730=CARTESIAN_POINT('Ctrl Pts',(-10.9775485453295,24.7703903596084,
4.15688777268823));
#104731=CARTESIAN_POINT('Ctrl Pts',(-10.9740299880956,24.7708199052824,
4.1620974630601));
#104732=CARTESIAN_POINT('Ctrl Pts',(-10.9720455930406,24.7710614381586,
4.16500739283712));
#104733=CARTESIAN_POINT('Ctrl Pts',(-10.9668676986757,24.7716897286675,
4.17252759723005));
#104734=CARTESIAN_POINT('Ctrl Pts',(-10.9636543138194,24.7720777558613,
4.17712397395204));
#104735=CARTESIAN_POINT('Ctrl Pts',(-10.942303085645,24.7746428588401,4.20720463085144));
#104736=CARTESIAN_POINT('Ctrl Pts',(-10.923190669809,24.7768772868424,4.23197819458875));
#104737=CARTESIAN_POINT('Ctrl Pts',(-10.880005956051,24.7817557488319,4.28356942238958));
#104738=CARTESIAN_POINT('Ctrl Pts',(-10.8556416763558,24.7844079493489,
4.31010406952791));
#104739=CARTESIAN_POINT('Ctrl Pts',(-10.7942681953594,24.7907991994936,
4.37108247915779));
#104740=CARTESIAN_POINT('Ctrl Pts',(-10.7561796642247,24.794537550629,4.40434474924715));
#104741=CARTESIAN_POINT('Ctrl Pts',(-10.6660180958196,24.8028110218165,
4.4733907771597));
#104742=CARTESIAN_POINT('Ctrl Pts',(-10.6129611859212,24.8072976730081,
4.50764608395494));
#104743=CARTESIAN_POINT('Ctrl Pts',(-10.5480076864262,24.8123730922583,
4.54254328992698));
#104744=CARTESIAN_POINT('Ctrl Pts',(-10.5385389146906,24.8131034392807,
4.54746588737711));
#104745=CARTESIAN_POINT('Ctrl Pts',(-10.5228662783851,24.8142972168318,
4.55534502160448));
#104746=CARTESIAN_POINT('Ctrl Pts',(-10.5167012833396,24.8147630257581,
4.55837708150735));
#104747=CARTESIAN_POINT('Ctrl Pts',(-10.5055373821334,24.8155999278717,
4.56374689920736));
#104748=CARTESIAN_POINT('Ctrl Pts',(-10.5005479463032,24.8159716068183,
4.56610377795259));
#104749=CARTESIAN_POINT('Ctrl Pts',(-10.4898274131765,24.816765305957,4.57107602443963));
#104750=CARTESIAN_POINT('Ctrl Pts',(-10.4840915072767,24.8171869894317,
4.57368066003593));
#104751=CARTESIAN_POINT('Ctrl Pts',(-10.4683589149601,24.8183357350052,
4.58067301635831));
#104752=CARTESIAN_POINT('Ctrl Pts',(-10.4583215383363,24.8190600242207,
4.58496802739729));
#104753=CARTESIAN_POINT('Ctrl Pts',(-10.3978096110724,24.8233784268121,
4.60987154956482));
#104754=CARTESIAN_POINT('Ctrl Pts',(-10.3460108542058,24.8268724573501,
4.62709570526503));
#104755=CARTESIAN_POINT('Ctrl Pts',(-10.2278172088294,24.8346155777747,
4.65747649500275));
#104756=CARTESIAN_POINT('Ctrl Pts',(-10.1611131367921,24.8388311140296,
4.66862920440857));
#104757=CARTESIAN_POINT('Ctrl Pts',(-10.0704127195105,24.8447069487161,
4.67587786445373));
#104758=CARTESIAN_POINT('Ctrl Pts',(-10.0469510018944,24.8462402573117,
4.67704807608586));
#104759=CARTESIAN_POINT('Ctrl Pts',(-10.0175322526035,24.8481948932828,
4.67763448103727));
#104760=CARTESIAN_POINT('Ctrl Pts',(-10.011592342945,24.8485911865705,4.67770792881751));
#104761=CARTESIAN_POINT('Ctrl Pts',(-10.0029659410544,24.8491693767408,
4.67774932906654));
#104762=CARTESIAN_POINT('Ctrl Pts',(-10.0002796214192,24.8493498039276,
4.6777530303329));
#104763=CARTESIAN_POINT('Ctrl Pts',(-9.99526997388056,24.849687011182,4.67774279339686));
#104764=CARTESIAN_POINT('Ctrl Pts',(-9.99295662562748,24.8498430187347,
4.67773123047548));
#104765=CARTESIAN_POINT('Ctrl Pts',(-9.99063336962939,24.85,4.67771275306651));
#104766=CARTESIAN_POINT('Ctrl Pts',(-9.81111852688625,24.5869833862071,
2.3377666957199));
#104767=CARTESIAN_POINT('Ctrl Pts',(-9.85758225208399,24.5899974122869,
2.33012084493045));
#104768=CARTESIAN_POINT('Ctrl Pts',(-9.90447666972509,24.5929707932202,
2.32524743637886));
#104769=CARTESIAN_POINT('Ctrl Pts',(-9.95144430870241,24.5959479723899,
2.32319483958211));
#104770=CARTESIAN_POINT('Ctrl Pts',(-9.99850100085462,24.5989307964518,
2.3211383509512));
#104771=CARTESIAN_POINT('Ctrl Pts',(-10.0456310486077,24.6019179804784,
2.32191398031387));
#104772=CARTESIAN_POINT('Ctrl Pts',(-10.0924623693727,24.6049688698172,
2.32552525705089));
#104773=CARTESIAN_POINT('Ctrl Pts',(-10.1265100711087,24.6071869531115,
2.32815075791698));
#104774=CARTESIAN_POINT('Ctrl Pts',(-10.1603995448042,24.609439100678,2.33227422482323));
#104775=CARTESIAN_POINT('Ctrl Pts',(-10.1939848786067,24.6117498453562,
2.33787895204113));
#104776=CARTESIAN_POINT('Ctrl Pts',(-10.1940023012851,24.6117510440747,
2.33788185954119));
#104777=CARTESIAN_POINT('Ctrl Pts',(-10.1940197238821,24.611752242809,2.33788476743961));
#104778=CARTESIAN_POINT('Ctrl Pts',(-10.1940371463977,24.6117534415591,
2.33788767573637));
#104779=CARTESIAN_POINT('Ctrl Pts',(-10.2367172506162,24.614690031112,2.34501215831637));
#104780=CARTESIAN_POINT('Ctrl Pts',(-10.2790701141076,24.6177291627391,
2.35456197197645));
#104781=CARTESIAN_POINT('Ctrl Pts',(-10.3208151990413,24.6208120221985,
2.3664622507935));
#104782=CARTESIAN_POINT('Ctrl Pts',(-10.3259059137602,24.6211879696436,
2.36791346174752));
#104783=CARTESIAN_POINT('Ctrl Pts',(-10.3309875465595,24.6215645673753,
2.3693995805412));
#104784=CARTESIAN_POINT('Ctrl Pts',(-10.3360595537553,24.6219417087332,
2.370920431718));
#104785=CARTESIAN_POINT('Ctrl Pts',(-10.3809908088543,24.6252826808388,
2.3843931555439));
#104786=CARTESIAN_POINT('Ctrl Pts',(-10.4251713239778,24.6286657673699,
2.4005953434563));
#104787=CARTESIAN_POINT('Ctrl Pts',(-10.4682696908998,24.6320320939319,
2.41939152864877));
#104788=CARTESIAN_POINT('Ctrl Pts',(-10.5113259988402,24.6353951353516,
2.43816937095576));
#104789=CARTESIAN_POINT('Ctrl Pts',(-10.5533024644096,24.6387411565441,
2.4595359027969));
#104790=CARTESIAN_POINT('Ctrl Pts',(-10.5938896487488,24.6420331412891,
2.48332486996171));
#104791=CARTESIAN_POINT('Ctrl Pts',(-10.6344549721495,24.6453233529159,
2.50710102398963));
#104792=CARTESIAN_POINT('Ctrl Pts',(-10.6736325624402,24.6485594959849,
2.53329695268629));
#104793=CARTESIAN_POINT('Ctrl Pts',(-10.7111326005979,24.6517290789581,
2.56171762936817));
#104794=CARTESIAN_POINT('Ctrl Pts',(-10.7486288368082,24.6548983405826,
2.59013542461513));
#104795=CARTESIAN_POINT('Ctrl Pts',(-10.7844477718312,24.6580011120596,
2.62077757904407));
#104796=CARTESIAN_POINT('Ctrl Pts',(-10.8183190897181,24.6610496044806,
2.65341995634774));
#104797=CARTESIAN_POINT('Ctrl Pts',(-10.8522250946285,24.6641012188093,
2.6860957621383));
#104798=CARTESIAN_POINT('Ctrl Pts',(-10.8841792539821,24.6670986487837,
2.72077604476894));
#104799=CARTESIAN_POINT('Ctrl Pts',(-10.9139323064,24.6700769647453,2.75720509748594));
#104800=CARTESIAN_POINT('Ctrl Pts',(-10.9437036423241,24.6730571109076,
2.7936565361686));
#104801=CARTESIAN_POINT('Ctrl Pts',(-10.9712707281535,24.6760185377855,
2.83185910709269));
#104802=CARTESIAN_POINT('Ctrl Pts',(-10.9964107211274,24.6790146045598,
2.87152292044512));
#104803=CARTESIAN_POINT('Ctrl Pts',(-11.0195880748556,24.6817767731687,
2.90809024300694));
#104804=CARTESIAN_POINT('Ctrl Pts',(-11.0407025532645,24.6845689829593,
2.94590008222233));
#104805=CARTESIAN_POINT('Ctrl Pts',(-11.0596054484233,24.6874407681847,
2.98469547749695));
#104806=CARTESIAN_POINT('Ctrl Pts',(-11.0612431100617,24.6876895667131,
2.98805653568687));
#104807=CARTESIAN_POINT('Ctrl Pts',(-11.0628642004715,24.6879389625114,
2.99142500702423));
#104808=CARTESIAN_POINT('Ctrl Pts',(-11.0644686388172,24.68818898779,2.9948007338952));
#104809=CARTESIAN_POINT('Ctrl Pts',(-11.069938513088,24.6890413775638,3.00630931046723));
#104810=CARTESIAN_POINT('Ctrl Pts',(-11.0752147010818,24.6899011034306,
3.01790177900417));
#104811=CARTESIAN_POINT('Ctrl Pts',(-11.0802940068402,24.6907694454115,
3.02957106735435));
#104812=CARTESIAN_POINT('Ctrl Pts',(-11.080302334643,24.6907708691062,3.02959019979827));
#104813=CARTESIAN_POINT('Ctrl Pts',(-11.0803106619167,24.6907722928241,
3.02960933244874));
#104814=CARTESIAN_POINT('Ctrl Pts',(-11.0803189886612,24.6907737165651,
3.02962846530571));
#104815=CARTESIAN_POINT('Ctrl Pts',(-11.0980581824247,24.6938068369181,
3.07038886749672));
#104816=CARTESIAN_POINT('Ctrl Pts',(-11.1134484878215,24.6969518887715,
3.1122243160909));
#104817=CARTESIAN_POINT('Ctrl Pts',(-11.1264093147121,24.7001441311768,
3.1548603050666));
#104818=CARTESIAN_POINT('Ctrl Pts',(-11.1283581804571,24.7006241354177,
3.1612713017659));
#104819=CARTESIAN_POINT('Ctrl Pts',(-11.1302521166983,24.7011052066318,
3.16770030250139));
#104820=CARTESIAN_POINT('Ctrl Pts',(-11.1320908541742,24.7015871247156,
3.17414627226733));
#104821=CARTESIAN_POINT('Ctrl Pts',(-11.1452476288099,24.7050354079559,
3.2202693173635));
#104822=CARTESIAN_POINT('Ctrl Pts',(-11.1555788799508,24.7085263128591,
3.26726742745412));
#104823=CARTESIAN_POINT('Ctrl Pts',(-11.1630189724679,24.7119977437618,
3.31480118396534));
#104824=CARTESIAN_POINT('Ctrl Pts',(-11.163505756299,24.7122248694905,3.31791118079));
#104825=CARTESIAN_POINT('Ctrl Pts',(-11.1639801586827,24.7124519118566,
3.32102345279043));
#104826=CARTESIAN_POINT('Ctrl Pts',(-11.164442159325,24.7126788534689,3.3241378973602));
#104827=CARTESIAN_POINT('Ctrl Pts',(-11.1719266982414,24.7163553707144,
3.37459276571997));
#104828=CARTESIAN_POINT('Ctrl Pts',(-11.1761583601084,24.7200050807238,
3.42562366407079));
#104829=CARTESIAN_POINT('Ctrl Pts',(-11.177088112557,24.7235849415198,3.47682444544406));
#104830=CARTESIAN_POINT('Ctrl Pts',(-11.1772259797544,24.7241157767712,
3.48441669028381));
#104831=CARTESIAN_POINT('Ctrl Pts',(-11.1772912923578,24.724645136589,3.49201266219816));
#104832=CARTESIAN_POINT('Ctrl Pts',(-11.1772839403217,24.7251729446244,
3.49961102606475));
#104833=CARTESIAN_POINT('Origin',(-10.,13.2,3.5));
#104834=CARTESIAN_POINT('',(-11.2887076826321,24.8493336655152,2.80606944570028));
#104835=CARTESIAN_POINT('Ctrl Pts',(-11.4635,24.3883362350912,3.49999997785042));
#104836=CARTESIAN_POINT('Ctrl Pts',(-11.4635000018663,24.395579963598,3.62331606172117));
#104837=CARTESIAN_POINT('Ctrl Pts',(-11.4479149340742,24.4031789408495,
3.74617229420536));
#104838=CARTESIAN_POINT('Ctrl Pts',(-11.4135023702327,24.4112209615172,
3.87953776065764));
#104839=CARTESIAN_POINT('Ctrl Pts',(-11.4097158080832,24.4120531990573,
3.89336906389607));
#104840=CARTESIAN_POINT('Ctrl Pts',(-11.3944544626202,24.4152158225676,
3.94606133427072));
#104841=CARTESIAN_POINT('Ctrl Pts',(-11.3815703952692,24.4175055471079,
3.98449732434018));
#104842=CARTESIAN_POINT('Ctrl Pts',(-11.3635408172435,24.4202952829669,
4.03168459175159));
#104843=CARTESIAN_POINT('Ctrl Pts',(-11.3598793841164,24.4208438625688,
4.04098071408713));
#104844=CARTESIAN_POINT('Ctrl Pts',(-11.3539475279854,24.4217051345132,
4.05560041503075));
#104845=CARTESIAN_POINT('Ctrl Pts',(-11.3517402773549,24.422019927099,4.06094915423817));
#104846=CARTESIAN_POINT('Ctrl Pts',(-11.3475794328349,24.4226029604457,
4.07086477634955));
#104847=CARTESIAN_POINT('Ctrl Pts',(-11.3456342046423,24.42287147745,4.07543506046806));
#104848=CARTESIAN_POINT('Ctrl Pts',(-11.3412742813686,24.4234644773029,
4.08553562258562));
#104849=CARTESIAN_POINT('Ctrl Pts',(-11.3388485659881,24.4237885821161,
4.09106106454632));
#104850=CARTESIAN_POINT('Ctrl Pts',(-11.3317313952652,24.4247230165747,
4.10700434748986));
#104851=CARTESIAN_POINT('Ctrl Pts',(-11.3269519738796,24.4253303518495,
4.11738258469905));
#104852=CARTESIAN_POINT('Ctrl Pts',(-11.2869594721666,24.4302541468916,
4.20161359863359));
#104853=CARTESIAN_POINT('Ctrl Pts',(-11.245730053618,24.4343494708593,4.27245401872569));
#104854=CARTESIAN_POINT('Ctrl Pts',(-11.1598023548768,24.4416896338265,
4.39515953833734));
#104855=CARTESIAN_POINT('Ctrl Pts',(-11.1169837864255,24.4449552872432,
4.44805012002431));
#104856=CARTESIAN_POINT('Ctrl Pts',(-11.0295668328515,24.4512703469944,
4.54185162390309));
#104857=CARTESIAN_POINT('Ctrl Pts',(-10.9858093329547,24.4542977738486,
4.5833471592725));
#104858=CARTESIAN_POINT('Ctrl Pts',(-10.9340911712786,24.4578968947417,
4.62665790456836));
#104859=CARTESIAN_POINT('Ctrl Pts',(-10.9285232061192,24.4582846449281,
4.63125107805963));
#104860=CARTESIAN_POINT('Ctrl Pts',(-10.9201781975705,24.4588665703848,
4.63803199885728));
#104861=CARTESIAN_POINT('Ctrl Pts',(-10.9174267499958,24.4590585634451,
4.64025124580611));
#104862=CARTESIAN_POINT('Ctrl Pts',(-10.912492148537,24.4594031724113,4.64420194586975));
#104863=CARTESIAN_POINT('Ctrl Pts',(-10.910312064616,24.4595555178638,4.64593715312667));
#104864=CARTESIAN_POINT('Ctrl Pts',(-10.9055693978202,24.4598871635893,
4.64968993768724));
#104865=CARTESIAN_POINT('Ctrl Pts',(-10.9030050561334,24.4600666200175,
4.65170515118098));
#104866=CARTESIAN_POINT('Ctrl Pts',(-10.8957850234587,24.4605722196446,
4.65734014887833));
#104867=CARTESIAN_POINT('Ctrl Pts',(-10.8911142125169,24.4608996884417,
4.66094034570658));
#104868=CARTESIAN_POINT('Ctrl Pts',(-10.8628120579187,24.4628855913374,
4.68248382919634));
#104869=CARTESIAN_POINT('Ctrl Pts',(-10.8386627672836,24.4645868936193,
4.69973212397364));
#104870=CARTESIAN_POINT('Ctrl Pts',(-10.7003484769693,24.4742939808631,
4.79230392769391));
#104871=CARTESIAN_POINT('Ctrl Pts',(-10.5765835940818,24.4827631050378,
4.85207111966067));
#104872=CARTESIAN_POINT('Ctrl Pts',(-10.4394697239234,24.491123169717,4.89597640648737));
#104873=CARTESIAN_POINT('Ctrl Pts',(-10.4326180876373,24.4915386264112,
4.89811493025721));
#104874=CARTESIAN_POINT('Ctrl Pts',(-10.3863888699656,24.4943261510023,
4.91217155789038));
#104875=CARTESIAN_POINT('Ctrl Pts',(-10.3465372549996,24.4966521934943,
4.92247575411468));
#104876=CARTESIAN_POINT('Ctrl Pts',(-10.2964727829022,24.4994801231183,
4.93319125224792));
#104877=CARTESIAN_POINT('Ctrl Pts',(-10.2866226167697,24.5000320879207,
4.93519363124327));
#104878=CARTESIAN_POINT('Ctrl Pts',(-10.2710522017688,24.5008977667151,
4.93819214693685));
#104879=CARTESIAN_POINT('Ctrl Pts',(-10.2653454395408,24.5012136096911,
4.9392559698209));
#104880=CARTESIAN_POINT('Ctrl Pts',(-10.2547846627948,24.501795484248,4.94115970323365));
#104881=CARTESIAN_POINT('Ctrl Pts',(-10.2499324635919,24.5020618115898,
4.94200911199761));
#104882=CARTESIAN_POINT('Ctrl Pts',(-10.2391514052299,24.502651340826,4.94384035448484));
#104883=CARTESIAN_POINT('Ctrl Pts',(-10.2332205823806,24.5029741618651,
4.94481020389869));
#104884=CARTESIAN_POINT('Ctrl Pts',(-10.2161384625526,24.5038997795505,
4.9474956668982));
#104885=CARTESIAN_POINT('Ctrl Pts',(-10.2049729446481,24.5044996793862,
4.94911891925363));
#104886=CARTESIAN_POINT('Ctrl Pts',(-10.1189888017754,24.5090821648202,
4.96060566999701));
#104887=CARTESIAN_POINT('Ctrl Pts',(-10.0435233147649,24.512879248679,4.96479857723339));
#104888=CARTESIAN_POINT('Ctrl Pts',(-9.88163229136688,24.520844135936,4.96126494639229));
#104889=CARTESIAN_POINT('Ctrl Pts',(-9.79554223507775,24.5249689316798,
4.95172386410779));
#104890=CARTESIAN_POINT('Ctrl Pts',(-9.69573501150379,24.5300355703903,
4.93160443934707));
#104891=CARTESIAN_POINT('Ctrl Pts',(-9.68071823376365,24.530805965361,4.92833034948654));
#104892=CARTESIAN_POINT('Ctrl Pts',(-9.63259659367964,24.5333083496372,
4.91704165517477));
#104893=CARTESIAN_POINT('Ctrl Pts',(-9.59972109482159,24.5350694079443,
4.9081082236652));
#104894=CARTESIAN_POINT('Ctrl Pts',(-9.5616180561903,24.5372024727957,4.8963121211659));
#104895=CARTESIAN_POINT('Ctrl Pts',(-9.55605687438356,24.5375161260877,
4.89455396716141));
#104896=CARTESIAN_POINT('Ctrl Pts',(-9.54707851662153,24.5380265052009,
4.89165633491366));
#104897=CARTESIAN_POINT('Ctrl Pts',(-9.5436547230652,24.5382220763641,4.89053738254849));
#104898=CARTESIAN_POINT('Ctrl Pts',(-9.53757649539273,24.5385710086285,
4.88852605114987));
#104899=CARTESIAN_POINT('Ctrl Pts',(-9.53492045651033,24.538724077553,4.88763868149646));
#104900=CARTESIAN_POINT('Ctrl Pts',(-9.52920025562792,24.5390550287183,
4.88570932203383));
#104901=CARTESIAN_POINT('Ctrl Pts',(-9.5261370379425,24.5392330527241,4.88466480320889));
#104902=CARTESIAN_POINT('Ctrl Pts',(-9.51765033131726,24.5397284337715,
4.8817394830145));
#104903=CARTESIAN_POINT('Ctrl Pts',(-9.51223446587876,24.5400470203795,
4.87983694083723));
#104904=CARTESIAN_POINT('Ctrl Pts',(-9.48166789665751,24.5418584323435,
4.86889675250147));
#104905=CARTESIAN_POINT('Ctrl Pts',(-9.45675873963097,24.543385765376,4.85920389838867));
#104906=CARTESIAN_POINT('Ctrl Pts',(-9.37704677461605,24.5484092102983,
4.82564458406915));
#104907=CARTESIAN_POINT('Ctrl Pts',(-9.32343814439683,24.5519977727624,
4.7991026054702));
#104908=CARTESIAN_POINT('Ctrl Pts',(-9.1701248636585,24.5626337651942,4.71112709619329));
#104909=CARTESIAN_POINT('Ctrl Pts',(-9.07597529543186,24.5696254019425,
4.64092463223607));
#104910=CARTESIAN_POINT('Ctrl Pts',(-8.97925383984117,24.5770862114638,
4.54889500252843));
#104911=CARTESIAN_POINT('Ctrl Pts',(-8.96751546543043,24.5779980380897,
4.53734235752755));
#104912=CARTESIAN_POINT('Ctrl Pts',(-8.95143117755654,24.5792568712628,
4.52096900141471));
#104913=CARTESIAN_POINT('Ctrl Pts',(-8.94691885059354,24.5796110954741,
4.51631411084658));
#104914=CARTESIAN_POINT('Ctrl Pts',(-8.93917155568424,24.5802211774092,
4.50821504939365));
#104915=CARTESIAN_POINT('Ctrl Pts',(-8.93592208732818,24.5804776560974,
4.50478493747898));
#104916=CARTESIAN_POINT('Ctrl Pts',(-8.92921402783208,24.5810083777484,
4.49763492826492));
#104917=CARTESIAN_POINT('Ctrl Pts',(-8.92575807271136,24.5812825069712,
4.49391263742694));
#104918=CARTESIAN_POINT('Ctrl Pts',(-8.9176823337168,24.5819247888391,4.48512320841413));
#104919=CARTESIAN_POINT('Ctrl Pts',(-8.91307862203848,24.5822922639096,
4.48004142096585));
#104920=CARTESIAN_POINT('Ctrl Pts',(-8.89810036189819,24.5834924193799,
4.46327236724111));
#104921=CARTESIAN_POINT('Ctrl Pts',(-8.88787708262172,24.5843188550253,
4.45145105355931));
#104922=CARTESIAN_POINT('Ctrl Pts',(-8.82905446905561,24.5891218810937,
4.38118990268194));
#104923=CARTESIAN_POINT('Ctrl Pts',(-8.7848757227542,24.5929177281757,4.31919706638321));
#104924=CARTESIAN_POINT('Ctrl Pts',(-8.70345403042831,24.6006596570788,
4.18375918724548));
#104925=CARTESIAN_POINT('Ctrl Pts',(-8.66718379933786,24.6045806957516,
4.11004755984359));
#104926=CARTESIAN_POINT('Ctrl Pts',(-8.63392977878911,24.6091291859393,
4.02513690643022));
#104927=CARTESIAN_POINT('Ctrl Pts',(-8.63066084081614,24.6095894608739,
4.01655288459715));
#104928=CARTESIAN_POINT('Ctrl Pts',(-8.62591918267693,24.6102778839544,
4.00374021046289));
#104929=CARTESIAN_POINT('Ctrl Pts',(-8.62438468157175,24.610504076599,3.99953457068266));
#104930=CARTESIAN_POINT('Ctrl Pts',(-8.61157673757472,24.6124216633605,
3.96392498613783));
#104931=CARTESIAN_POINT('Ctrl Pts',(-8.60136179717959,24.6141481840516,
3.93215321390143));
#104932=CARTESIAN_POINT('Ctrl Pts',(-8.59065790584223,24.6162424510754,
3.89448789498059));
#104933=CARTESIAN_POINT('Ctrl Pts',(-8.58910680518603,24.6165541441918,
3.88890388048037));
#104934=CARTESIAN_POINT('Ctrl Pts',(-8.58664891288582,24.6170618547681,
3.8798471217667));
#104935=CARTESIAN_POINT('Ctrl Pts',(-8.58572164321746,24.6172567344192,
3.87637994146533));
#104936=CARTESIAN_POINT('Ctrl Pts',(-8.58409716027383,24.6176042139065,
3.87021502175787));
#104937=CARTESIAN_POINT('Ctrl Pts',(-8.58339487498002,24.6177565231765,
3.86751861665172));
#104938=CARTESIAN_POINT('Ctrl Pts',(-8.58190269489624,24.6180847051419,
3.86172160675026));
#104939=CARTESIAN_POINT('Ctrl Pts',(-8.58111526902468,24.6182607144955,
3.85862042235416));
#104940=CARTESIAN_POINT('Ctrl Pts',(-8.5789568448732,24.6187510792355,3.85000132629544));
#104941=CARTESIAN_POINT('Ctrl Pts',(-8.57760783866035,24.6190666595984,
3.84447803167807));
#104942=CARTESIAN_POINT('Ctrl Pts',(-8.57012627559957,24.6208692607581,
3.81305257397498));
#104943=CARTESIAN_POINT('Ctrl Pts',(-8.56466947326265,24.6223910501948,
3.78699629919708));
#104944=CARTESIAN_POINT('Ctrl Pts',(-8.54932364263577,24.6273957936799,
3.70226284497424));
#104945=CARTESIAN_POINT('Ctrl Pts',(-8.54230133417534,24.6309723995269,
3.64312920424746));
#104946=CARTESIAN_POINT('Ctrl Pts',(-8.53207499372629,24.6417452004105,
3.464690987229));
#104947=CARTESIAN_POINT('Ctrl Pts',(-8.53982592728949,24.6488867605369,
3.34523565727496));
#104948=CARTESIAN_POINT('Ctrl Pts',(-8.5650444587117,24.6564706953814,3.21189487508679));
#104949=CARTESIAN_POINT('Ctrl Pts',(-8.56836792683034,24.6573800027911,
3.19580991689321));
#104950=CARTESIAN_POINT('Ctrl Pts',(-8.57337056494595,24.6586338798893,
3.17350011417296));
#104951=CARTESIAN_POINT('Ctrl Pts',(-8.57482106808563,24.6589857107325,
3.16722570065227));
#104952=CARTESIAN_POINT('Ctrl Pts',(-8.57739807127232,24.6595911519306,
3.15640439105564));
#104953=CARTESIAN_POINT('Ctrl Pts',(-8.57850506558081,24.6598453837492,
3.15185298760238));
#104954=CARTESIAN_POINT('Ctrl Pts',(-8.58084515730162,24.6603709560869,
3.1424289661995));
#104955=CARTESIAN_POINT('Ctrl Pts',(-8.58208154456644,24.6606421868409,
3.13755722329685));
#104956=CARTESIAN_POINT('Ctrl Pts',(-8.58504173066293,24.6612767747781,
3.12614019124224));
#104957=CARTESIAN_POINT('Ctrl Pts',(-8.58678589489024,24.6616394700238,
3.11960026840541));
#104958=CARTESIAN_POINT('Ctrl Pts',(-8.59263318847584,24.6628198925167,
3.0982706489947));
#104959=CARTESIAN_POINT('Ctrl Pts',(-8.59692368266008,24.6636315605696,
3.08353309255072));
#104960=CARTESIAN_POINT('Ctrl Pts',(-8.62061907680284,24.6678479460841,
3.00666776536701));
#104961=CARTESIAN_POINT('Ctrl Pts',(-8.64392146022601,24.6711230271572,
2.94581531298684));
#104962=CARTESIAN_POINT('Ctrl Pts',(-8.71120619595036,24.6790336963597,
2.80003090210626));
#104963=CARTESIAN_POINT('Ctrl Pts',(-8.75959512102653,24.6835644107795,
2.71747821255996));
#104964=CARTESIAN_POINT('Ctrl Pts',(-8.84147816930817,24.6905304984309,
2.60468519608415));
#104965=CARTESIAN_POINT('Ctrl Pts',(-8.86886636110479,24.6927757703943,
2.57032401669929));
#104966=CARTESIAN_POINT('Ctrl Pts',(-8.90221808844528,24.6954835989025,
2.53213991235389));
#104967=CARTESIAN_POINT('Ctrl Pts',(-8.90671636453008,24.6958483040477,
2.52706158292328));
#104968=CARTESIAN_POINT('Ctrl Pts',(-8.9135767666852,24.6964040823174,2.51942418206164));
#104969=CARTESIAN_POINT('Ctrl Pts',(-8.9159130500219,24.6965932744127,2.51684189420938));
#104970=CARTESIAN_POINT('Ctrl Pts',(-8.9201300306212,24.696934681482,2.51221418313363));
#104971=CARTESIAN_POINT('Ctrl Pts',(-8.92200735548343,24.6970866438092,
2.51016575689477));
#104972=CARTESIAN_POINT('Ctrl Pts',(-8.92612155707991,24.6974196164102,
2.50570216924225));
#104973=CARTESIAN_POINT('Ctrl Pts',(-8.92836073875178,24.6976007986044,
2.50328921961814));
#104974=CARTESIAN_POINT('Ctrl Pts',(-8.93472158718561,24.6981153156287,
2.49648096169963));
#104975=CARTESIAN_POINT('Ctrl Pts',(-8.93886223483111,24.6984500469811,
2.49210357784372));
#104976=CARTESIAN_POINT('Ctrl Pts',(-8.96514761182479,24.7005729972829,
2.46465688362201));
#104977=CARTESIAN_POINT('Ctrl Pts',(-8.98801494050295,24.7024110248755,
2.44229457314978));
#104978=CARTESIAN_POINT('Ctrl Pts',(-9.06913004502535,24.7088449214015,
2.36801060646379));
#104979=CARTESIAN_POINT('Ctrl Pts',(-9.13078472063797,24.7135840159466,
2.32000722160854));
#104980=CARTESIAN_POINT('Ctrl Pts',(-9.28170458027993,24.7244392028596,
2.22077670231669));
#104981=CARTESIAN_POINT('Ctrl Pts',(-9.37314312970547,24.7304734505406,
2.17356958565135));
#104982=CARTESIAN_POINT('Ctrl Pts',(-9.47872953172093,24.7367537743011,
2.13243892198275));
#104983=CARTESIAN_POINT('Ctrl Pts',(-9.48871864341625,24.7373418199948,
2.12867305645963));
#104984=CARTESIAN_POINT('Ctrl Pts',(-9.50483337108708,24.7382808602949,
2.12279841371202));
#104985=CARTESIAN_POINT('Ctrl Pts',(-9.51093321359506,24.7386341189606,
2.12062047282893));
#104986=CARTESIAN_POINT('Ctrl Pts',(-9.52181242709276,24.7392603271643,
2.11681730217711));
#104987=CARTESIAN_POINT('Ctrl Pts',(-9.52658609819783,24.7395337934034,
2.11517618127699));
#104988=CARTESIAN_POINT('Ctrl Pts',(-9.53657714288246,24.7401034547862,
2.11179910009288));
#104989=CARTESIAN_POINT('Ctrl Pts',(-9.54179600802381,24.740399495334,2.11006777652027));
#104990=CARTESIAN_POINT('Ctrl Pts',(-9.55544474031845,24.7411698138853,
2.10562512846453));
#104991=CARTESIAN_POINT('Ctrl Pts',(-9.5638897461,24.7416425648028,2.10296080500888));
#104992=CARTESIAN_POINT('Ctrl Pts',(-9.60161143856802,24.7437375506052,
2.09143533247172));
#104993=CARTESIAN_POINT('Ctrl Pts',(-9.63113854289351,24.7453326734003,
2.08341633970984));
#104994=CARTESIAN_POINT('Ctrl Pts',(-9.76256127341549,24.7522668315409,
2.05211286210986));
#104995=CARTESIAN_POINT('Ctrl Pts',(-9.86652560519187,24.7572924626429,
2.03885655074291));
#104996=CARTESIAN_POINT('Ctrl Pts',(-10.049821750975,24.7662462257915,2.03522622605583));
#104997=CARTESIAN_POINT('Ctrl Pts',(-10.1286117379348,24.7701356663777,
2.04003411296748));
#104998=CARTESIAN_POINT('Ctrl Pts',(-10.2136108745967,24.7747166634902,
2.05215591160948));
#104999=CARTESIAN_POINT('Ctrl Pts',(-10.2205938664149,24.77509590483,2.05320338257555));
#105000=CARTESIAN_POINT('Ctrl Pts',(-10.2310693060105,24.7756695302105,
2.05485233193566));
#105001=CARTESIAN_POINT('Ctrl Pts',(-10.234567696452,24.7758618898867,2.05541604538168));
#105002=CARTESIAN_POINT('Ctrl Pts',(-10.2408116964493,24.7762066848808,
2.05644545233857));
#105003=CARTESIAN_POINT('Ctrl Pts',(-10.2435580608097,24.7763588513825,
2.05690628307582));
#105004=CARTESIAN_POINT('Ctrl Pts',(-10.2463215290558,24.7765124767258,
2.05737809711842));
#105005=CARTESIAN_POINT('Ctrl Pts',(-10.24633997186,24.7765135020118,2.05738124626981));
#105006=CARTESIAN_POINT('Ctrl Pts',(-10.2463760006676,24.7765155049964,
2.0573873989829));
#105007=CARTESIAN_POINT('Ctrl Pts',(-10.2463935866133,24.7765164826898,
2.05739040250173));
#105008=CARTESIAN_POINT('Ctrl Pts',(-10.2464279463137,24.7765183929633,
2.05739627147121));
#105009=CARTESIAN_POINT('Ctrl Pts',(-10.2464447200985,24.7765193255432,
2.05739913689714));
#105010=CARTESIAN_POINT('Ctrl Pts',(-10.2464794233633,24.7765212549957,
2.05740506579658));
#105011=CARTESIAN_POINT('Ctrl Pts',(-10.2464973528097,24.7765222518692,
2.05740812930731));
#105012=CARTESIAN_POINT('Ctrl Pts',(-10.2465330208745,24.7765242350491,
2.05741422440733));
#105013=CARTESIAN_POINT('Ctrl Pts',(-10.2465507594836,24.7765252213545,
2.05741725598776));
#105014=CARTESIAN_POINT('Ctrl Pts',(-10.2465860492748,24.776527183586,2.05742328778672));
#105015=CARTESIAN_POINT('Ctrl Pts',(-10.2466036004998,24.7765281595141,
2.05742628800551));
#105016=CARTESIAN_POINT('Ctrl Pts',(-10.2466385190393,24.776530101185,2.05743225766117));
#105017=CARTESIAN_POINT('Ctrl Pts',(-10.2466558863204,24.7765310669256,
2.05743522708548));
#105018=CARTESIAN_POINT('Ctrl Pts',(-10.246690440319,24.7765329884064,2.05744113570391));
#105019=CARTESIAN_POINT('Ctrl Pts',(-10.2467076270006,24.7765339441443,
2.05744407488523));
#105020=CARTESIAN_POINT('Ctrl Pts',(-10.2467418230542,24.7765358457994,
2.05744992355424));
#105021=CARTESIAN_POINT('Ctrl Pts',(-10.2467588324099,24.7765367917153,
2.05745283303266));
#105022=CARTESIAN_POINT('Ctrl Pts',(-10.2467926769059,24.7765386738973,
2.05745862280581));
#105023=CARTESIAN_POINT('Ctrl Pts',(-10.2468095120883,24.7765396101654,
2.0574615031014));
#105024=CARTESIAN_POINT('Ctrl Pts',(-10.24684301143,24.7765414732282,2.05746723503623));
#105025=CARTESIAN_POINT('Ctrl Pts',(-10.2468596755882,24.7765424000224,
2.05747008666916));
#105026=CARTESIAN_POINT('Ctrl Pts',(-10.246892835798,24.7765442442984,2.05747576175936));
#105027=CARTESIAN_POINT('Ctrl Pts',(-10.2469093319104,24.7765451617833,
2.05747858522112));
#105028=CARTESIAN_POINT('Ctrl Pts',(-10.2469421592163,24.7765469876168,
2.05748420449685));
#105029=CARTESIAN_POINT('Ctrl Pts',(-10.246958490336,24.776547895961,2.05748700029238));
#105030=CARTESIAN_POINT('Ctrl Pts',(-10.246990990437,24.7765497036668,2.05749256469436));
#105031=CARTESIAN_POINT('Ctrl Pts',(-10.2470071594422,24.7765506030293,
2.05749533329926));
#105032=CARTESIAN_POINT('Ctrl Pts',(-10.2470393381155,24.7765523929265,
2.05750084378281));
#105033=CARTESIAN_POINT('Ctrl Pts',(-10.2470553478132,24.7765532834625,
2.05750358566105));
#105034=CARTESIAN_POINT('Ctrl Pts',(-10.2470872108334,24.7765550558702,
2.05750904318216));
#105035=CARTESIAN_POINT('Ctrl Pts',(-10.2471030640796,24.7765559377375,
2.05751175880661));
#105036=CARTESIAN_POINT('Ctrl Pts',(-10.2471346167457,24.7765576929486,
2.05751716424087));
#105037=CARTESIAN_POINT('Ctrl Pts',(-10.2471503162071,24.7765585662944,
2.0575198540526));
#105038=CARTESIAN_POINT('Ctrl Pts',(-10.2471815640315,24.7765603046135,
2.05752520831324));
#105039=CARTESIAN_POINT('Ctrl Pts',(-10.2471971123952,24.7765611695865,
2.05752787275722));
#105040=CARTESIAN_POINT('Ctrl Pts',(-10.2472280605454,24.7765628912992,
2.05753317669935));
#105041=CARTESIAN_POINT('Ctrl Pts',(-10.2472434603715,24.7765637480408,
2.05753581619937));
#105042=CARTESIAN_POINT('Ctrl Pts',(-10.2472741141421,24.7765654534398,
2.05754107070088));
#105043=CARTESIAN_POINT('Ctrl Pts',(-10.2472893680398,24.7765663020943,
2.05754368568958));
#105044=CARTESIAN_POINT('Ctrl Pts',(-10.2506106921682,24.7767510881966,
2.05811311735182));
#105045=CARTESIAN_POINT('Ctrl Pts',(-10.2539147711035,24.7769356469184,
2.05869129262764));
#105046=CARTESIAN_POINT('Ctrl Pts',(-10.2633945038406,24.777467209496,2.06038374355463));
#105047=CARTESIAN_POINT('Ctrl Pts',(-10.2695649408737,24.7778157029102,
2.06152637482485));
#105048=CARTESIAN_POINT('Ctrl Pts',(-10.309905386508,24.78010954313,2.06926522280969));
#105049=CARTESIAN_POINT('Ctrl Pts',(-10.3438358665295,24.7821116019836,
2.07703833997617));
#105050=CARTESIAN_POINT('Ctrl Pts',(-10.4750927500418,24.7900605614435,
2.11207647409098));
#105051=CARTESIAN_POINT('Ctrl Pts',(-10.5697689891208,24.7962172688534,
2.14818300691642));
#105052=CARTESIAN_POINT('Ctrl Pts',(-10.7219531574316,24.8062743759023,
2.22507325015998));
#105053=CARTESIAN_POINT('Ctrl Pts',(-10.7816325622165,24.8102710585901,
2.26076345786754));
#105054=CARTESIAN_POINT('Ctrl Pts',(-10.8471794523685,24.8146999884512,
2.30658897239966));
#105055=CARTESIAN_POINT('Ctrl Pts',(-10.8557356383931,24.8152790883476,
2.31270920560289));
#105056=CARTESIAN_POINT('Ctrl Pts',(-10.8695022649851,24.8162125626134,
2.32278259531661));
#105057=CARTESIAN_POINT('Ctrl Pts',(-10.8747533986159,24.8165690406242,
2.32667928501118));
#105058=CARTESIAN_POINT('Ctrl Pts',(-10.8840463434081,24.817200692118,2.33367233037473));
#105059=CARTESIAN_POINT('Ctrl Pts',(-10.8880984200942,24.8174763873705,
2.33675481202467));
#105060=CARTESIAN_POINT('Ctrl Pts',(-10.8965953259198,24.8180551073032,
2.34328882623105));
#105061=CARTESIAN_POINT('Ctrl Pts',(-10.9010365056694,24.8183579475871,
2.34674498282833));
#105062=CARTESIAN_POINT('Ctrl Pts',(-10.9127247917844,24.8191559676965,
2.35594962211374));
#105063=CARTESIAN_POINT('Ctrl Pts',(-10.9199375872474,24.8196494540083,
2.36174139429228));
#105064=CARTESIAN_POINT('Ctrl Pts',(-10.9534299806413,24.8219464180653,
2.38916162396316));
#105065=CARTESIAN_POINT('Ctrl Pts',(-10.9790058968157,24.8237160800438,
2.41163502741689));
#105066=CARTESIAN_POINT('Ctrl Pts',(-11.0486162052943,24.8286040907748,
2.4772424776392));
#105067=CARTESIAN_POINT('Ctrl Pts',(-11.0907444791636,24.8316459644391,
2.52229546849885));
#105068=CARTESIAN_POINT('Ctrl Pts',(-11.1903499069329,24.839294572911,2.64329506440552));
#105069=CARTESIAN_POINT('Ctrl Pts',(-11.2434844536331,24.8438285581612,
2.72242722466037));
#105070=CARTESIAN_POINT('Ctrl Pts',(-11.2885639077417,24.8486931558207,
2.80614460752589));
#105071=CARTESIAN_POINT('',(-10.2623899083091,24.85,2.06021397908663));
#105072=CARTESIAN_POINT('Origin',(-10.,24.85,3.5));
#105073=CARTESIAN_POINT('Ctrl Pts',(-10.2623899083091,24.85,2.06021397908664));
#105074=CARTESIAN_POINT('Ctrl Pts',(-10.2594291274866,24.8498363566195,
2.05967439959548));
#105075=CARTESIAN_POINT('Ctrl Pts',(-10.256466711301,24.8496722872369,2.05914395823387));
#105076=CARTESIAN_POINT('Ctrl Pts',(-10.2495003369242,24.8492857040767,
2.05791874490304));
#105077=CARTESIAN_POINT('Ctrl Pts',(-10.2454950964487,24.8490628530452,
2.05723150803905));
#105078=CARTESIAN_POINT('Ctrl Pts',(-10.2318922187377,24.8483040924933,
2.05495574909106));
#105079=CARTESIAN_POINT('Ctrl Pts',(-10.2222817924645,24.8477648259318,
2.05344627314409));
#105080=CARTESIAN_POINT('Ctrl Pts',(-10.1366597278067,24.8429354567096,
2.04087129779938));
#105081=CARTESIAN_POINT('Ctrl Pts',(-10.0599065236917,24.8384371606082,
2.03571107639373));
#105082=CARTESIAN_POINT('Ctrl Pts',(-9.9114909712501,24.8297375046267,2.03742409576804));
#105083=CARTESIAN_POINT('Ctrl Pts',(-9.84002556585704,24.8255488279043,
2.04350711946446));
#105084=CARTESIAN_POINT('Ctrl Pts',(-9.73415547869234,24.8194489279163,
2.06040810974973));
#105085=CARTESIAN_POINT('Ctrl Pts',(-9.69923591611017,24.8174533692662,
2.06729649282874));
#105086=CARTESIAN_POINT('Ctrl Pts',(-9.65492351731635,24.8149439803839,
2.07772952557621));
#105087=CARTESIAN_POINT('Ctrl Pts',(-9.64527003937403,24.8143986904231,
2.08010643275622));
#105088=CARTESIAN_POINT('Ctrl Pts',(-9.62969205842779,24.8135209256829,
2.08411087592061));
#105089=CARTESIAN_POINT('Ctrl Pts',(-9.62375236723478,24.8131867597424,
2.08567765218341));
#105090=CARTESIAN_POINT('Ctrl Pts',(-9.61239062822369,24.8125485100706,
2.08875130067945));
#105091=CARTESIAN_POINT('Ctrl Pts',(-9.60696707107859,24.8122442608207,
2.09025213804092));
#105092=CARTESIAN_POINT('Ctrl Pts',(-9.59461306451122,24.8115521574829,
2.09374764358471));
#105093=CARTESIAN_POINT('Ctrl Pts',(-9.58768840368262,24.8111648897485,
2.09576233947958));
#105094=CARTESIAN_POINT('Ctrl Pts',(-9.56939847084298,24.8101436835533,
2.10123066129191));
#105095=CARTESIAN_POINT('Ctrl Pts',(-9.55805975092885,24.8095123166296,
2.10477164371196));
#105096=CARTESIAN_POINT('Ctrl Pts',(-9.44711984981179,24.8033497224776,
2.14090533450214));
#105097=CARTESIAN_POINT('Ctrl Pts',(-9.35124464501,24.7981709366138,2.18396996148269));
#105098=CARTESIAN_POINT('Ctrl Pts',(-9.2074362515418,24.7900845131843,2.26813332286317));
#105099=CARTESIAN_POINT('Ctrl Pts',(-9.15612277868303,24.7871179047295,
2.30270149573792));
#105100=CARTESIAN_POINT('Ctrl Pts',(-9.07312472955213,24.7819668770101,
2.36660750829619));
#105101=CARTESIAN_POINT('Ctrl Pts',(-9.04027133112096,24.7798218370941,
2.39428904757625));
#105102=CARTESIAN_POINT('Ctrl Pts',(-8.99251277724177,24.7764642644149,
2.43826321416674));
#105103=CARTESIAN_POINT('Ctrl Pts',(-8.97667927815003,24.7753078888398,
2.4535153594305));
#105104=CARTESIAN_POINT('Ctrl Pts',(-8.9573893874117,24.7738356455471,2.47295347379868));
#105105=CARTESIAN_POINT('Ctrl Pts',(-8.9536039602147,24.7735435862806,2.47681048551136));
#105106=CARTESIAN_POINT('Ctrl Pts',(-8.9476144688594,24.7730762779439,2.4829812417967));
#105107=CARTESIAN_POINT('Ctrl Pts',(-8.94539643301385,24.7729020752378,
2.48528142975762));
#105108=CARTESIAN_POINT('Ctrl Pts',(-8.94125808053997,24.7725748560262,
2.48960128431257));
#105109=CARTESIAN_POINT('Ctrl Pts',(-8.93933596065272,24.7724219786784,
2.4916192127733));
#105110=CARTESIAN_POINT('Ctrl Pts',(-8.93500671525298,24.7720755884838,
2.49619032356477));
#105111=CARTESIAN_POINT('Ctrl Pts',(-8.93260303121468,24.7718818085198,
2.49874664888472));
#105112=CARTESIAN_POINT('Ctrl Pts',(-8.92626014115257,24.7713666314852,
2.50554112952221));
#105113=CARTESIAN_POINT('Ctrl Pts',(-8.92233687401905,24.7710440414058,
2.50979400421134));
#105114=CARTESIAN_POINT('Ctrl Pts',(-8.89337719090628,24.7686342084671,
2.54156265153593));
#105115=CARTESIAN_POINT('Ctrl Pts',(-8.86937479010189,24.7664768400813,
2.56999873215808));
#105116=CARTESIAN_POINT('Ctrl Pts',(-8.7883482310404,24.7586993941512,2.67377031262303));
#105117=CARTESIAN_POINT('Ctrl Pts',(-8.73755798709282,24.7528962203545,
2.75367815763544));
#105118=CARTESIAN_POINT('Ctrl Pts',(-8.6706006785835,24.7440600485939,2.88567406886136));
#105119=CARTESIAN_POINT('Ctrl Pts',(-8.64901589062444,24.7409184795032,
2.93471973653624));
#105120=CARTESIAN_POINT('Ctrl Pts',(-8.6230749560714,24.7367160872126,3.00369817624602));
#105121=CARTESIAN_POINT('Ctrl Pts',(-8.61637362965541,24.7355799342274,
3.02269904348583));
#105122=CARTESIAN_POINT('Ctrl Pts',(-8.60542880601142,24.7336314169476,
3.0559021658724));
#105123=CARTESIAN_POINT('Ctrl Pts',(-8.60100489649089,24.7328130529847,
3.07004136745481));
#105124=CARTESIAN_POINT('Ctrl Pts',(-8.59495357559442,24.7316469384374,
3.09046505487861));
#105125=CARTESIAN_POINT('Ctrl Pts',(-8.59315219487416,24.7312932573747,
3.09669666350399));
#105126=CARTESIAN_POINT('Ctrl Pts',(-8.59009106938137,24.7306805393406,
3.10755629750223));
#105127=CARTESIAN_POINT('Ctrl Pts',(-8.58881254406872,24.7304208644429,
3.11217888492791));
#105128=CARTESIAN_POINT('Ctrl Pts',(-8.58639071393676,24.7299215642372,
3.12110572856197));
#105129=CARTESIAN_POINT('Ctrl Pts',(-8.585244288526,24.7296818350373,3.12540907637286));
#105130=CARTESIAN_POINT('Ctrl Pts',(-8.58257537698971,24.7291155787591,
3.13561443681155));
#105131=CARTESIAN_POINT('Ctrl Pts',(-8.58107007635882,24.7287896376719,
3.14152088765067));
#105132=CARTESIAN_POINT('Ctrl Pts',(-8.575895979721,24.7276454689081,3.16236615632213));
#105133=CARTESIAN_POINT('Ctrl Pts',(-8.57242577636303,24.7268339518618,
3.17735354631624));
#105134=CARTESIAN_POINT('Ctrl Pts',(-8.54073177751143,24.7189532020088,
3.32477559623948));
#105135=CARTESIAN_POINT('Ctrl Pts',(-8.53078058614313,24.7125837730757,
3.46045864479805));
#105136=CARTESIAN_POINT('Ctrl Pts',(-8.54311181185355,24.7034578039853,
3.64886156462657));
#105137=CARTESIAN_POINT('Ctrl Pts',(-8.54951165455615,24.7008456605647,
3.70190512406436));
#105138=CARTESIAN_POINT('Ctrl Pts',(-8.56309925339042,24.6968466833171,
3.77885745477992));
#105139=CARTESIAN_POINT('Ctrl Pts',(-8.56802205626959,24.6955543758325,
3.80312414779316));
#105140=CARTESIAN_POINT('Ctrl Pts',(-8.57475636307608,24.6939400496898,
3.83247791672164));
#105141=CARTESIAN_POINT('Ctrl Pts',(-8.57598380297924,24.6936510743543,
3.83769639974791));
#105142=CARTESIAN_POINT('Ctrl Pts',(-8.5779590661662,24.6931939501931,3.84589196899726));
#105143=CARTESIAN_POINT('Ctrl Pts',(-8.57868763310969,24.6930269483273,
3.84887365450549));
#105144=CARTESIAN_POINT('Ctrl Pts',(-8.58009416556339,24.6927075804416,
3.85455240104829));
#105145=CARTESIAN_POINT('Ctrl Pts',(-8.58077044850768,24.6925553165901,
3.8572498616597));
#105146=CARTESIAN_POINT('Ctrl Pts',(-8.58233499923653,24.6922060118392,
3.86341576020236));
#105147=CARTESIAN_POINT('Ctrl Pts',(-8.58322831146318,24.6920086835411,
3.86688288479015));
#105148=CARTESIAN_POINT('Ctrl Pts',(-8.58595346981265,24.6914130519202,
3.87730138884182));
#105149=CARTESIAN_POINT('Ctrl Pts',(-8.58782379238331,24.6910126417514,
3.88424247799121));
#105150=CARTESIAN_POINT('Ctrl Pts',(-8.6080231778388,24.686775995411,3.9570658750242));
#105151=CARTESIAN_POINT('Ctrl Pts',(-8.63089566489016,24.6827176243203,
4.02159376841027));
#105152=CARTESIAN_POINT('Ctrl Pts',(-8.69836500900632,24.6725707099685,
4.17653850077667));
#105153=CARTESIAN_POINT('Ctrl Pts',(-8.74795193193392,24.6664707888472,
4.26441976847686));
#105154=CARTESIAN_POINT('Ctrl Pts',(-8.83224632023054,24.6580391922193,
4.38329851656673));
#105155=CARTESIAN_POINT('Ctrl Pts',(-8.86001182765142,24.6554863607658,
4.41885390904803));
#105156=CARTESIAN_POINT('Ctrl Pts',(-8.89595055852964,24.6524394681986,
4.46073355825489));
#105157=CARTESIAN_POINT('Ctrl Pts',(-8.90260325712436,24.6518853607138,
4.46832563477504));
#105158=CARTESIAN_POINT('Ctrl Pts',(-8.91320950731871,24.6510172282972,
4.48017980742984));
#105159=CARTESIAN_POINT('Ctrl Pts',(-8.91711073153144,24.6507010834561,
4.48448812255364));
#105160=CARTESIAN_POINT('Ctrl Pts',(-8.92445670384538,24.6501116381319,
4.49250414566848));
#105161=CARTESIAN_POINT('Ctrl Pts',(-8.92789520938317,24.6498380867601,
4.49621743604652));
#105162=CARTESIAN_POINT('Ctrl Pts',(-8.93561663412909,24.6492289971289,
4.50446963312238));
#105163=CARTESIAN_POINT('Ctrl Pts',(-8.93990947702241,24.6488938793912,
4.50899914673763));
#105164=CARTESIAN_POINT('Ctrl Pts',(-8.95083950925738,24.6480493627953,
4.52038501185914));
#105165=CARTESIAN_POINT('Ctrl Pts',(-8.95751508060099,24.6475415869777,
4.52720421835969));
#105166=CARTESIAN_POINT('Ctrl Pts',(-8.9966891442227,24.6446069756169,4.56644592139786));
#105167=CARTESIAN_POINT('Ctrl Pts',(-9.03063352376917,24.6422433383268,
4.59739178513435));
#105168=CARTESIAN_POINT('Ctrl Pts',(-9.16117987816289,24.633685300483,4.70561387469747));
#105169=CARTESIAN_POINT('Ctrl Pts',(-9.26598987975165,24.6278595022033,
4.77214370741468));
#105170=CARTESIAN_POINT('Ctrl Pts',(-9.41182376773701,24.6197144978389,
4.84062852762631));
#105171=CARTESIAN_POINT('Ctrl Pts',(-9.44633523751368,24.6177804703049,
4.8552457441372));
#105172=CARTESIAN_POINT('Ctrl Pts',(-9.48734177391967,24.6154337611059,
4.87078613349755));
#105173=CARTESIAN_POINT('Ctrl Pts',(-9.49333162252724,24.6150897798904,
4.87301137392175));
#105174=CARTESIAN_POINT('Ctrl Pts',(-9.50255520585566,24.6145579871835,
4.8763693783042));
#105175=CARTESIAN_POINT('Ctrl Pts',(-9.50577874114772,24.6143717384551,
4.87753015777379));
#105176=CARTESIAN_POINT('Ctrl Pts',(-9.51168709327346,24.6140295974502,
4.87963431869737));
#105177=CARTESIAN_POINT('Ctrl Pts',(-9.51437065346074,24.6138739068898,
4.88058121308144));
#105178=CARTESIAN_POINT('Ctrl Pts',(-9.5203627398795,24.6135255933434,4.88267588836327));
#105179=CARTESIAN_POINT('Ctrl Pts',(-9.5236726129921,24.6133327426844,4.88381961737125));
#105180=CARTESIAN_POINT('Ctrl Pts',(-9.53334725792986,24.6127677974792,
4.88712387576559));
#105181=CARTESIAN_POINT('Ctrl Pts',(-9.53972276040559,24.6123939291749,
4.88925242040763));
#105182=CARTESIAN_POINT('Ctrl Pts',(-9.58432240659645,24.6097686921195,
4.90380189305999));
#105183=CARTESIAN_POINT('Ctrl Pts',(-9.62302644756556,24.6074404703867,
4.9146865424151));
#105184=CARTESIAN_POINT('Ctrl Pts',(-9.75920354549396,24.5991877266641,
4.94699827364544));
#105185=CARTESIAN_POINT('Ctrl Pts',(-9.8583829156248,24.5930905596194,4.96004549770521));
#105186=CARTESIAN_POINT('Ctrl Pts',(-10.0220096834828,24.583415024782,4.96472960852542));
#105187=CARTESIAN_POINT('Ctrl Pts',(-10.0859542143189,24.5797239646815,
4.96237162434377));
#105188=CARTESIAN_POINT('Ctrl Pts',(-10.1647329946187,24.5753089594819,
4.95427932492971));
#105189=CARTESIAN_POINT('Ctrl Pts',(-10.1798945711884,24.5744651323343,
4.95248176661586));
#105190=CARTESIAN_POINT('Ctrl Pts',(-10.2017665091955,24.573255985346,4.94954088811324));
#105191=CARTESIAN_POINT('Ctrl Pts',(-10.2085010349554,24.5728847991195,
4.9485875296794));
#105192=CARTESIAN_POINT('Ctrl Pts',(-10.2202522670661,24.5722390050332,
4.94684034448711));
#105193=CARTESIAN_POINT('Ctrl Pts',(-10.2252719048963,24.5719637547877,
4.9460672921226));
#105194=CARTESIAN_POINT('Ctrl Pts',(-10.2349818645042,24.5714324545567,
4.9445201176456));
#105195=CARTESIAN_POINT('Ctrl Pts',(-10.2396726328913,24.5711763069097,
4.94374924301355));
#105196=CARTESIAN_POINT('Ctrl Pts',(-10.2508358201856,24.5705679179475,
4.94185879528529));
#105197=CARTESIAN_POINT('Ctrl Pts',(-10.2573046527188,24.5702163294641,
4.9407184707012));
#105198=CARTESIAN_POINT('Ctrl Pts',(-10.2804258077683,24.5689629438389,
4.93648198575687));
#105199=CARTESIAN_POINT('Ctrl Pts',(-10.2970321296506,24.5680688368206,
4.93314028421529));
#105200=CARTESIAN_POINT('Ctrl Pts',(-10.4232811516126,24.5613107676496,
4.90544633022203));
#105201=CARTESIAN_POINT('Ctrl Pts',(-10.5298502132546,24.5558721878848,
4.86883446621369));
#105202=CARTESIAN_POINT('Ctrl Pts',(-10.7102209707958,24.5461494729348,
4.78261117248292));
#105203=CARTESIAN_POINT('Ctrl Pts',(-10.7856900925438,24.5418802834471,
4.73781762438034));
#105204=CARTESIAN_POINT('Ctrl Pts',(-10.8639450952309,24.5367548153914,
4.68131755219346));
#105205=CARTESIAN_POINT('Ctrl Pts',(-10.8711501083713,24.5362758105037,
4.67601435681554));
#105206=CARTESIAN_POINT('Ctrl Pts',(-10.8813941578492,24.5355838378299,
4.66832850467759));
#105207=CARTESIAN_POINT('Ctrl Pts',(-10.8844732311435,24.5353744189112,
4.66599925344385));
#105208=CARTESIAN_POINT('Ctrl Pts',(-10.8897905057381,24.5350102172733,
4.66194367143839));
#105209=CARTESIAN_POINT('Ctrl Pts',(-10.8920330133011,24.5348558257488,
4.66022297113469));
#105210=CARTESIAN_POINT('Ctrl Pts',(-10.8966939342908,24.5345332454733,
4.65662509512259));
#105211=CARTESIAN_POINT('Ctrl Pts',(-10.899111454672,24.5343649805011,4.65474681821634));
#105212=CARTESIAN_POINT('Ctrl Pts',(-10.905496296162,24.5339181022548,4.64975395110147));
#105213=CARTESIAN_POINT('Ctrl Pts',(-10.9094534031084,24.5336385948903,
4.64662644155455));
#105214=CARTESIAN_POINT('Ctrl Pts',(-10.9261746208772,24.532446944159,4.63326977395955));
#105215=CARTESIAN_POINT('Ctrl Pts',(-10.9387824430841,24.5315221616816,
4.62284784674164));
#105216=CARTESIAN_POINT('Ctrl Pts',(-11.0306268022558,24.5246055754881,
4.5442989036557));
#105217=CARTESIAN_POINT('Ctrl Pts',(-11.1025349205422,24.5182068137967,
4.46807391483109));
#105218=CARTESIAN_POINT('Ctrl Pts',(-11.2036854259467,24.5081851635343,
4.33481653555556));
#105219=CARTESIAN_POINT('Ctrl Pts',(-11.2384033829476,24.5044777918534,
4.2823909842636));
#105220=CARTESIAN_POINT('Ctrl Pts',(-11.2866596134648,24.4989271085745,
4.19821859625217));
#105221=CARTESIAN_POINT('Ctrl Pts',(-11.3026268927655,24.4970047640162,
4.16795630382618));
#105222=CARTESIAN_POINT('Ctrl Pts',(-11.3214916805296,24.494616809187,4.12894770061124));
#105223=CARTESIAN_POINT('Ctrl Pts',(-11.325386549232,24.4941167315327,4.12069797185017));
#105224=CARTESIAN_POINT('Ctrl Pts',(-11.331511122883,24.4933187147972,4.10740495130876));
#105225=CARTESIAN_POINT('Ctrl Pts',(-11.3337898650438,24.4930190922183,
4.10238462987594));
#105226=CARTESIAN_POINT('Ctrl Pts',(-11.3380659612539,24.4924515972576,
4.09282068563827));
#105227=CARTESIAN_POINT('Ctrl Pts',(-11.3400686728381,24.4921835442227,
4.08827955506737));
#105228=CARTESIAN_POINT('Ctrl Pts',(-11.3445763650981,24.4915749528857,
4.07791593089748));
#105229=CARTESIAN_POINT('Ctrl Pts',(-11.3470667080947,24.491234916802,4.07208715284194));
#105230=CARTESIAN_POINT('Ctrl Pts',(-11.3534337245679,24.4903554051297,
4.05691271196101));
#105231=CARTESIAN_POINT('Ctrl Pts',(-11.3572515273751,24.4898179199295,
4.04754261374875));
#105232=CARTESIAN_POINT('Ctrl Pts',(-11.3828935532509,24.4861351589582,
3.98269239327272));
#105233=CARTESIAN_POINT('Ctrl Pts',(-11.4014083083704,24.4831031324559,
3.92596051283679));
#105234=CARTESIAN_POINT('Ctrl Pts',(-11.4430675317994,24.4748791585684,
3.76572625701971));
#105235=CARTESIAN_POINT('Ctrl Pts',(-11.4585112309955,24.46987996121,3.66061611863117));
#105236=CARTESIAN_POINT('Ctrl Pts',(-11.4631583753308,24.4636910495957,
3.53651482612231));
#105237=CARTESIAN_POINT('Ctrl Pts',(-11.4634999999691,24.4627726088713,
3.51825682543672));
#105238=CARTESIAN_POINT('Ctrl Pts',(-11.4635,24.4618423224409,3.5000000024766));
#105239=CARTESIAN_POINT('Origin',(-10.,24.85,3.5));
#105240=CARTESIAN_POINT('',(-11.3004035488554,24.85,2.82859635082588));
#105241=CARTESIAN_POINT('',(-11.4635,24.85,3.5));
#105242=CARTESIAN_POINT('Origin',(-10.,24.85,3.5));
#105243=CARTESIAN_POINT('Ctrl Pts',(-11.3004035488553,24.85,2.82859635082581));
#105244=CARTESIAN_POINT('Ctrl Pts',(-11.3125618755898,24.85,2.85843423653158));
#105245=CARTESIAN_POINT('Ctrl Pts',(-11.3236469117651,24.85,2.88866598859084));
#105246=CARTESIAN_POINT('Ctrl Pts',(-11.3336107592203,24.85,2.91926079192103));
#105247=CARTESIAN_POINT('Ctrl Pts',(-11.351398587096,24.85,2.97387976295373));
#105248=CARTESIAN_POINT('Ctrl Pts',(-11.3656158973012,24.85,3.02965613094422));
#105249=CARTESIAN_POINT('Ctrl Pts',(-11.3763225973211,24.85,3.08625266725227));
#105250=CARTESIAN_POINT('Ctrl Pts',(-11.3802128743286,24.85,3.10681700579705));
#105251=CARTESIAN_POINT('Ctrl Pts',(-11.3836391895696,24.85,3.12748960196462));
#105252=CARTESIAN_POINT('Ctrl Pts',(-11.3866028162641,24.85,3.14825403475913));
#105253=CARTESIAN_POINT('Ctrl Pts',(-11.3891864342721,24.85,3.16635596459899));
#105254=CARTESIAN_POINT('Ctrl Pts',(-11.3914188580782,24.85,3.18453415298079));
#105255=CARTESIAN_POINT('Ctrl Pts',(-11.3932974125123,24.85,3.20274227033469));
#105256=CARTESIAN_POINT('Ctrl Pts',(-11.3992038488262,24.85,3.25999112274849));
#105257=CARTESIAN_POINT('Ctrl Pts',(-11.4016259665454,24.85,3.31758827200733));
#105258=CARTESIAN_POINT('Ctrl Pts',(-11.4006269322846,24.85,3.37519248066477));
#105259=CARTESIAN_POINT('Ctrl Pts',(-11.3999593676723,24.85,3.41368418483278));
#105260=CARTESIAN_POINT('Ctrl Pts',(-11.3977631279099,24.85,3.45217902944069));
#105261=CARTESIAN_POINT('Ctrl Pts',(-11.3940446763944,24.85,3.49057134449431));
#105262=CARTESIAN_POINT('Ctrl Pts',(-11.3924040169226,24.85,3.50751084607837));
#105263=CARTESIAN_POINT('Ctrl Pts',(-11.3904668951253,24.85,3.52443032836664));
#105264=CARTESIAN_POINT('Ctrl Pts',(-11.3882332939498,24.85,3.54132038036121));
#105265=CARTESIAN_POINT('Ctrl Pts',(-11.3867101763176,24.85,3.55283789579101));
#105266=CARTESIAN_POINT('Ctrl Pts',(-11.385048893467,24.85,3.56434288508996));
#105267=CARTESIAN_POINT('Ctrl Pts',(-11.383252385453,24.85,3.57581506234222));
#105268=CARTESIAN_POINT('Ctrl Pts',(-11.3745487112871,24.85,3.63139516106727));
#105269=CARTESIAN_POINT('Ctrl Pts',(-11.3626636031163,24.85,3.68630052936635));
#105270=CARTESIAN_POINT('Ctrl Pts',(-11.3476521220032,24.85,3.74021322586292));
#105271=CARTESIAN_POINT('Ctrl Pts',(-11.3330120872859,24.85,3.79279189831172));
#105272=CARTESIAN_POINT('Ctrl Pts',(-11.3153979702509,24.85,3.84442733350712));
#105273=CARTESIAN_POINT('Ctrl Pts',(-11.2948184588981,24.85,3.89480080308046));
#105274=CARTESIAN_POINT('Ctrl Pts',(-11.28259085348,24.85,3.92473090680962));
#105275=CARTESIAN_POINT('Ctrl Pts',(-11.2693156001385,24.85,3.95421497642643));
#105276=CARTESIAN_POINT('Ctrl Pts',(-11.2549882247325,24.85,3.98318007522436));
#105277=CARTESIAN_POINT('Ctrl Pts',(-11.2448400683478,24.85,4.00369620912678));
#105278=CARTESIAN_POINT('Ctrl Pts',(-11.2341639691643,24.85,4.0239518800964));
#105279=CARTESIAN_POINT('Ctrl Pts',(-11.2229570283328,24.85,4.04391943548386));
#105280=CARTESIAN_POINT('Ctrl Pts',(-11.2180985058252,24.85,4.05257592959147));
#105281=CARTESIAN_POINT('Ctrl Pts',(-11.2131400386115,24.85,4.06117831142199));
#105282=CARTESIAN_POINT('Ctrl Pts',(-11.2080890554702,24.85,4.06971182776291));
#105283=CARTESIAN_POINT('Ctrl Pts',(-11.1812246840833,24.85,4.11509854670538));
#105284=CARTESIAN_POINT('Ctrl Pts',(-11.1516963968566,24.85,4.15863054938992));
#105285=CARTESIAN_POINT('Ctrl Pts',(-11.1195205442675,24.85,4.20001692638652));
#105286=CARTESIAN_POINT('Ctrl Pts',(-11.1125970057767,24.85,4.20892236792339));
#105287=CARTESIAN_POINT('Ctrl Pts',(-11.1055507414306,24.85,4.21772833257868));
#105288=CARTESIAN_POINT('Ctrl Pts',(-11.0983816907031,24.85,4.22643169138809));
#105289=CARTESIAN_POINT('Ctrl Pts',(-11.0643171649521,24.85,4.26778664918564));
#105290=CARTESIAN_POINT('Ctrl Pts',(-11.0274823323406,24.85,4.30682867683741));
#105291=CARTESIAN_POINT('Ctrl Pts',(-10.9881733610665,24.85,4.34342341161918));
#105292=CARTESIAN_POINT('Ctrl Pts',(-10.9564831645753,24.85,4.37292543871853));
#105293=CARTESIAN_POINT('Ctrl Pts',(-10.9231840933228,24.85,4.40083613613505));
#105294=CARTESIAN_POINT('Ctrl Pts',(-10.8884241147858,24.85,4.42706182455881));
#105295=CARTESIAN_POINT('Ctrl Pts',(-10.8802209909417,24.85,4.43325091267364));
#105296=CARTESIAN_POINT('Ctrl Pts',(-10.8719430995626,24.85,4.43934102278144));
#105297=CARTESIAN_POINT('Ctrl Pts',(-10.8635972985758,24.85,4.44532811031609));
#105298=CARTESIAN_POINT('Ctrl Pts',(-10.8209284670976,24.85,4.47593775814561));
#105299=CARTESIAN_POINT('Ctrl Pts',(-10.7764485190081,24.85,4.50388699710063));
#105300=CARTESIAN_POINT('Ctrl Pts',(-10.7304487595703,24.85,4.52906821597762));
#105301=CARTESIAN_POINT('Ctrl Pts',(-10.6846750591674,24.85,4.55412568546749));
#105302=CARTESIAN_POINT('Ctrl Pts',(-10.6373952802604,24.85,4.57644253090575));
#105303=CARTESIAN_POINT('Ctrl Pts',(-10.5888840527018,24.85,4.59586320662698));
#105304=CARTESIAN_POINT('Ctrl Pts',(-10.5645845311458,24.85,4.60559112224716));
#105305=CARTESIAN_POINT('Ctrl Pts',(-10.5399759463448,24.85,4.61459157026943));
#105306=CARTESIAN_POINT('Ctrl Pts',(-10.515093012538,24.85,4.62283999060172));
#105307=CARTESIAN_POINT('Ctrl Pts',(-10.4967624813286,24.85,4.62891636115766));
#105308=CARTESIAN_POINT('Ctrl Pts',(-10.4782830689616,24.85,4.63458454898126));
#105309=CARTESIAN_POINT('Ctrl Pts',(-10.4596689220486,24.85,4.6398335167748));
#105310=CARTESIAN_POINT('Ctrl Pts',(-10.4506717510829,24.85,4.64237061185912));
#105311=CARTESIAN_POINT('Ctrl Pts',(-10.4416440578635,24.85,4.6448093832563));
#105312=CARTESIAN_POINT('Ctrl Pts',(-10.4325999392588,24.85,4.64714563599666));
#105313=CARTESIAN_POINT('Ctrl Pts',(-10.3837719044625,24.85,4.65975876449322));
#105314=CARTESIAN_POINT('Ctrl Pts',(-10.3343687941817,24.85,4.66941559578891));
#105315=CARTESIAN_POINT('Ctrl Pts',(-10.2846440492021,24.85,4.67598884653307));
#105316=CARTESIAN_POINT('Ctrl Pts',(-10.2359323305191,24.85,4.68242818254602));
#105317=CARTESIAN_POINT('Ctrl Pts',(-10.1869110047086,24.85,4.68590832870446));
#105318=CARTESIAN_POINT('Ctrl Pts',(-10.1378247465409,24.85,4.68626042890209));
#105319=CARTESIAN_POINT('Ctrl Pts',(-10.0887384883732,24.85,4.68661252909973));
#105320=CARTESIAN_POINT('Ctrl Pts',(-10.039586391101,24.85,4.68383676613634));
#105321=CARTESIAN_POINT('Ctrl Pts',(-9.99063336962943,24.85,4.67771275306651));
#105322=CARTESIAN_POINT('Ctrl Pts',(-8.88741263453866,24.85,3.88631788102315));
#105323=CARTESIAN_POINT('Ctrl Pts',(-8.81508513359861,24.85,3.73963918744251));
#105324=CARTESIAN_POINT('Ctrl Pts',(-8.78311241042471,24.85,3.59288578274215));
#105325=CARTESIAN_POINT('Ctrl Pts',(-8.76395555587307,24.85,3.29953678129824));
#105326=CARTESIAN_POINT('Ctrl Pts',(-8.78327471948896,24.85,3.14104654297177));
#105327=CARTESIAN_POINT('Ctrl Pts',(-8.87385485848026,24.85,2.84353830916111));
#105328=CARTESIAN_POINT('Ctrl Pts',(-8.9447791067978,24.85,2.70306361360872));
#105329=CARTESIAN_POINT('Ctrl Pts',(-9.13798618895579,24.85,2.4539623946865));
#105330=CARTESIAN_POINT('Ctrl Pts',(-9.26068603117401,24.85,2.34761760023775));
#105331=CARTESIAN_POINT('Ctrl Pts',(-9.52437211317925,24.85,2.18773266971445));
#105332=CARTESIAN_POINT('Ctrl Pts',(-9.66339960403327,24.85,2.13073968047222));
#105333=CARTESIAN_POINT('Ctrl Pts',(-9.95596335995801,24.85,2.05973084110956));
#105334=CARTESIAN_POINT('Ctrl Pts',(-10.1100968233425,24.85,2.04702898053788));
#105335=CARTESIAN_POINT('Ctrl Pts',(-10.2623899083091,24.85,2.06021397908666));
#105336=CARTESIAN_POINT('Origin',(-10.,24.85,3.5));
#105337=CARTESIAN_POINT('Ctrl Pts',(-10.5090140092792,13.1337998239626,
2.44023125247533));
#105338=CARTESIAN_POINT('Ctrl Pts',(-10.8605022655926,13.1601924775763,
2.60904375492577));
#105339=CARTESIAN_POINT('Ctrl Pts',(-11.3762582958501,13.2129702164138,
3.3207757270411));
#105340=CARTESIAN_POINT('Ctrl Pts',(-10.8990613565784,13.2921330404754,
4.55894989925235));
#105341=CARTESIAN_POINT('Ctrl Pts',(-9.60213183554956,13.3712882961471,
4.82960051060231));
#105342=CARTESIAN_POINT('Ctrl Pts',(-8.6680683892318,13.4504435518189,3.89129233265225));
#105343=CARTESIAN_POINT('Ctrl Pts',(-8.94638477794343,13.5295988074907,
2.59588490110802));
#105344=CARTESIAN_POINT('Ctrl Pts',(-10.1841644808861,13.6087540631624,
2.12409172341792));
#105345=CARTESIAN_POINT('Ctrl Pts',(-11.2541792099669,13.6879093188342,
2.90481120670036));
#105346=CARTESIAN_POINT('Ctrl Pts',(-11.182332230381,13.767064574506,4.22755695617222));
#105347=CARTESIAN_POINT('Ctrl Pts',(-10.0339701846483,13.8462198301777,
4.88781414517024));
#105348=CARTESIAN_POINT('Ctrl Pts',(-8.85469118695272,13.9253750858495,
4.28452438368559));
#105349=CARTESIAN_POINT('Ctrl Pts',(-8.71818818692633,14.0045303415213,
2.96692304576068));
#105350=CARTESIAN_POINT('Ctrl Pts',(-9.74875435949711,14.083685597193,2.13468707585548));
#105351=CARTESIAN_POINT('Ctrl Pts',(-11.0080732815695,14.1628408528648,
2.54553861657238));
#105352=CARTESIAN_POINT('Ctrl Pts',(-11.3495611174537,14.2419961085365,
3.82541187780965));
#105353=CARTESIAN_POINT('Ctrl Pts',(-10.4622981596486,14.3211513642083,
4.80900243763703));
#105354=CARTESIAN_POINT('Ctrl Pts',(-9.154121563492,14.4003066198801,4.60077124308019));
#105355=CARTESIAN_POINT('Ctrl Pts',(-8.61610143836823,14.4794618755519,
3.3903079498792));
#105356=CARTESIAN_POINT('Ctrl Pts',(-9.3380953065286,14.5586171312236,2.2797174047905));
#105357=CARTESIAN_POINT('Ctrl Pts',(-10.6627410645075,14.6377723868954,
2.28017139776325));
#105358=CARTESIAN_POINT('Ctrl Pts',(-11.3839734156908,14.7169276425671,
3.39125671511969));
#105359=CARTESIAN_POINT('Ctrl Pts',(-10.8451236777656,14.7960828982389,
4.60135074808574));
#105360=CARTESIAN_POINT('Ctrl Pts',(-9.53680453925627,14.8752381539106,
4.80868540180449));
#105361=CARTESIAN_POINT('Ctrl Pts',(-8.65021625863274,14.9543934095824,
3.82448630689678));
#105362=CARTESIAN_POINT('Ctrl Pts',(-8.99258099578772,15.0335486652542,
2.54484846228196));
#105363=CARTESIAN_POINT('Ctrl Pts',(-10.2521820169156,15.112703920926,2.1348583434421));
#105364=CARTESIAN_POINT('Ctrl Pts',(-11.2821759977529,15.1918591765977,
2.96780433840964));
#105365=CARTESIAN_POINT('Ctrl Pts',(-11.1447725563174,15.2710144322695,
4.28530459413146));
#105366=CARTESIAN_POINT('Ctrl Pts',(-9.96507497325763,15.3501696879412,
4.88779960875228));
#105367=CARTESIAN_POINT('Ctrl Pts',(-8.81717597805976,15.429324943613,4.22672886591294));
#105368=CARTESIAN_POINT('Ctrl Pts',(-8.74621627703462,15.5084801992848,
2.90398499394259));
#105369=CARTESIAN_POINT('Ctrl Pts',(-9.81680335943576,15.5876354549565,
2.12390171050809));
#105370=CARTESIAN_POINT('Ctrl Pts',(-11.0541875791356,15.6667907106283,
2.59673035065145));
#105371=CARTESIAN_POINT('Ctrl Pts',(-11.3317535956899,15.7459459663,3.89196922303317));
#105372=CARTESIAN_POINT('Ctrl Pts',(-10.3967827084337,15.8251012219718,
4.83032740095482));
#105373=CARTESIAN_POINT('Ctrl Pts',(-9.10054853769248,15.9042564776436,
4.55744719886774));
#105374=CARTESIAN_POINT('Ctrl Pts',(-8.62324821084428,15.9834117333153,
3.3217809704406));
#105375=CARTESIAN_POINT('Ctrl Pts',(-9.39945480685586,16.0625669889871,
2.24837985697228));
#105376=CARTESIAN_POINT('Ctrl Pts',(-10.7224466426081,16.1417222446589,
2.3145556276125));
#105377=CARTESIAN_POINT('Ctrl Pts',(-11.3876642339107,16.2208775003306,
3.46005647279232));
#105378=CARTESIAN_POINT('Ctrl Pts',(-10.789439324166,16.3000327560024,4.64192515731166));
#105379=CARTESIAN_POINT('Ctrl Pts',(-9.47244457819178,16.3791880116741,
4.78409220399535));
#105380=CARTESIAN_POINT('Ctrl Pts',(-8.63577924136583,16.4583432673459,
3.75711715841716));
#105381=CARTESIAN_POINT('Ctrl Pts',(-9.04121155694682,16.5374985230177,
2.49604171754569));
#105382=CARTESIAN_POINT('Ctrl Pts',(-10.3196029348599,16.6166537786894,
2.14905163848878));
#105383=CARTESIAN_POINT('Ctrl Pts',(-11.3070017790651,16.6958090343612,
3.03207494087031));
#105384=CARTESIAN_POINT('Ctrl Pts',(-11.1043997885858,16.774964290033,4.34113531516184));
#105385=CARTESIAN_POINT('Ctrl Pts',(-9.89626231124403,16.8541195457047,
4.88435761397571));
#105386=CARTESIAN_POINT('Ctrl Pts',(-8.78257607198402,16.9332748013765,
4.16714802775323));
#105387=CARTESIAN_POINT('Ctrl Pts',(-8.77733169845742,17.0124300570483,
2.84251255841355));
#105388=CARTESIAN_POINT('Ctrl Pts',(-9.88530409531549,17.09158531272,2.11650718798777));
#105389=CARTESIAN_POINT('Ctrl Pts',(-11.0977049822458,17.1707405683918,
2.65014631647928));
#105390=CARTESIAN_POINT('Ctrl Pts',(-11.3106658790912,17.2498958240635,
3.95756143284488));
#105391=CARTESIAN_POINT('Ctrl Pts',(-10.3302898462604,17.3290510797353,
4.84837536646819));
#105392=CARTESIAN_POINT('Ctrl Pts',(-9.04919104546304,17.4082063354071,
4.5115185828314));
#105393=CARTESIAN_POINT('Ctrl Pts',(-8.63378613096917,17.4873615910788,
3.25369292436326));
#105394=CARTESIAN_POINT('Ctrl Pts',(-9.4622935588648,17.5665168467506,2.2201252816769));
#105395=CARTESIAN_POINT('Ctrl Pts',(-10.7803727103917,17.6456721024224,
2.35185978891218));
#105396=CARTESIAN_POINT('Ctrl Pts',(-11.3879370090656,17.7248273580941,
3.52895462496553));
#105397=CARTESIAN_POINT('Ctrl Pts',(-10.7318104499819,17.8039826137659,
4.67968681298818));
#105398=CARTESIAN_POINT('Ctrl Pts',(-9.40938407382203,17.8831378694376,
4.75633607732401));
#105399=CARTESIAN_POINT('Ctrl Pts',(-8.62470252432374,17.9622931251094,
3.68911468700078));
#105400=CARTESIAN_POINT('Ctrl Pts',(-9.09220377228481,18.0414483807812,
2.4497078880678));
#105401=CARTESIAN_POINT('Ctrl Pts',(-10.3862366179896,18.1206036364529,
2.16657254176879));
#105402=CARTESIAN_POINT('Ctrl Pts',(-11.3286081996048,18.1997588921247,
3.09749812002438));
#105403=CARTESIAN_POINT('Ctrl Pts',(-11.0613067020991,18.2789141477965,
4.394894181186));
#105404=CARTESIAN_POINT('Ctrl Pts',(-9.82770517227246,18.3580694034682,
4.87750571823832));
#105405=CARTESIAN_POINT('Ctrl Pts',(-8.75097488171399,18.43722465914,4.10592389400942));
#105406=CARTESIAN_POINT('Ctrl Pts',(-8.81145875345403,18.5163799148118,
2.78265962284292));
#105407=CARTESIAN_POINT('Ctrl Pts',(-9.95408734611271,18.5955351704835,
2.11252043631124));
#105408=CARTESIAN_POINT('Ctrl Pts',(-11.1385185570414,18.6746904261553,
2.70565561202124));
#105409=CARTESIAN_POINT('Ctrl Pts',(-11.2863497763831,18.7538456818271,
4.02202659342217));
#105410=CARTESIAN_POINT('Ctrl Pts',(-10.2629834257514,18.8330009374988,
4.8631020611902));
#105411=CARTESIAN_POINT('Ctrl Pts',(-9.00017555241863,18.9121561931706,
4.4630984297877));
#105412=CARTESIAN_POINT('Ctrl Pts',(-8.64768926105856,18.9913114488423,
3.18621157321436));
#105413=CARTESIAN_POINT('Ctrl Pts',(-9.52645677047307,19.0704667045141,
2.19502324878559));
#105414=CARTESIAN_POINT('Ctrl Pts',(-10.8363765915541,19.1496219601858,
2.39199200880984));
#105415=CARTESIAN_POINT('Ctrl Pts',(-11.3847910665814,19.2287772158577,
3.59778145712457));
#105416=CARTESIAN_POINT('Ctrl Pts',(-10.6723790060287,19.3079324715294,
4.71454270558623));
#105417=CARTESIAN_POINT('Ctrl Pts',(-9.34777835383489,19.3870877272012,
4.72548538780132));
#105418=CARTESIAN_POINT('Ctrl Pts',(-8.61701339166654,19.4662429828729,
3.62064639493691));
#105419=CARTESIAN_POINT('Ctrl Pts',(-9.1454320393717,19.5453982385447,2.40596110119043));
#105420=CARTESIAN_POINT('Ctrl Pts',(-10.4519189366623,19.6245534942164,
2.18737789667895));
#105421=CARTESIAN_POINT('Ctrl Pts',(-11.3469420391427,19.7037087498882,
3.16391272765676));
#105422=CARTESIAN_POINT('Ctrl Pts',(-11.0155994422605,19.78286400556,4.44644877532865));
#105423=CARTESIAN_POINT('Ctrl Pts',(-9.75957242386244,19.8620192612317,
4.86726079885059));
#105424=CARTESIAN_POINT('Ctrl Pts',(-8.72245024619805,19.9411745169035,
4.04320726983491));
#105425=CARTESIAN_POINT('Ctrl Pts',(-8.84851338145853,20.0203297725752,
2.72457361486673));
#105426=CARTESIAN_POINT('Ctrl Pts',(-10.0229836873447,20.0994850282471,
2.11195127551048));
#105427=CARTESIAN_POINT('Ctrl Pts',(-11.176527772959,20.1786402839188,2.76312150872955));
#105428=CARTESIAN_POINT('Ctrl Pts',(-11.2588651821356,20.2577955395905,
4.08520591644964));
#105429=CARTESIAN_POINT('Ctrl Pts',(-10.195029233715,20.3369507952623,4.87447121084345));
#105430=CARTESIAN_POINT('Ctrl Pts',(-8.95362279179843,20.4161060509341,
4.41230600655548));
#105431=CARTESIAN_POINT('Ctrl Pts',(-8.6649233554112,20.4952613066058,3.11950313468514));
#105432=CARTESIAN_POINT('Ctrl Pts',(-9.59178639711394,20.5744165622776,
2.17313558874325));
#105433=CARTESIAN_POINT('Ctrl Pts',(-10.8903203393042,20.6535718179494,
2.43485343503247));
#105434=CARTESIAN_POINT('Ctrl Pts',(-11.3782341554329,20.7327270736211,
3.66636743743653));
#105435=CARTESIAN_POINT('Ctrl Pts',(-10.6112913817496,20.8118823292929,
4.74640697929671));
#105436=CARTESIAN_POINT('Ctrl Pts',(-9.28777916327362,20.8910375849647,
4.69161612576101));
#105437=CARTESIAN_POINT('Ctrl Pts',(-8.61273078299548,20.9701928406364,
3.55188093091511));
#105438=CARTESIAN_POINT('Ctrl Pts',(-9.20076524821148,21.0493480963082,
2.36490911246084));
#105439=CARTESIAN_POINT('Ctrl Pts',(-10.5164881045002,21.1285033519799,
2.21141645620059));
#105440=CARTESIAN_POINT('Ctrl Pts',(-11.3619581384099,21.2076586076517,
3.2311551736411));
#105441=CARTESIAN_POINT('Ctrl Pts',(-10.9673905935855,21.2868138633234,
4.49567211012625));
#105442=CARTESIAN_POINT('Ctrl Pts',(-9.69203188820424,21.3659691189952,
4.85364809073771));
#105443=CARTESIAN_POINT('Ctrl Pts',(-8.69707242631543,21.445124374667,3.9791526366132));
#105444=CARTESIAN_POINT('Ctrl Pts',(-8.88840431081413,21.5242796303387,
2.66839760989743));
#105445=CARTESIAN_POINT('Ctrl Pts',(-10.091823415966,21.6034348860105,2.11480110752238));
#105446=CARTESIAN_POINT('Ctrl Pts',(-11.2116390070345,21.6825901416822,
2.82240245862798));
#105447=CARTESIAN_POINT('Ctrl Pts',(-11.2282797954346,21.7617453973541,
4.14694378084031));
#105448=CARTESIAN_POINT('Ctrl Pts',(-10.1265946525276,21.8409006530258,
4.88245481133823));
#105449=CARTESIAN_POINT('Ctrl Pts',(-8.90964743072545,21.9200559086976,
4.3592664232458));
#105450=CARTESIAN_POINT('Ctrl Pts',(-8.68544596361199,21.9992111643693,
3.05373192265566));
#105451=CARTESIAN_POINT('Ctrl Pts',(-9.65812152114782,22.0783664200411,
2.15451621446482));
#105452=CARTESIAN_POINT('Ctrl Pts',(-10.9420710812999,22.1575216757129,
2.48033849282147));
#105453=CARTESIAN_POINT('Ctrl Pts',(-11.368282426372,22.2366769313846,3.73454362732737));
#105454=CARTESIAN_POINT('Ctrl Pts',(-10.5486980460349,22.3158321870564,
4.77520114715896));
#105455=CARTESIAN_POINT('Ctrl Pts',(-9.22953429003054,22.3949874427282,
4.65481171678237));
#105456=CARTESIAN_POINT('Ctrl Pts',(-8.61186524708977,22.4741426983999,
3.4829876756009));
#105457=CARTESIAN_POINT('Ctrl Pts',(-9.25806710397417,22.5532979540717,
2.32665303970874));
#105458=CARTESIAN_POINT('Ctrl Pts',(-10.5797850770295,22.6324532097434,
2.23862900937123));
#105459=CARTESIAN_POINT('Ctrl Pts',(-11.3736195102213,22.7116084654152,
3.29905982880227));
#105460=CARTESIAN_POINT('Ctrl Pts',(-10.9167989025253,22.790763721087,4.54244294028871));
#105461=CARTESIAN_POINT('Ctrl Pts',(-9.62524992855897,22.8699189767587,
4.83670112444038));
#105462=CARTESIAN_POINT('Ctrl Pts',(-8.67490393222552,22.9490742324305,
3.91391777108728));
#105463=CARTESIAN_POINT('Ctrl Pts',(-8.93103328280782,23.0282294881023,
2.6142699794191));
#105464=CARTESIAN_POINT('Ctrl Pts',(-10.1604369698711,23.107384743774,2.12106291135225));
#105465=CARTESIAN_POINT('Ctrl Pts',(-11.2437657716457,23.1865399994458,
2.88335244562916));
#105466=CARTESIAN_POINT('Ctrl Pts',(-11.1946689586256,23.2656952551175,
4.20708811094663));
#105467=CARTESIAN_POINT('Ctrl Pts',(-10.0578482372994,23.3448505107893,
4.88703320755515));
#105468=CARTESIAN_POINT('Ctrl Pts',(-8.86835780799071,23.424005766461,4.30411030628588));
#105469=CARTESIAN_POINT('Ctrl Pts',(-8.70920649628835,23.5031610221328,
2.9890599785474));
#105470=CARTESIAN_POINT('Ctrl Pts',(-9.72529882267551,23.5823162778046,
2.1392109193126));
#105471=CARTESIAN_POINT('Ctrl Pts',(-10.9915012041141,23.6614715334763,
2.52833527778638));
#105472=CARTESIAN_POINT('Ctrl Pts',(-11.3549606661359,23.7406267891481,
3.80214184282734));
#105473=CARTESIAN_POINT('Ctrl Pts',(-10.4847526509621,23.8197820448198,
4.80085477316038));
#105474=CARTESIAN_POINT('Ctrl Pts',(-9.17318820920556,23.8989373004917,
4.61516187852302));
#105475=CARTESIAN_POINT('Ctrl Pts',(-8.61441698141044,23.9780925561634,
3.41413812328771));
#105476=CARTESIAN_POINT('Ctrl Pts',(-9.31720017393552,24.0572478118352,
2.29128366298484));
#105477=CARTESIAN_POINT('Ctrl Pts',(-10.6416468237176,24.1364030675069,
2.26895514761134));
#105478=CARTESIAN_POINT('Ctrl Pts',(-11.3819110892539,24.2155583231787,
3.36744673195469));
#105479=CARTESIAN_POINT('Ctrl Pts',(-10.8639227816716,24.2947135788505,
4.58667042735669));
#105480=CARTESIAN_POINT('Ctrl Pts',(-9.55944130977617,24.3738688345222,
4.8164148973843));
#105481=CARTESIAN_POINT('Ctrl Pts',(-8.65590291890877,24.453024090194,3.84775305145438));
#105482=CARTESIAN_POINT('Ctrl Pts',(-8.97648042349053,24.5321793458658,
2.56215183432611));
#105483=CARTESIAN_POINT('Ctrl Pts',(-10.2282993048877,24.6113346015375,
2.13105295154821));
#105484=CARTESIAN_POINT('Ctrl Pts',(-11.2735200365463,24.6904898572092,
2.94517306433958));
#105485=CARTESIAN_POINT('Ctrl Pts',(-11.1567064504975,24.7696514771236,
4.2669496034009));
#105486=CARTESIAN_POINT('Ctrl Pts',(-10.3802617790044,24.8224280118139,
4.67883450561543));
#105487=CARTESIAN_POINT('Ctrl Pts',(-9.99036782849491,24.8488194612803,
4.67563271633731));
#105488=CARTESIAN_POINT('Ctrl Pts',(-10.5513374813396,13.1902385453535,
2.35211365225463));
#105489=CARTESIAN_POINT('Ctrl Pts',(-10.9320512660756,13.2166311989672,
2.5349625684396));
#105490=CARTESIAN_POINT('Ctrl Pts',(-11.4906913536254,13.2694089378048,
3.30587359591926));
#105491=CARTESIAN_POINT('Ctrl Pts',(-10.9738164664813,13.3485717618664,
4.64699941391677));
#105492=CARTESIAN_POINT('Ctrl Pts',(-9.56904991278341,13.4277270175382,
4.94015406912171));
#105493=CARTESIAN_POINT('Ctrl Pts',(-8.55732100450931,13.5068822732099,
3.92382748847622));
#105494=CARTESIAN_POINT('Ctrl Pts',(-8.85877883075876,13.5860375288817,
2.52070958288531));
#105495=CARTESIAN_POINT('Ctrl Pts',(-10.1994773801761,13.6651927845534,
2.00968776902748));
#105496=CARTESIAN_POINT('Ctrl Pts',(-11.3584616418533,13.7443480402252,
2.85532247789389));
#105497=CARTESIAN_POINT('Ctrl Pts',(-11.2806407331068,13.823503295897,4.28805182654041));
#105498=CARTESIAN_POINT('Ctrl Pts',(-10.0367947359074,13.9026585515687,
5.00320804814235));
#105499=CARTESIAN_POINT('Ctrl Pts',(-8.75946110552875,13.9818138072405,
4.34975597894302));
#105500=CARTESIAN_POINT('Ctrl Pts',(-8.61160816070229,14.0609690629123,
2.92259878912427));
#105501=CARTESIAN_POINT('Ctrl Pts',(-9.72786379921332,14.140124318584,2.02116410331367));
#105502=CARTESIAN_POINT('Ctrl Pts',(-11.091892509704,14.2192795742558,2.46617710793435));
#105503=CARTESIAN_POINT('Ctrl Pts',(-11.4617743595397,14.2984348299276,
3.85246920878199));
#105504=CARTESIAN_POINT('Ctrl Pts',(-10.5007373045184,14.3775900855993,
4.91784330858839));
#105505=CARTESIAN_POINT('Ctrl Pts',(-9.08378850443773,14.4567453412711,
4.69229811680502));
#105506=CARTESIAN_POINT('Ctrl Pts',(-8.50103310814551,14.5359005969429,
3.3811872806365));
#105507=CARTESIAN_POINT('Ctrl Pts',(-9.28305928730295,14.6150558526146,
2.17825340697768));
#105508=CARTESIAN_POINT('Ctrl Pts',(-10.7178466262713,14.6942111082864,
2.178745148536));
#105509=CARTESIAN_POINT('Ctrl Pts',(-11.4990479698752,14.7733663639581,
3.382214933763));
#105510=CARTESIAN_POINT('Ctrl Pts',(-10.9153939801766,14.8525216196299,
4.69292580646453));
#105511=CARTESIAN_POINT('Ctrl Pts',(-9.49829078563862,14.9316768753017,
4.9174999118759));
#105512=CARTESIAN_POINT('Ctrl Pts',(-8.5379845058244,15.0108321309734,3.85146667854391));
#105513=CARTESIAN_POINT('Ctrl Pts',(-8.90881616947513,15.0899873866452,
2.4654295687286));
#105514=CARTESIAN_POINT('Ctrl Pts',(-10.2731504349797,15.1691426423169,
2.02134961144923));
#105515=CARTESIAN_POINT('Ctrl Pts',(-11.3887863051869,15.2482978979887,
2.92355335945149));
#105516=CARTESIAN_POINT('Ctrl Pts',(-11.239958049093,15.3274531536604,4.35060106228906));
#105517=CARTESIAN_POINT('Ctrl Pts',(-9.96217102883449,15.4066084093323,
5.00319230305103));
#105518=CARTESIAN_POINT('Ctrl Pts',(-8.71882658387331,15.485763665004,4.28715488227258));
#105519=CARTESIAN_POINT('Ctrl Pts',(-8.64196672908225,15.5649189206758,
2.85442756723797));
#105520=CARTESIAN_POINT('Ctrl Pts',(-9.80157093408568,15.6440741763475,
2.00948195693348));
#105521=CARTESIAN_POINT('Ctrl Pts',(-11.1418411166389,15.7232294320193,
2.52162532982622));
#105522=CARTESIAN_POINT('Ctrl Pts',(-11.4424861788233,15.802384687691,3.92456066090555));
#105523=CARTESIAN_POINT('Ctrl Pts',(-10.4297743777558,15.8815399433628,
4.94094139891786));
#105524=CARTESIAN_POINT('Ctrl Pts',(-9.02576099129743,15.9606951990346,
4.64537176707374));
#105525=CARTESIAN_POINT('Ctrl Pts',(-8.50877412011141,16.0398504547064,
3.306962423248));
#105526=CARTESIAN_POINT('Ctrl Pts',(-9.34952070437594,16.1190057103781,
2.14431020625923));
#105527=CARTESIAN_POINT('Ctrl Pts',(-10.7825166008728,16.1981609660499,
2.21598835665465));
#105528=CARTESIAN_POINT('Ctrl Pts',(-11.5030456720688,16.2773162217216,
3.45673525033684));
#105529=CARTESIAN_POINT('Ctrl Pts',(-10.8550795866552,16.3564714773934,
4.73687389469326));
#105530=CARTESIAN_POINT('Ctrl Pts',(-9.42857942566512,16.4356267330652,
4.89086184005273));
#105531=CARTESIAN_POINT('Ctrl Pts',(-8.52234708014868,16.5147819887369,
3.77849592338659));
#105532=CARTESIAN_POINT('Ctrl Pts',(-8.96149026216576,16.5939372444087,
2.41256464315734));
#105533=CARTESIAN_POINT('Ctrl Pts',(-10.3461772641267,16.6730925000805,
2.03672304990142));
#105534=CARTESIAN_POINT('Ctrl Pts',(-11.415676299355,16.7522477557522,2.99316793083631));
#105535=CARTESIAN_POINT('Ctrl Pts',(-11.1962283684358,16.831403011424,4.41107399339338));
#105536=CARTESIAN_POINT('Ctrl Pts',(-9.88763673495018,16.9105582670957,
4.99946411346035));
#105537=CARTESIAN_POINT('Ctrl Pts',(-8.6813497664918,16.9897135227675,4.22262001948248));
#105538=CARTESIAN_POINT('Ctrl Pts',(-8.67566933405057,17.0688687784393,
2.78784382463254));
#105539=CARTESIAN_POINT('Ctrl Pts',(-9.87576736581714,17.148024034111,2.00147259501467));
#105540=CARTESIAN_POINT('Ctrl Pts',(-11.188976902664,17.2271792897828,2.57948272377994));
#105541=CARTESIAN_POINT('Ctrl Pts',(-11.4196450617917,17.3063345454545,
3.99560672858512));
#105542=CARTESIAN_POINT('Ctrl Pts',(-10.3577527703159,17.3854898011263,
4.960490015789));
#105543=CARTESIAN_POINT('Ctrl Pts',(-8.97013322880461,17.4646450567981,
4.59562428070742));
#105544=CARTESIAN_POINT('Ctrl Pts',(-8.52018824670579,17.5438003124699,
3.23321299563051));
#105545=CARTESIAN_POINT('Ctrl Pts',(-9.41758436987738,17.6229555681416,
2.11370632091287));
#105546=CARTESIAN_POINT('Ctrl Pts',(-10.8452591025203,17.7021108238134,
2.25639428254181));
#105547=CARTESIAN_POINT('Ctrl Pts',(-11.5033411279189,17.7812660794852,
3.5313621427124));
#105548=CARTESIAN_POINT('Ctrl Pts',(-10.7926589896463,17.8604213351569,
4.77777535467742));
#105549=CARTESIAN_POINT('Ctrl Pts',(-9.36027556954837,17.9395765908287,
4.86079784831231));
#105550=CARTESIAN_POINT('Ctrl Pts',(-8.51034935677729,18.0187318465004,
3.70483918578783));
#105551=CARTESIAN_POINT('Ctrl Pts',(-9.01672237574194,18.0978871021722,
2.36237825068194));
#105552=CARTESIAN_POINT('Ctrl Pts',(-10.4183514014968,18.177042357844,2.05570078039427));
#105553=CARTESIAN_POINT('Ctrl Pts',(-11.4390792494977,18.2561976135157,
3.06403091330536));
#105554=CARTESIAN_POINT('Ctrl Pts',(-11.1495521800918,18.3353528691875,
4.46930279899226));
#105555=CARTESIAN_POINT('Ctrl Pts',(-9.81337921032534,18.4145081248593,
4.99204249662981));
#105556=CARTESIAN_POINT('Ctrl Pts',(-8.64712100199181,18.493663380531,4.15630522444703));
#105557=CARTESIAN_POINT('Ctrl Pts',(-8.71263398375444,18.5728186362028,
2.72301424008924));
#105558=CARTESIAN_POINT('Ctrl Pts',(-9.9502698030027,18.6519738918746,1.99715435310386));
#105559=CARTESIAN_POINT('Ctrl Pts',(-11.2331840425896,18.7311291475463,
2.63960750352496));
#105560=CARTESIAN_POINT('Ctrl Pts',(-11.3933071249595,18.8102844032181,
4.06543203519537));
#105561=CARTESIAN_POINT('Ctrl Pts',(-10.2848499588316,18.8894396588898,
4.97644120500673));
#105562=CARTESIAN_POINT('Ctrl Pts',(-8.91704219793103,18.9685949145616,
4.54317809113592));
#105563=CARTESIAN_POINT('Ctrl Pts',(-8.53524739357896,19.0477501702333,
3.16012070838186));
#105564=CARTESIAN_POINT('Ctrl Pts',(-9.48708262108046,19.1269054259051,
2.08651710541289));
#105565=CARTESIAN_POINT('Ctrl Pts',(-10.9059195916668,19.2060606815769,
2.29986341430553));
#105566=CARTESIAN_POINT('Ctrl Pts',(-11.4999336067621,19.2852159372486,
3.60591178496073));
#105567=CARTESIAN_POINT('Ctrl Pts',(-10.7282859428849,19.3643711929204,
4.81552944333614));
#105568=CARTESIAN_POINT('Ctrl Pts',(-9.29354746015517,19.4435264485922,
4.82738198715927));
#105569=CARTESIAN_POINT('Ctrl Pts',(-8.50202088849231,19.5226817042639,
3.63067789550905));
#105570=CARTESIAN_POINT('Ctrl Pts',(-9.07437646418891,19.6018369599357,
2.31499400809925));
#105571=CARTESIAN_POINT('Ctrl Pts',(-10.4894950704046,19.6809922156074,
2.07823605794153));
#105572=CARTESIAN_POINT('Ctrl Pts',(-11.4589375102327,19.7601474712792,
3.13596775949951));
#105573=CARTESIAN_POINT('Ctrl Pts',(-11.1000444552377,19.839302726951,4.52514405201858));
#105574=CARTESIAN_POINT('Ctrl Pts',(-9.7395813634678,19.9184579826227,4.98094573318362));
#105575=CARTESIAN_POINT('Ctrl Pts',(-8.61622460147083,19.9976132382945,
4.08837384145925));
#105576=CARTESIAN_POINT('Ctrl Pts',(-8.75276962816412,20.0767684939663,
2.66009849954996));
#105577=CARTESIAN_POINT('Ctrl Pts',(-10.024894733861,20.155923749638,1.99653786774855));
#105578=CARTESIAN_POINT('Ctrl Pts',(-11.2743536469417,20.2350790053098,
2.70185157181484));
#105579=CARTESIAN_POINT('Ctrl Pts',(-11.3635372430076,20.3142342609816,
4.13386458949784));
#105580=CARTESIAN_POINT('Ctrl Pts',(-10.2112455149443,20.3933895166533,
4.98875567616181));
#105581=CARTESIAN_POINT('Ctrl Pts',(-8.86661867063735,20.4725447723251,
4.4881623819698));
#105582=CARTESIAN_POINT('Ctrl Pts',(-8.55391446756972,20.5517000279969,
3.08786559985373));
#105583=CARTESIAN_POINT('Ctrl Pts',(-9.55784427233645,20.6308552836686,
2.06280953127903));
#105584=CARTESIAN_POINT('Ctrl Pts',(-10.9643486515284,20.7100105393404,
2.34628868030886));
#105585=CARTESIAN_POINT('Ctrl Pts',(-11.4928315018848,20.7891657950121,
3.68020054902433));
#105586=CARTESIAN_POINT('Ctrl Pts',(-10.6621190077965,20.8683210506839,
4.85004316612566));
#105587=CARTESIAN_POINT('Ctrl Pts',(-9.2285594598184,20.9474763063557,4.79069656536787));
#105588=CARTESIAN_POINT('Ctrl Pts',(-8.49738218968395,21.0266315620274,
3.55619472403284));
#105589=CARTESIAN_POINT('Ctrl Pts',(-9.13431051598326,21.1057868176992,
2.27052863060953));
#105590=CARTESIAN_POINT('Ctrl Pts',(-10.5594330322662,21.1849420733709,
2.10427337443985));
#105591=CARTESIAN_POINT('Ctrl Pts',(-11.4752021673908,21.2640973290427,
3.20880127710866));
#105592=CARTESIAN_POINT('Ctrl Pts',(-11.0478271395602,21.3432525847144,
4.57846020626129));
#105593=CARTESIAN_POINT('Ctrl Pts',(-9.66642497063913,21.4224078403863,
4.96620115627938));
#105594=CARTESIAN_POINT('Ctrl Pts',(-8.58873666785621,21.501563096058,4.01899319671312));
#105595=CARTESIAN_POINT('Ctrl Pts',(-8.79597740657156,21.5807183517298,
2.59925157485461));
#105596=CARTESIAN_POINT('Ctrl Pts',(-10.099458344886,21.6598736074015,1.9996246574538));
#105597=CARTESIAN_POINT('Ctrl Pts',(-11.3123843081986,21.7390288630733,
2.76606161124914));
#105598=CARTESIAN_POINT('Ctrl Pts',(-11.3304087440624,21.818184118745,4.20073583083093));
#105599=CARTESIAN_POINT('Ctrl Pts',(-10.1371207385322,21.8973393744168,
4.99740309668184));
#105600=CARTESIAN_POINT('Ctrl Pts',(-8.81898684838297,21.9764946300886,
4.4307126659695));
#105601=CARTESIAN_POINT('Ctrl Pts',(-8.57614348859796,22.0556498857604,
3.01662564628873));
#105602=CARTESIAN_POINT('Ctrl Pts',(-9.62969502603374,22.1348051414321,
2.04264199417463));
#105603=CARTESIAN_POINT('Ctrl Pts',(-11.0204023616999,22.2139603971039,
2.3955557274683));
#105604=CARTESIAN_POINT('Ctrl Pts',(-11.4820523069404,22.2931156527756,
3.75404544943282));
#105605=CARTESIAN_POINT('Ctrl Pts',(-10.5943211644514,22.3722709084474,
4.88123151005539));
#105606=CARTESIAN_POINT('Ctrl Pts',(-9.16547164469076,22.4514261641192,
4.75083194518341));
#105607=CARTESIAN_POINT('Ctrl Pts',(-8.49644468624091,22.5305814197909,
3.48157313568008));
#105608=CARTESIAN_POINT('Ctrl Pts',(-9.19637690365897,22.6097366754627,
2.22909164378287));
#105609=CARTESIAN_POINT('Ctrl Pts',(-10.6279930183855,22.6888919311344,
2.13374859565661));
#105610=CARTESIAN_POINT('Ctrl Pts',(-11.4878331583777,22.7680471868062,
3.28235206523099));
#105611=CARTESIAN_POINT('Ctrl Pts',(-10.9930288530349,22.8472024424779,
4.62911993513292));
#105612=CARTESIAN_POINT('Ctrl Pts',(-9.59409022786481,22.9263576981498,
4.94784508445347));
#105613=CARTESIAN_POINT('Ctrl Pts',(-8.56472490889904,23.0055129538215,
3.94833418576464));
#105614=CARTESIAN_POINT('Ctrl Pts',(-8.84215089025304,23.0846682094933,
2.54062334279264));
#105615=CARTESIAN_POINT('Ctrl Pts',(-10.1737769752306,23.163823465165,2.00640711744365));
#105616=CARTESIAN_POINT('Ctrl Pts',(-11.3471823474695,23.2429787208368,
2.83207946480194));
#105617=CARTESIAN_POINT('Ctrl Pts',(-11.2940032350308,23.3221339765085,
4.2658810387686));
#105618=CARTESIAN_POINT('Ctrl Pts',(-10.0626581997178,23.4012892321803,
5.00236217716447));
#105619=CARTESIAN_POINT('Ctrl Pts',(-8.77426407810743,23.4804444878521,
4.37097043088206));
#105620=CARTESIAN_POINT('Ctrl Pts',(-8.60187966088841,23.5595997435238,
2.94657636252054));
#105621=CARTESIAN_POINT('Ctrl Pts',(-9.70245798255812,23.6387549991956,
2.02606409508629));
#105622=CARTESIAN_POINT('Ctrl Pts',(-11.0739424979592,23.7179102548674,
2.4475433467726));
#105623=CARTESIAN_POINT('Ctrl Pts',(-11.4676228696329,23.7970655105391,
3.82726431806394));
#105624=CARTESIAN_POINT('Ctrl Pts',(-10.5250588407825,23.8762207662109,
4.90901818250252));
#105625=CARTESIAN_POINT('Ctrl Pts',(-9.10444050268076,23.9553760218826,
4.70788530410297));
#105626=CARTESIAN_POINT('Ctrl Pts',(-8.49920859204261,24.0345312775544,
3.40699888414332));
#105627=CARTESIAN_POINT('Ctrl Pts',(-9.26042676724236,24.1136865332262,
2.1907813758452));
#105628=CARTESIAN_POINT('Ctrl Pts',(-10.6949984425754,24.192841788898,2.16659629016257));
#105629=CARTESIAN_POINT('Ctrl Pts',(-11.49681416522,24.2719970445697,3.35642519927706));
#105630=CARTESIAN_POINT('Ctrl Pts',(-10.9357561910591,24.3511523002415,
4.67702484714226));
#105631=CARTESIAN_POINT('Ctrl Pts',(-9.52280975725156,24.4303075559132,
4.92587209917784));
#105632=CARTESIAN_POINT('Ctrl Pts',(-8.54414400025217,24.509462811585,3.87666800524516));
#105633=CARTESIAN_POINT('Ctrl Pts',(-8.89137686757647,24.5886180672568,
2.48417168070902));
#105634=CARTESIAN_POINT('Ctrl Pts',(-10.2472819243751,24.6677733229285,
2.01722780901545));
#105635=CARTESIAN_POINT('Ctrl Pts',(-11.3794106185394,24.7469285786003,
2.89904034130693));
#105636=CARTESIAN_POINT('Ctrl Pts',(-11.2528842221252,24.8260901985145,
4.3307198916829));
#105637=CARTESIAN_POINT('Ctrl Pts',(-10.4118797668908,24.8788667332049,
4.77685217969272));
#105638=CARTESIAN_POINT('Ctrl Pts',(-9.98956693316758,24.9052581826713,
4.77338416819561));
#105639=CARTESIAN_POINT('Ctrl Pts',(-10.5936609534001,13.2466772667445,
2.26399605203392));
#105640=CARTESIAN_POINT('Ctrl Pts',(-11.0036002665585,13.2730699203582,
2.46088138195343));
#105641=CARTESIAN_POINT('Ctrl Pts',(-11.6051244114009,13.3258476591958,
3.29097146479741));
#105642=CARTESIAN_POINT('Ctrl Pts',(-11.0485715763842,13.4050104832573,
4.73504892858119));
#105643=CARTESIAN_POINT('Ctrl Pts',(-9.53596799001725,13.4841657389291,
5.0507076276411));
#105644=CARTESIAN_POINT('Ctrl Pts',(-8.44657361978682,13.5633209946008,
3.95636264430017));
#105645=CARTESIAN_POINT('Ctrl Pts',(-8.77117288357405,13.6424762502726,
2.44553426466258));
#105646=CARTESIAN_POINT('Ctrl Pts',(-10.2147902794661,13.7216315059443,
1.89528381463706));
#105647=CARTESIAN_POINT('Ctrl Pts',(-11.4627440737396,13.8007867616161,
2.80583374908742));
#105648=CARTESIAN_POINT('Ctrl Pts',(-11.3789492358326,13.8799420172879,
4.3485466969086));
#105649=CARTESIAN_POINT('Ctrl Pts',(-10.0396192871665,13.9590972729597,
5.11860195111448));
#105650=CARTESIAN_POINT('Ctrl Pts',(-8.6642310241048,14.0382525286314,4.41498757420045));
#105651=CARTESIAN_POINT('Ctrl Pts',(-8.50502813447824,14.1174077843032,
2.87827453248787));
#105652=CARTESIAN_POINT('Ctrl Pts',(-9.70697323892953,14.1965630399749,
1.90764113077184));
#105653=CARTESIAN_POINT('Ctrl Pts',(-11.1757117378384,14.2757182956467,
2.38681559929634));
#105654=CARTESIAN_POINT('Ctrl Pts',(-11.5739876016257,14.3548735513185,
3.8795265397543));
#105655=CARTESIAN_POINT('Ctrl Pts',(-10.5391764493883,14.4340288069902,
5.02668417953975));
#105656=CARTESIAN_POINT('Ctrl Pts',(-9.01345544538346,14.513184062662,4.78382499052982));
#105657=CARTESIAN_POINT('Ctrl Pts',(-8.3859647779228,14.5923393183338,3.37206661139379));
#105658=CARTESIAN_POINT('Ctrl Pts',(-9.22802326807728,14.6714945740055,
2.07678940916483));
#105659=CARTESIAN_POINT('Ctrl Pts',(-10.7729521880352,14.7506498296773,
2.07731889930876));
#105660=CARTESIAN_POINT('Ctrl Pts',(-11.6141225240595,14.829805085349,3.37317315240631));
#105661=CARTESIAN_POINT('Ctrl Pts',(-10.9856642825877,14.9089603410208,
4.78450086484332));
#105662=CARTESIAN_POINT('Ctrl Pts',(-9.45977703202094,14.9881155966926,
5.02631442194729));
#105663=CARTESIAN_POINT('Ctrl Pts',(-8.42575275301606,15.0672708523643,
3.87844705019104));
#105664=CARTESIAN_POINT('Ctrl Pts',(-8.82505134316252,15.1464261080361,
2.38601067517526));
#105665=CARTESIAN_POINT('Ctrl Pts',(-10.2941188530438,15.2255813637079,
1.90784087945636));
#105666=CARTESIAN_POINT('Ctrl Pts',(-11.495396612621,15.3047366193796,2.87930238049334));
#105667=CARTESIAN_POINT('Ctrl Pts',(-11.3351435418684,15.3838918750514,
4.41589753044666));
#105668=CARTESIAN_POINT('Ctrl Pts',(-9.95926708441137,15.4630471307231,
5.11858499734976));
#105669=CARTESIAN_POINT('Ctrl Pts',(-8.62047718968688,15.5422023863949,
4.34758089863223));
#105670=CARTESIAN_POINT('Ctrl Pts',(-8.53771718112988,15.6213576420667,
2.80487014053335));
#105671=CARTESIAN_POINT('Ctrl Pts',(-9.78633850873561,15.7005128977384,
1.89506220335889));
#105672=CARTESIAN_POINT('Ctrl Pts',(-11.2294946541421,15.7796681534102,
2.44652030900095));
#105673=CARTESIAN_POINT('Ctrl Pts',(-11.5532187619568,15.858823409082,3.95715209877795));
#105674=CARTESIAN_POINT('Ctrl Pts',(-10.462766047078,15.9379786647537,5.05155539688088));
#105675=CARTESIAN_POINT('Ctrl Pts',(-8.95097344490238,16.0171339204255,
4.73329633527975));
#105676=CARTESIAN_POINT('Ctrl Pts',(-8.39430002937858,16.0962891760973,
3.2921438760554));
#105677=CARTESIAN_POINT('Ctrl Pts',(-9.29958660189599,16.175444431769,2.04024055554619));
#105678=CARTESIAN_POINT('Ctrl Pts',(-10.8425865591376,16.2545996874408,
2.1174210856968));
#105679=CARTESIAN_POINT('Ctrl Pts',(-11.6184271102268,16.3337549431125,
3.45341402788135));
#105680=CARTESIAN_POINT('Ctrl Pts',(-10.9207198491445,16.4129101987843,
4.83182263207488));
#105681=CARTESIAN_POINT('Ctrl Pts',(-9.38471427313846,16.4920654544561,
4.99763147611009));
#105682=CARTESIAN_POINT('Ctrl Pts',(-8.40891491893154,16.5712207101278,
3.79987468835603));
#105683=CARTESIAN_POINT('Ctrl Pts',(-8.88176896738465,16.6503759657996,
2.32908756876899));
#105684=CARTESIAN_POINT('Ctrl Pts',(-10.3727515933935,16.7295312214714,
1.92439446131403));
#105685=CARTESIAN_POINT('Ctrl Pts',(-11.5243508196448,16.8086864771431,
2.95426092080234));
#105686=CARTESIAN_POINT('Ctrl Pts',(-11.2880569482855,16.8878417328149,
4.48101267162488));
#105687=CARTESIAN_POINT('Ctrl Pts',(-9.87901115865631,16.9669969884866,
5.11457061294499));
#105688=CARTESIAN_POINT('Ctrl Pts',(-8.5801234609996,17.0461522441584,4.27809201121172));
#105689=CARTESIAN_POINT('Ctrl Pts',(-8.5740069696437,17.1253074998302,2.73317509085155));
#105690=CARTESIAN_POINT('Ctrl Pts',(-9.86623063631879,17.2044627555019,
1.88643800204158));
#105691=CARTESIAN_POINT('Ctrl Pts',(-11.2802488230823,17.2836180111737,
2.5088191310806));
#105692=CARTESIAN_POINT('Ctrl Pts',(-11.528624244492,17.3627732668455,4.03365202432535));
#105693=CARTESIAN_POINT('Ctrl Pts',(-10.3852156943715,17.4419285225172,
5.07260466510981));
#105694=CARTESIAN_POINT('Ctrl Pts',(-8.89107541214616,17.521083778189,4.67972997858343));
#105695=CARTESIAN_POINT('Ctrl Pts',(-8.40659036244245,17.6002390338608,
3.21273306689779));
#105696=CARTESIAN_POINT('Ctrl Pts',(-9.37287518088994,17.6793942895325,
2.00728736014882));
#105697=CARTESIAN_POINT('Ctrl Pts',(-10.9101454946488,17.7585495452043,
2.16092877617142));
#105698=CARTESIAN_POINT('Ctrl Pts',(-11.6187452467723,17.8377048008761,
3.53376966045927));
#105699=CARTESIAN_POINT('Ctrl Pts',(-10.8535075293106,17.9168600565478,
4.87586389636666));
#105700=CARTESIAN_POINT('Ctrl Pts',(-9.31116706527467,17.9960153122196,
4.9652596193006));
#105701=CARTESIAN_POINT('Ctrl Pts',(-8.39599618923083,18.0751705678913,
3.72056368457489));
#105702=CARTESIAN_POINT('Ctrl Pts',(-8.94124097919904,18.1543258235631,
2.27504861329608));
#105703=CARTESIAN_POINT('Ctrl Pts',(-10.4504661850041,18.2334810792348,
1.94482901901976));
#105704=CARTESIAN_POINT('Ctrl Pts',(-11.5495502993905,18.3126363349066,
3.03056370658632));
#105705=CARTESIAN_POINT('Ctrl Pts',(-11.2377976580847,18.3917915905784,
4.54371141679851));
#105706=CARTESIAN_POINT('Ctrl Pts',(-9.79905324837822,18.4709468462501,
5.1065792750213));
#105707=CARTESIAN_POINT('Ctrl Pts',(-8.54326712226964,18.5501021019219,
4.20668655488465));
#105708=CARTESIAN_POINT('Ctrl Pts',(-8.61380921405485,18.6292573575937,
2.66336885733557));
#105709=CARTESIAN_POINT('Ctrl Pts',(-9.94645225989268,18.7084126132654,
1.88178826989647));
#105710=CARTESIAN_POINT('Ctrl Pts',(-11.3278495281379,18.7875678689372,
2.57355939502869));
#105711=CARTESIAN_POINT('Ctrl Pts',(-11.5002644735358,18.866723124609,4.10883747696858));
#105712=CARTESIAN_POINT('Ctrl Pts',(-10.3067164919117,18.9458783802807,
5.08978034882327));
#105713=CARTESIAN_POINT('Ctrl Pts',(-8.83390884344341,19.0250336359525,
4.62325775248417));
#105714=CARTESIAN_POINT('Ctrl Pts',(-8.42280552609934,19.1041888916243,
3.13402984354935));
#105715=CARTESIAN_POINT('Ctrl Pts',(-9.44770847168781,19.183344147296,1.97801096204018));
#105716=CARTESIAN_POINT('Ctrl Pts',(-10.9754625917795,19.2624994029678,
2.20773481980123));
#105717=CARTESIAN_POINT('Ctrl Pts',(-11.6150761469429,19.3416546586395,
3.6140421127969));
#105718=CARTESIAN_POINT('Ctrl Pts',(-10.7841928797412,19.4208099143114,
4.91651618108603));
#105719=CARTESIAN_POINT('Ctrl Pts',(-9.23931656647548,19.4999651699831,
4.92927858651721));
#105720=CARTESIAN_POINT('Ctrl Pts',(-8.38702838531804,19.5791204256548,
3.64070939608118));
#105721=CARTESIAN_POINT('Ctrl Pts',(-9.00332088900616,19.6582756813266,
2.22402691500807));
#105722=CARTESIAN_POINT('Ctrl Pts',(-10.527071204147,19.7374309369984,1.9690942192041));
#105723=CARTESIAN_POINT('Ctrl Pts',(-11.570932981323,19.8165861926701,3.10802279134227));
#105724=CARTESIAN_POINT('Ctrl Pts',(-11.1844894682147,19.8957414483419,
4.60383932870849));
#105725=CARTESIAN_POINT('Ctrl Pts',(-9.71959030307317,19.9748967040136,
5.09463066751667));
#105726=CARTESIAN_POINT('Ctrl Pts',(-8.50999895674359,20.0540519596854,
4.13354041308357));
#105727=CARTESIAN_POINT('Ctrl Pts',(-8.65702587486972,20.1332072153571,
2.59562338423319));
#105728=CARTESIAN_POINT('Ctrl Pts',(-10.0268057803772,20.212362471029,1.88112445998662));
#105729=CARTESIAN_POINT('Ctrl Pts',(-11.3721795209244,20.2915177267007,
2.64058163490015));
#105730=CARTESIAN_POINT('Ctrl Pts',(-11.4682093038797,20.3706729823725,
4.18252326254603));
#105731=CARTESIAN_POINT('Ctrl Pts',(-10.2274617961735,20.4498282380442,
5.10304014148018));
#105732=CARTESIAN_POINT('Ctrl Pts',(-8.77961454947628,20.528983493716,4.56401875738413));
#105733=CARTESIAN_POINT('Ctrl Pts',(-8.44290557972825,20.6081387493877,
3.05622806502234));
#105734=CARTESIAN_POINT('Ctrl Pts',(-9.52390214755894,20.6872940050596,
1.95248347381479));
#105735=CARTESIAN_POINT('Ctrl Pts',(-11.0383769637525,20.7664492607313,
2.25772392558526));
#105736=CARTESIAN_POINT('Ctrl Pts',(-11.6074288483367,20.845604516403,3.69403366061213));
#105737=CARTESIAN_POINT('Ctrl Pts',(-10.7129466338434,20.9247597720748,
4.95367935295463));
#105738=CARTESIAN_POINT('Ctrl Pts',(-9.1693397563632,21.0039150277466,4.88977700497472));
#105739=CARTESIAN_POINT('Ctrl Pts',(-8.38203359637242,21.0830702834183,
3.56050851715058));
#105740=CARTESIAN_POINT('Ctrl Pts',(-9.06785578375502,21.1622255390901,
2.17614814875822));
#105741=CARTESIAN_POINT('Ctrl Pts',(-10.6023779600323,21.2413807947618,
1.99713029267914));
#105742=CARTESIAN_POINT('Ctrl Pts',(-11.5884461963717,21.3205360504337,
3.18644738057619));
#105743=CARTESIAN_POINT('Ctrl Pts',(-11.1282636855349,21.3996913061054,
4.66124830239637));
#105744=CARTESIAN_POINT('Ctrl Pts',(-9.64081805307402,21.4788465617771,
5.07875422182102));
#105745=CARTESIAN_POINT('Ctrl Pts',(-8.480400909397,21.5580018174489,4.05883375681306));
#105746=CARTESIAN_POINT('Ctrl Pts',(-8.70355050232897,21.6371570731207,
2.53010553981177));
#105747=CARTESIAN_POINT('Ctrl Pts',(-10.1070932738061,21.7163123287924,
1.88444820738525));
#105748=CARTESIAN_POINT('Ctrl Pts',(-11.4131296093626,21.7954675844642,
2.70972076387029));
#105749=CARTESIAN_POINT('Ctrl Pts',(-11.4325376926902,21.874622840136,4.25452788082157));
#105750=CARTESIAN_POINT('Ctrl Pts',(-10.1476468245369,21.9537780958077,
5.11235138202542));
#105751=CARTESIAN_POINT('Ctrl Pts',(-8.7283262660405,22.0329333514795,4.50215890869321));
#105752=CARTESIAN_POINT('Ctrl Pts',(-8.46684101358396,22.1120886071513,
2.9795193699218));
#105753=CARTESIAN_POINT('Ctrl Pts',(-9.60126853091967,22.191243862823,1.93076777388446));
#105754=CARTESIAN_POINT('Ctrl Pts',(-11.0987336420998,22.2703991184948,
2.31077296211515));
#105755=CARTESIAN_POINT('Ctrl Pts',(-11.5958221875089,22.3495543741665,
3.77354727153826));
#105756=CARTESIAN_POINT('Ctrl Pts',(-10.6399442828679,22.4287096298383,
4.98726187295182));
#105757=CARTESIAN_POINT('Ctrl Pts',(-9.101408999351,22.5078648855101,4.84685217358446));
#105758=CARTESIAN_POINT('Ctrl Pts',(-8.38102412539203,22.5870201411818,
3.48015859575926));
#105759=CARTESIAN_POINT('Ctrl Pts',(-9.13468670334375,22.6661753968536,
2.131530247857));
#105760=CARTESIAN_POINT('Ctrl Pts',(-10.6762009597416,22.7453306525254,
2.02886818194197));
#105761=CARTESIAN_POINT('Ctrl Pts',(-11.6020468065343,22.8244859081971,
3.2656443016597));
#105762=CARTESIAN_POINT('Ctrl Pts',(-11.0692588035446,22.9036411638689,
4.71579692997711));
#105763=CARTESIAN_POINT('Ctrl Pts',(-9.5629305271706,22.9827964195406,5.05898904446656));
#105764=CARTESIAN_POINT('Ctrl Pts',(-8.4545458855726,23.0619516752124,3.98275060044199));
#105765=CARTESIAN_POINT('Ctrl Pts',(-8.75326849769826,23.1411069308841,
2.4669767061662));
#105766=CARTESIAN_POINT('Ctrl Pts',(-10.1871169805901,23.220262186556,1.89175132353505));
#105767=CARTESIAN_POINT('Ctrl Pts',(-11.4505989232932,23.2994174422277,
2.7808064839747));
#105768=CARTESIAN_POINT('Ctrl Pts',(-11.3933375114359,23.3785726978995,
4.32467396659057));
#105769=CARTESIAN_POINT('Ctrl Pts',(-10.0674681621363,23.4577279535712,
5.1176911467738));
#105770=CARTESIAN_POINT('Ctrl Pts',(-8.68017034822411,23.536883209243,4.43783055547826));
#105771=CARTESIAN_POINT('Ctrl Pts',(-8.49455282548853,23.6160384649147,
2.90409274649368));
#105772=CARTESIAN_POINT('Ctrl Pts',(-9.67961714244069,23.6951937205865,
1.91291727085999));
#105773=CARTESIAN_POINT('Ctrl Pts',(-11.1563837918041,23.7743489762583,
2.36675141575881));
#105774=CARTESIAN_POINT('Ctrl Pts',(-11.5802850731297,23.8535042319301,
3.85238679330052));
#105775=CARTESIAN_POINT('Ctrl Pts',(-10.5653650306028,23.9326594876018,
5.01718159184469));
#105776=CARTESIAN_POINT('Ctrl Pts',(-9.03569279615594,24.0118147432736,
4.80060872968292));
#105777=CARTESIAN_POINT('Ctrl Pts',(-8.38400020267482,24.0909699989453,
3.39985964499894));
#105778=CARTESIAN_POINT('Ctrl Pts',(-9.20365336054916,24.1701252546171,
2.09027908870557));
#105779=CARTESIAN_POINT('Ctrl Pts',(-10.7483500614332,24.2492805102888,
2.06423743271381));
#105780=CARTESIAN_POINT('Ctrl Pts',(-11.6117172411862,24.3284357659606,
3.34540366659943));
#105781=CARTESIAN_POINT('Ctrl Pts',(-11.0075896004464,24.4075910216325,
4.76737926692783));
#105782=CARTESIAN_POINT('Ctrl Pts',(-9.48617820472693,24.4867462773041,
5.03532930097137));
#105783=CARTESIAN_POINT('Ctrl Pts',(-8.43238508159559,24.5659015329759,
3.90558295903594));
#105784=CARTESIAN_POINT('Ctrl Pts',(-8.80627331166242,24.6450567886476,
2.40619152709192));
#105785=CARTESIAN_POINT('Ctrl Pts',(-10.2662645438622,24.7242120443195,
1.90340266648265));
#105786=CARTESIAN_POINT('Ctrl Pts',(-11.4853012005323,24.8033672999912,
2.8529076182743));
#105787=CARTESIAN_POINT('Ctrl Pts',(-11.349061993753,24.8825289199055,4.39449017996491));
#105788=CARTESIAN_POINT('Ctrl Pts',(-10.4434977547771,24.9353054545958,
4.87486985377003));
#105789=CARTESIAN_POINT('Ctrl Pts',(-9.98876603784026,24.9616969040622,
4.87113562005391));
#105790=CARTESIAN_POINT('Ctrl Pts',(-10.6359844254605,13.3031159881355,
2.17587845181322));
#105791=CARTESIAN_POINT('Ctrl Pts',(-11.0751492670415,13.3295086417492,
2.38680019546726));
#105792=CARTESIAN_POINT('Ctrl Pts',(-11.7195574691764,13.3822863805868,
3.27606933367556));
#105793=CARTESIAN_POINT('Ctrl Pts',(-11.1233266862871,13.4614492046484,
4.82309844324562));
#105794=CARTESIAN_POINT('Ctrl Pts',(-9.50288606725111,13.5406044603201,
5.16126118616049));
#105795=CARTESIAN_POINT('Ctrl Pts',(-8.33582623506433,13.6197597159919,
3.98889780012413));
#105796=CARTESIAN_POINT('Ctrl Pts',(-8.68356693638938,13.6989149716636,
2.37035894643987));
#105797=CARTESIAN_POINT('Ctrl Pts',(-10.2301031787562,13.7780702273355,
1.78087986024663));
#105798=CARTESIAN_POINT('Ctrl Pts',(-11.5670265056259,13.8572254830071,
2.75634502028094));
#105799=CARTESIAN_POINT('Ctrl Pts',(-11.4772577385584,13.9363807386789,
4.40904156727679));
#105800=CARTESIAN_POINT('Ctrl Pts',(-10.0424438384259,14.0155359943506,
5.2339958540866));
#105801=CARTESIAN_POINT('Ctrl Pts',(-8.56900094268083,14.0946912500225,
4.48021916945787));
#105802=CARTESIAN_POINT('Ctrl Pts',(-8.3984481082542,14.1738465056942,2.83395027585145));
#105803=CARTESIAN_POINT('Ctrl Pts',(-9.68608267864575,14.2530017613659,
1.79411815823003));
#105804=CARTESIAN_POINT('Ctrl Pts',(-11.2595309659728,14.3321570170378,
2.30745409065834));
#105805=CARTESIAN_POINT('Ctrl Pts',(-11.6862008437117,14.4113122727095,
3.90658387072663));
#105806=CARTESIAN_POINT('Ctrl Pts',(-10.5776155942583,14.4904675283814,
5.13552505049112));
#105807=CARTESIAN_POINT('Ctrl Pts',(-8.94312238632918,14.5696227840531,
4.87535186425462));
#105808=CARTESIAN_POINT('Ctrl Pts',(-8.27089644770011,14.6487780397248,
3.36294594215109));
#105809=CARTESIAN_POINT('Ctrl Pts',(-9.1729872488516,14.7279332953965,1.97532541135201));
#105810=CARTESIAN_POINT('Ctrl Pts',(-10.828057749799,14.8070885510684,1.97589265008151));
#105811=CARTESIAN_POINT('Ctrl Pts',(-11.7291970782439,14.8862438067401,
3.36413137104963));
#105812=CARTESIAN_POINT('Ctrl Pts',(-11.0559345849988,14.9653990624118,
4.87607592322209));
#105813=CARTESIAN_POINT('Ctrl Pts',(-9.42126327840329,15.0445543180837,
5.1351289320187));
#105814=CARTESIAN_POINT('Ctrl Pts',(-8.31352100020771,15.1237095737555,
3.90542742183816));
#105815=CARTESIAN_POINT('Ctrl Pts',(-8.74128651684992,15.2028648294271,
2.30659178162193));
#105816=CARTESIAN_POINT('Ctrl Pts',(-10.3150872711079,15.2820200850989,
1.79433214746349));
#105817=CARTESIAN_POINT('Ctrl Pts',(-11.602006920055,15.3611753407707,2.83505140153521));
#105818=CARTESIAN_POINT('Ctrl Pts',(-11.4303290346439,15.4403305964424,
4.48119399860425));
#105819=CARTESIAN_POINT('Ctrl Pts',(-9.95636313998825,15.5194858521142,
5.2339776916485));
#105820=CARTESIAN_POINT('Ctrl Pts',(-8.52212779550044,15.5986411077859,
4.40800691499187));
#105821=CARTESIAN_POINT('Ctrl Pts',(-8.43346763317752,15.6777963634578,
2.75531271382871));
#105822=CARTESIAN_POINT('Ctrl Pts',(-9.77110608338552,15.7569516191295,
1.78064244978428));
#105823=CARTESIAN_POINT('Ctrl Pts',(-11.3171481916453,15.8361068748012,
2.3714152881757));
#105824=CARTESIAN_POINT('Ctrl Pts',(-11.6639513450902,15.9152621304731,
3.98974353665035));
#105825=CARTESIAN_POINT('Ctrl Pts',(-10.4957577164001,15.9944173861447,
5.16216939484391));
#105826=CARTESIAN_POINT('Ctrl Pts',(-8.87618589850731,16.0735726418165,
4.82122090348578));
#105827=CARTESIAN_POINT('Ctrl Pts',(-8.27982593864574,16.1527278974884,
3.27732532886281));
#105828=CARTESIAN_POINT('Ctrl Pts',(-9.24965249941607,16.2318831531601,
1.93617090483314));
#105829=CARTESIAN_POINT('Ctrl Pts',(-10.9026565174023,16.3110384088318,
2.01885381473895));
#105830=CARTESIAN_POINT('Ctrl Pts',(-11.7338085483849,16.3901936645035,
3.45009280542587));
#105831=CARTESIAN_POINT('Ctrl Pts',(-10.9863601116336,16.4693489201754,
4.92677136945647));
#105832=CARTESIAN_POINT('Ctrl Pts',(-9.3408491206118,16.5485041758471,5.10440111216747));
#105833=CARTESIAN_POINT('Ctrl Pts',(-8.2954827577144,16.6276594315189,3.82125345332548));
#105834=CARTESIAN_POINT('Ctrl Pts',(-8.80204767260358,16.7068146871907,
2.24561049438064));
#105835=CARTESIAN_POINT('Ctrl Pts',(-10.3993259226603,16.7859699428624,
1.81206587272666));
#105836=CARTESIAN_POINT('Ctrl Pts',(-11.6330253399346,16.8651251985341,
2.91535391076835));
#105837=CARTESIAN_POINT('Ctrl Pts',(-11.3798855281354,16.944280454206,4.55095134985639));
#105838=CARTESIAN_POINT('Ctrl Pts',(-9.87038558236248,17.0234357098778,
5.22967711242965));
#105839=CARTESIAN_POINT('Ctrl Pts',(-8.47889715550738,17.1025909655494,
4.33356400294095));
#105840=CARTESIAN_POINT('Ctrl Pts',(-8.47234460523684,17.1817462212212,
2.67850635707057));
#105841=CARTESIAN_POINT('Ctrl Pts',(-9.85669390682044,17.2609014768931,
1.77140340906848));
#105842=CARTESIAN_POINT('Ctrl Pts',(-11.3715207435005,17.3400567325647,
2.43815553838126));
#105843=CARTESIAN_POINT('Ctrl Pts',(-11.6376034271924,17.4192119882365,
4.07169732006558));
#105844=CARTESIAN_POINT('Ctrl Pts',(-10.4126786184271,17.4983672439082,
5.18471931443062));
#105845=CARTESIAN_POINT('Ctrl Pts',(-8.81201759548772,17.5775224995801,
4.76383567645944));
#105846=CARTESIAN_POINT('Ctrl Pts',(-8.29299247817908,17.6566777552518,
3.19225313816505));
#105847=CARTESIAN_POINT('Ctrl Pts',(-9.32816599190252,17.7358330109235,
1.90086839938479));
#105848=CARTESIAN_POINT('Ctrl Pts',(-10.9750318867773,17.8149882665954,
2.06546326980104));
#105849=CARTESIAN_POINT('Ctrl Pts',(-11.7341493656255,17.8941435222671,
3.53617717820614));
#105850=CARTESIAN_POINT('Ctrl Pts',(-10.9143560689751,17.9732987779388,
4.97395243805591));
#105851=CARTESIAN_POINT('Ctrl Pts',(-9.26205856100099,18.0524540336107,
5.06972139028892));
#105852=CARTESIAN_POINT('Ctrl Pts',(-8.28164302168439,18.1316092892824,
3.73628818336193));
#105853=CARTESIAN_POINT('Ctrl Pts',(-8.86575958265614,18.2107645449541,
2.18771897591022));
#105854=CARTESIAN_POINT('Ctrl Pts',(-10.4825809685115,18.289919800626,1.83395725764526));
#105855=CARTESIAN_POINT('Ctrl Pts',(-11.6600213492834,18.3690750562978,
2.99709649986729));
#105856=CARTESIAN_POINT('Ctrl Pts',(-11.3260431360774,18.4482303119694,
4.61812003460476));
#105857=CARTESIAN_POINT('Ctrl Pts',(-9.7847272864311,18.5273855676412,5.22111605341277));
#105858=CARTESIAN_POINT('Ctrl Pts',(-8.43941324254747,18.6065408233129,
4.25706788532226));
#105859=CARTESIAN_POINT('Ctrl Pts',(-8.51498444435524,18.6856960789847,
2.60372347458188));
#105860=CARTESIAN_POINT('Ctrl Pts',(-9.94263471678268,18.7648513346564,
1.76642218668908));
#105861=CARTESIAN_POINT('Ctrl Pts',(-11.4225150136859,18.8440065903283,
2.50751128653242));
#105862=CARTESIAN_POINT('Ctrl Pts',(-11.6072218221122,18.9231618460001,
4.1522429187418));
#105863=CARTESIAN_POINT('Ctrl Pts',(-10.3285830249918,19.0023171016717,
5.20311949263982));
#105864=CARTESIAN_POINT('Ctrl Pts',(-8.75077548895581,19.0814723573435,
4.70333741383239));
#105865=CARTESIAN_POINT('Ctrl Pts',(-8.31036365861973,19.1606276130152,
3.10793897871686));
#105866=CARTESIAN_POINT('Ctrl Pts',(-9.40833432229519,19.2397828686871,
1.86950481866748));
#105867=CARTESIAN_POINT('Ctrl Pts',(-11.045005591892,19.3189381243588,2.11560622529692));
#105868=CARTESIAN_POINT('Ctrl Pts',(-11.7302186871239,19.3980933800307,
3.62217244063306));
#105869=CARTESIAN_POINT('Ctrl Pts',(-10.8400998165974,19.4772486357024,
5.01750291883593));
#105870=CARTESIAN_POINT('Ctrl Pts',(-9.18508567279581,19.5564038913741,
5.03117518587516));
#105871=CARTESIAN_POINT('Ctrl Pts',(-8.27203588214378,19.6355591470458,
3.65074089665331));
#105872=CARTESIAN_POINT('Ctrl Pts',(-8.93226531382342,19.7147144027176,
2.1330598219169));
#105873=CARTESIAN_POINT('Ctrl Pts',(-10.5646473378894,19.7938696583894,
1.85995238046668));
#105874=CARTESIAN_POINT('Ctrl Pts',(-11.682928452413,19.8730249140611,3.08007782318505));
#105875=CARTESIAN_POINT('Ctrl Pts',(-11.2689344811918,19.9521801697329,
4.6825346053984));
#105876=CARTESIAN_POINT('Ctrl Pts',(-9.6995992426785,20.0313354254047,5.20831560184972));
#105877=CARTESIAN_POINT('Ctrl Pts',(-8.40377331201639,20.1104906810765,
4.1787069847079));
#105878=CARTESIAN_POINT('Ctrl Pts',(-8.56128212157532,20.1896459367483,
2.53114826891643));
#105879=CARTESIAN_POINT('Ctrl Pts',(-10.0287168268935,20.2688011924199,
1.76571105222467));
#105880=CARTESIAN_POINT('Ctrl Pts',(-11.4700053949071,20.3479564480918,
2.57931169798544));
#105881=CARTESIAN_POINT('Ctrl Pts',(-11.5728813647517,20.4271117037635,
4.23118193559423));
#105882=CARTESIAN_POINT('Ctrl Pts',(-10.2436780774028,20.5062669594352,
5.21732460679853));
#105883=CARTESIAN_POINT('Ctrl Pts',(-8.6926104283152,20.5854222151071,4.63987513279845));
#105884=CARTESIAN_POINT('Ctrl Pts',(-8.33189669188675,20.6645774707789,
3.02459053019094));
#105885=CARTESIAN_POINT('Ctrl Pts',(-9.48996002278146,20.7437327264505,
1.84215741635058));
#105886=CARTESIAN_POINT('Ctrl Pts',(-11.1124052759767,20.8228879821223,
2.16915917086166));
#105887=CARTESIAN_POINT('Ctrl Pts',(-11.7220261947885,20.9020432377942,
3.70786677219993));
#105888=CARTESIAN_POINT('Ctrl Pts',(-10.7637742598904,20.9811984934658,
5.05731553978359));
#105889=CARTESIAN_POINT('Ctrl Pts',(-9.11012005290798,21.0603537491376,
4.98885744458157));
#105890=CARTESIAN_POINT('Ctrl Pts',(-8.26668500306089,21.1395090048093,
3.5648223102683));
#105891=CARTESIAN_POINT('Ctrl Pts',(-9.00140105152678,21.2186642604812,
2.08176766690691));
#105892=CARTESIAN_POINT('Ctrl Pts',(-10.6453228877982,21.2978195161528,
1.88998721091841));
#105893=CARTESIAN_POINT('Ctrl Pts',(-11.7016902253526,21.3769747718248,
3.16409348404373));
#105894=CARTESIAN_POINT('Ctrl Pts',(-11.2087002315096,21.4561300274965,
4.74403639853141));
#105895=CARTESIAN_POINT('Ctrl Pts',(-9.61521113550892,21.5352852831683,
5.19130728736269));
#105896=CARTESIAN_POINT('Ctrl Pts',(-8.37206515093778,21.6144405388399,
4.09867431691298));
#105897=CARTESIAN_POINT('Ctrl Pts',(-8.6111235980864,21.6935957945117,2.46095950476894));
#105898=CARTESIAN_POINT('Ctrl Pts',(-10.114728202726,21.7727510501836,1.76927175731667));
#105899=CARTESIAN_POINT('Ctrl Pts',(-11.5138749105269,21.8519063058552,
2.65337991649145));
#105900=CARTESIAN_POINT('Ctrl Pts',(-11.534666641318,21.9310615615271,4.3083199308122));
#105901=CARTESIAN_POINT('Ctrl Pts',(-10.1581729105416,22.0102168171988,
5.227299667369));
#105902=CARTESIAN_POINT('Ctrl Pts',(-8.63766568369801,22.0893720728705,
4.57360515141694));
#105903=CARTESIAN_POINT('Ctrl Pts',(-8.35753853856994,22.1685273285423,
2.94241309355486));
#105904=CARTESIAN_POINT('Ctrl Pts',(-9.57284203580558,22.2476825842141,
1.81889355359428));
#105905=CARTESIAN_POINT('Ctrl Pts',(-11.1770649224999,22.3268378398858,
2.22599019676199));
#105906=CARTESIAN_POINT('Ctrl Pts',(-11.7095920680774,22.4059930955575,
3.79304909364371));
#105907=CARTESIAN_POINT('Ctrl Pts',(-10.6855674012843,22.4851483512294,
5.09329223584824));
#105908=CARTESIAN_POINT('Ctrl Pts',(-9.03734635401123,22.5643036069012,
4.94287240198551));
#105909=CARTESIAN_POINT('Ctrl Pts',(-8.26560356454317,22.6434588625728,
3.47874405583843));
#105910=CARTESIAN_POINT('Ctrl Pts',(-9.07299650302853,22.7226141182447,
2.03396885193113));
#105911=CARTESIAN_POINT('Ctrl Pts',(-10.7244089010975,22.8017693739163,
1.92398776822735));
#105912=CARTESIAN_POINT('Ctrl Pts',(-11.7162604546908,22.8809246295881,
3.2489365380884));
#105913=CARTESIAN_POINT('Ctrl Pts',(-11.1454887540544,22.9600798852599,
4.80247392482133));
#105914=CARTESIAN_POINT('Ctrl Pts',(-9.53177082647642,23.0392351409316,
5.17013300447963));
#105915=CARTESIAN_POINT('Ctrl Pts',(-8.34436686224613,23.1183903966035,
4.01716701511935));
#105916=CARTESIAN_POINT('Ctrl Pts',(-8.66438610514347,23.1975456522753,
2.39333006953975));
#105917=CARTESIAN_POINT('Ctrl Pts',(-10.2004569859495,23.2767009079471,
1.77709552962646));
#105918=CARTESIAN_POINT('Ctrl Pts',(-11.5540154991171,23.3558561636188,
2.72953350314748));
#105919=CARTESIAN_POINT('Ctrl Pts',(-11.4926717878413,23.4350114192905,
4.38346689441255));
#105920=CARTESIAN_POINT('Ctrl Pts',(-10.0722781245547,23.5141666749622,
5.23302011638312));
#105921=CARTESIAN_POINT('Ctrl Pts',(-8.58607661834083,23.5933219306341,
4.50469068007444));
#105922=CARTESIAN_POINT('Ctrl Pts',(-8.3872259900886,23.6724771863059,2.8616091304668));
#105923=CARTESIAN_POINT('Ctrl Pts',(-9.6567763023233,23.7516324419776,1.79977044663367));
#105924=CARTESIAN_POINT('Ctrl Pts',(-11.2388250856492,23.8307876976494,
2.28595948474501));
#105925=CARTESIAN_POINT('Ctrl Pts',(-11.6929472766268,23.9099429533211,
3.87750926853712));
#105926=CARTESIAN_POINT('Ctrl Pts',(-10.6056712204232,23.9890982089928,
5.12534500118684));
#105927=CARTESIAN_POINT('Ctrl Pts',(-8.96694508963116,24.0682534646645,
4.89333215526286));
#105928=CARTESIAN_POINT('Ctrl Pts',(-8.26879181330697,24.1474087203365,
3.39272040585454));
#105929=CARTESIAN_POINT('Ctrl Pts',(-9.14687995385603,24.2265639760081,
1.98977680156594));
#105930=CARTESIAN_POINT('Ctrl Pts',(-10.8017016802907,24.30571923168,1.96187857526504));
#105931=CARTESIAN_POINT('Ctrl Pts',(-11.7266203171524,24.3848744873517,
3.33438213392181));
#105932=CARTESIAN_POINT('Ctrl Pts',(-11.0794230098339,24.4640297430234,
4.8577336867134));
#105933=CARTESIAN_POINT('Ctrl Pts',(-9.44954665220232,24.5431849986951,
5.1447865027649));
#105934=CARTESIAN_POINT('Ctrl Pts',(-8.320626162939,24.6223402543669,3.93449791282671));
#105935=CARTESIAN_POINT('Ctrl Pts',(-8.72116975574837,24.7014955100387,
2.32821137347482));
#105936=CARTESIAN_POINT('Ctrl Pts',(-10.2852471633496,24.7806507657105,
1.78957752394988));
#105937=CARTESIAN_POINT('Ctrl Pts',(-11.5911917825255,24.8598060213822,
2.80677489524165));
#105938=CARTESIAN_POINT('Ctrl Pts',(-11.4452397653807,24.9389676412965,
4.45826046824691));
#105939=CARTESIAN_POINT('Ctrl Pts',(-10.4751157426634,24.9917441759868,
4.97288752784733));
#105940=CARTESIAN_POINT('Ctrl Pts',(-9.98796514251294,25.0181356254532,
4.96888707191221));
#105941=CARTESIAN_POINT('Ctrl Pts',(-11.2893010323265,24.8491715501582,
2.80576613662465));
#105942=CARTESIAN_POINT('Ctrl Pts',(-11.2911828539987,24.8493085424027,
2.80954992823753));
#105943=CARTESIAN_POINT('Ctrl Pts',(-11.2930478994451,24.8494459706458,
2.8133420285908));
#105944=CARTESIAN_POINT('Ctrl Pts',(-11.2967488969198,24.8497221006906,
2.82095216262323));
#105945=CARTESIAN_POINT('Ctrl Pts',(-11.2985847475564,24.8498608035729,
2.82477020296673));
#105946=CARTESIAN_POINT('Ctrl Pts',(-11.3004035488554,24.85,2.82859635082591));
#105947=CARTESIAN_POINT('Ctrl Pts',(-10.6340070945752,13.3,2.18095972236309));
#105948=CARTESIAN_POINT('Ctrl Pts',(-10.7649118977414,13.3,2.2597766501823));
#105949=CARTESIAN_POINT('Ctrl Pts',(-10.8821009016869,13.3,2.36060058848546));
#105950=CARTESIAN_POINT('Ctrl Pts',(-11.0770809467795,13.3,2.58998815869127));
#105951=CARTESIAN_POINT('Ctrl Pts',(-11.1560983945165,13.3,2.71786393184818));
#105952=CARTESIAN_POINT('Ctrl Pts',(-11.2754706506363,13.3,3.00226080557722));
#105953=CARTESIAN_POINT('Ctrl Pts',(-11.3122290867249,13.3,3.16041690251937));
#105954=CARTESIAN_POINT('Ctrl Pts',(-11.3221189530405,13.3,3.47550855713216));
#105955=CARTESIAN_POINT('Ctrl Pts',(-11.2969289416632,13.3,3.63084327221525));
#105956=CARTESIAN_POINT('Ctrl Pts',(-11.1953388723352,13.3,3.92477402681276));
#105957=CARTESIAN_POINT('Ctrl Pts',(-11.1178102771856,13.3,4.06435062655608));
#105958=CARTESIAN_POINT('Ctrl Pts',(-10.9298861008457,13.3,4.29041448834001));
#105959=CARTESIAN_POINT('Ctrl Pts',(-10.817769113814,13.3,4.39034265231198));
#105960=CARTESIAN_POINT('Ctrl Pts',(-10.6730394577712,13.3,4.46649518921549));
#105961=CARTESIAN_POINT('Origin',(-10.,13.3,3.5));
#105962=CARTESIAN_POINT('',(-9.34259215682144,13.3,2.1924652288649));
#105963=CARTESIAN_POINT('',(-10.,13.3,4.9635));
#105964=CARTESIAN_POINT('Origin',(-10.,13.3,3.5));
#105965=CARTESIAN_POINT('Ctrl Pts',(-9.34259215682146,13.3,2.19246522886492));
#105966=CARTESIAN_POINT('Ctrl Pts',(-9.31521779133866,13.3,2.20945799843699));
#105967=CARTESIAN_POINT('Ctrl Pts',(-9.28848021785727,13.3,2.22740026541353));
#105968=CARTESIAN_POINT('Ctrl Pts',(-9.26243629817129,13.3,2.24629525384867));
#105969=CARTESIAN_POINT('Ctrl Pts',(-9.21594140958665,13.3,2.28002751814271));
#105970=CARTESIAN_POINT('Ctrl Pts',(-9.17165482603987,13.3,2.31679483974346));
#105971=CARTESIAN_POINT('Ctrl Pts',(-9.12972630031258,13.3,2.35628918066472));
#105972=CARTESIAN_POINT('Ctrl Pts',(-9.11328522426273,13.3,2.37177576053754));
#105973=CARTESIAN_POINT('Ctrl Pts',(-9.0972077460164,13.3,2.38768135360173));
#105974=CARTESIAN_POINT('Ctrl Pts',(-9.08150295565413,13.3,2.40399019950359));
#105975=CARTESIAN_POINT('Ctrl Pts',(-9.06902583680322,13.3,2.41694722751508));
#105976=CARTESIAN_POINT('Ctrl Pts',(-9.05678329388114,13.3,2.43016012005021));
#105977=CARTESIAN_POINT('Ctrl Pts',(-9.04480148606494,13.3,2.44359617390108));
#105978=CARTESIAN_POINT('Ctrl Pts',(-9.00650633540295,13.3,2.48653925180841));
#105979=CARTESIAN_POINT('Ctrl Pts',(-8.97082703665313,13.3,2.53180331423269));
#105980=CARTESIAN_POINT('Ctrl Pts',(-8.93791405473512,13.3,2.57907594938494));
#105981=CARTESIAN_POINT('Ctrl Pts',(-8.90697991548926,13.3,2.62350638968843));
#105982=CARTESIAN_POINT('Ctrl Pts',(-8.87848954676292,13.3,2.66971220198839));
#105983=CARTESIAN_POINT('Ctrl Pts',(-8.8526081156124,13.3,2.71744597458528));
#105984=CARTESIAN_POINT('Ctrl Pts',(-8.84707051117102,13.3,2.72765911734387));
#105985=CARTESIAN_POINT('Ctrl Pts',(-8.8416520475112,13.3,2.73794333779959));
#105986=CARTESIAN_POINT('Ctrl Pts',(-8.83636226986782,13.3,2.74828049613421));
#105987=CARTESIAN_POINT('Ctrl Pts',(-8.81074658205689,13.3,2.79833806728434));
#105988=CARTESIAN_POINT('Ctrl Pts',(-8.78809853079567,13.3,2.84971852311362));
#105989=CARTESIAN_POINT('Ctrl Pts',(-8.76856023990328,13.3,2.90213268419753));
#105990=CARTESIAN_POINT('Ctrl Pts',(-8.74946444936866,13.3,2.95335977701847));
#105991=CARTESIAN_POINT('Ctrl Pts',(-8.73333901424337,13.3,3.00557532995757));
#105992=CARTESIAN_POINT('Ctrl Pts',(-8.72036517763863,13.3,3.05851505090622));
#105993=CARTESIAN_POINT('Ctrl Pts',(-8.71286934006812,13.3,3.08910180495198));
#105994=CARTESIAN_POINT('Ctrl Pts',(-8.70642646300776,13.3,3.11993031884901));
#105995=CARTESIAN_POINT('Ctrl Pts',(-8.70107944044095,13.3,3.15094851201392));
#105996=CARTESIAN_POINT('Ctrl Pts',(-8.6978504963647,13.3,3.16967968619995));
#105997=CARTESIAN_POINT('Ctrl Pts',(-8.69502128966433,13.3,3.18848000645603));
#105998=CARTESIAN_POINT('Ctrl Pts',(-8.69260235178538,13.3,3.20733768073485));
#105999=CARTESIAN_POINT('Ctrl Pts',(-8.69053148333976,13.3,3.22348185829385));
#106000=CARTESIAN_POINT('Ctrl Pts',(-8.68876097039777,13.3,3.23967513535794));
#106001=CARTESIAN_POINT('Ctrl Pts',(-8.68730098700498,13.3,3.25586630701112));
#106002=CARTESIAN_POINT('Ctrl Pts',(-8.68271778980999,13.3,3.30669382523563));
#106003=CARTESIAN_POINT('Ctrl Pts',(-8.68117918886184,13.3,3.3575752015979));
#106004=CARTESIAN_POINT('Ctrl Pts',(-8.68282898128772,13.3,3.40828825099132));
#106005=CARTESIAN_POINT('Ctrl Pts',(-8.68319575405777,13.3,3.41956249695818));
#106006=CARTESIAN_POINT('Ctrl Pts',(-8.68372028641139,13.3,3.43082840054581));
#106007=CARTESIAN_POINT('Ctrl Pts',(-8.68440446650174,13.3,3.44208346590591));
#106008=CARTESIAN_POINT('Ctrl Pts',(-8.68766251977198,13.3,3.49567988448072));
#106009=CARTESIAN_POINT('Ctrl Pts',(-8.69453705507356,13.3,3.54903238816311));
#106010=CARTESIAN_POINT('Ctrl Pts',(-8.70486643643529,13.3,3.60185630631317));
#106011=CARTESIAN_POINT('Ctrl Pts',(-8.70971531879739,13.3,3.62665323809881));
#106012=CARTESIAN_POINT('Ctrl Pts',(-8.71532619270893,13.3,3.65133335363798));
#106013=CARTESIAN_POINT('Ctrl Pts',(-8.72168558588098,13.3,3.67586495389262));
#106014=CARTESIAN_POINT('Ctrl Pts',(-8.72619429323909,13.3,3.69325746345788));
#106015=CARTESIAN_POINT('Ctrl Pts',(-8.73107929177658,13.3,3.71057528883275));
#106016=CARTESIAN_POINT('Ctrl Pts',(-8.73633631363297,13.3,3.72780656509595));
#106017=CARTESIAN_POINT('Ctrl Pts',(-8.73933492736524,13.3,3.73763531282399));
#106018=CARTESIAN_POINT('Ctrl Pts',(-8.74245220717161,13.3,3.74742793277564));
#106019=CARTESIAN_POINT('Ctrl Pts',(-8.74568498220576,13.3,3.75717712187213));
#106020=CARTESIAN_POINT('Ctrl Pts',(-8.76222845779434,13.3,3.80706784118373));
#106021=CARTESIAN_POINT('Ctrl Pts',(-8.78180660508961,13.3,3.85586874502093));
#106022=CARTESIAN_POINT('Ctrl Pts',(-8.80424653825476,13.3,3.90332080785399));
#106023=CARTESIAN_POINT('Ctrl Pts',(-8.82645061601556,13.3,3.95027412475122));
#106024=CARTESIAN_POINT('Ctrl Pts',(-8.85145745690028,13.3,3.99590765632431));
#106025=CARTESIAN_POINT('Ctrl Pts',(-8.8791380940311,13.3,4.03993822048699));
#106026=CARTESIAN_POINT('Ctrl Pts',(-8.89317285365425,13.3,4.06226279275655));
#106027=CARTESIAN_POINT('Ctrl Pts',(-8.90789551638605,13.3,4.08417468939178));
#106028=CARTESIAN_POINT('Ctrl Pts',(-8.92329211937121,13.3,4.10563273885798));
#106029=CARTESIAN_POINT('Ctrl Pts',(-8.93455023908675,13.3,4.12132303690524));
#106030=CARTESIAN_POINT('Ctrl Pts',(-8.94616873015292,13.3,4.13677061829437));
#106031=CARTESIAN_POINT('Ctrl Pts',(-8.95814263522597,13.3,4.15195823856277));
#106032=CARTESIAN_POINT('Ctrl Pts',(-8.9639302347199,13.3,4.15929919064508));
#106033=CARTESIAN_POINT('Ctrl Pts',(-8.96980032039377,13.3,4.16657853776216));
#106034=CARTESIAN_POINT('Ctrl Pts',(-8.97574395339132,13.3,4.17378460022058));
#106035=CARTESIAN_POINT('Ctrl Pts',(-9.00783287843214,13.3,4.2126892227238));
#106036=CARTESIAN_POINT('Ctrl Pts',(-9.04212471772084,13.3,4.24954017180012));
#106037=CARTESIAN_POINT('Ctrl Pts',(-9.07848924761864,13.3,4.28408550552319));
#106038=CARTESIAN_POINT('Ctrl Pts',(-9.11411291247182,13.3,4.31792703720943));
#106039=CARTESIAN_POINT('Ctrl Pts',(-9.15172641996041,13.3,4.34955652077773));
#106040=CARTESIAN_POINT('Ctrl Pts',(-9.19123107437835,13.3,4.37869353424287));
#106041=CARTESIAN_POINT('Ctrl Pts',(-9.23073572879629,13.3,4.407830547708));
#106042=CARTESIAN_POINT('Ctrl Pts',(-9.27213215627179,13.3,4.43447577192636));
#106043=CARTESIAN_POINT('Ctrl Pts',(-9.31533557546055,13.3,4.45829519891842));
#106044=CARTESIAN_POINT('Origin',(-10.,13.3,3.5));
#106045=CARTESIAN_POINT('Ctrl Pts',(-9.14640484551624,13.1319226084129,
4.69534642251162));
#106046=CARTESIAN_POINT('Ctrl Pts',(-8.74996755407482,13.158314057538,4.41226235778059));
#106047=CARTESIAN_POINT('Ctrl Pts',(-8.26764348151547,13.2110905918871,
3.4257644765553));
#106048=CARTESIAN_POINT('Ctrl Pts',(-9.12022709537494,13.2902522114602,
2.00399222931921));
#106049=CARTESIAN_POINT('Ctrl Pts',(-10.7745379170022,13.3694074671319,
1.94868204332565));
#106050=CARTESIAN_POINT('Ctrl Pts',(-11.723237150978,13.4485627228037,3.30369389649766));
#106051=CARTESIAN_POINT('Ctrl Pts',(-11.1031746725215,13.5277179784755,
4.8385355444873));
#106052=CARTESIAN_POINT('Ctrl Pts',(-9.47858070734822,13.6068732341472,
5.1540948536134));
#106053=CARTESIAN_POINT('Ctrl Pts',(-8.32878742394358,13.686028489819,3.96392887501833));
#106054=CARTESIAN_POINT('Ctrl Pts',(-8.70057184656685,13.7651837454908,
2.35120927629056));
#106055=CARTESIAN_POINT('Ctrl Pts',(-10.2554772506561,13.8443390011625,
1.78452309056729));
#106056=CARTESIAN_POINT('Ctrl Pts',(-11.5777671320349,13.9234942568343,
2.77970463020884));
#106057=CARTESIAN_POINT('Ctrl Pts',(-11.4635336479878,14.0026495125061,
4.43072368178711));
#106058=CARTESIAN_POINT('Ctrl Pts',(-10.0167777334889,14.0818047681778,
5.23432466554119));
#106059=CARTESIAN_POINT('Ctrl Pts',(-8.55474717092323,14.1609600238496,
4.45886123527889));
#106060=CARTESIAN_POINT('Ctrl Pts',(-8.4085918471124,14.2401152795213,2.81036935499744));
#106061=CARTESIAN_POINT('Ctrl Pts',(-9.71138439389651,14.3192705351931,
1.78977498532776));
#106062=CARTESIAN_POINT('Ctrl Pts',(-11.2769559220394,14.3984257908649,
2.32630786842705));
#106063=CARTESIAN_POINT('Ctrl Pts',(-11.6798828962121,14.4775810465366,
3.93146607007081));
#106064=CARTESIAN_POINT('Ctrl Pts',(-10.5533076620495,14.5567363022084,
5.14378220205025));
#106065=CARTESIAN_POINT('Ctrl Pts',(-8.92295610591595,14.6358915578802,
4.85946530170135));
#106066=CARTESIAN_POINT('Ctrl Pts',(-8.27323299078649,14.7150468135519,
3.33738044165135));
#106067=CARTESIAN_POINT('Ctrl Pts',(-9.19569915917786,14.7942020692237,
1.96335770044252));
#106068=CARTESIAN_POINT('Ctrl Pts',(-10.8504662952567,14.8733573248955,
1.9884192039403));
#106069=CARTESIAN_POINT('Ctrl Pts',(-11.7308996735887,14.9525125805672,
3.38974694470339));
#106070=CARTESIAN_POINT('Ctrl Pts',(-11.0353810597377,15.031667836239,4.89145803910818));
#106071=CARTESIAN_POINT('Ctrl Pts',(-9.39716722968648,15.1108230919107,
5.1262724457309));
#106072=CARTESIAN_POINT('Ctrl Pts',(-8.30782143563832,15.1899783475825,
3.88039600672407));
#106073=CARTESIAN_POINT('Ctrl Pts',(-8.75917278251741,15.2691336032543,
2.28817607231548));
#106074=CARTESIAN_POINT('Ctrl Pts',(-10.3402742552705,15.348288858926,1.7992993070502));
#106075=CARTESIAN_POINT('Ctrl Pts',(-11.6115623412065,15.4274441145978,
2.85887892249356));
#106076=CARTESIAN_POINT('Ctrl Pts',(-11.4155528595928,15.5065993702696,
4.50218736636369));
#106077=CARTESIAN_POINT('Ctrl Pts',(-9.93070880145079,15.5857546259413,
5.23302283466301));
#106078=CARTESIAN_POINT('Ctrl Pts',(-8.5089530920962,15.6649098816131,4.38597321294798));
#106079=CARTESIAN_POINT('Ctrl Pts',(-8.44476788752832,15.7440651372849,
2.73226144295864));
#106080=CARTESIAN_POINT('Ctrl Pts',(-9.79659262388905,15.8232203929566,
1.77756136394283));
#106081=CARTESIAN_POINT('Ctrl Pts',(-11.3336159967253,15.9023756486284,
2.39110965875215));
#106082=CARTESIAN_POINT('Ctrl Pts',(-11.656406784211,15.9815309043001,4.01428200518281));
#106083=CARTESIAN_POINT('Ctrl Pts',(-10.4710699720557,16.0606861599719,
5.16921014167275));
#106084=CARTESIAN_POINT('Ctrl Pts',(-8.85683270320632,16.1398414156437,
4.80435345944898));
#106085=CARTESIAN_POINT('Ctrl Pts',(-8.28342801711096,16.2189966713154,
3.25190718834359));
#106086=CARTESIAN_POINT('Ctrl Pts',(-9.27293022613473,16.2981519269872,
1.92534481248533));
#106087=CARTESIAN_POINT('Ctrl Pts',(-10.9244159547161,16.3773071826589,
2.03247672648724));
#106088=CARTESIAN_POINT('Ctrl Pts',(-11.7342381329274,16.4564624383307,
3.47576131324842));
#106089=CARTESIAN_POINT('Ctrl Pts',(-10.9650687146612,16.5356176940025,
4.94111477392245));
#106090=CARTESIAN_POINT('Ctrl Pts',(-9.31722216345621,16.6147729496742,
5.09436001002277));
#106091=CARTESIAN_POINT('Ctrl Pts',(-8.29103214585774,16.693928205346,3.79597008150099));
#106092=CARTESIAN_POINT('Ctrl Pts',(-8.82082560544542,16.7730834610178,
2.228104893137));
#106093=CARTESIAN_POINT('Ctrl Pts',(-10.4242354412573,16.8522387166895,
1.8182765667279));
#106094=CARTESIAN_POINT('Ctrl Pts',(-11.6413867904435,16.9313939723613,
2.93962617852609));
#106095=CARTESIAN_POINT('Ctrl Pts',(-11.3640859652301,17.010549228033,4.57118574257565));
#106096=CARTESIAN_POINT('Ctrl Pts',(-9.84481021449978,17.0897044837048,
5.22745059151099));
#106097=CARTESIAN_POINT('Ctrl Pts',(-8.4668318799151,17.1688597393766,4.31090377431026));
#106098=CARTESIAN_POINT('Ctrl Pts',(-8.48477463115914,17.2480149950483,
2.65604413785062));
#106099=CARTESIAN_POINT('Ctrl Pts',(-9.88230192661505,17.3271702507201,
1.76959063249279));
#106100=CARTESIAN_POINT('Ctrl Pts',(-11.3869911309622,17.4063255063919,
2.45864270383911));
#106101=CARTESIAN_POINT('Ctrl Pts',(-11.6288506819897,17.4854807620636,
4.0958312440758));
#106102=CARTESIAN_POINT('Ctrl Pts',(-10.3876719524339,17.5646360177354,
5.19052650760978));
#106103=CARTESIAN_POINT('Ctrl Pts',(-8.79352511344672,17.6437912734072,
4.7460287973203));
#106104=CARTESIAN_POINT('Ctrl Pts',(-8.29785124138321,17.7229465290789,
3.16704501929752));
#106105=CARTESIAN_POINT('Ctrl Pts',(-9.35195218673424,17.8021017847507,
1.89121056463045));
#106106=CARTESIAN_POINT('Ctrl Pts',(-10.9960886248091,17.8812570404224,
2.08014899825329));
#106107=CARTESIAN_POINT('Ctrl Pts',(-11.7333048781308,17.9604122960942,
3.56183538698199));
#106108=CARTESIAN_POINT('Ctrl Pts',(-10.8923792461265,18.0395675517659,
4.98722180481529));
#106109=CARTESIAN_POINT('Ctrl Pts',(-9.23895889165499,18.1187228074378,
5.05852040315301));
#106110=CARTESIAN_POINT('Ctrl Pts',(-8.27845232556989,18.1978780631095,
3.71081513299456));
#106111=CARTESIAN_POINT('Ctrl Pts',(-8.8853829292997,18.2770333187813,2.1711666013609));
#106112=CARTESIAN_POINT('Ctrl Pts',(-10.5071516654119,18.356188574453,1.84139618838458));
#106113=CARTESIAN_POINT('Ctrl Pts',(-11.6671682334563,18.4353438301248,
3.02175372767848));
#106114=CARTESIAN_POINT('Ctrl Pts',(-11.3092591022783,18.5144990857966,
4.63754561171706));
#106115=CARTESIAN_POINT('Ctrl Pts',(-9.75929388557313,18.5936543414683,
5.21762335280841));
#106116=CARTESIAN_POINT('Ctrl Pts',(-8.42848711353859,18.6728095971401,
4.23383694600431));
#106117=CARTESIAN_POINT('Ctrl Pts',(-8.52851362464164,18.7519648528118,
2.58190563514964));
#106118=CARTESIAN_POINT('Ctrl Pts',(-9.96830113909682,18.8311201084836,
1.76588218455242));
#106119=CARTESIAN_POINT('Ctrl Pts',(-11.4369498774138,18.9102753641554,
2.5287407836031));
#106120=CARTESIAN_POINT('Ctrl Pts',(-11.597282452041,18.9894306198272,4.17591285239826));
#106121=CARTESIAN_POINT('Ctrl Pts',(-10.30331903289,19.0685858754989,5.20767882809444));
#106122=CARTESIAN_POINT('Ctrl Pts',(-8.73318927020649,19.1477411311707,
4.68463496086992));
#106123=CARTESIAN_POINT('Ctrl Pts',(-8.31646713862804,19.2268963868424,
3.08300297325283));
#106124=CARTESIAN_POINT('Ctrl Pts',(-9.43257039592116,19.3060516425142,
1.86103903034569));
#106125=CARTESIAN_POINT('Ctrl Pts',(-11.0653077644253,19.385206898186,2.13131859708315));
#106126=CARTESIAN_POINT('Ctrl Pts',(-11.7281022077035,19.4643621538577,
3.64775714996454));
#106127=CARTESIAN_POINT('Ctrl Pts',(-10.8174917004099,19.5435174095295,
5.02966556325107));
#106128=CARTESIAN_POINT('Ctrl Pts',(-9.16257018955271,19.6226726652012,
5.01884190362575));
#106129=CARTESIAN_POINT('Ctrl Pts',(-8.27011296098191,19.701827920873,3.62514091206507));
#106130=CARTESIAN_POINT('Ctrl Pts',(-8.95268573873123,19.7809831765448,
2.11750144528891));
#106131=CARTESIAN_POINT('Ctrl Pts',(-10.5888186914164,19.8601384322165,
1.86860122463147));
#106132=CARTESIAN_POINT('Ctrl Pts',(-11.6888431662962,19.9392936878883,
3.10505927623311));
#106133=CARTESIAN_POINT('Ctrl Pts',(-11.2512073183408,20.01844894356,4.70110351850519));
#106134=CARTESIAN_POINT('Ctrl Pts',(-9.67437045548402,20.0976041992318,
5.20356532465696));
#106135=CARTESIAN_POINT('Ctrl Pts',(-8.39401324244765,20.1767594549036,
4.15496255633562));
#106136=CARTESIAN_POINT('Ctrl Pts',(-8.57587713162465,20.2559147105753,
2.51002855020681));
#106137=CARTESIAN_POINT('Ctrl Pts',(-10.0543784310982,20.3350699662471,
1.76644515464131));
#106138=CARTESIAN_POINT('Ctrl Pts',(-11.4833691794522,20.4142252219189,
2.60123123491824));
#106139=CARTESIAN_POINT('Ctrl Pts',(-11.5617798521189,20.4933804775906,
4.25432957594862));
#106140=CARTESIAN_POINT('Ctrl Pts',(-10.2182189885692,20.5725357332624,
5.22062485413386));
#106141=CARTESIAN_POINT('Ctrl Pts',(-8.67597379061322,20.6516909889342,
4.62032317323714));
#106142=CARTESIAN_POINT('Ctrl Pts',(-8.33922985482189,20.7308462446059,
2.99998805962229));
#106143=CARTESIAN_POINT('Ctrl Pts',(-9.51458627775735,20.8100015002777,
1.83490452709347));
#106144=CARTESIAN_POINT('Ctrl Pts',(-11.1319028754137,20.8891567559494,
2.18585948382011));
#106145=CARTESIAN_POINT('Ctrl Pts',(-11.7186429366803,20.9683120116212,
3.73331496273064));
#106146=CARTESIAN_POINT('Ctrl Pts',(-10.740590537881,21.047467267293,5.0683415032564));
#106147=CARTESIAN_POINT('Ctrl Pts',(-9.08824421511444,21.1266225229647,
4.97542224612582));
#106148=CARTESIAN_POINT('Ctrl Pts',(-8.26603459332348,21.2057777786365,
3.53915844844108));
#106149=CARTESIAN_POINT('Ctrl Pts',(-9.02256825582621,21.2849330343083,
2.06724161104649));
#106150=CARTESIAN_POINT('Ctrl Pts',(-10.6690353599237,21.36408828998,1.8998246649798));
#106151=CARTESIAN_POINT('Ctrl Pts',(-11.7063582000309,21.4432435456518,
3.18933762889195));
#106152=CARTESIAN_POINT('Ctrl Pts',(-11.1900736045309,21.5223988013236,
4.76170290933883));
#106153=CARTESIAN_POINT('Ctrl Pts',(-9.59024910463943,21.6015540569953,
5.18531113429732));
#106154=CARTESIAN_POINT('Ctrl Pts',(-8.36349518146937,21.6807093126671,
4.07447488592744));
#106155=CARTESIAN_POINT('Ctrl Pts',(-8.62674848798312,21.7598645683389,
2.44058992813047));
#106156=CARTESIAN_POINT('Ctrl Pts',(-10.1403217800601,21.8390198240106,
1.77127815607141));
#106157=CARTESIAN_POINT('Ctrl Pts',(-11.526134698685,21.9181750796824,2.6759355018536));
#106158=CARTESIAN_POINT('Ctrl Pts',(-11.522430330979,21.9973303353541,4.33088826141085));
#106159=CARTESIAN_POINT('Ctrl Pts',(-10.1325814349091,22.0764855910259,
5.22933269753159));
#106160=CARTESIAN_POINT('Ctrl Pts',(-8.62201960582365,22.1556408466977,
4.55325184495658));
#106161=CARTESIAN_POINT('Ctrl Pts',(-8.36608332164426,22.2347961023694,
2.91820475782117));
#106162=CARTESIAN_POINT('Ctrl Pts',(-9.59779781360324,22.3139513580411,
1.81287142846536));
#106163=CARTESIAN_POINT('Ctrl Pts',(-11.1957099230445,22.393106613713,2.24363731526574));
#106164=CARTESIAN_POINT('Ctrl Pts',(-11.7049503647936,22.4722618693847,
3.81829808229183));
#106165=CARTESIAN_POINT('Ctrl Pts',(-10.6618651788015,22.5514171250564,
5.10315435960114));
#106166=CARTESIAN_POINT('Ctrl Pts',(-9.01616404542407,22.6305723807283,
4.92836838045495));
#106167=CARTESIAN_POINT('Ctrl Pts',(-8.26622726836883,22.7097276364,3.45307953105006));
#106168=CARTESIAN_POINT('Ctrl Pts',(-9.09485834826755,22.7888828920717,
2.0205108969932));
#106169=CARTESIAN_POINT('Ctrl Pts',(-10.7476040843601,22.8680381477436,
1.93498960075163));
#106170=CARTESIAN_POINT('Ctrl Pts',(-11.7196701916628,22.9471934034153,
3.27438119455899));
#106171=CARTESIAN_POINT('Ctrl Pts',(-11.1260085443793,23.0263486590871,
4.81919451720226));
#106172=CARTESIAN_POINT('Ctrl Pts',(-9.50713703565121,23.1055039147588,
5.16290574620378));
#106173=CARTESIAN_POINT('Ctrl Pts',(-8.33700810572673,23.1846591704306,
3.9925721865046));
#106174=CARTESIAN_POINT('Ctrl Pts',(-8.68100238130063,23.2638144261023,
2.37376081282388));
#106175=CARTESIAN_POINT('Ctrl Pts',(-10.2259195084625,23.3429696817741,
1.78036927452147));
#106176=CARTESIAN_POINT('Ctrl Pts',(-11.5651410675949,23.4221249374458,
2.75266959436419));
#106177=CARTESIAN_POINT('Ctrl Pts',(-11.4793308685935,23.5012801931177,
4.4054002959104));
#106178=CARTESIAN_POINT('Ctrl Pts',(-10.0466172046406,23.5804354487894,
5.23378097889537));
#106179=CARTESIAN_POINT('Ctrl Pts',(-8.57145981851902,23.6595907044612,
4.48358605052702));
#106180=CARTESIAN_POINT('Ctrl Pts',(-8.39696100206443,23.7387459601329,
2.83785476917708));
#106181=CARTESIAN_POINT('Ctrl Pts',(-9.68200079264003,23.8179012158047,
1.79499351538082));
#106182=CARTESIAN_POINT('Ctrl Pts',(-11.2565702958328,23.8970564714764,
2.30451071544906));
#106183=CARTESIAN_POINT('Ctrl Pts',(-11.68706098934,23.9762117271482,3.90249537746301));
#106184=CARTESIAN_POINT('Ctrl Pts',(-10.5815042229309,24.05536698282,5.13402184238338));
#106185=CARTESIAN_POINT('Ctrl Pts',(-8.94651741854107,24.1345222384917,
4.87778957136504));
#106186=CARTESIAN_POINT('Ctrl Pts',(-8.27067096015597,24.2136774941635,
3.36712891673609));
#106187=CARTESIAN_POINT('Ctrl Pts',(-9.16941545665505,24.2928327498353,
1.97739998955691));
#106188=CARTESIAN_POINT('Ctrl Pts',(-10.8242593981243,24.371988005507,1.97405625657309));
#106189=CARTESIAN_POINT('Ctrl Pts',(-11.7288843588558,24.4511432611788,
3.35989062967651));
#106190=CARTESIAN_POINT('Ctrl Pts',(-11.0589050694329,24.5302985168505,
4.87360926711793));
#106191=CARTESIAN_POINT('Ctrl Pts',(-9.42574840582899,24.6094537725223,
5.13607197096169));
#106192=CARTESIAN_POINT('Ctrl Pts',(-8.3136275442009,24.6886090281941,3.91010675923693));
#106193=CARTESIAN_POINT('Ctrl Pts',(-8.74057475057857,24.7677748232262,
2.30812637245377));
#106194=CARTESIAN_POINT('Ctrl Pts',(-9.78464073208413,24.8205555330345,
1.96751243971017));
#106195=CARTESIAN_POINT('Ctrl Pts',(-10.2639206363603,24.8469511576188,
2.05506967699429));
#106196=CARTESIAN_POINT('Ctrl Pts',(-9.20319421055138,13.1883418974182,
4.61582047396927));
#106197=CARTESIAN_POINT('Ctrl Pts',(-8.83313174321593,13.2147333465434,
4.3515698857443));
#106198=CARTESIAN_POINT('Ctrl Pts',(-8.38289651005301,13.2675098808925,
3.43070333804874));
#106199=CARTESIAN_POINT('Ctrl Pts',(-9.17875805629518,13.3466715004656,
2.10352106443306));
#106200=CARTESIAN_POINT('Ctrl Pts',(-10.7230082002845,13.4258267561374,
2.05189064434031));
#106201=CARTESIAN_POINT('Ctrl Pts',(-11.6085908305356,13.5049820118091,
3.31675406783516));
#106202=CARTESIAN_POINT('Ctrl Pts',(-11.0297808758882,13.5841372674809,
4.74948327743878));
#106203=CARTESIAN_POINT('Ctrl Pts',(-9.51327053705405,13.6632925231527,
5.04404854424627));
#106204=CARTESIAN_POINT('Ctrl Pts',(-8.43997256895578,13.7424477788244,
3.93306386120543));
#106205=CARTESIAN_POINT('Ctrl Pts',(-8.78702231357646,13.8216030344962,
2.42763789167694));
#106206=CARTESIAN_POINT('Ctrl Pts',(-10.2384804451219,13.9007582901679,
1.89865312505424));
#106207=CARTESIAN_POINT('Ctrl Pts',(-11.4727988773174,13.9799135458397,
2.82762561063302));
#106208=CARTESIAN_POINT('Ctrl Pts',(-11.3661653040601,14.0590688015115,
4.36880298479835));
#106209=CARTESIAN_POINT('Ctrl Pts',(-10.0156615171812,14.1382240571832,
5.11894069691916));
#106210=CARTESIAN_POINT('Ctrl Pts',(-8.65089929883466,14.217379312855,4.39506855742421));
#106211=CARTESIAN_POINT('Ctrl Pts',(-8.51446763382406,14.2965345685268,
2.85625022279848));
#106212=CARTESIAN_POINT('Ctrl Pts',(-9.73058588177254,14.3756898241985,
1.90355561322882));
#106213=CARTESIAN_POINT('Ctrl Pts',(-11.1920005241443,14.4548450798703,
2.40439316512615));
#106214=CARTESIAN_POINT('Ctrl Pts',(-11.5681209180563,14.534000335542,3.90276079447873));
#106215=CARTESIAN_POINT('Ctrl Pts',(-10.5164963111043,14.6131555912138,
5.03442198951837));
#106216=CARTESIAN_POINT('Ctrl Pts',(-8.99461143167394,14.6923108468856,
4.76902058576619));
#106217=CARTESIAN_POINT('Ctrl Pts',(-8.38811415137153,14.7714661025573,
3.34819945979173));
#106218=CARTESIAN_POINT('Ctrl Pts',(-9.249208992039,14.8506213582291,2.06558993550106));
#106219=CARTESIAN_POINT('Ctrl Pts',(-10.793885092051,14.9297766139009,2.08898410658372));
#106220=CARTESIAN_POINT('Ctrl Pts',(-11.6157435683949,15.0089318695726,
3.39708203906353));
#106221=CARTESIAN_POINT('Ctrl Pts',(-10.966497546701,15.0880871252444,4.79888485836913));
#106222=CARTESIAN_POINT('Ctrl Pts',(-9.43727346748395,15.1672423809162,
5.01807715071069));
#106223=CARTESIAN_POINT('Ctrl Pts',(-8.42040143997807,15.2463976365879,
3.85508840326556));
#106224=CARTESIAN_POINT('Ctrl Pts',(-8.84172455126754,15.3255528922597,
2.36879826308837));
#106225=CARTESIAN_POINT('Ctrl Pts',(-10.3176359368674,15.4047081479315,
1.91244628540419));
#106226=CARTESIAN_POINT('Ctrl Pts',(-11.5043457039156,15.4838634036032,
2.90153246698827));
#106227=CARTESIAN_POINT('Ctrl Pts',(-11.3213766594965,15.563018659275,4.43551221728033));
#106228=CARTESIAN_POINT('Ctrl Pts',(-9.93531871886594,15.6421739149467,
5.11772547636037));
#106229=CARTESIAN_POINT('Ctrl Pts',(-8.60815188287271,15.7213291706185,
4.32702974784375));
#106230=CARTESIAN_POINT('Ctrl Pts',(-8.54823689585808,15.8004844262903,
2.7833388008119));
#106231=CARTESIAN_POINT('Ctrl Pts',(-9.81012524022611,15.879639681962,1.89215455948744));
#106232=CARTESIAN_POINT('Ctrl Pts',(-11.2448910253417,15.9587949376338,
2.46488371667913));
#106233=CARTESIAN_POINT('Ctrl Pts',(-11.5462066629694,16.0379501933055,
3.98006701653167));
#106234=CARTESIAN_POINT('Ctrl Pts',(-10.439729863739,16.1171054489773,5.05815821786802));
#106235=CARTESIAN_POINT('Ctrl Pts',(-8.93288719411203,16.1962607046491,
4.71757531367999));
#106236=CARTESIAN_POINT('Ctrl Pts',(-8.39763090642369,16.2754159603208,
3.26841270992457));
#106237=CARTESIAN_POINT('Ctrl Pts',(-9.32130190511764,16.3545712159926,
2.03010603070281));
#106238=CARTESIAN_POINT('Ctrl Pts',(-10.8629149084403,16.4337264716644,
2.1301104987027));
#106239=CARTESIAN_POINT('Ctrl Pts',(-11.6188599212877,16.5128817273361,
3.47737390397444));
#106240=CARTESIAN_POINT('Ctrl Pts',(-10.9008630555346,16.5920369830079,
4.84523794926625));
#106241=CARTESIAN_POINT('Ctrl Pts',(-9.36264711648426,16.6711922386796,
4.98828783736456));
#106242=CARTESIAN_POINT('Ctrl Pts',(-8.4047291353409,16.7503474943514,3.77627930313895));
#106243=CARTESIAN_POINT('Ctrl Pts',(-8.89927563504166,16.8295027500232,
2.31272359689913));
#106244=CARTESIAN_POINT('Ctrl Pts',(-10.3960112166845,16.908658005695,1.930160995123));
#106245=CARTESIAN_POINT('Ctrl Pts',(-11.5321859437461,16.9878132613667,
2.97690763840396));
#106246=CARTESIAN_POINT('Ctrl Pts',(-11.2733338382859,17.0669685170385,
4.49992015743727));
#106247=CARTESIAN_POINT('Ctrl Pts',(-9.85513493264302,17.1461237727102,
5.11252395245242));
#106248=CARTESIAN_POINT('Ctrl Pts',(-8.56883297911816,17.225279028382,4.25695465076404));
#106249=CARTESIAN_POINT('Ctrl Pts',(-8.58558200586084,17.3044342840538,
2.71219220438708));
#106250=CARTESIAN_POINT('Ctrl Pts',(-9.89013233523239,17.3835895397255,
1.88471411780712));
#106251=CARTESIAN_POINT('Ctrl Pts',(-11.2947151319445,17.4627447953973,
2.52792381364047));
#106252=CARTESIAN_POINT('Ctrl Pts',(-11.5204838578795,17.541900051069,4.05619081518931));
#106253=CARTESIAN_POINT('Ctrl Pts',(-10.36188028304,17.6210553067408,5.07805641398524));
#106254=CARTESIAN_POINT('Ctrl Pts',(-8.87379143452213,17.7002105624126,
4.66313096941719));
#106255=CARTESIAN_POINT('Ctrl Pts',(-8.41109455900217,17.7793658180843,
3.18919638911266));
#106256=CARTESIAN_POINT('Ctrl Pts',(-9.39506656435745,17.8585210737561,
1.99824272153759));
#106257=CARTESIAN_POINT('Ctrl Pts',(-10.9298192227108,17.9376763294279,
2.17461115213288));
#106258=CARTESIAN_POINT('Ctrl Pts',(-11.6179887555821,18.0168315850996,
3.55772150191017));
#106259=CARTESIAN_POINT('Ctrl Pts',(-10.8330095900408,18.0959868407714,
4.88827749671063));
#106260=CARTESIAN_POINT('Ctrl Pts',(-9.2895906707619,18.1751420964431,4.95483262607923));
#106261=CARTESIAN_POINT('Ctrl Pts',(-8.39298624577207,18.2542973521149,
3.69678968137423));
#106262=CARTESIAN_POINT('Ctrl Pts',(-8.95953798438631,18.3334526077867,
2.25957338829005));
#106263=CARTESIAN_POINT('Ctrl Pts',(-10.4734110555877,18.4126078634584,
1.95174247703412));
#106264=CARTESIAN_POINT('Ctrl Pts',(-11.5562521570384,18.4917631191302,
3.05357127255664));
#106265=CARTESIAN_POINT('Ctrl Pts',(-11.2221545859343,18.5709183748019,
4.56186512940809));
#106266=CARTESIAN_POINT('Ctrl Pts',(-9.77530797296171,18.6500736304738,
5.10335051624982));
#106267=CARTESIAN_POINT('Ctrl Pts',(-8.53303927564717,18.7292288861455,
4.18501504960061));
#106268=CARTESIAN_POINT('Ctrl Pts',(-8.62641106053443,18.8083841418173,
2.6429861084259));
#106269=CARTESIAN_POINT('Ctrl Pts',(-9.97041005240727,18.887539397489,1.88125239151542));
#106270=CARTESIAN_POINT('Ctrl Pts',(-11.341350141758,18.9666946531608,2.59335829448514));
#106271=CARTESIAN_POINT('Ctrl Pts',(-11.4910158504129,19.0458499088325,
4.13094462418708));
#106272=CARTESIAN_POINT('Ctrl Pts',(-10.2831393315521,19.1250051645043,
5.09406759703012));
#106273=CARTESIAN_POINT('Ctrl Pts',(-8.81746971227177,19.2041604201761,
4.6058216418476));
#106274=CARTESIAN_POINT('Ctrl Pts',(-8.42847194759504,19.2833156758479,
3.11074562882687));
#106275=CARTESIAN_POINT('Ctrl Pts',(-9.47032127436574,19.3624709315196,
1.97007848809699));
#106276=CARTESIAN_POINT('Ctrl Pts',(-10.9944332389656,19.4416261871914,
2.22237645677081));
#106277=CARTESIAN_POINT('Ctrl Pts',(-11.6131322168643,19.5207814428631,
3.63792692227193));
#106278=CARTESIAN_POINT('Ctrl Pts',(-10.7631042846145,19.5999366985349,
4.92789748783868));
#106279=CARTESIAN_POINT('Ctrl Pts',(-9.21828408032049,19.6790919542066,
4.91779392222309));
#106280=CARTESIAN_POINT('Ctrl Pts',(-8.38520169597802,19.7582472098784,
3.61681533418571));
#106281=CARTESIAN_POINT('Ctrl Pts',(-9.02236316318391,19.8374024655502,
2.209478554896));
#106282=CARTESIAN_POINT('Ctrl Pts',(-10.5496448050245,19.9165577212219,
1.97713757243713));
#106283=CARTESIAN_POINT('Ctrl Pts',(-11.5764850647372,19.9957129768937,
3.13133453425377));
#106284=CARTESIAN_POINT('Ctrl Pts',(-11.1679649653791,20.0748682325655,
4.62119455252864));
#106285=CARTESIAN_POINT('Ctrl Pts',(-9.69603446678095,20.1540234882372,
5.09022776343139));
#106286=CARTESIAN_POINT('Ctrl Pts',(-8.50085893825222,20.233178743909,4.11138814345296));
#106287=CARTESIAN_POINT('Ctrl Pts',(-8.67062349118661,20.3123339995808,
2.57589097894878));
#106288=CARTESIAN_POINT('Ctrl Pts',(-10.0507606545005,20.3914892552525,
1.88177790741573));
#106289=CARTESIAN_POINT('Ctrl Pts',(-11.384681185066,20.4706445109243,2.66102598330019));
#106290=CARTESIAN_POINT('Ctrl Pts',(-11.4578752251296,20.549799766596,4.20414431257134));
#106291=CARTESIAN_POINT('Ctrl Pts',(-10.2037009612183,20.6289550222678,
5.10615232881938));
#106292=CARTESIAN_POINT('Ctrl Pts',(-8.76406075704688,20.7081102779396,
4.54578849329186));
#106293=CARTESIAN_POINT('Ctrl Pts',(-8.44972026882971,20.7872655336113,
3.03325366622149));
#106294=CARTESIAN_POINT('Ctrl Pts',(-9.54688067038685,20.8664207892831,
1.94568270353057));
#106295=CARTESIAN_POINT('Ctrl Pts',(-11.0565978022317,20.9455760449549,
2.27328875879759));
#106296=CARTESIAN_POINT('Ctrl Pts',(-11.6043022675897,21.0247313006266,
3.71779260588845));
#106297=CARTESIAN_POINT('Ctrl Pts',(-10.6913193275462,21.1038865562984,
4.96400033208134));
#106298=CARTESIAN_POINT('Ctrl Pts',(-9.14890298504629,21.1830418119701,
4.87726295822911));
#106299=CARTESIAN_POINT('Ctrl Pts',(-8.38139466058816,21.2621970676419,
3.5365532515734));
#106300=CARTESIAN_POINT('Ctrl Pts',(-9.08759642266299,21.3413523233137,
2.16256248854919));
#106301=CARTESIAN_POINT('Ctrl Pts',(-10.6245246887038,21.4205075789854,
2.00628372902598));
#106302=CARTESIAN_POINT('Ctrl Pts',(-11.5928348298557,21.4996628346572,
3.2100058797634));
#106303=CARTESIAN_POINT('Ctrl Pts',(-11.1108984545884,21.578818090329,4.67776228865001));
#106304=CARTESIAN_POINT('Ctrl Pts',(-9.61750967781382,21.6579733460008,
5.07318801750046));
#106305=CARTESIAN_POINT('Ctrl Pts',(-8.47237123240889,21.7371286016725,
4.03625528752755));
#106306=CARTESIAN_POINT('Ctrl Pts',(-8.71811039531279,21.8162838573443,
2.51107208231946));
#106307=CARTESIAN_POINT('Ctrl Pts',(-10.1309862247346,21.895439113016,1.88628937107586));
#106308=CARTESIAN_POINT('Ctrl Pts',(-11.4246015303662,21.9745943686878,
2.7307602034137));
#106309=CARTESIAN_POINT('Ctrl Pts',(-11.4211436128521,22.0537496243595,
4.27560957744361));
#106310=CARTESIAN_POINT('Ctrl Pts',(-10.1237608418393,22.1329048800313,
5.11428084266634));
#106311=CARTESIAN_POINT('Ctrl Pts',(-8.71369612390732,22.2120601357031,
4.4831793952912));
#106312=CARTESIAN_POINT('Ctrl Pts',(-8.47478718458996,22.2912153913748,
2.95691137677308));
#106313=CARTESIAN_POINT('Ctrl Pts',(-9.62455617400543,22.3703706470466,
1.92511545867901));
#106314=CARTESIAN_POINT('Ctrl Pts',(-11.1161597909483,22.4495259027183,
2.32722265281731));
#106315=CARTESIAN_POINT('Ctrl Pts',(-11.5915206573679,22.5286811583902,
3.79712183042311));
#106316=CARTESIAN_POINT('Ctrl Pts',(-10.6178315370386,22.6078364140618,
4.99649710216846));
#106317=CARTESIAN_POINT('Ctrl Pts',(-9.08161828197361,22.6869916697337,
4.83333956856887));
#106318=CARTESIAN_POINT('Ctrl Pts',(-8.3815745170351,22.7661469254054,3.45620113222694));
#106319=CARTESIAN_POINT('Ctrl Pts',(-9.15507708240484,22.8453021810772,
2.11894075135078));
#106320=CARTESIAN_POINT('Ctrl Pts',(-10.6978662654123,22.9244574367489,
2.03910915482813));
#106321=CARTESIAN_POINT('Ctrl Pts',(-11.605261179684,23.0036126924207,3.28939152894722));
#106322=CARTESIAN_POINT('Ctrl Pts',(-11.0510956188272,23.0827679480924,
4.73142900143493));
#106323=CARTESIAN_POINT('Ctrl Pts',(-9.53992702356022,23.1619232037643,
5.0522732514618));
#106324=CARTESIAN_POINT('Ctrl Pts',(-8.4476463318674,23.2410784594359,3.95980154393634));
#106325=CARTESIAN_POINT('Ctrl Pts',(-8.76875479748452,23.3202337151078,
2.4486890829546));
#106326=CARTESIAN_POINT('Ctrl Pts',(-10.2108891684152,23.3993889707795,
1.89477566082987));
#106327=CARTESIAN_POINT('Ctrl Pts',(-11.4610128202023,23.4785442264513,
2.80238920556933));
#106328=CARTESIAN_POINT('Ctrl Pts',(-11.3809115415121,23.5576994821231,
4.34516435427308));
#106329=CARTESIAN_POINT('Ctrl Pts',(-10.0435157795242,23.6368547377948,
5.1184331815417));
#106330=CARTESIAN_POINT('Ctrl Pts',(-8.66650006026283,23.7160099934666,
4.41814844));
#106331=CARTESIAN_POINT('Ctrl Pts',(-8.50361058452884,23.7951652491383,
2.8819070426957));
#106332=CARTESIAN_POINT('Ctrl Pts',(-9.70315716047176,23.8743205048101,
1.90842695643741));
#106333=CARTESIAN_POINT('Ctrl Pts',(-11.1729711459929,23.9534757604818,
2.38404616854922));
#106334=CARTESIAN_POINT('Ctrl Pts',(-11.5748214553443,24.0326310161536,
3.87571751116932));
#106335=CARTESIAN_POINT('Ctrl Pts',(-10.5428169653803,24.1117862718254,
5.02531098291438));
#106336=CARTESIAN_POINT('Ctrl Pts',(-9.01660521901929,24.1909415274972,
4.78612574865134));
#106337=CARTESIAN_POINT('Ctrl Pts',(-8.38572257167664,24.2700967831689,
3.375968780002));
#106338=CARTESIAN_POINT('Ctrl Pts',(-9.22467393437342,24.3492520388406,
2.07869799639465));
#106339=CARTESIAN_POINT('Ctrl Pts',(-10.7694217299418,24.4284072945125,
2.07557672071041));
#106340=CARTESIAN_POINT('Ctrl Pts',(-11.6138623317943,24.5075625501842,
3.36921205346196));
#106341=CARTESIAN_POINT('Ctrl Pts',(-10.9884565128663,24.586717805856,4.78222355847577));
#106342=CARTESIAN_POINT('Ctrl Pts',(-9.46395314871217,24.6658730615277,
5.02722471720835));
#106343=CARTESIAN_POINT('Ctrl Pts',(-8.42582127031864,24.7450283171995,
3.8828225105725));
#106344=CARTESIAN_POINT('Ctrl Pts',(-8.82436383940853,24.8241941122316,
2.38742127725138));
#106345=CARTESIAN_POINT('Ctrl Pts',(-9.79896850329409,24.8769748220399,
2.06946826152566));
#106346=CARTESIAN_POINT('Ctrl Pts',(-10.2463620955464,24.9033704466242,
2.15120034869797));
#106347=CARTESIAN_POINT('Ctrl Pts',(-9.25998357558652,13.2447611864237,
4.53629452542694));
#106348=CARTESIAN_POINT('Ctrl Pts',(-8.91629593235703,13.2711526355489,
4.290877413708));
#106349=CARTESIAN_POINT('Ctrl Pts',(-8.49814953859056,13.323929169898,3.43564219954219));
#106350=CARTESIAN_POINT('Ctrl Pts',(-9.23728901721539,13.4030907894711,
2.20304989954692));
#106351=CARTESIAN_POINT('Ctrl Pts',(-10.6714784835667,13.4822460451429,
2.15509924535495));
#106352=CARTESIAN_POINT('Ctrl Pts',(-11.4939445100931,13.5614013008146,
3.32981423917266));
#106353=CARTESIAN_POINT('Ctrl Pts',(-10.9563870792549,13.6405565564864,
4.66043101039028));
#106354=CARTESIAN_POINT('Ctrl Pts',(-9.54796036675987,13.7197118121582,
4.93400223487913));
#106355=CARTESIAN_POINT('Ctrl Pts',(-8.55115771396801,13.7988670678299,
3.90219884739254));
#106356=CARTESIAN_POINT('Ctrl Pts',(-8.87347278058603,13.8780223235017,
2.50406650706332));
#106357=CARTESIAN_POINT('Ctrl Pts',(-10.2214836395877,13.9571775791735,
2.0127831595412));
#106358=CARTESIAN_POINT('Ctrl Pts',(-11.3678306225998,14.0363328348452,
2.87554659105721));
#106359=CARTESIAN_POINT('Ctrl Pts',(-11.2687969601324,14.115488090517,4.30688228780959));
#106360=CARTESIAN_POINT('Ctrl Pts',(-10.0145453008736,14.1946433461887,
5.00355672829712));
#106361=CARTESIAN_POINT('Ctrl Pts',(-8.74705142674612,14.2737986018605,
4.33127587956952));
#106362=CARTESIAN_POINT('Ctrl Pts',(-8.62034342053574,14.3529538575323,
2.90213109059951));
#106363=CARTESIAN_POINT('Ctrl Pts',(-9.74978736964855,14.432109113204,2.01733624112986));
#106364=CARTESIAN_POINT('Ctrl Pts',(-11.1070451262493,14.5112643688758,
2.48247846182523));
#106365=CARTESIAN_POINT('Ctrl Pts',(-11.4563589399006,14.5904196245476,
3.87405551888664));
#106366=CARTESIAN_POINT('Ctrl Pts',(-10.479684960159,14.6695748802193,4.92506177698652));
#106367=CARTESIAN_POINT('Ctrl Pts',(-9.06626675743199,14.7487301358911,
4.678575869831));
#106368=CARTESIAN_POINT('Ctrl Pts',(-8.50299531195658,14.8278853915628,
3.35901847793213));
#106369=CARTESIAN_POINT('Ctrl Pts',(-9.30271882490017,14.9070406472346,
2.16782217055959));
#106370=CARTESIAN_POINT('Ctrl Pts',(-10.737303888845,14.9861959029064,2.18954900922713));
#106371=CARTESIAN_POINT('Ctrl Pts',(-11.5005874632012,15.0653511585781,
3.40441713342364));
#106372=CARTESIAN_POINT('Ctrl Pts',(-10.8976140336643,15.1445064142499,
4.70631167763009));
#106373=CARTESIAN_POINT('Ctrl Pts',(-9.4773797052814,15.2236616699217,4.90988185569045));
#106374=CARTESIAN_POINT('Ctrl Pts',(-8.53298144431783,15.3028169255934,
3.82978079980707));
#106375=CARTESIAN_POINT('Ctrl Pts',(-8.92427632001765,15.3819721812652,
2.44942045386124));
#106376=CARTESIAN_POINT('Ctrl Pts',(-10.2949976184642,15.4611274369369,
2.02559326375819));
#106377=CARTESIAN_POINT('Ctrl Pts',(-11.3971290666245,15.5402826926087,
2.94418601148299));
#106378=CARTESIAN_POINT('Ctrl Pts',(-11.2272004594,15.6194379482805,4.36883706819697));
#106379=CARTESIAN_POINT('Ctrl Pts',(-9.93992863628107,15.6985932039522,
5.00242811805772));
#106380=CARTESIAN_POINT('Ctrl Pts',(-8.7073506736492,15.777748459624,4.26808628273949));
#106381=CARTESIAN_POINT('Ctrl Pts',(-8.65170590418785,15.8569037152958,
2.83441615866517));
#106382=CARTESIAN_POINT('Ctrl Pts',(-9.82365785656318,15.9360589709675,
2.00674775503204));
#106383=CARTESIAN_POINT('Ctrl Pts',(-11.1561660539582,16.0152142266393,
2.5386577746061));
#106384=CARTESIAN_POINT('Ctrl Pts',(-11.436006541728,16.094369482311,3.94585202788052));
#106385=CARTESIAN_POINT('Ctrl Pts',(-10.4083897554222,16.1735247379828,
4.94710629406329));
#106386=CARTESIAN_POINT('Ctrl Pts',(-9.00894168501776,16.2526799936546,
4.63079716791098));
#106387=CARTESIAN_POINT('Ctrl Pts',(-8.51183379573641,16.3318352493264,
3.28491823150556));
#106388=CARTESIAN_POINT('Ctrl Pts',(-9.36967358410055,16.4109905049981,
2.13486724892028));
#106389=CARTESIAN_POINT('Ctrl Pts',(-10.8014138621645,16.4901457606699,
2.22774427091815));
#106390=CARTESIAN_POINT('Ctrl Pts',(-11.503481709648,16.5693010163416,3.47898649470048));
#106391=CARTESIAN_POINT('Ctrl Pts',(-10.836657396408,16.6484562720134,4.74936112461004));
#106392=CARTESIAN_POINT('Ctrl Pts',(-9.40807206951228,16.7276115276852,
4.88221566470634));
#106393=CARTESIAN_POINT('Ctrl Pts',(-8.51842612482407,16.8067667833569,
3.75658852477692));
#106394=CARTESIAN_POINT('Ctrl Pts',(-8.97772566463787,16.8859220390287,
2.39734230066127));
#106395=CARTESIAN_POINT('Ctrl Pts',(-10.3677869921117,16.9650772947004,
2.0420454235181));
#106396=CARTESIAN_POINT('Ctrl Pts',(-11.4229850970487,17.0442325503722,
3.01418909828181));
#106397=CARTESIAN_POINT('Ctrl Pts',(-11.1825817113415,17.123387806044,4.4286545722989));
#106398=CARTESIAN_POINT('Ctrl Pts',(-9.8654596507863,17.2025430617157,4.99759731339386));
#106399=CARTESIAN_POINT('Ctrl Pts',(-8.6708340783212,17.2816983173875,4.20300552721785));
#106400=CARTESIAN_POINT('Ctrl Pts',(-8.68638938056257,17.3608535730592,
2.76834027092352));
#106401=CARTESIAN_POINT('Ctrl Pts',(-9.89796274384974,17.440008828731,1.99983760312146));
#106402=CARTESIAN_POINT('Ctrl Pts',(-11.2024391329266,17.5191640844028,
2.59720492344182));
#106403=CARTESIAN_POINT('Ctrl Pts',(-11.4121170337693,17.5983193400746,
4.01655038630282));
#106404=CARTESIAN_POINT('Ctrl Pts',(-10.3360886136461,17.6774745957463,
4.96558632036072));
#106405=CARTESIAN_POINT('Ctrl Pts',(-8.95405775559752,17.7566298514181,
4.58023314151408));
#106406=CARTESIAN_POINT('Ctrl Pts',(-8.52433787662112,17.8357851070898,
3.2113477589278));
#106407=CARTESIAN_POINT('Ctrl Pts',(-9.43818094198068,17.9149403627616,
2.10527487844473));
#106408=CARTESIAN_POINT('Ctrl Pts',(-10.8635498206126,17.9940956184334,
2.26907330601246));
#106409=CARTESIAN_POINT('Ctrl Pts',(-11.5026726330335,18.0732508741052,
3.55360761683835));
#106410=CARTESIAN_POINT('Ctrl Pts',(-10.7736399339552,18.1524061297769,
4.78933318860598));
#106411=CARTESIAN_POINT('Ctrl Pts',(-9.34022244986883,18.2315613854487,
4.85114484900545));
#106412=CARTESIAN_POINT('Ctrl Pts',(-8.50752016597425,18.3107166411204,
3.68276422975389));
#106413=CARTESIAN_POINT('Ctrl Pts',(-9.03369303947292,18.3898718967922,
2.34798017521921));
#106414=CARTESIAN_POINT('Ctrl Pts',(-10.4396704457635,18.469027152464,2.06208876568365));
#106415=CARTESIAN_POINT('Ctrl Pts',(-11.4453360806203,18.5481824081357,
3.08538881743479));
#106416=CARTESIAN_POINT('Ctrl Pts',(-11.1350500695903,18.6273376638075,
4.48618464709913));
#106417=CARTESIAN_POINT('Ctrl Pts',(-9.7913220603503,18.7064929194792,4.98907767969123));
#106418=CARTESIAN_POINT('Ctrl Pts',(-8.63759143775575,18.785648175151,4.13619315319688));
#106419=CARTESIAN_POINT('Ctrl Pts',(-8.72430849642721,18.8648034308228,
2.70406658170217));
#106420=CARTESIAN_POINT('Ctrl Pts',(-9.97251896571771,18.9439586864945,
1.9966225984784));
#106421=CARTESIAN_POINT('Ctrl Pts',(-11.2457504061023,19.0231139421663,
2.65797580536718));
#106422=CARTESIAN_POINT('Ctrl Pts',(-11.3847492487849,19.1022691978381,
4.08597639597589));
#106423=CARTESIAN_POINT('Ctrl Pts',(-10.2629596302143,19.1814244535098,
4.98045636596579));
#106424=CARTESIAN_POINT('Ctrl Pts',(-8.90175015433707,19.2605797091816,
4.52700832282528));
#106425=CARTESIAN_POINT('Ctrl Pts',(-8.54047675656204,19.3397349648533,
3.13848828440091));
#106426=CARTESIAN_POINT('Ctrl Pts',(-9.5080721528103,19.4188902205251,2.07911794584829));
#106427=CARTESIAN_POINT('Ctrl Pts',(-10.9235587135059,19.4980454761969,
2.31343431645849));
#106428=CARTESIAN_POINT('Ctrl Pts',(-11.4981622260253,19.5772007318686,
3.62809669457932));
#106429=CARTESIAN_POINT('Ctrl Pts',(-10.7087168688192,19.6563559875404,
4.82612941242628));
#106430=CARTESIAN_POINT('Ctrl Pts',(-9.27399797108825,19.7355112432122,
4.81674594082043));
#106431=CARTESIAN_POINT('Ctrl Pts',(-8.50029043097417,19.8146664988839,
3.60848975630635));
#106432=CARTESIAN_POINT('Ctrl Pts',(-9.09204058763656,19.8938217545557,
2.30145566450311));
#106433=CARTESIAN_POINT('Ctrl Pts',(-10.5104709186327,19.9729770102274,
2.08567392024281));
#106434=CARTESIAN_POINT('Ctrl Pts',(-11.464126963178,20.0521322658992,3.15760979227444));
#106435=CARTESIAN_POINT('Ctrl Pts',(-11.0847226124176,20.131287521571,4.5412855865521));
#106436=CARTESIAN_POINT('Ctrl Pts',(-9.71769847807786,20.2104427772427,
4.97689020220581));
#106437=CARTESIAN_POINT('Ctrl Pts',(-8.60770463405684,20.2895980329145,
4.06781373057032));
#106438=CARTESIAN_POINT('Ctrl Pts',(-8.76536985074856,20.3687532885863,
2.64175340769075));
#106439=CARTESIAN_POINT('Ctrl Pts',(-10.0471428779031,20.447908544258,1.99711066019015));
#106440=CARTESIAN_POINT('Ctrl Pts',(-11.2859931906797,20.5270637999298,
2.72082073168215));
#106441=CARTESIAN_POINT('Ctrl Pts',(-11.3539705981402,20.6062190556016,
4.15395904919404));
#106442=CARTESIAN_POINT('Ctrl Pts',(-10.1891829338672,20.6853743112733,
4.99167980350491));
#106443=CARTESIAN_POINT('Ctrl Pts',(-8.85214772348058,20.7645295669451,
4.47125381334657));
#106444=CARTESIAN_POINT('Ctrl Pts',(-8.56021068283754,20.8436848226168,
3.06651927282067));
#106445=CARTESIAN_POINT('Ctrl Pts',(-9.57917506301629,20.9228400782886,
2.05646087996767));
#106446=CARTESIAN_POINT('Ctrl Pts',(-10.9812927290496,21.0019953339603,
2.36071803377508));
#106447=CARTESIAN_POINT('Ctrl Pts',(-11.4899615984991,21.0811505896321,
3.70227024904624));
#106448=CARTESIAN_POINT('Ctrl Pts',(-10.6420481172114,21.1603058453039,
4.85965916090628));
#106449=CARTESIAN_POINT('Ctrl Pts',(-9.20956175497811,21.2394611009757,
4.77910367033238));
#106450=CARTESIAN_POINT('Ctrl Pts',(-8.49675472785286,21.3186163566474,
3.53394805470571));
#106451=CARTESIAN_POINT('Ctrl Pts',(-9.15262458949975,21.3977716123192,
2.25788336605189));
#106452=CARTESIAN_POINT('Ctrl Pts',(-10.5800140174839,21.4769268679909,
2.11274279307217));
#106453=CARTESIAN_POINT('Ctrl Pts',(-11.4793114596804,21.5560821236627,
3.23067413063488));
#106454=CARTESIAN_POINT('Ctrl Pts',(-11.0317233046461,21.6352373793345,
4.59382166796118));
#106455=CARTESIAN_POINT('Ctrl Pts',(-9.64477025098822,21.7143926350062,
4.96106490070361));
#106456=CARTESIAN_POINT('Ctrl Pts',(-8.58124728334842,21.793547890678,3.99803568912767));
#106457=CARTESIAN_POINT('Ctrl Pts',(-8.80947230264245,21.8727031463497,
2.58155423650846));
#106458=CARTESIAN_POINT('Ctrl Pts',(-10.1216506694092,21.9518584020216,
2.0013005860803));
#106459=CARTESIAN_POINT('Ctrl Pts',(-11.3230683620472,22.0310136576933,
2.78558490497384));
#106460=CARTESIAN_POINT('Ctrl Pts',(-11.3198568947254,22.1101689133651,
4.22033089347637));
#106461=CARTESIAN_POINT('Ctrl Pts',(-10.1149402487698,22.1893241690368,
4.99922898780111));
#106462=CARTESIAN_POINT('Ctrl Pts',(-8.80537264199095,22.2684794247086,
4.41310694562581));
#106463=CARTESIAN_POINT('Ctrl Pts',(-8.58349104753574,22.3476346803803,
2.99561799572498));
#106464=CARTESIAN_POINT('Ctrl Pts',(-9.65131453440758,22.4267899360521,
2.03735948889266));
#106465=CARTESIAN_POINT('Ctrl Pts',(-11.036609658852,22.5059451917238,2.41080799036886));
#106466=CARTESIAN_POINT('Ctrl Pts',(-11.4780909499422,22.5851004473957,
3.77594557855443));
#106467=CARTESIAN_POINT('Ctrl Pts',(-10.5737978952759,22.6642557030673,
4.88983984473576));
#106468=CARTESIAN_POINT('Ctrl Pts',(-9.1470725185231,22.7434109587392,4.73831075668277));
#106469=CARTESIAN_POINT('Ctrl Pts',(-8.49692176570142,22.8225662144109,
3.45932273340382));
#106470=CARTESIAN_POINT('Ctrl Pts',(-9.21529581654213,22.9017214700827,
2.21737060570834));
#106471=CARTESIAN_POINT('Ctrl Pts',(-10.6481284464643,22.9808767257544,
2.14322870890463));
#106472=CARTESIAN_POINT('Ctrl Pts',(-11.4908521677052,23.0600319814262,
3.30440186333547));
#106473=CARTESIAN_POINT('Ctrl Pts',(-10.9761826932751,23.139187237098,4.64366348566761));
#106474=CARTESIAN_POINT('Ctrl Pts',(-9.5727170114692,23.2183424927698,4.94164075671982));
#106475=CARTESIAN_POINT('Ctrl Pts',(-8.55828455800811,23.2974977484415,
3.92703090136812));
#106476=CARTESIAN_POINT('Ctrl Pts',(-8.8565072136684,23.3766530041133,2.52361735308531));
#106477=CARTESIAN_POINT('Ctrl Pts',(-10.1958588283679,23.455808259785,2.00918204713828));
#106478=CARTESIAN_POINT('Ctrl Pts',(-11.3568845728098,23.5349635154568,
2.85210881677446));
#106479=CARTESIAN_POINT('Ctrl Pts',(-11.2824922144306,23.6141187711285,
4.28492841263576));
#106480=CARTESIAN_POINT('Ctrl Pts',(-10.0404143544081,23.6932740268003,
5.00308538418801));
#106481=CARTESIAN_POINT('Ctrl Pts',(-8.76154030200664,23.772429282472,4.35271082947298));
#106482=CARTESIAN_POINT('Ctrl Pts',(-8.61026016699327,23.8515845381438,
2.92595931621431));
#106483=CARTESIAN_POINT('Ctrl Pts',(-9.72431352830351,23.9307397938156,
2.021860397494));
#106484=CARTESIAN_POINT('Ctrl Pts',(-11.0893719961529,24.0098950494874,
2.46358162164939));
#106485=CARTESIAN_POINT('Ctrl Pts',(-11.4625819213487,24.0890503051591,
3.84893964487562));
#106486=CARTESIAN_POINT('Ctrl Pts',(-10.5041297078297,24.1682055608308,
4.91660012344537));
#106487=CARTESIAN_POINT('Ctrl Pts',(-9.08669301949751,24.2473608165027,
4.69446192593765));
#106488=CARTESIAN_POINT('Ctrl Pts',(-8.50077418319726,24.3265160721744,
3.38480864326793));
#106489=CARTESIAN_POINT('Ctrl Pts',(-9.27993241209184,24.4056713278462,
2.1799960032324));
#106490=CARTESIAN_POINT('Ctrl Pts',(-10.7145840617594,24.4848265835179,
2.17709718484775));
#106491=CARTESIAN_POINT('Ctrl Pts',(-11.4988403047328,24.5639818391897,
3.3785334772474));
#106492=CARTESIAN_POINT('Ctrl Pts',(-10.9180079562998,24.6431370948615,
4.69083784983361));
#106493=CARTESIAN_POINT('Ctrl Pts',(-9.50215789159537,24.7222923505332,
4.91837746345501));
#106494=CARTESIAN_POINT('Ctrl Pts',(-8.5380149964364,24.801447606205,3.85553826190807));
#106495=CARTESIAN_POINT('Ctrl Pts',(-8.90815292823849,24.8806134012371,
2.46671618204897));
#106496=CARTESIAN_POINT('Ctrl Pts',(-9.81329627450407,24.9333941110454,
2.17142408334115));
#106497=CARTESIAN_POINT('Ctrl Pts',(-10.2288035547324,24.9597897356297,
2.24733102040164));
#106498=CARTESIAN_POINT('Ctrl Pts',(-9.31677294062166,13.3011804754291,
4.45676857688459));
#106499=CARTESIAN_POINT('Ctrl Pts',(-8.99946012149813,13.3275719245543,
4.2301849416717));
#106500=CARTESIAN_POINT('Ctrl Pts',(-8.61340256712811,13.3803484589035,
3.44058106103564));
#106501=CARTESIAN_POINT('Ctrl Pts',(-9.29581997813561,13.4595100784765,
2.30257873466078));
#106502=CARTESIAN_POINT('Ctrl Pts',(-10.6199487668489,13.5386653341483,
2.25830784636961));
#106503=CARTESIAN_POINT('Ctrl Pts',(-11.3792981896508,13.6178205898201,
3.34287441051017));
#106504=CARTESIAN_POINT('Ctrl Pts',(-10.8829932826216,13.6969758454918,
4.57137874334175));
#106505=CARTESIAN_POINT('Ctrl Pts',(-9.5826501964657,13.7761311011636,4.82395592551201));
#106506=CARTESIAN_POINT('Ctrl Pts',(-8.6623428589802,13.8552863568353,3.87133383357965));
#106507=CARTESIAN_POINT('Ctrl Pts',(-8.95992324759565,13.9344416125071,
2.58049512244971));
#106508=CARTESIAN_POINT('Ctrl Pts',(-10.2044868340536,14.0135968681788,
2.12691319402816));
#106509=CARTESIAN_POINT('Ctrl Pts',(-11.2628623678821,14.0927521238507,
2.9234675714814));
#106510=CARTESIAN_POINT('Ctrl Pts',(-11.1714286162047,14.1719073795224,
4.24496159082084));
#106511=CARTESIAN_POINT('Ctrl Pts',(-10.0134290845659,14.2510626351942,
4.88817275967509));
#106512=CARTESIAN_POINT('Ctrl Pts',(-8.84320355465755,14.3302178908659,
4.26748320171483));
#106513=CARTESIAN_POINT('Ctrl Pts',(-8.72621920724741,14.4093731465377,
2.94801195840054));
#106514=CARTESIAN_POINT('Ctrl Pts',(-9.76898885752458,14.4885284022094,
2.13111686903091));
#106515=CARTESIAN_POINT('Ctrl Pts',(-11.0220897283542,14.5676836578812,
2.56056375852433));
#106516=CARTESIAN_POINT('Ctrl Pts',(-11.3445969617449,14.646838913553,3.84535024329455));
#106517=CARTESIAN_POINT('Ctrl Pts',(-10.4428736092137,14.7259941692247,
4.81570156445467));
#106518=CARTESIAN_POINT('Ctrl Pts',(-9.13792208319002,14.8051494248965,
4.58813115389582));
#106519=CARTESIAN_POINT('Ctrl Pts',(-8.61787647254162,14.8843046805683,
3.36983749607252));
#106520=CARTESIAN_POINT('Ctrl Pts',(-9.35622865776133,14.96345993624,2.27005440561813));
#106521=CARTESIAN_POINT('Ctrl Pts',(-10.680722685639,15.0426151919118,2.29011391187054));
#106522=CARTESIAN_POINT('Ctrl Pts',(-11.3854313580073,15.1217704475836,
3.41175222778377));
#106523=CARTESIAN_POINT('Ctrl Pts',(-10.8287305206277,15.2009257032553,
4.61373849689104));
#106524=CARTESIAN_POINT('Ctrl Pts',(-9.51748594307886,15.2800809589271,
4.80168656067022));
#106525=CARTESIAN_POINT('Ctrl Pts',(-8.64556144865758,15.3592362145988,
3.80447319634858));
#106526=CARTESIAN_POINT('Ctrl Pts',(-9.00682808876778,15.4383914702706,
2.53004264463413));
#106527=CARTESIAN_POINT('Ctrl Pts',(-10.2723593000609,15.5175467259424,
2.13874024211219));
#106528=CARTESIAN_POINT('Ctrl Pts',(-11.2899124293335,15.5967019816141,
2.98683955597768));
#106529=CARTESIAN_POINT('Ctrl Pts',(-11.1330242593036,15.6758572372859,
4.30216191911361));
#106530=CARTESIAN_POINT('Ctrl Pts',(-9.94453855369621,15.7550124929577,
4.88713075975507));
#106531=CARTESIAN_POINT('Ctrl Pts',(-8.80654946442569,15.8341677486294,
4.20914281763525));
#106532=CARTESIAN_POINT('Ctrl Pts',(-8.75517491251764,15.9133230043012,
2.88549351651843));
#106533=CARTESIAN_POINT('Ctrl Pts',(-9.83719047290022,15.9924782599729,
2.12134095057665));
#106534=CARTESIAN_POINT('Ctrl Pts',(-11.0674410825746,16.0716335156447,
2.61243183253307));
#106535=CARTESIAN_POINT('Ctrl Pts',(-11.3258064204865,16.1507887713165,
3.91163703922939));
#106536=CARTESIAN_POINT('Ctrl Pts',(-10.3770496471056,16.2299440269882,
4.83605437025856));
#106537=CARTESIAN_POINT('Ctrl Pts',(-9.08499617592348,16.30909928266,4.54401902214198));
#106538=CARTESIAN_POINT('Ctrl Pts',(-8.62603668504912,16.3882545383318,
3.30142375308653));
#106539=CARTESIAN_POINT('Ctrl Pts',(-9.41804526308345,16.4674097940035,
2.23962846713776));
#106540=CARTESIAN_POINT('Ctrl Pts',(-10.7399128158888,16.5465650496753,
2.32537804313361));
#106541=CARTESIAN_POINT('Ctrl Pts',(-11.3881034980083,16.625720305347,3.48059908542653));
#106542=CARTESIAN_POINT('Ctrl Pts',(-10.7724517372814,16.7048755610188,
4.65348429995384));
#106543=CARTESIAN_POINT('Ctrl Pts',(-9.45349702254033,16.7840308166906,
4.77614349204813));
#106544=CARTESIAN_POINT('Ctrl Pts',(-8.6321231143072,16.8631860723623,3.73689774641489));
#106545=CARTESIAN_POINT('Ctrl Pts',(-9.05617569423413,16.9423413280341,
2.4819610044234));
#106546=CARTESIAN_POINT('Ctrl Pts',(-10.3395627675389,17.0214965837059,
2.15392985191321));
#106547=CARTESIAN_POINT('Ctrl Pts',(-11.3137842503515,17.1006518393776,
3.05147055815968));
#106548=CARTESIAN_POINT('Ctrl Pts',(-11.0918295843972,17.1798070950494,
4.35738898716052));
#106549=CARTESIAN_POINT('Ctrl Pts',(-9.87578436892954,17.2589623507211,
4.88267067433529));
#106550=CARTESIAN_POINT('Ctrl Pts',(-8.77283517752426,17.3381176063929,
4.14905640367165));
#106551=CARTESIAN_POINT('Ctrl Pts',(-8.78719675526428,17.4172728620647,
2.82448833745998));
#106552=CARTESIAN_POINT('Ctrl Pts',(-9.90579315246707,17.4964281177364,
2.11496108843579));
#106553=CARTESIAN_POINT('Ctrl Pts',(-11.1101631339089,17.5755833734082,
2.66648603324317));
#106554=CARTESIAN_POINT('Ctrl Pts',(-11.3037502096591,17.6547386290799,
3.97690995741632));
#106555=CARTESIAN_POINT('Ctrl Pts',(-10.3102969442523,17.7338938847517,
4.85311622673618));
#106556=CARTESIAN_POINT('Ctrl Pts',(-9.03432407667294,17.8130491404235,
4.49733531361096));
#106557=CARTESIAN_POINT('Ctrl Pts',(-8.63758119424006,17.8922043960953,
3.23349912874295));
#106558=CARTESIAN_POINT('Ctrl Pts',(-9.48129531960395,17.971359651767,2.21230703535186));
#106559=CARTESIAN_POINT('Ctrl Pts',(-10.7972804185142,18.0505149074388,
2.36353545989204));
#106560=CARTESIAN_POINT('Ctrl Pts',(-11.387356510485,18.1296701631105,3.54949373176654));
#106561=CARTESIAN_POINT('Ctrl Pts',(-10.7142702778696,18.2088254187823,
4.69038888050132));
#106562=CARTESIAN_POINT('Ctrl Pts',(-9.39085422897575,18.2879806744541,
4.74745707193165));
#106563=CARTESIAN_POINT('Ctrl Pts',(-8.62205408617643,18.3671359301258,
3.66873877813356));
#106564=CARTESIAN_POINT('Ctrl Pts',(-9.10784809455951,18.4462911857976,
2.43638696214837));
#106565=CARTESIAN_POINT('Ctrl Pts',(-10.4059298359393,18.5254464414694,
2.17243505433318));
#106566=CARTESIAN_POINT('Ctrl Pts',(-11.3344200042023,18.6046016971411,
3.11720636231295));
#106567=CARTESIAN_POINT('Ctrl Pts',(-11.0479455532464,18.6837569528129,
4.41050416479016));
#106568=CARTESIAN_POINT('Ctrl Pts',(-9.80733614773888,18.7629122084847,
4.87480484313264));
#106569=CARTESIAN_POINT('Ctrl Pts',(-8.74214359986434,18.8420674641564,
4.08737125679317));
#106570=CARTESIAN_POINT('Ctrl Pts',(-8.82220593232,18.9212227198282,2.76514705497843));
#106571=CARTESIAN_POINT('Ctrl Pts',(-9.97462787902816,19.0003779754999,
2.11199280544139));
#106572=CARTESIAN_POINT('Ctrl Pts',(-11.1501506704466,19.0795332311717,
2.72259331624922));
#106573=CARTESIAN_POINT('Ctrl Pts',(-11.2784826471567,19.1586884868435,
4.0410081677647));
#106574=CARTESIAN_POINT('Ctrl Pts',(-10.2427799288765,19.2378437425152,
4.86684513490147));
#106575=CARTESIAN_POINT('Ctrl Pts',(-8.98603059640236,19.316998998187,4.44819500380294));
#106576=CARTESIAN_POINT('Ctrl Pts',(-8.65248156552903,19.3961542538588,
3.16623093997496));
#106577=CARTESIAN_POINT('Ctrl Pts',(-9.54582303125486,19.4753095095305,
2.18815740359959));
#106578=CARTESIAN_POINT('Ctrl Pts',(-10.8526841880462,19.5544647652023,
2.40449217614617));
#106579=CARTESIAN_POINT('Ctrl Pts',(-11.3831922351862,19.6336200208741,
3.6182664668867));
#106580=CARTESIAN_POINT('Ctrl Pts',(-10.6543294530239,19.7127752765458,
4.7243613370139));
#106581=CARTESIAN_POINT('Ctrl Pts',(-9.32971186185602,19.7919305322176,
4.71569795941777));
#106582=CARTESIAN_POINT('Ctrl Pts',(-8.61537916597029,19.8710857878893,
3.60016417842699));
#106583=CARTESIAN_POINT('Ctrl Pts',(-9.16171801208923,19.9502410435611,
2.39343277411021));
#106584=CARTESIAN_POINT('Ctrl Pts',(-10.4712970322408,20.0293962992329,
2.19421026804849));
#106585=CARTESIAN_POINT('Ctrl Pts',(-11.3517688616188,20.1085515549046,
3.18388505029508));
#106586=CARTESIAN_POINT('Ctrl Pts',(-11.0014802594559,20.1877068105764,
4.46137662057556));
#106587=CARTESIAN_POINT('Ctrl Pts',(-9.73936248937481,20.2668620662481,
4.86355264098023));
#106588=CARTESIAN_POINT('Ctrl Pts',(-8.71455032986141,20.34601732192,4.02423931768769));
#106589=CARTESIAN_POINT('Ctrl Pts',(-8.86011621031052,20.4251725775915,
2.70761583643271));
#106590=CARTESIAN_POINT('Ctrl Pts',(-10.0435251013056,20.5043278332634,
2.11244341296457));
#106591=CARTESIAN_POINT('Ctrl Pts',(-11.1873051962935,20.5834830889351,
2.78061548006411));
#106592=CARTESIAN_POINT('Ctrl Pts',(-11.250065971151,20.6626383446069,4.10377378581674));
#106593=CARTESIAN_POINT('Ctrl Pts',(-10.1746649065162,20.7417936002788,
4.87720727819045));
#106594=CARTESIAN_POINT('Ctrl Pts',(-8.94023468991426,20.8209488559505,
4.39671913340127));
#106595=CARTESIAN_POINT('Ctrl Pts',(-8.67070109684536,20.9001041116222,
3.09978487941987));
#106596=CARTESIAN_POINT('Ctrl Pts',(-9.61146945564575,20.979259367294,2.16723905640477));
#106597=CARTESIAN_POINT('Ctrl Pts',(-10.9059876558676,21.0584146229658,
2.44814730875257));
#106598=CARTESIAN_POINT('Ctrl Pts',(-11.3756209294084,21.1375698786376,
3.68674789220404));
#106599=CARTESIAN_POINT('Ctrl Pts',(-10.5927769068766,21.2167251343092,
4.75531798973122));
#106600=CARTESIAN_POINT('Ctrl Pts',(-9.27022052490997,21.2958803899811,
4.68094438243568));
#106601=CARTESIAN_POINT('Ctrl Pts',(-8.61211479511756,21.3750356456528,
3.53134285783803));
#106602=CARTESIAN_POINT('Ctrl Pts',(-9.2176527563365,21.4541909013246,2.35320424355459));
#106603=CARTESIAN_POINT('Ctrl Pts',(-10.5355033462641,21.5333461569963,
2.21920185711835));
#106604=CARTESIAN_POINT('Ctrl Pts',(-11.3657880895052,21.6125014126681,
3.25134238150634));
#106605=CARTESIAN_POINT('Ctrl Pts',(-10.9525481547035,21.6916566683399,
4.50988104727235));
#106606=CARTESIAN_POINT('Ctrl Pts',(-9.67203082416259,21.7708119240117,
4.84894178390677));
#106607=CARTESIAN_POINT('Ctrl Pts',(-8.69012333428795,21.8499671796834,
3.95981609072778));
#106608=CARTESIAN_POINT('Ctrl Pts',(-8.90083420997211,21.9291224353551,
2.65203639069745));
#106609=CARTESIAN_POINT('Ctrl Pts',(-10.1123151140836,22.0082776910269,
2.11631180108475));
#106610=CARTESIAN_POINT('Ctrl Pts',(-11.2215351937282,22.0874329466986,
2.84040960653396));
#106611=CARTESIAN_POINT('Ctrl Pts',(-11.2185701765987,22.1665882023705,
4.16505220950913));
#106612=CARTESIAN_POINT('Ctrl Pts',(-10.1061196557001,22.2457434580421,
4.88417713293588));
#106613=CARTESIAN_POINT('Ctrl Pts',(-8.89704916007462,22.324898713714,4.34303449596042));
#106614=CARTESIAN_POINT('Ctrl Pts',(-8.69219491048146,22.4040539693857,
3.0343246146769));
#106615=CARTESIAN_POINT('Ctrl Pts',(-9.67807289480975,22.4832092250576,
2.14960351910631));
#106616=CARTESIAN_POINT('Ctrl Pts',(-10.9570595267557,22.5623644807292,
2.49439332792044));
#106617=CARTESIAN_POINT('Ctrl Pts',(-11.3646612425165,22.6415197364011,
3.7547693266857));
#106618=CARTESIAN_POINT('Ctrl Pts',(-10.5297642535131,22.7206749920728,
4.78318258730308));
#106619=CARTESIAN_POINT('Ctrl Pts',(-9.21252675507264,22.7998302477446,
4.64328194479669));
#106620=CARTESIAN_POINT('Ctrl Pts',(-8.6122690143677,22.8789855034163,3.4624443345807));
#106621=CARTESIAN_POINT('Ctrl Pts',(-9.27551455067946,22.958140759088,2.31580046006593));
#106622=CARTESIAN_POINT('Ctrl Pts',(-10.5983906275165,23.0372960147598,
2.24734826298114));
#106623=CARTESIAN_POINT('Ctrl Pts',(-11.3764431557264,23.1164512704317,
3.3194121977237));
#106624=CARTESIAN_POINT('Ctrl Pts',(-10.9012697677231,23.1956065261034,
4.55589796990028));
#106625=CARTESIAN_POINT('Ctrl Pts',(-9.60550699937822,23.2747617817751,
4.83100826197783));
#106626=CARTESIAN_POINT('Ctrl Pts',(-8.66892278414878,23.3539170374469,
3.89426025879988));
#106627=CARTESIAN_POINT('Ctrl Pts',(-8.94425962985228,23.4330722931186,
2.59854562321601));
#106628=CARTESIAN_POINT('Ctrl Pts',(-10.1808284883205,23.5122275487905,
2.12358843344668));
#106629=CARTESIAN_POINT('Ctrl Pts',(-11.2527563254173,23.591382804462,2.90182842797959));
#106630=CARTESIAN_POINT('Ctrl Pts',(-11.1840728873491,23.670538060134,4.22469247099844));
#106631=CARTESIAN_POINT('Ctrl Pts',(-10.0373129292917,23.7496933158057,
4.88773758683433));
#106632=CARTESIAN_POINT('Ctrl Pts',(-8.85658054375048,23.8288485714775,
4.28727321894597));
#106633=CARTESIAN_POINT('Ctrl Pts',(-8.71690974945766,23.9080038271492,
2.97001158973293));
#106634=CARTESIAN_POINT('Ctrl Pts',(-9.74546989613527,23.9871590828211,
2.13529383855059));
#106635=CARTESIAN_POINT('Ctrl Pts',(-11.0057728463129,24.0663143384927,
2.54311707474954));
#106636=CARTESIAN_POINT('Ctrl Pts',(-11.3503423873531,24.1454695941646,
3.82216177858194));
#106637=CARTESIAN_POINT('Ctrl Pts',(-10.465442450279,24.2246248498363,4.80788926397637));
#106638=CARTESIAN_POINT('Ctrl Pts',(-9.15678081997574,24.3037801055081,
4.60279810322396));
#106639=CARTESIAN_POINT('Ctrl Pts',(-8.61582579471792,24.3829353611798,
3.39364850653384));
#106640=CARTESIAN_POINT('Ctrl Pts',(-9.33519088981022,24.4620906168515,
2.28129401007015));
#106641=CARTESIAN_POINT('Ctrl Pts',(-10.6597463935769,24.5412458725233,
2.27861764898507));
#106642=CARTESIAN_POINT('Ctrl Pts',(-11.3838182776712,24.620401128195,3.38785490103285));
#106643=CARTESIAN_POINT('Ctrl Pts',(-10.8475593997332,24.6995563838669,
4.59945214119144));
#106644=CARTESIAN_POINT('Ctrl Pts',(-9.54036263447855,24.7787116395386,
4.80953020970168));
#106645=CARTESIAN_POINT('Ctrl Pts',(-8.65020872255413,24.8578668952104,
3.82825401324364));
#106646=CARTESIAN_POINT('Ctrl Pts',(-8.99194201706846,24.9370326902426,
2.54601108684658));
#106647=CARTESIAN_POINT('Ctrl Pts',(-9.82762404571402,24.9898134000508,
2.27337990515665));
#106648=CARTESIAN_POINT('Ctrl Pts',(-10.2112450139185,25.0162090246351,
2.3434616921053));
#106649=CARTESIAN_POINT('Ctrl Pts',(-9.36563614293035,13.3013173138078,
2.18112163397617));
#106650=CARTESIAN_POINT('Ctrl Pts',(-9.36179253662721,13.301100711406,2.18297352663203));
#106651=CARTESIAN_POINT('Ctrl Pts',(-9.35795682031215,13.3008830480983,
2.18484156183112));
#106652=CARTESIAN_POINT('Ctrl Pts',(-9.35027234948581,13.3004438276433,
2.18862405105439));
#106653=CARTESIAN_POINT('Ctrl Pts',(-9.34643267341032,13.3002227704914,
2.19053427774748));
#106654=CARTESIAN_POINT('Ctrl Pts',(-9.34259215682144,13.3,2.1924652288649));
#106655=CARTESIAN_POINT('Origin',(-10.,13.3,3.5));
#106656=CARTESIAN_POINT('',(-10.,13.2,5.0635));
#106657=CARTESIAN_POINT('Origin',(-10.,13.2,3.5));
#106658=CARTESIAN_POINT('Origin',(-10.,13.3,5.0635));
#106659=CARTESIAN_POINT('Origin',(-10.,13.2,3.5));
#106660=CARTESIAN_POINT('',(-10.,13.2,0.95));
#106661=CARTESIAN_POINT('Origin',(-10.,13.2,3.5));
#106662=CARTESIAN_POINT('Origin',(-10.,25.025,3.5));
#106663=CARTESIAN_POINT('',(-11.1135,25.2,3.5));
#106664=CARTESIAN_POINT('',(-11.2885,25.025,3.5));
#106665=CARTESIAN_POINT('Origin',(-10.,25.2,3.5));
#106666=CARTESIAN_POINT('Origin',(-10.,25.2,3.5));
#106667=CARTESIAN_POINT('Origin',(-7.21791809774051,12.6,3.99055610190908));
#106668=CARTESIAN_POINT('',(-7.30151407930766,12.6,4.02978650022929));
#106669=CARTESIAN_POINT('',(-7.28305503829031,12.6,3.92510007650003));
#106670=CARTESIAN_POINT('Origin',(-10.,12.6,3.5));
#106671=CARTESIAN_POINT('',(-7.43949984216826,12.6,3.95148526193402));
#106672=CARTESIAN_POINT('',(-7.02412006173947,12.6,4.18719618236609));
#106673=CARTESIAN_POINT('',(-7.43949984216826,12.6,3.95148526193402));
#106674=CARTESIAN_POINT('Origin',(-6.96855264488606,10.2,3.87205770140218));
#106675=CARTESIAN_POINT('',(-7.28305503829031,10.5,3.92510007650003));
#106676=CARTESIAN_POINT('',(-7.28305503829031,13.2,3.92510007650003));
#106677=CARTESIAN_POINT('',(-7.43949984216826,10.35,3.95148526193402));
#106678=CARTESIAN_POINT('',(-7.43949984216826,10.2,3.95148526193402));
#106679=CARTESIAN_POINT('Ctrl Pts',(-7.28305503829031,10.5,3.92510007650003));
#106680=CARTESIAN_POINT('Ctrl Pts',(-7.36347059168573,10.422647555638,3.93866255499417));
#106681=CARTESIAN_POINT('Ctrl Pts',(-7.43949984216826,10.35,3.95148526193402));
#106682=CARTESIAN_POINT('Origin',(-7.43949984216826,10.2,3.95148526193402));
#106683=CARTESIAN_POINT('',(-7.30151407930766,10.5,4.02978650022929));
#106684=CARTESIAN_POINT('',(-7.30151407930766,13.2,4.02978650022929));
#106685=CARTESIAN_POINT('Ctrl Pts',(-7.43949984216826,10.35,3.95148526193402));
#106686=CARTESIAN_POINT('Ctrl Pts',(-7.37244134059122,10.4226475556382,
3.98953820017093));
#106687=CARTESIAN_POINT('Ctrl Pts',(-7.30151407930766,10.5,4.0297865002293));
#106688=CARTESIAN_POINT('Origin',(-10.,13.2,3.5));
#106689=CARTESIAN_POINT('',(-12.7494863164095,12.6,3.44684930972108));
#106690=CARTESIAN_POINT('',(-12.75,12.6,3.5));
#106691=CARTESIAN_POINT('Origin',(-10.,12.6,3.5));
#106692=CARTESIAN_POINT('',(-12.75,13.,3.5));
#106693=CARTESIAN_POINT('',(-12.75,13.2,3.5));
#106694=CARTESIAN_POINT('',(-10.,13.,0.75));
#106695=CARTESIAN_POINT('Origin',(-10.,13.,3.5));
#106696=CARTESIAN_POINT('Origin',(-10.,13.,3.5));
#106697=CARTESIAN_POINT('',(-12.7494863164095,12.6,3.55315069027892));
#106698=CARTESIAN_POINT('Origin',(-10.,12.6,3.5));
#106699=CARTESIAN_POINT('',(-12.7494863164095,10.5,3.55315069027892));
#106700=CARTESIAN_POINT('',(-12.7494863164095,13.2,3.55315069027892));
#106701=CARTESIAN_POINT('',(-12.7169449617097,10.5,3.92510007650003));
#106702=CARTESIAN_POINT('Origin',(-10.,10.5,3.5));
#106703=CARTESIAN_POINT('',(-12.7169449617097,12.6,3.92510007650003));
#106704=CARTESIAN_POINT('',(-12.7169449617097,13.2,3.92510007650003));
#106705=CARTESIAN_POINT('',(-12.6984859206923,12.6,4.0297865002293));
#106706=CARTESIAN_POINT('Origin',(-10.,12.6,3.5));
#106707=CARTESIAN_POINT('',(-12.6984859206923,10.5,4.02978650022929));
#106708=CARTESIAN_POINT('',(-12.6984859206923,13.2,4.02978650022929));
#106709=CARTESIAN_POINT('',(-12.6018506091889,10.5,4.39043439256555));
#106710=CARTESIAN_POINT('Origin',(-10.,10.5,3.5));
#106711=CARTESIAN_POINT('',(-12.6018506091889,12.6,4.39043439256555));
#106712=CARTESIAN_POINT('',(-12.6018506091889,13.2,4.39043439256555));
#106713=CARTESIAN_POINT('',(-12.5654933957747,12.6,4.49032501545511));
#106714=CARTESIAN_POINT('Origin',(-10.,12.6,3.5));
#106715=CARTESIAN_POINT('',(-12.5654933957747,10.5,4.49032501545511));
#106716=CARTESIAN_POINT('',(-12.5654933957747,13.2,4.49032501545511));
#106717=CARTESIAN_POINT('',(-12.4077003425078,10.5,4.82871331019451));
#106718=CARTESIAN_POINT('Origin',(-10.,10.5,3.5));
#106719=CARTESIAN_POINT('',(-12.4077003425078,12.6,4.82871331019451));
#106720=CARTESIAN_POINT('',(-12.4077003425078,13.2,4.82871331019451));
#106721=CARTESIAN_POINT('',(-12.3545496522288,12.6,4.92077300621495));
#106722=CARTESIAN_POINT('Origin',(-10.,12.6,3.5));
#106723=CARTESIAN_POINT('',(-12.3545496522288,10.5,4.92077300621495));
#106724=CARTESIAN_POINT('',(-12.3545496522288,13.2,4.92077300621495));
#106725=CARTESIAN_POINT('',(-12.1403933192747,10.5,5.22661994625458));
#106726=CARTESIAN_POINT('Origin',(-10.,10.5,3.5));
#106727=CARTESIAN_POINT('',(-12.1403933192747,12.6,5.22661994625458));
#106728=CARTESIAN_POINT('',(-12.1403933192747,13.2,5.22661994625458));
#106729=CARTESIAN_POINT('',(-12.0720641089596,12.6,5.30805152812679));
#106730=CARTESIAN_POINT('Origin',(-10.,12.6,3.5));
#106731=CARTESIAN_POINT('',(-12.0720641089596,10.5,5.30805152812679));
#106732=CARTESIAN_POINT('',(-12.0720641089596,13.2,5.30805152812679));
#106733=CARTESIAN_POINT('',(-11.8080515281268,10.5,5.57206410895956));
#106734=CARTESIAN_POINT('Origin',(-10.,10.5,3.5));
#106735=CARTESIAN_POINT('',(-11.8080515281268,12.6,5.57206410895956));
#106736=CARTESIAN_POINT('',(-11.8080515281268,13.2,5.57206410895956));
#106737=CARTESIAN_POINT('',(-11.7266199462546,12.6,5.64039331927471));
#106738=CARTESIAN_POINT('Origin',(-10.,12.6,3.5));
#106739=CARTESIAN_POINT('',(-11.7266199462546,10.5,5.64039331927471));
#106740=CARTESIAN_POINT('',(-11.7266199462546,13.2,5.64039331927471));
#106741=CARTESIAN_POINT('',(-11.420773006215,10.5,5.85454965222883));
#106742=CARTESIAN_POINT('Origin',(-10.,10.5,3.5));
#106743=CARTESIAN_POINT('',(-11.420773006215,12.6,5.85454965222883));
#106744=CARTESIAN_POINT('',(-11.420773006215,13.2,5.85454965222883));
#106745=CARTESIAN_POINT('',(-11.3287133101945,12.6,5.90770034250775));
#106746=CARTESIAN_POINT('Origin',(-10.,12.6,3.5));
#106747=CARTESIAN_POINT('',(-11.3287133101945,10.5,5.90770034250775));
#106748=CARTESIAN_POINT('',(-11.3287133101945,13.2,5.90770034250775));
#106749=CARTESIAN_POINT('',(-10.9903250154551,10.5,6.06549339577475));
#106750=CARTESIAN_POINT('Origin',(-10.,10.5,3.5));
#106751=CARTESIAN_POINT('',(-10.9903250154551,12.6,6.06549339577475));
#106752=CARTESIAN_POINT('',(-10.9903250154551,13.2,6.06549339577475));
#106753=CARTESIAN_POINT('',(-10.8904343925656,12.6,6.10185060918885));
#106754=CARTESIAN_POINT('Origin',(-10.,12.6,3.5));
#106755=CARTESIAN_POINT('',(-10.8904343925656,10.5,6.10185060918885));
#106756=CARTESIAN_POINT('',(-10.8904343925656,13.2,6.10185060918885));
#106757=CARTESIAN_POINT('',(-10.5297865002293,10.5,6.19848592069234));
#106758=CARTESIAN_POINT('Origin',(-10.,10.5,3.5));
#106759=CARTESIAN_POINT('',(-10.5297865002293,12.6,6.19848592069234));
#106760=CARTESIAN_POINT('',(-10.5297865002293,13.2,6.19848592069234));
#106761=CARTESIAN_POINT('',(-10.4251000765,12.6,6.21694496170969));
#106762=CARTESIAN_POINT('Origin',(-10.,12.6,3.5));
#106763=CARTESIAN_POINT('',(-10.4251000765,10.5,6.21694496170969));
#106764=CARTESIAN_POINT('',(-10.4251000765,13.2,6.21694496170969));
#106765=CARTESIAN_POINT('',(-10.0531506902789,10.5,6.24948631640946));
#106766=CARTESIAN_POINT('Origin',(-10.,10.5,3.5));
#106767=CARTESIAN_POINT('',(-10.0531506902789,12.6,6.24948631640946));
#106768=CARTESIAN_POINT('',(-10.0531506902789,13.2,6.24948631640946));
#106769=CARTESIAN_POINT('',(-9.94684930972108,12.6,6.24948631640946));
#106770=CARTESIAN_POINT('Origin',(-10.,12.6,3.5));
#106771=CARTESIAN_POINT('',(-9.94684930972108,10.5,6.24948631640946));
#106772=CARTESIAN_POINT('',(-9.94684930972108,13.2,6.24948631640946));
#106773=CARTESIAN_POINT('',(-9.57489992349997,10.5,6.21694496170969));
#106774=CARTESIAN_POINT('Origin',(-10.,10.5,3.5));
#106775=CARTESIAN_POINT('',(-9.57489992349997,12.6,6.21694496170969));
#106776=CARTESIAN_POINT('',(-9.57489992349997,13.2,6.21694496170969));
#106777=CARTESIAN_POINT('',(-9.47021349977071,12.6,6.19848592069234));
#106778=CARTESIAN_POINT('Origin',(-10.,12.6,3.5));
#106779=CARTESIAN_POINT('',(-9.47021349977071,10.5,6.19848592069234));
#106780=CARTESIAN_POINT('',(-9.47021349977071,13.2,6.19848592069234));
#106781=CARTESIAN_POINT('',(-9.10956560743445,10.5,6.10185060918886));
#106782=CARTESIAN_POINT('Origin',(-10.,10.5,3.5));
#106783=CARTESIAN_POINT('',(-9.10956560743445,12.6,6.10185060918886));
#106784=CARTESIAN_POINT('',(-9.10956560743445,13.2,6.10185060918886));
#106785=CARTESIAN_POINT('',(-9.0096749845449,12.6,6.06549339577475));
#106786=CARTESIAN_POINT('Origin',(-10.,12.6,3.5));
#106787=CARTESIAN_POINT('',(-9.0096749845449,10.5,6.06549339577475));
#106788=CARTESIAN_POINT('',(-9.0096749845449,13.2,6.06549339577475));
#106789=CARTESIAN_POINT('',(-8.67128668980549,10.5,5.90770034250775));
#106790=CARTESIAN_POINT('Origin',(-10.,10.5,3.5));
#106791=CARTESIAN_POINT('',(-8.67128668980549,12.6,5.90770034250775));
#106792=CARTESIAN_POINT('',(-8.67128668980549,13.2,5.90770034250775));
#106793=CARTESIAN_POINT('',(-8.57922699378505,12.6,5.85454965222883));
#106794=CARTESIAN_POINT('Origin',(-10.,12.6,3.5));
#106795=CARTESIAN_POINT('',(-8.57922699378505,10.5,5.85454965222883));
#106796=CARTESIAN_POINT('',(-8.57922699378505,13.2,5.85454965222883));
#106797=CARTESIAN_POINT('',(-8.27338005374542,10.5,5.64039331927471));
#106798=CARTESIAN_POINT('Origin',(-10.,10.5,3.5));
#106799=CARTESIAN_POINT('',(-8.27338005374542,12.6,5.64039331927471));
#106800=CARTESIAN_POINT('',(-8.27338005374542,13.2,5.64039331927471));
#106801=CARTESIAN_POINT('',(-8.19194847187321,12.6,5.57206410895956));
#106802=CARTESIAN_POINT('Origin',(-10.,12.6,3.5));
#106803=CARTESIAN_POINT('',(-8.19194847187321,10.5,5.57206410895956));
#106804=CARTESIAN_POINT('',(-8.19194847187321,13.2,5.57206410895956));
#106805=CARTESIAN_POINT('',(-7.92793589104044,10.5,5.30805152812679));
#106806=CARTESIAN_POINT('Origin',(-10.,10.5,3.5));
#106807=CARTESIAN_POINT('',(-7.92793589104044,12.6,5.30805152812679));
#106808=CARTESIAN_POINT('',(-7.92793589104044,13.2,5.30805152812679));
#106809=CARTESIAN_POINT('',(-7.85960668072529,12.6,5.22661994625458));
#106810=CARTESIAN_POINT('Origin',(-10.,12.6,3.5));
#106811=CARTESIAN_POINT('',(-7.85960668072529,10.5,5.22661994625458));
#106812=CARTESIAN_POINT('',(-7.85960668072529,13.2,5.22661994625458));
#106813=CARTESIAN_POINT('',(-7.64545034777117,10.5,4.92077300621495));
#106814=CARTESIAN_POINT('Origin',(-10.,10.5,3.5));
#106815=CARTESIAN_POINT('',(-7.64545034777117,12.6,4.92077300621495));
#106816=CARTESIAN_POINT('',(-7.64545034777117,13.2,4.92077300621495));
#106817=CARTESIAN_POINT('',(-7.59229965749225,12.6,4.82871331019451));
#106818=CARTESIAN_POINT('Origin',(-10.,12.6,3.5));
#106819=CARTESIAN_POINT('',(-7.59229965749225,10.5,4.82871331019451));
#106820=CARTESIAN_POINT('',(-7.59229965749225,13.2,4.82871331019451));
#106821=CARTESIAN_POINT('',(-7.43450660422526,10.5,4.49032501545511));
#106822=CARTESIAN_POINT('Origin',(-10.,10.5,3.5));
#106823=CARTESIAN_POINT('',(-7.43450660422526,12.6,4.49032501545511));
#106824=CARTESIAN_POINT('',(-7.43450660422526,13.2,4.49032501545511));
#106825=CARTESIAN_POINT('',(-7.39814939081115,12.6,4.39043439256555));
#106826=CARTESIAN_POINT('Origin',(-10.,12.6,3.5));
#106827=CARTESIAN_POINT('',(-7.39814939081115,10.5,4.39043439256555));
#106828=CARTESIAN_POINT('',(-7.39814939081115,13.2,4.39043439256555));
#106829=CARTESIAN_POINT('Origin',(-10.,10.5,3.5));
#106830=CARTESIAN_POINT('',(-7.25051368359054,10.5,3.55315069027892));
#106831=CARTESIAN_POINT('Origin',(-10.,10.5,3.5));
#106832=CARTESIAN_POINT('',(-7.25051368359054,12.6,3.55315069027892));
#106833=CARTESIAN_POINT('',(-7.25051368359054,13.2,3.55315069027892));
#106834=CARTESIAN_POINT('',(-7.25051368359054,12.6,3.44684930972108));
#106835=CARTESIAN_POINT('Origin',(-10.,12.6,3.5));
#106836=CARTESIAN_POINT('',(-7.25051368359054,10.5,3.44684930972108));
#106837=CARTESIAN_POINT('',(-7.25051368359054,13.2,3.44684930972108));
#106838=CARTESIAN_POINT('',(-7.28305503829031,10.5,3.07489992349997));
#106839=CARTESIAN_POINT('Origin',(-10.,10.5,3.5));
#106840=CARTESIAN_POINT('',(-7.28305503829031,12.6,3.07489992349997));
#106841=CARTESIAN_POINT('',(-7.28305503829031,13.2,3.07489992349997));
#106842=CARTESIAN_POINT('',(-7.30151407930766,12.6,2.9702134997707));
#106843=CARTESIAN_POINT('Origin',(-10.,12.6,3.5));
#106844=CARTESIAN_POINT('',(-7.30151407930766,10.5,2.9702134997707));
#106845=CARTESIAN_POINT('',(-7.30151407930766,13.2,2.9702134997707));
#106846=CARTESIAN_POINT('',(-7.39814939081114,10.5,2.60956560743445));
#106847=CARTESIAN_POINT('Origin',(-10.,10.5,3.5));
#106848=CARTESIAN_POINT('',(-7.39814939081114,12.6,2.60956560743445));
#106849=CARTESIAN_POINT('',(-7.39814939081114,13.2,2.60956560743445));
#106850=CARTESIAN_POINT('',(-7.43450660422525,12.6,2.50967498454489));
#106851=CARTESIAN_POINT('Origin',(-10.,12.6,3.5));
#106852=CARTESIAN_POINT('',(-7.43450660422525,10.5,2.50967498454489));
#106853=CARTESIAN_POINT('',(-7.43450660422525,13.2,2.50967498454489));
#106854=CARTESIAN_POINT('',(-7.59229965749225,10.5,2.17128668980549));
#106855=CARTESIAN_POINT('Origin',(-10.,10.5,3.5));
#106856=CARTESIAN_POINT('',(-7.59229965749225,12.6,2.17128668980549));
#106857=CARTESIAN_POINT('',(-7.59229965749225,13.2,2.17128668980549));
#106858=CARTESIAN_POINT('',(-7.64545034777117,12.6,2.07922699378505));
#106859=CARTESIAN_POINT('Origin',(-10.,12.6,3.5));
#106860=CARTESIAN_POINT('',(-7.64545034777117,10.5,2.07922699378505));
#106861=CARTESIAN_POINT('',(-7.64545034777117,13.2,2.07922699378505));
#106862=CARTESIAN_POINT('',(-7.85960668072529,10.5,1.77338005374542));
#106863=CARTESIAN_POINT('Origin',(-10.,10.5,3.5));
#106864=CARTESIAN_POINT('',(-7.85960668072529,12.6,1.77338005374542));
#106865=CARTESIAN_POINT('',(-7.85960668072529,13.2,1.77338005374542));
#106866=CARTESIAN_POINT('',(-7.92793589104044,12.6,1.69194847187321));
#106867=CARTESIAN_POINT('Origin',(-10.,12.6,3.5));
#106868=CARTESIAN_POINT('',(-7.92793589104044,10.5,1.69194847187321));
#106869=CARTESIAN_POINT('',(-7.92793589104044,13.2,1.69194847187321));
#106870=CARTESIAN_POINT('',(-8.19194847187321,10.5,1.42793589104044));
#106871=CARTESIAN_POINT('Origin',(-10.,10.5,3.5));
#106872=CARTESIAN_POINT('',(-8.19194847187321,12.6,1.42793589104044));
#106873=CARTESIAN_POINT('',(-8.19194847187321,13.2,1.42793589104044));
#106874=CARTESIAN_POINT('',(-8.27338005374542,12.6,1.35960668072529));
#106875=CARTESIAN_POINT('Origin',(-10.,12.6,3.5));
#106876=CARTESIAN_POINT('',(-8.27338005374542,10.5,1.35960668072529));
#106877=CARTESIAN_POINT('',(-8.27338005374542,13.2,1.35960668072529));
#106878=CARTESIAN_POINT('',(-8.57922699378505,10.5,1.14545034777117));
#106879=CARTESIAN_POINT('Origin',(-10.,10.5,3.5));
#106880=CARTESIAN_POINT('',(-8.57922699378505,12.6,1.14545034777117));
#106881=CARTESIAN_POINT('',(-8.57922699378505,13.2,1.14545034777117));
#106882=CARTESIAN_POINT('',(-8.67128668980549,12.6,1.09229965749225));
#106883=CARTESIAN_POINT('Origin',(-10.,12.6,3.5));
#106884=CARTESIAN_POINT('',(-8.67128668980549,10.5,1.09229965749225));
#106885=CARTESIAN_POINT('',(-8.67128668980549,13.2,1.09229965749225));
#106886=CARTESIAN_POINT('',(-9.00967498454489,10.5,0.934506604225252));
#106887=CARTESIAN_POINT('Origin',(-10.,10.5,3.5));
#106888=CARTESIAN_POINT('',(-9.00967498454489,12.6,0.934506604225254));
#106889=CARTESIAN_POINT('',(-9.00967498454489,13.2,0.934506604225252));
#106890=CARTESIAN_POINT('',(-9.10956560743445,12.6,0.898149390811144));
#106891=CARTESIAN_POINT('Origin',(-10.,12.6,3.5));
#106892=CARTESIAN_POINT('',(-9.10956560743445,10.5,0.898149390811144));
#106893=CARTESIAN_POINT('',(-9.10956560743445,13.2,0.898149390811144));
#106894=CARTESIAN_POINT('',(-9.47021349977071,10.5,0.801514079307658));
#106895=CARTESIAN_POINT('Origin',(-10.,10.5,3.5));
#106896=CARTESIAN_POINT('',(-9.4702134997707,12.6,0.801514079307658));
#106897=CARTESIAN_POINT('',(-9.47021349977071,13.2,0.801514079307658));
#106898=CARTESIAN_POINT('',(-9.57489992349997,12.6,0.783055038290311));
#106899=CARTESIAN_POINT('Origin',(-10.,12.6,3.5));
#106900=CARTESIAN_POINT('',(-9.57489992349997,10.5,0.783055038290311));
#106901=CARTESIAN_POINT('',(-9.57489992349997,13.2,0.783055038290311));
#106902=CARTESIAN_POINT('',(-9.94684930972108,10.5,0.750513683590538));
#106903=CARTESIAN_POINT('Origin',(-10.,10.5,3.5));
#106904=CARTESIAN_POINT('',(-9.94684930972108,12.6,0.750513683590538));
#106905=CARTESIAN_POINT('',(-9.94684930972108,13.2,0.750513683590538));
#106906=CARTESIAN_POINT('',(-10.0531506902789,12.6,0.750513683590537));
#106907=CARTESIAN_POINT('Origin',(-10.,12.6,3.5));
#106908=CARTESIAN_POINT('',(-10.0531506902789,10.5,0.750513683590537));
#106909=CARTESIAN_POINT('',(-10.0531506902789,13.2,0.750513683590537));
#106910=CARTESIAN_POINT('',(-10.4251000765,10.5,0.783055038290311));
#106911=CARTESIAN_POINT('Origin',(-10.,10.5,3.5));
#106912=CARTESIAN_POINT('',(-10.4251000765,12.6,0.78305503829031));
#106913=CARTESIAN_POINT('',(-10.4251000765,13.2,0.783055038290311));
#106914=CARTESIAN_POINT('',(-10.5297865002293,12.6,0.801514079307658));
#106915=CARTESIAN_POINT('Origin',(-10.,12.6,3.5));
#106916=CARTESIAN_POINT('',(-10.5297865002293,10.5,0.801514079307658));
#106917=CARTESIAN_POINT('',(-10.5297865002293,13.2,0.801514079307658));
#106918=CARTESIAN_POINT('',(-10.8904343925655,10.5,0.898149390811144));
#106919=CARTESIAN_POINT('Origin',(-10.,10.5,3.5));
#106920=CARTESIAN_POINT('',(-10.8904343925656,12.6,0.898149390811144));
#106921=CARTESIAN_POINT('',(-10.8904343925655,13.2,0.898149390811144));
#106922=CARTESIAN_POINT('',(-10.9903250154551,12.6,0.934506604225253));
#106923=CARTESIAN_POINT('Origin',(-10.,12.6,3.5));
#106924=CARTESIAN_POINT('',(-10.9903250154551,10.5,0.934506604225253));
#106925=CARTESIAN_POINT('',(-10.9903250154551,13.2,0.934506604225253));
#106926=CARTESIAN_POINT('',(-11.3287133101945,10.5,1.09229965749225));
#106927=CARTESIAN_POINT('Origin',(-10.,10.5,3.5));
#106928=CARTESIAN_POINT('',(-11.3287133101945,12.6,1.09229965749225));
#106929=CARTESIAN_POINT('',(-11.3287133101945,13.2,1.09229965749225));
#106930=CARTESIAN_POINT('',(-11.420773006215,12.6,1.14545034777117));
#106931=CARTESIAN_POINT('Origin',(-10.,12.6,3.5));
#106932=CARTESIAN_POINT('',(-11.420773006215,10.5,1.14545034777117));
#106933=CARTESIAN_POINT('',(-11.420773006215,13.2,1.14545034777117));
#106934=CARTESIAN_POINT('',(-11.7266199462546,10.5,1.35960668072529));
#106935=CARTESIAN_POINT('Origin',(-10.,10.5,3.5));
#106936=CARTESIAN_POINT('',(-11.7266199462546,12.6,1.35960668072529));
#106937=CARTESIAN_POINT('',(-11.7266199462546,13.2,1.35960668072529));
#106938=CARTESIAN_POINT('',(-11.8080515281268,12.6,1.42793589104044));
#106939=CARTESIAN_POINT('Origin',(-10.,12.6,3.5));
#106940=CARTESIAN_POINT('',(-11.8080515281268,10.5,1.42793589104044));
#106941=CARTESIAN_POINT('',(-11.8080515281268,13.2,1.42793589104044));
#106942=CARTESIAN_POINT('',(-12.0720641089596,10.5,1.69194847187321));
#106943=CARTESIAN_POINT('Origin',(-10.,10.5,3.5));
#106944=CARTESIAN_POINT('',(-12.0720641089596,12.6,1.69194847187321));
#106945=CARTESIAN_POINT('',(-12.0720641089596,13.2,1.69194847187321));
#106946=CARTESIAN_POINT('',(-12.1403933192747,12.6,1.77338005374542));
#106947=CARTESIAN_POINT('Origin',(-10.,12.6,3.5));
#106948=CARTESIAN_POINT('',(-12.1403933192747,10.5,1.77338005374542));
#106949=CARTESIAN_POINT('',(-12.1403933192747,13.2,1.77338005374542));
#106950=CARTESIAN_POINT('',(-12.3545496522288,10.5,2.07922699378504));
#106951=CARTESIAN_POINT('Origin',(-10.,10.5,3.5));
#106952=CARTESIAN_POINT('',(-12.3545496522288,12.6,2.07922699378504));
#106953=CARTESIAN_POINT('',(-12.3545496522288,13.2,2.07922699378504));
#106954=CARTESIAN_POINT('',(-12.4077003425078,12.6,2.17128668980549));
#106955=CARTESIAN_POINT('Origin',(-10.,12.6,3.5));
#106956=CARTESIAN_POINT('',(-12.4077003425078,10.5,2.17128668980549));
#106957=CARTESIAN_POINT('',(-12.4077003425078,13.2,2.17128668980549));
#106958=CARTESIAN_POINT('',(-12.5654933957747,10.5,2.50967498454489));
#106959=CARTESIAN_POINT('Origin',(-10.,10.5,3.5));
#106960=CARTESIAN_POINT('',(-12.5654933957747,12.6,2.50967498454489));
#106961=CARTESIAN_POINT('',(-12.5654933957747,13.2,2.50967498454489));
#106962=CARTESIAN_POINT('',(-12.6018506091889,12.6,2.60956560743445));
#106963=CARTESIAN_POINT('Origin',(-10.,12.6,3.5));
#106964=CARTESIAN_POINT('',(-12.6018506091889,10.5,2.60956560743445));
#106965=CARTESIAN_POINT('',(-12.6018506091889,13.2,2.60956560743445));
#106966=CARTESIAN_POINT('',(-12.6984859206923,10.5,2.9702134997707));
#106967=CARTESIAN_POINT('Origin',(-10.,10.5,3.5));
#106968=CARTESIAN_POINT('',(-12.6984859206923,12.6,2.9702134997707));
#106969=CARTESIAN_POINT('',(-12.6984859206923,13.2,2.9702134997707));
#106970=CARTESIAN_POINT('',(-12.7169449617097,12.6,3.07489992349997));
#106971=CARTESIAN_POINT('Origin',(-10.,12.6,3.5));
#106972=CARTESIAN_POINT('',(-12.7169449617097,10.5,3.07489992349997));
#106973=CARTESIAN_POINT('',(-12.7169449617097,13.2,3.07489992349997));
#106974=CARTESIAN_POINT('',(-12.7494863164095,10.5,3.44684930972108));
#106975=CARTESIAN_POINT('Origin',(-10.,10.5,3.5));
#106976=CARTESIAN_POINT('',(-12.7494863164095,13.2,3.44684930972108));
#106977=CARTESIAN_POINT('Origin',(-7.07921428367087,10.2,4.39281061781755));
#106978=CARTESIAN_POINT('',(-7.55679918595664,12.6,4.38925237264674));
#106979=CARTESIAN_POINT('',(-7.55679918595664,12.6,4.38925237264674));
#106980=CARTESIAN_POINT('',(-7.55679918595664,10.35,4.38925237264674));
#106981=CARTESIAN_POINT('',(-7.55679918595664,10.2,4.38925237264674));
#106982=CARTESIAN_POINT('Ctrl Pts',(-7.39814939081114,10.5,4.39043439256555));
#106983=CARTESIAN_POINT('Ctrl Pts',(-7.47969835093245,10.4226475556384,
4.38982681223345));
#106984=CARTESIAN_POINT('Ctrl Pts',(-7.55679918595664,10.35,4.38925237264674));
#106985=CARTESIAN_POINT('Origin',(-7.55679918595664,10.2,4.38925237264674));
#106986=CARTESIAN_POINT('Ctrl Pts',(-7.55679918595664,10.35,4.38925237264674));
#106987=CARTESIAN_POINT('Ctrl Pts',(-7.49736727707808,10.4226475556379,
4.43837178784313));
#106988=CARTESIAN_POINT('Ctrl Pts',(-7.43450660422525,10.5,4.49032501545511));
#106989=CARTESIAN_POINT('',(-7.18866072953509,12.6,4.69351225646904));
#106990=CARTESIAN_POINT('Origin',(-7.34536834627981,12.6,4.46620690489502));
#106991=CARTESIAN_POINT('Origin',(-10.,10.35,3.5));
#106992=CARTESIAN_POINT('',(-12.6,10.35,3.5));
#106993=CARTESIAN_POINT('Ctrl Pts',(-12.6,10.35,3.5));
#106994=CARTESIAN_POINT('Ctrl Pts',(-12.6726475556384,10.4226475556384,
3.47416975799524));
#106995=CARTESIAN_POINT('Ctrl Pts',(-12.7494863164095,10.5,3.44684930972108));
#106996=CARTESIAN_POINT('',(-12.5605001578317,10.35,3.04851473806598));
#106997=CARTESIAN_POINT('Ctrl Pts',(-12.7169449617097,10.5,3.07489992349997));
#106998=CARTESIAN_POINT('Ctrl Pts',(-12.6365294083145,10.4226475556383,
3.06133744500587));
#106999=CARTESIAN_POINT('Ctrl Pts',(-12.5605001578317,10.35,3.04851473806598));
#107000=CARTESIAN_POINT('Ctrl Pts',(-12.5605001578317,10.35,3.04851473806598));
#107001=CARTESIAN_POINT('Ctrl Pts',(-12.627558659409,10.4226475556384,3.01046179982895));
#107002=CARTESIAN_POINT('Ctrl Pts',(-12.6984859206923,10.5,2.9702134997707));
#107003=CARTESIAN_POINT('',(-12.4432008140434,10.35,2.61074762735326));
#107004=CARTESIAN_POINT('Ctrl Pts',(-12.6018506091889,10.5,2.60956560743445));
#107005=CARTESIAN_POINT('Ctrl Pts',(-12.5203016490671,10.422647555638,2.61017318776655));
#107006=CARTESIAN_POINT('Ctrl Pts',(-12.4432008140434,10.35,2.61074762735326));
#107007=CARTESIAN_POINT('Ctrl Pts',(-12.4432008140434,10.35,2.61074762735326));
#107008=CARTESIAN_POINT('Ctrl Pts',(-12.5026327229221,10.4226475556382,
2.56162821215673));
#107009=CARTESIAN_POINT('Ctrl Pts',(-12.5654933957747,10.5,2.50967498454489));
#107010=CARTESIAN_POINT('',(-12.2516660498395,10.35,2.2));
#107011=CARTESIAN_POINT('Ctrl Pts',(-12.4077003425078,10.5,2.17128668980549));
#107012=CARTESIAN_POINT('Ctrl Pts',(-12.3274957995478,10.4226475556385,
2.1860458679428));
#107013=CARTESIAN_POINT('Ctrl Pts',(-12.2516660498395,10.35,2.2));
#107014=CARTESIAN_POINT('Ctrl Pts',(-12.2516660498395,10.35,2.2));
#107015=CARTESIAN_POINT('Ctrl Pts',(-12.3016655575428,10.4226475556383,
2.14130657641884));
#107016=CARTESIAN_POINT('Ctrl Pts',(-12.3545496522288,10.5,2.07922699378504));
#107017=CARTESIAN_POINT('',(-11.9917155521093,10.35,1.828752214815));
#107018=CARTESIAN_POINT('Ctrl Pts',(-12.1403933192747,10.5,1.77338005374542));
#107019=CARTESIAN_POINT('Ctrl Pts',(-12.063970167928,10.4226475556382,1.80184237952885));
#107020=CARTESIAN_POINT('Ctrl Pts',(-11.9917155521093,10.35,1.828752214815));
#107021=CARTESIAN_POINT('Ctrl Pts',(-11.9917155521093,10.35,1.828752214815));
#107022=CARTESIAN_POINT('Ctrl Pts',(-12.0307634488964,10.4226475556383,
1.76226815282458));
#107023=CARTESIAN_POINT('Ctrl Pts',(-12.0720641089596,10.5,1.69194847187321));
#107024=CARTESIAN_POINT('',(-11.671247785185,10.35,1.50828444789066));
#107025=CARTESIAN_POINT('Ctrl Pts',(-11.8080515281268,10.5,1.42793589104044));
#107026=CARTESIAN_POINT('Ctrl Pts',(-11.7377318471755,10.4226475556384,
1.46923655110355));
#107027=CARTESIAN_POINT('Ctrl Pts',(-11.671247785185,10.35,1.50828444789066));
#107028=CARTESIAN_POINT('Ctrl Pts',(-11.671247785185,10.35,1.50828444789066));
#107029=CARTESIAN_POINT('Ctrl Pts',(-11.6981576204711,10.4226475556381,
1.43602983207208));
#107030=CARTESIAN_POINT('Ctrl Pts',(-11.7266199462546,10.5,1.35960668072529));
#107031=CARTESIAN_POINT('',(-11.3,10.35,1.24833395016046));
#107032=CARTESIAN_POINT('Ctrl Pts',(-11.420773006215,10.5,1.14545034777117));
#107033=CARTESIAN_POINT('Ctrl Pts',(-11.3586934235811,10.4226475556382,
1.19833444245727));
#107034=CARTESIAN_POINT('Ctrl Pts',(-11.3,10.35,1.24833395016046));
#107035=CARTESIAN_POINT('Ctrl Pts',(-11.3,10.35,1.24833395016046));
#107036=CARTESIAN_POINT('Ctrl Pts',(-11.3139541320571,10.4226475556381,
1.17250420045271));
#107037=CARTESIAN_POINT('Ctrl Pts',(-11.3287133101945,10.5,1.09229965749225));
#107038=CARTESIAN_POINT('',(-10.8892523726467,10.35,1.05679918595664));
#107039=CARTESIAN_POINT('Ctrl Pts',(-10.9903250154551,10.5,0.934506604225252));
#107040=CARTESIAN_POINT('Ctrl Pts',(-10.9383717878433,10.4226475556382,
0.997367277077879));
#107041=CARTESIAN_POINT('Ctrl Pts',(-10.8892523726467,10.35,1.05679918595664));
#107042=CARTESIAN_POINT('Ctrl Pts',(-10.8892523726467,10.35,1.05679918595664));
#107043=CARTESIAN_POINT('Ctrl Pts',(-10.8898268122334,10.4226475556381,
0.9796983509328));
#107044=CARTESIAN_POINT('Ctrl Pts',(-10.8904343925655,10.5,0.898149390811143));
#107045=CARTESIAN_POINT('',(-10.451485261934,10.35,0.939499842168259));
#107046=CARTESIAN_POINT('Ctrl Pts',(-10.5297865002293,10.5,0.801514079307656));
#107047=CARTESIAN_POINT('Ctrl Pts',(-10.4895382001709,10.4226475556381,
0.87244134059127));
#107048=CARTESIAN_POINT('Ctrl Pts',(-10.451485261934,10.35,0.939499842168259));
#107049=CARTESIAN_POINT('Ctrl Pts',(-10.451485261934,10.35,0.939499842168259));
#107050=CARTESIAN_POINT('Ctrl Pts',(-10.4386625549941,10.4226475556383,
0.863470591685507));
#107051=CARTESIAN_POINT('Ctrl Pts',(-10.4251000765,10.5,0.783055038290308));
#107052=CARTESIAN_POINT('',(-10.,10.35,0.9));
#107053=CARTESIAN_POINT('Ctrl Pts',(-10.0531506902789,10.5,0.750513683590536));
#107054=CARTESIAN_POINT('Ctrl Pts',(-10.0258302420047,10.4226475556382,
0.827352444361817));
#107055=CARTESIAN_POINT('Ctrl Pts',(-10.,10.35,0.9));
#107056=CARTESIAN_POINT('Ctrl Pts',(-10.,10.35,0.9));
#107057=CARTESIAN_POINT('Ctrl Pts',(-9.97416975799534,10.4226475556381,
0.827352444361882));
#107058=CARTESIAN_POINT('Ctrl Pts',(-9.94684930972108,10.5,0.750513683590536));
#107059=CARTESIAN_POINT('',(-9.54851473806598,10.35,0.939499842168258));
#107060=CARTESIAN_POINT('Ctrl Pts',(-9.57489992349997,10.5,0.783055038290309));
#107061=CARTESIAN_POINT('Ctrl Pts',(-9.56133744500588,10.4226475556384,
0.863470591685391));
#107062=CARTESIAN_POINT('Ctrl Pts',(-9.54851473806598,10.35,0.939499842168258));
#107063=CARTESIAN_POINT('Ctrl Pts',(-9.54851473806598,10.35,0.939499842168258));
#107064=CARTESIAN_POINT('Ctrl Pts',(-9.51046179982901,10.4226475556383,
0.87244134059112));
#107065=CARTESIAN_POINT('Ctrl Pts',(-9.4702134997707,10.5,0.801514079307657));
#107066=CARTESIAN_POINT('',(-9.11074762735326,10.35,1.05679918595664));
#107067=CARTESIAN_POINT('Ctrl Pts',(-9.10956560743445,10.5,0.898149390811143));
#107068=CARTESIAN_POINT('Ctrl Pts',(-9.11017318776655,10.4226475556384,
0.979698350932521));
#107069=CARTESIAN_POINT('Ctrl Pts',(-9.11074762735326,10.35,1.05679918595664));
#107070=CARTESIAN_POINT('Ctrl Pts',(-9.11074762735326,10.35,1.05679918595664));
#107071=CARTESIAN_POINT('Ctrl Pts',(-9.06162821215675,10.4226475556381,
0.997367277077925));
#107072=CARTESIAN_POINT('Ctrl Pts',(-9.00967498454489,10.5,0.934506604225251));
#107073=CARTESIAN_POINT('',(-8.7,10.35,1.24833395016046));
#107074=CARTESIAN_POINT('Ctrl Pts',(-8.67128668980549,10.5,1.09229965749225));
#107075=CARTESIAN_POINT('Ctrl Pts',(-8.6860458679429,10.422647555638,1.17250420045278));
#107076=CARTESIAN_POINT('Ctrl Pts',(-8.7,10.35,1.24833395016046));
#107077=CARTESIAN_POINT('Ctrl Pts',(-8.7,10.35,1.24833395016046));
#107078=CARTESIAN_POINT('Ctrl Pts',(-8.64130657641881,10.4226475556384,
1.19833444245718));
#107079=CARTESIAN_POINT('Ctrl Pts',(-8.57922699378504,10.5,1.14545034777116));
#107080=CARTESIAN_POINT('',(-8.328752214815,10.35,1.50828444789066));
#107081=CARTESIAN_POINT('Ctrl Pts',(-8.27338005374542,10.5,1.35960668072529));
#107082=CARTESIAN_POINT('Ctrl Pts',(-8.30184237952875,10.4226475556385,
1.43602983207171));
#107083=CARTESIAN_POINT('Ctrl Pts',(-8.328752214815,10.35,1.50828444789066));
#107084=CARTESIAN_POINT('Ctrl Pts',(-8.328752214815,10.35,1.50828444789066));
#107085=CARTESIAN_POINT('Ctrl Pts',(-8.26226815282446,10.4226475556384,
1.46923655110356));
#107086=CARTESIAN_POINT('Ctrl Pts',(-8.19194847187321,10.5,1.42793589104044));
#107087=CARTESIAN_POINT('',(-8.00828444789066,10.35,1.828752214815));
#107088=CARTESIAN_POINT('Ctrl Pts',(-7.92793589104044,10.5,1.69194847187321));
#107089=CARTESIAN_POINT('Ctrl Pts',(-7.96923655110352,10.4226475556385,
1.76226815282441));
#107090=CARTESIAN_POINT('Ctrl Pts',(-8.00828444789066,10.35,1.828752214815));
#107091=CARTESIAN_POINT('Ctrl Pts',(-8.00828444789066,10.35,1.828752214815));
#107092=CARTESIAN_POINT('Ctrl Pts',(-7.93602983207183,10.4226475556384,
1.8018423795288));
#107093=CARTESIAN_POINT('Ctrl Pts',(-7.85960668072529,10.5,1.77338005374542));
#107094=CARTESIAN_POINT('',(-7.74833395016046,10.35,2.2));
#107095=CARTESIAN_POINT('Ctrl Pts',(-7.64545034777117,10.5,2.07922699378504));
#107096=CARTESIAN_POINT('Ctrl Pts',(-7.69833444245728,10.4226475556382,
2.14130657641894));
#107097=CARTESIAN_POINT('Ctrl Pts',(-7.74833395016046,10.35,2.2));
#107098=CARTESIAN_POINT('Ctrl Pts',(-7.74833395016046,10.35,2.2));
#107099=CARTESIAN_POINT('Ctrl Pts',(-7.67250420045245,10.4226475556383,
2.18604586794284));
#107100=CARTESIAN_POINT('Ctrl Pts',(-7.59229965749225,10.5,2.17128668980549));
#107101=CARTESIAN_POINT('',(-7.55679918595664,10.35,2.61074762735326));
#107102=CARTESIAN_POINT('Ctrl Pts',(-7.43450660422525,10.5,2.50967498454489));
#107103=CARTESIAN_POINT('Ctrl Pts',(-7.49736727707784,10.4226475556382,
2.56162821215668));
#107104=CARTESIAN_POINT('Ctrl Pts',(-7.55679918595664,10.35,2.61074762735326));
#107105=CARTESIAN_POINT('Ctrl Pts',(-7.55679918595664,10.35,2.61074762735326));
#107106=CARTESIAN_POINT('Ctrl Pts',(-7.47969835093274,10.4226475556382,
2.61017318776655));
#107107=CARTESIAN_POINT('Ctrl Pts',(-7.39814939081114,10.5,2.60956560743445));
#107108=CARTESIAN_POINT('',(-7.43949984216826,10.35,3.04851473806598));
#107109=CARTESIAN_POINT('Ctrl Pts',(-7.30151407930766,10.5,2.9702134997707));
#107110=CARTESIAN_POINT('Ctrl Pts',(-7.37244134059122,10.4226475556382,
3.01046179982907));
#107111=CARTESIAN_POINT('Ctrl Pts',(-7.43949984216826,10.35,3.04851473806598));
#107112=CARTESIAN_POINT('Ctrl Pts',(-7.43949984216826,10.35,3.04851473806598));
#107113=CARTESIAN_POINT('Ctrl Pts',(-7.36347059168553,10.4226475556382,
3.06133744500586));
#107114=CARTESIAN_POINT('Ctrl Pts',(-7.28305503829031,10.5,3.07489992349997));
#107115=CARTESIAN_POINT('',(-7.4,10.35,3.5));
#107116=CARTESIAN_POINT('Ctrl Pts',(-7.25051368359054,10.5,3.44684930972108));
#107117=CARTESIAN_POINT('Ctrl Pts',(-7.32735244436168,10.4226475556383,
3.47416975799527));
#107118=CARTESIAN_POINT('Ctrl Pts',(-7.4,10.35,3.5));
#107119=CARTESIAN_POINT('Ctrl Pts',(-7.4,10.35,3.5));
#107120=CARTESIAN_POINT('Ctrl Pts',(-7.32735244436169,10.4226475556383,
3.52583024200473));
#107121=CARTESIAN_POINT('Ctrl Pts',(-7.25051368359054,10.5,3.55315069027892));
#107122=CARTESIAN_POINT('',(-7.74833395016046,10.35,4.8));
#107123=CARTESIAN_POINT('Ctrl Pts',(-7.59229965749225,10.5,4.82871331019451));
#107124=CARTESIAN_POINT('Ctrl Pts',(-7.67250420045251,10.4226475556383,
4.81395413205715));
#107125=CARTESIAN_POINT('Ctrl Pts',(-7.74833395016046,10.35,4.8));
#107126=CARTESIAN_POINT('Ctrl Pts',(-7.74833395016046,10.35,4.8));
#107127=CARTESIAN_POINT('Ctrl Pts',(-7.6983344424572,10.4226475556383,4.85869342358116));
#107128=CARTESIAN_POINT('Ctrl Pts',(-7.64545034777117,10.5,4.92077300621496));
#107129=CARTESIAN_POINT('',(-8.00828444789066,10.35,5.171247785185));
#107130=CARTESIAN_POINT('Ctrl Pts',(-7.85960668072529,10.5,5.22661994625458));
#107131=CARTESIAN_POINT('Ctrl Pts',(-7.93602983207187,10.4226475556384,
5.19815762047119));
#107132=CARTESIAN_POINT('Ctrl Pts',(-8.00828444789066,10.35,5.171247785185));
#107133=CARTESIAN_POINT('Ctrl Pts',(-8.00828444789066,10.35,5.171247785185));
#107134=CARTESIAN_POINT('Ctrl Pts',(-7.96923655110368,10.4226475556382,
5.23773184717532));
#107135=CARTESIAN_POINT('Ctrl Pts',(-7.92793589104044,10.5,5.30805152812679));
#107136=CARTESIAN_POINT('',(-8.328752214815,10.35,5.49171555210934));
#107137=CARTESIAN_POINT('Ctrl Pts',(-8.19194847187321,10.5,5.57206410895956));
#107138=CARTESIAN_POINT('Ctrl Pts',(-8.26226815282441,10.4226475556384,
5.53076344889647));
#107139=CARTESIAN_POINT('Ctrl Pts',(-8.328752214815,10.35,5.49171555210934));
#107140=CARTESIAN_POINT('Ctrl Pts',(-8.328752214815,10.35,5.49171555210934));
#107141=CARTESIAN_POINT('Ctrl Pts',(-8.3018423795289,10.4226475556381,5.56397016792788));
#107142=CARTESIAN_POINT('Ctrl Pts',(-8.27338005374542,10.5,5.64039331927471));
#107143=CARTESIAN_POINT('',(-8.7,10.35,5.75166604983954));
#107144=CARTESIAN_POINT('Ctrl Pts',(-8.57922699378504,10.5,5.85454965222883));
#107145=CARTESIAN_POINT('Ctrl Pts',(-8.64130657641894,10.4226475556382,
5.80166555754271));
#107146=CARTESIAN_POINT('Ctrl Pts',(-8.7,10.35,5.75166604983954));
#107147=CARTESIAN_POINT('Ctrl Pts',(-8.7,10.35,5.75166604983954));
#107148=CARTESIAN_POINT('Ctrl Pts',(-8.68604586794282,10.4226475556384,
5.82749579954766));
#107149=CARTESIAN_POINT('Ctrl Pts',(-8.67128668980549,10.5,5.90770034250775));
#107150=CARTESIAN_POINT('',(-9.11074762735326,10.35,5.94320081404336));
#107151=CARTESIAN_POINT('Ctrl Pts',(-9.00967498454489,10.5,6.06549339577475));
#107152=CARTESIAN_POINT('Ctrl Pts',(-9.06162821215668,10.4226475556382,
6.00263272292216));
#107153=CARTESIAN_POINT('Ctrl Pts',(-9.11074762735326,10.35,5.94320081404336));
#107154=CARTESIAN_POINT('Ctrl Pts',(-9.11074762735326,10.35,5.94320081404336));
#107155=CARTESIAN_POINT('Ctrl Pts',(-9.11017318776655,10.4226475556383,
6.02030164906735));
#107156=CARTESIAN_POINT('Ctrl Pts',(-9.10956560743445,10.5,6.10185060918886));
#107157=CARTESIAN_POINT('',(-9.54851473806598,10.35,6.06050015783174));
#107158=CARTESIAN_POINT('Ctrl Pts',(-9.4702134997707,10.5,6.19848592069234));
#107159=CARTESIAN_POINT('Ctrl Pts',(-9.5104617998291,10.4226475556381,6.12755865940872));
#107160=CARTESIAN_POINT('Ctrl Pts',(-9.54851473806598,10.35,6.06050015783174));
#107161=CARTESIAN_POINT('Ctrl Pts',(-9.54851473806598,10.35,6.06050015783174));
#107162=CARTESIAN_POINT('Ctrl Pts',(-9.56133744500587,10.4226475556383,
6.13652940831454));
#107163=CARTESIAN_POINT('Ctrl Pts',(-9.57489992349997,10.5,6.21694496170969));
#107164=CARTESIAN_POINT('',(-10.,10.35,6.1));
#107165=CARTESIAN_POINT('Ctrl Pts',(-9.94684930972108,10.5,6.24948631640946));
#107166=CARTESIAN_POINT('Ctrl Pts',(-9.97416975799534,10.4226475556381,
6.17264755563811));
#107167=CARTESIAN_POINT('Ctrl Pts',(-10.,10.35,6.1));
#107168=CARTESIAN_POINT('Ctrl Pts',(-10.,10.35,6.1));
#107169=CARTESIAN_POINT('Ctrl Pts',(-10.0258302420047,10.4226475556382,
6.17264755563824));
#107170=CARTESIAN_POINT('Ctrl Pts',(-10.0531506902789,10.5,6.24948631640946));
#107171=CARTESIAN_POINT('',(-10.451485261934,10.35,6.06050015783174));
#107172=CARTESIAN_POINT('Ctrl Pts',(-10.4251000765,10.5,6.21694496170969));
#107173=CARTESIAN_POINT('Ctrl Pts',(-10.4386625549941,10.4226475556383,
6.13652940831459));
#107174=CARTESIAN_POINT('Ctrl Pts',(-10.451485261934,10.35,6.06050015783174));
#107175=CARTESIAN_POINT('Ctrl Pts',(-10.451485261934,10.35,6.06050015783174));
#107176=CARTESIAN_POINT('Ctrl Pts',(-10.4895382001709,10.4226475556381,
6.12755865940872));
#107177=CARTESIAN_POINT('Ctrl Pts',(-10.5297865002293,10.5,6.19848592069234));
#107178=CARTESIAN_POINT('',(-10.8892523726467,10.35,5.94320081404336));
#107179=CARTESIAN_POINT('Ctrl Pts',(-10.8904343925656,10.5,6.10185060918886));
#107180=CARTESIAN_POINT('Ctrl Pts',(-10.8898268122335,10.4226475556381,
6.02030164906721));
#107181=CARTESIAN_POINT('Ctrl Pts',(-10.8892523726467,10.35,5.94320081404336));
#107182=CARTESIAN_POINT('Ctrl Pts',(-10.8892523726467,10.35,5.94320081404336));
#107183=CARTESIAN_POINT('Ctrl Pts',(-10.9383717878434,10.4226475556383,
6.00263272292223));
#107184=CARTESIAN_POINT('Ctrl Pts',(-10.9903250154551,10.5,6.06549339577475));
#107185=CARTESIAN_POINT('',(-11.3,10.35,5.75166604983954));
#107186=CARTESIAN_POINT('Ctrl Pts',(-11.3287133101945,10.5,5.90770034250776));
#107187=CARTESIAN_POINT('Ctrl Pts',(-11.3139541320571,10.4226475556383,
5.8274957995475));
#107188=CARTESIAN_POINT('Ctrl Pts',(-11.3,10.35,5.75166604983954));
#107189=CARTESIAN_POINT('Ctrl Pts',(-11.3,10.35,5.75166604983954));
#107190=CARTESIAN_POINT('Ctrl Pts',(-11.358693423581,10.4226475556382,5.8016655575427));
#107191=CARTESIAN_POINT('Ctrl Pts',(-11.420773006215,10.5,5.85454965222883));
#107192=CARTESIAN_POINT('',(-11.671247785185,10.35,5.49171555210934));
#107193=CARTESIAN_POINT('Ctrl Pts',(-11.7266199462546,10.5,5.64039331927471));
#107194=CARTESIAN_POINT('Ctrl Pts',(-11.6981576204711,10.4226475556381,
5.56397016792789));
#107195=CARTESIAN_POINT('Ctrl Pts',(-11.671247785185,10.35,5.49171555210934));
#107196=CARTESIAN_POINT('Ctrl Pts',(-11.671247785185,10.35,5.49171555210934));
#107197=CARTESIAN_POINT('Ctrl Pts',(-11.7377318471755,10.4226475556384,
5.53076344889643));
#107198=CARTESIAN_POINT('Ctrl Pts',(-11.8080515281268,10.5,5.57206410895956));
#107199=CARTESIAN_POINT('',(-11.9917155521093,10.35,5.171247785185));
#107200=CARTESIAN_POINT('Ctrl Pts',(-12.0720641089596,10.5,5.30805152812679));
#107201=CARTESIAN_POINT('Ctrl Pts',(-12.0307634488963,10.4226475556381,
5.23773184717531));
#107202=CARTESIAN_POINT('Ctrl Pts',(-11.9917155521093,10.35,5.171247785185));
#107203=CARTESIAN_POINT('Ctrl Pts',(-11.9917155521093,10.35,5.171247785185));
#107204=CARTESIAN_POINT('Ctrl Pts',(-12.0639701679281,10.4226475556383,
5.19815762047119));
#107205=CARTESIAN_POINT('Ctrl Pts',(-12.1403933192747,10.5,5.22661994625458));
#107206=CARTESIAN_POINT('',(-12.2516660498395,10.35,4.8));
#107207=CARTESIAN_POINT('Ctrl Pts',(-12.3545496522288,10.5,4.92077300621495));
#107208=CARTESIAN_POINT('Ctrl Pts',(-12.3016655575427,10.4226475556382,
4.85869342358103));
#107209=CARTESIAN_POINT('Ctrl Pts',(-12.2516660498395,10.35,4.8));
#107210=CARTESIAN_POINT('Ctrl Pts',(-12.2516660498395,10.35,4.8));
#107211=CARTESIAN_POINT('Ctrl Pts',(-12.3274957995474,10.4226475556382,
4.81395413205714));
#107212=CARTESIAN_POINT('Ctrl Pts',(-12.4077003425078,10.5,4.82871331019451));
#107213=CARTESIAN_POINT('',(-12.4432008140434,10.35,4.38925237264674));
#107214=CARTESIAN_POINT('Ctrl Pts',(-12.5654933957747,10.5,4.49032501545511));
#107215=CARTESIAN_POINT('Ctrl Pts',(-12.5026327229219,10.4226475556379,
4.43837178784312));
#107216=CARTESIAN_POINT('Ctrl Pts',(-12.4432008140434,10.35,4.38925237264674));
#107217=CARTESIAN_POINT('Ctrl Pts',(-12.4432008140434,10.35,4.38925237264674));
#107218=CARTESIAN_POINT('Ctrl Pts',(-12.5203016490672,10.4226475556381,
4.38982681223345));
#107219=CARTESIAN_POINT('Ctrl Pts',(-12.6018506091889,10.5,4.39043439256555));
#107220=CARTESIAN_POINT('',(-12.5605001578317,10.35,3.95148526193402));
#107221=CARTESIAN_POINT('Ctrl Pts',(-12.6984859206923,10.5,4.0297865002293));
#107222=CARTESIAN_POINT('Ctrl Pts',(-12.6275586594092,10.4226475556386,
3.98953820017117));
#107223=CARTESIAN_POINT('Ctrl Pts',(-12.5605001578317,10.35,3.95148526193402));
#107224=CARTESIAN_POINT('Ctrl Pts',(-12.5605001578317,10.35,3.95148526193402));
#107225=CARTESIAN_POINT('Ctrl Pts',(-12.6365294083143,10.4226475556381,
3.93866255499416));
#107226=CARTESIAN_POINT('Ctrl Pts',(-12.7169449617097,10.5,3.92510007650003));
#107227=CARTESIAN_POINT('Ctrl Pts',(-12.7494863164095,10.5,3.55315069027892));
#107228=CARTESIAN_POINT('Ctrl Pts',(-12.6726475556383,10.4226475556383,
3.52583024200474));
#107229=CARTESIAN_POINT('Ctrl Pts',(-12.6,10.35,3.5));
#107230=CARTESIAN_POINT('',(-12.45,10.2,3.5));
#107231=CARTESIAN_POINT('',(-12.6,10.35,3.5));
#107232=CARTESIAN_POINT('Origin',(-10.,10.2,3.5));
#107233=CARTESIAN_POINT('Origin',(-7.55347823430896,12.6,4.9125));
#107234=CARTESIAN_POINT('',(-7.74833395016046,12.6,4.8));
#107235=CARTESIAN_POINT('',(-7.43862251845746,12.6,5.16356406460551));
#107236=CARTESIAN_POINT('',(-7.74833395016046,12.6,4.8));
#107237=CARTESIAN_POINT('Origin',(-7.27862251845746,10.2,4.88643593539449));
#107238=CARTESIAN_POINT('',(-7.74833395016046,10.2,4.8));
#107239=CARTESIAN_POINT('Origin',(-7.74833395016046,10.2,4.8));
#107240=CARTESIAN_POINT('Origin',(-7.56071843093727,10.2,5.33793509864491));
#107241=CARTESIAN_POINT('',(-8.00828444789066,12.6,5.171247785185));
#107242=CARTESIAN_POINT('',(-8.00828444789066,12.6,5.171247785185));
#107243=CARTESIAN_POINT('',(-8.00828444789066,10.2,5.171247785185));
#107244=CARTESIAN_POINT('Origin',(-8.00828444789066,10.2,5.171247785185));
#107245=CARTESIAN_POINT('',(-7.76641046603697,12.6,5.58306932044298));
#107246=CARTESIAN_POINT('Origin',(-7.83592444818889,12.6,5.31587499736447));
#107247=CARTESIAN_POINT('Origin',(-8.18412500263553,12.6,5.66407555181111));
#107248=CARTESIAN_POINT('',(-8.328752214815,12.6,5.49171555210934));
#107249=CARTESIAN_POINT('',(-8.16206490135509,12.6,5.93928156906273));
#107250=CARTESIAN_POINT('',(-8.328752214815,12.6,5.49171555210934));
#107251=CARTESIAN_POINT('Origin',(-7.91693067955702,10.2,5.73358953396304));
#107252=CARTESIAN_POINT('',(-8.328752214815,10.2,5.49171555210934));
#107253=CARTESIAN_POINT('Origin',(-8.328752214815,10.2,5.49171555210934));
#107254=CARTESIAN_POINT('Origin',(-8.33643593539449,10.2,6.06137748154254));
#107255=CARTESIAN_POINT('',(-8.7,12.6,5.75166604983954));
#107256=CARTESIAN_POINT('',(-8.7,12.6,5.75166604983954));
#107257=CARTESIAN_POINT('',(-8.7,10.2,5.75166604983954));
#107258=CARTESIAN_POINT('Origin',(-8.7,10.2,5.75166604983954));
#107259=CARTESIAN_POINT('',(-8.61356406460551,12.6,6.22137748154254));
#107260=CARTESIAN_POINT('Origin',(-8.5875,12.6,5.94652176569104));
#107261=CARTESIAN_POINT('Origin',(-9.03379309510499,12.6,6.15463165372019));
#107262=CARTESIAN_POINT('',(-9.11074762735326,12.6,5.94320081404336));
#107263=CARTESIAN_POINT('',(-9.10718938218246,12.6,6.42078571632913));
#107264=CARTESIAN_POINT('',(-9.11074762735326,12.6,5.94320081404336));
#107265=CARTESIAN_POINT('Origin',(-8.80648774353097,10.2,6.31133927046491));
#107266=CARTESIAN_POINT('',(-9.11074762735326,10.2,5.94320081404336));
#107267=CARTESIAN_POINT('Origin',(-9.11074762735326,10.2,5.94320081404336));
#107268=CARTESIAN_POINT('Origin',(-9.31280381763391,10.2,6.47587993826052));
#107269=CARTESIAN_POINT('',(-9.54851473806598,12.6,6.06050015783174));
#107270=CARTESIAN_POINT('',(-9.54851473806598,12.6,6.06050015783174));
#107271=CARTESIAN_POINT('',(-9.54851473806598,10.2,6.06050015783174));
#107272=CARTESIAN_POINT('Origin',(-9.54851473806598,10.2,6.06050015783174));
#107273=CARTESIAN_POINT('',(-9.62794229859782,12.6,6.53144735511394));
#107274=CARTESIAN_POINT('Origin',(-9.50944389809092,12.6,6.28208190225949));
#107275=CARTESIAN_POINT('Origin',(-10.,12.6,6.325));
#107276=CARTESIAN_POINT('',(-10.,12.6,6.1));
#107277=CARTESIAN_POINT('',(-10.16,12.6,6.55));
#107278=CARTESIAN_POINT('',(-10.,12.6,6.1));
#107279=CARTESIAN_POINT('Origin',(-9.84,10.2,6.55));
#107280=CARTESIAN_POINT('',(-10.,10.2,6.1));
#107281=CARTESIAN_POINT('Origin',(-10.,10.2,6.1));
#107282=CARTESIAN_POINT('Origin',(-10.3720577014022,10.2,6.53144735511395));
#107283=CARTESIAN_POINT('',(-10.451485261934,12.6,6.06050015783174));
#107284=CARTESIAN_POINT('',(-10.451485261934,12.6,6.06050015783174));
#107285=CARTESIAN_POINT('',(-10.451485261934,10.2,6.06050015783174));
#107286=CARTESIAN_POINT('Origin',(-10.451485261934,10.2,6.06050015783174));
#107287=CARTESIAN_POINT('',(-10.6871961823661,12.6,6.47587993826053));
#107288=CARTESIAN_POINT('Origin',(-10.4905561019091,12.6,6.28208190225949));
#107289=CARTESIAN_POINT('Origin',(-10.966206904895,12.6,6.15463165372019));
#107290=CARTESIAN_POINT('',(-10.8892523726467,12.6,5.94320081404336));
#107291=CARTESIAN_POINT('',(-11.193512256469,12.6,6.31133927046491));
#107292=CARTESIAN_POINT('',(-10.8892523726467,12.6,5.94320081404336));
#107293=CARTESIAN_POINT('Origin',(-10.8928106178175,10.2,6.42078571632913));
#107294=CARTESIAN_POINT('',(-10.8892523726467,10.2,5.94320081404336));
#107295=CARTESIAN_POINT('Origin',(-10.8892523726467,10.2,5.94320081404336));
#107296=CARTESIAN_POINT('Origin',(-11.3864359353945,10.2,6.22137748154254));
#107297=CARTESIAN_POINT('',(-11.3,12.6,5.75166604983954));
#107298=CARTESIAN_POINT('',(-11.3,12.6,5.75166604983954));
#107299=CARTESIAN_POINT('',(-11.3,10.2,5.75166604983954));
#107300=CARTESIAN_POINT('Origin',(-11.3,10.2,5.75166604983954));
#107301=CARTESIAN_POINT('',(-11.6635640646055,12.6,6.06137748154254));
#107302=CARTESIAN_POINT('Origin',(-11.4125,12.6,5.94652176569104));
#107303=CARTESIAN_POINT('Origin',(-11.8158749973645,12.6,5.66407555181111));
#107304=CARTESIAN_POINT('',(-11.671247785185,12.6,5.49171555210934));
#107305=CARTESIAN_POINT('',(-12.083069320443,12.6,5.73358953396303));
#107306=CARTESIAN_POINT('',(-11.671247785185,12.6,5.49171555210934));
#107307=CARTESIAN_POINT('Origin',(-11.8379350986449,10.2,5.93928156906273));
#107308=CARTESIAN_POINT('',(-11.671247785185,10.2,5.49171555210934));
#107309=CARTESIAN_POINT('Origin',(-11.671247785185,10.2,5.49171555210934));
#107310=CARTESIAN_POINT('Origin',(-12.233589533963,10.2,5.58306932044298));
#107311=CARTESIAN_POINT('',(-11.9917155521093,12.6,5.171247785185));
#107312=CARTESIAN_POINT('',(-11.9917155521093,12.6,5.171247785185));
#107313=CARTESIAN_POINT('',(-11.9917155521093,10.2,5.171247785185));
#107314=CARTESIAN_POINT('Origin',(-11.9917155521093,10.2,5.171247785185));
#107315=CARTESIAN_POINT('',(-12.4392815690627,12.6,5.33793509864491));
#107316=CARTESIAN_POINT('Origin',(-12.1640755518111,12.6,5.31587499736447));
#107317=CARTESIAN_POINT('Origin',(-12.446521765691,12.6,4.9125));
#107318=CARTESIAN_POINT('',(-12.2516660498395,12.6,4.8));
#107319=CARTESIAN_POINT('',(-12.7213774815425,12.6,4.88643593539449));
#107320=CARTESIAN_POINT('',(-12.2516660498395,12.6,4.8));
#107321=CARTESIAN_POINT('Origin',(-12.5613774815425,10.2,5.16356406460551));
#107322=CARTESIAN_POINT('',(-12.2516660498395,10.2,4.8));
#107323=CARTESIAN_POINT('Origin',(-12.2516660498395,10.2,4.8));
#107324=CARTESIAN_POINT('Origin',(-12.8113392704649,10.2,4.69351225646903));
#107325=CARTESIAN_POINT('',(-12.4432008140434,12.6,4.38925237264674));
#107326=CARTESIAN_POINT('',(-12.4432008140434,12.6,4.38925237264674));
#107327=CARTESIAN_POINT('',(-12.4432008140434,10.2,4.38925237264674));
#107328=CARTESIAN_POINT('Origin',(-12.4432008140434,10.2,4.38925237264674));
#107329=CARTESIAN_POINT('',(-12.9207857163291,12.6,4.39281061781754));
#107330=CARTESIAN_POINT('Origin',(-12.6546316537202,12.6,4.46620690489501));
#107331=CARTESIAN_POINT('Origin',(-12.7820819022595,12.6,3.99055610190908));
#107332=CARTESIAN_POINT('',(-12.5605001578317,12.6,3.95148526193402));
#107333=CARTESIAN_POINT('',(-13.0314473551139,12.6,3.87205770140218));
#107334=CARTESIAN_POINT('',(-12.5605001578317,12.6,3.95148526193402));
#107335=CARTESIAN_POINT('Origin',(-12.9758799382605,10.2,4.18719618236609));
#107336=CARTESIAN_POINT('',(-12.5605001578317,10.2,3.95148526193402));
#107337=CARTESIAN_POINT('Origin',(-12.5605001578317,10.2,3.95148526193402));
#107338=CARTESIAN_POINT('Origin',(-13.05,10.2,3.66));
#107339=CARTESIAN_POINT('',(-12.6,12.6,3.5));
#107340=CARTESIAN_POINT('',(-12.6,12.6,3.5));
#107341=CARTESIAN_POINT('',(-12.6,10.2,3.5));
#107342=CARTESIAN_POINT('Origin',(-12.6,10.2,3.5));
#107343=CARTESIAN_POINT('',(-13.05,12.6,3.34));
#107344=CARTESIAN_POINT('Origin',(-12.825,12.6,3.5));
#107345=CARTESIAN_POINT('Origin',(-12.7820819022595,12.6,3.00944389809092));
#107346=CARTESIAN_POINT('',(-12.5605001578317,12.6,3.04851473806598));
#107347=CARTESIAN_POINT('',(-12.9758799382605,12.6,2.81280381763391));
#107348=CARTESIAN_POINT('',(-12.5605001578317,12.6,3.04851473806598));
#107349=CARTESIAN_POINT('Origin',(-13.0314473551139,10.2,3.12794229859781));
#107350=CARTESIAN_POINT('',(-12.5605001578317,10.2,3.04851473806598));
#107351=CARTESIAN_POINT('Origin',(-12.5605001578317,10.2,3.04851473806598));
#107352=CARTESIAN_POINT('Origin',(-12.9207857163291,10.2,2.60718938218245));
#107353=CARTESIAN_POINT('',(-12.4432008140434,12.6,2.61074762735326));
#107354=CARTESIAN_POINT('',(-12.4432008140434,12.6,2.61074762735326));
#107355=CARTESIAN_POINT('',(-12.4432008140434,10.2,2.61074762735326));
#107356=CARTESIAN_POINT('Origin',(-12.4432008140434,10.2,2.61074762735326));
#107357=CARTESIAN_POINT('',(-12.8113392704649,12.6,2.30648774353096));
#107358=CARTESIAN_POINT('Origin',(-12.6546316537202,12.6,2.53379309510498));
#107359=CARTESIAN_POINT('Origin',(-12.446521765691,12.6,2.0875));
#107360=CARTESIAN_POINT('',(-12.2516660498395,12.6,2.2));
#107361=CARTESIAN_POINT('',(-12.5613774815425,12.6,1.83643593539449));
#107362=CARTESIAN_POINT('',(-12.2516660498395,12.6,2.2));
#107363=CARTESIAN_POINT('Origin',(-12.7213774815425,10.2,2.11356406460551));
#107364=CARTESIAN_POINT('',(-12.2516660498395,10.2,2.2));
#107365=CARTESIAN_POINT('Origin',(-12.2516660498395,10.2,2.2));
#107366=CARTESIAN_POINT('Origin',(-12.4392815690627,10.2,1.66206490135509));
#107367=CARTESIAN_POINT('',(-11.9917155521093,12.6,1.828752214815));
#107368=CARTESIAN_POINT('',(-11.9917155521093,12.6,1.828752214815));
#107369=CARTESIAN_POINT('',(-11.9917155521093,10.2,1.828752214815));
#107370=CARTESIAN_POINT('Origin',(-11.9917155521093,10.2,1.828752214815));
#107371=CARTESIAN_POINT('',(-12.233589533963,12.6,1.41693067955702));
#107372=CARTESIAN_POINT('Origin',(-12.1640755518111,12.6,1.68412500263553));
#107373=CARTESIAN_POINT('Origin',(-11.8158749973645,12.6,1.33592444818889));
#107374=CARTESIAN_POINT('',(-11.671247785185,12.6,1.50828444789066));
#107375=CARTESIAN_POINT('',(-11.8379350986449,12.6,1.06071843093727));
#107376=CARTESIAN_POINT('',(-11.671247785185,12.6,1.50828444789066));
#107377=CARTESIAN_POINT('Origin',(-12.083069320443,10.2,1.26641046603696));
#107378=CARTESIAN_POINT('',(-11.671247785185,10.2,1.50828444789066));
#107379=CARTESIAN_POINT('Origin',(-11.671247785185,10.2,1.50828444789066));
#107380=CARTESIAN_POINT('Origin',(-11.6635640646055,10.2,0.938622518457461));
#107381=CARTESIAN_POINT('',(-11.3,12.6,1.24833395016046));
#107382=CARTESIAN_POINT('',(-11.3,12.6,1.24833395016046));
#107383=CARTESIAN_POINT('',(-11.3,10.2,1.24833395016046));
#107384=CARTESIAN_POINT('Origin',(-11.3,10.2,1.24833395016046));
#107385=CARTESIAN_POINT('',(-11.3864359353945,12.6,0.778622518457461));
#107386=CARTESIAN_POINT('Origin',(-11.4125,12.6,1.05347823430896));
#107387=CARTESIAN_POINT('Origin',(-10.966206904895,12.6,0.845368346279809));
#107388=CARTESIAN_POINT('',(-10.8892523726467,12.6,1.05679918595664));
#107389=CARTESIAN_POINT('',(-10.8928106178175,12.6,0.579214283670874));
#107390=CARTESIAN_POINT('',(-10.8892523726467,12.6,1.05679918595664));
#107391=CARTESIAN_POINT('Origin',(-11.193512256469,10.2,0.688660729535087));
#107392=CARTESIAN_POINT('',(-10.8892523726467,10.2,1.05679918595664));
#107393=CARTESIAN_POINT('Origin',(-10.8892523726467,10.2,1.05679918595664));
#107394=CARTESIAN_POINT('Origin',(-10.6871961823661,10.2,0.524120061739474));
#107395=CARTESIAN_POINT('',(-10.451485261934,12.6,0.939499842168259));
#107396=CARTESIAN_POINT('',(-10.451485261934,12.6,0.939499842168259));
#107397=CARTESIAN_POINT('',(-10.451485261934,10.2,0.939499842168259));
#107398=CARTESIAN_POINT('Origin',(-10.451485261934,10.2,0.939499842168259));
#107399=CARTESIAN_POINT('',(-10.3720577014022,12.6,0.468552644886056));
#107400=CARTESIAN_POINT('Origin',(-10.4905561019091,12.6,0.717918097740512));
#107401=CARTESIAN_POINT('Origin',(-10.,12.6,0.675));
#107402=CARTESIAN_POINT('',(-10.,12.6,0.9));
#107403=CARTESIAN_POINT('',(-9.84,12.6,0.45));
#107404=CARTESIAN_POINT('',(-10.,12.6,0.9));
#107405=CARTESIAN_POINT('Origin',(-10.16,10.2,0.45));
#107406=CARTESIAN_POINT('',(-10.,10.2,0.9));
#107407=CARTESIAN_POINT('Origin',(-10.,10.2,0.9));
#107408=CARTESIAN_POINT('Origin',(-9.62794229859782,10.2,0.468552644886056));
#107409=CARTESIAN_POINT('',(-9.54851473806598,12.6,0.939499842168258));
#107410=CARTESIAN_POINT('',(-9.54851473806598,12.6,0.939499842168258));
#107411=CARTESIAN_POINT('',(-9.54851473806598,10.2,0.939499842168258));
#107412=CARTESIAN_POINT('Origin',(-9.54851473806598,10.2,0.939499842168258));
#107413=CARTESIAN_POINT('',(-9.31280381763391,12.6,0.524120061739474));
#107414=CARTESIAN_POINT('Origin',(-9.50944389809092,12.6,0.717918097740512));
#107415=CARTESIAN_POINT('Origin',(-9.03379309510498,12.6,0.845368346279809));
#107416=CARTESIAN_POINT('',(-9.11074762735326,12.6,1.05679918595664));
#107417=CARTESIAN_POINT('',(-8.80648774353096,12.6,0.688660729535087));
#107418=CARTESIAN_POINT('',(-9.11074762735326,12.6,1.05679918595664));
#107419=CARTESIAN_POINT('Origin',(-9.10718938218246,10.2,0.579214283670872));
#107420=CARTESIAN_POINT('',(-9.11074762735326,10.2,1.05679918595664));
#107421=CARTESIAN_POINT('Origin',(-9.11074762735326,10.2,1.05679918595664));
#107422=CARTESIAN_POINT('Origin',(-8.61356406460551,10.2,0.778622518457462));
#107423=CARTESIAN_POINT('',(-8.7,12.6,1.24833395016046));
#107424=CARTESIAN_POINT('',(-8.7,12.6,1.24833395016046));
#107425=CARTESIAN_POINT('',(-8.7,10.2,1.24833395016046));
#107426=CARTESIAN_POINT('Origin',(-8.7,10.2,1.24833395016046));
#107427=CARTESIAN_POINT('',(-8.33643593539449,12.6,0.938622518457463));
#107428=CARTESIAN_POINT('Origin',(-8.5875,12.6,1.05347823430896));
#107429=CARTESIAN_POINT('Origin',(-8.18412500263553,12.6,1.33592444818889));
#107430=CARTESIAN_POINT('',(-8.328752214815,12.6,1.50828444789066));
#107431=CARTESIAN_POINT('',(-7.91693067955702,12.6,1.26641046603696));
#107432=CARTESIAN_POINT('',(-8.328752214815,12.6,1.50828444789066));
#107433=CARTESIAN_POINT('Origin',(-8.16206490135509,10.2,1.06071843093727));
#107434=CARTESIAN_POINT('',(-8.328752214815,10.2,1.50828444789066));
#107435=CARTESIAN_POINT('Origin',(-8.328752214815,10.2,1.50828444789066));
#107436=CARTESIAN_POINT('Origin',(-7.76641046603696,10.2,1.41693067955702));
#107437=CARTESIAN_POINT('',(-8.00828444789066,12.6,1.828752214815));
#107438=CARTESIAN_POINT('',(-8.00828444789066,12.6,1.828752214815));
#107439=CARTESIAN_POINT('',(-8.00828444789066,10.2,1.828752214815));
#107440=CARTESIAN_POINT('Origin',(-8.00828444789066,10.2,1.828752214815));
#107441=CARTESIAN_POINT('',(-7.56071843093727,12.6,1.66206490135509));
#107442=CARTESIAN_POINT('Origin',(-7.83592444818889,12.6,1.68412500263553));
#107443=CARTESIAN_POINT('Origin',(-7.55347823430896,12.6,2.0875));
#107444=CARTESIAN_POINT('',(-7.74833395016046,12.6,2.2));
#107445=CARTESIAN_POINT('',(-7.27862251845746,12.6,2.11356406460551));
#107446=CARTESIAN_POINT('',(-7.74833395016046,12.6,2.2));
#107447=CARTESIAN_POINT('Origin',(-7.43862251845746,10.2,1.83643593539449));
#107448=CARTESIAN_POINT('',(-7.74833395016046,10.2,2.2));
#107449=CARTESIAN_POINT('Origin',(-7.74833395016046,10.2,2.2));
#107450=CARTESIAN_POINT('Origin',(-7.18866072953509,10.2,2.30648774353096));
#107451=CARTESIAN_POINT('',(-7.55679918595664,12.6,2.61074762735326));
#107452=CARTESIAN_POINT('',(-7.55679918595664,12.6,2.61074762735326));
#107453=CARTESIAN_POINT('',(-7.55679918595664,10.2,2.61074762735326));
#107454=CARTESIAN_POINT('Origin',(-7.55679918595664,10.2,2.61074762735326));
#107455=CARTESIAN_POINT('',(-7.07921428367087,12.6,2.60718938218246));
#107456=CARTESIAN_POINT('Origin',(-7.34536834627981,12.6,2.53379309510498));
#107457=CARTESIAN_POINT('Origin',(-7.21791809774051,12.6,3.00944389809092));
#107458=CARTESIAN_POINT('',(-7.43949984216826,12.6,3.04851473806598));
#107459=CARTESIAN_POINT('',(-6.96855264488606,12.6,3.12794229859781));
#107460=CARTESIAN_POINT('',(-7.43949984216826,12.6,3.04851473806598));
#107461=CARTESIAN_POINT('Origin',(-7.02412006173947,10.2,2.81280381763391));
#107462=CARTESIAN_POINT('',(-7.43949984216826,10.2,3.04851473806598));
#107463=CARTESIAN_POINT('Origin',(-7.43949984216826,10.2,3.04851473806598));
#107464=CARTESIAN_POINT('Origin',(-6.95,10.2,3.34));
#107465=CARTESIAN_POINT('',(-7.4,12.6,3.5));
#107466=CARTESIAN_POINT('',(-7.4,12.6,3.5));
#107467=CARTESIAN_POINT('',(-7.4,10.2,3.5));
#107468=CARTESIAN_POINT('Origin',(-7.4,10.2,3.5));
#107469=CARTESIAN_POINT('',(-6.95,12.6,3.66));
#107470=CARTESIAN_POINT('Origin',(-7.175,12.6,3.5));
#107471=CARTESIAN_POINT('Origin',(-10.,13.,3.5));
#107472=CARTESIAN_POINT('Origin',(-10.,13.,0.95));
#107473=CARTESIAN_POINT('Origin',(-10.,10.2,3.5));
#107474=CARTESIAN_POINT('',(-11.5933756729741,10.2,3.5));
#107475=CARTESIAN_POINT('Origin',(-10.,10.2,3.5));
#107476=CARTESIAN_POINT('Origin',(-10.,10.3,3.5));
#107477=CARTESIAN_POINT('',(-11.3903449147952,10.4,3.5918519675297));
#107478=CARTESIAN_POINT('',(-11.4433756729741,10.35,3.5));
#107479=CARTESIAN_POINT('Ctrl Pts',(-11.3903449147952,10.4,3.59185196752971));
#107480=CARTESIAN_POINT('Ctrl Pts',(-11.4163929392269,10.3769827337472,
3.54673546577726));
#107481=CARTESIAN_POINT('Ctrl Pts',(-11.4433756729741,10.35,3.5));
#107482=CARTESIAN_POINT('',(-10.7747185946659,10.4,4.65814803247029));
#107483=CARTESIAN_POINT('Origin',(-10.,10.4,3.5));
#107484=CARTESIAN_POINT('',(-10.721687836487,10.35,4.75));
#107485=CARTESIAN_POINT('Ctrl Pts',(-10.721687836487,10.35,4.75));
#107486=CARTESIAN_POINT('Ctrl Pts',(-10.7486705702342,10.3769827337472,
4.70326453422273));
#107487=CARTESIAN_POINT('Ctrl Pts',(-10.7747185946659,10.4,4.65814803247029));
#107488=CARTESIAN_POINT('',(-10.6156263201293,10.4,4.75));
#107489=CARTESIAN_POINT('Ctrl Pts',(-10.6156263201293,10.4,4.75));
#107490=CARTESIAN_POINT('Ctrl Pts',(-10.6677223689926,10.3769827337472,
4.75));
#107491=CARTESIAN_POINT('Ctrl Pts',(-10.721687836487,10.35,4.75));
#107492=CARTESIAN_POINT('',(-9.38437367987071,10.4,4.75));
#107493=CARTESIAN_POINT('Origin',(-10.,10.4,3.5));
#107494=CARTESIAN_POINT('',(-9.27831216351297,10.35,4.75));
#107495=CARTESIAN_POINT('Ctrl Pts',(-9.27831216351297,10.35,4.75));
#107496=CARTESIAN_POINT('Ctrl Pts',(-9.33227763100738,10.3769827337472,
4.75));
#107497=CARTESIAN_POINT('Ctrl Pts',(-9.38437367987072,10.4,4.75));
#107498=CARTESIAN_POINT('',(-9.2252814053341,10.4,4.65814803247029));
#107499=CARTESIAN_POINT('Ctrl Pts',(-9.22528140533409,10.4,4.65814803247029));
#107500=CARTESIAN_POINT('Ctrl Pts',(-9.25132942976576,10.3769827337472,
4.70326453422274));
#107501=CARTESIAN_POINT('Ctrl Pts',(-9.27831216351297,10.35,4.75));
#107502=CARTESIAN_POINT('',(-8.60965508520481,10.4,3.5918519675297));
#107503=CARTESIAN_POINT('Origin',(-10.,10.4,3.5));
#107504=CARTESIAN_POINT('',(-8.55662432702594,10.35,3.5));
#107505=CARTESIAN_POINT('Ctrl Pts',(-8.55662432702594,10.35,3.5));
#107506=CARTESIAN_POINT('Ctrl Pts',(-8.58360706077314,10.3769827337472,
3.54673546577726));
#107507=CARTESIAN_POINT('Ctrl Pts',(-8.60965508520481,10.4,3.59185196752971));
#107508=CARTESIAN_POINT('',(-8.60965508520481,10.4,3.4081480324703));
#107509=CARTESIAN_POINT('Ctrl Pts',(-8.60965508520481,10.4,3.40814803247029));
#107510=CARTESIAN_POINT('Ctrl Pts',(-8.58360706077314,10.3769827337472,
3.45326453422273));
#107511=CARTESIAN_POINT('Ctrl Pts',(-8.55662432702594,10.35,3.5));
#107512=CARTESIAN_POINT('',(-9.2252814053341,10.4,2.34185196752971));
#107513=CARTESIAN_POINT('Origin',(-10.,10.4,3.5));
#107514=CARTESIAN_POINT('',(-9.27831216351297,10.35,2.25));
#107515=CARTESIAN_POINT('Ctrl Pts',(-9.27831216351297,10.35,2.25));
#107516=CARTESIAN_POINT('Ctrl Pts',(-9.25132942976577,10.3769827337472,
2.29673546577726));
#107517=CARTESIAN_POINT('Ctrl Pts',(-9.22528140533409,10.4,2.34185196752971));
#107518=CARTESIAN_POINT('',(-9.38437367987071,10.4,2.25));
#107519=CARTESIAN_POINT('Ctrl Pts',(-9.38437367987072,10.4,2.25));
#107520=CARTESIAN_POINT('Ctrl Pts',(-9.33227763100738,10.3769827337472,
2.25));
#107521=CARTESIAN_POINT('Ctrl Pts',(-9.27831216351297,10.35,2.25));
#107522=CARTESIAN_POINT('',(-10.6156263201293,10.4,2.25));
#107523=CARTESIAN_POINT('Origin',(-10.,10.4,3.5));
#107524=CARTESIAN_POINT('',(-10.721687836487,10.35,2.25));
#107525=CARTESIAN_POINT('Ctrl Pts',(-10.721687836487,10.35,2.25));
#107526=CARTESIAN_POINT('Ctrl Pts',(-10.6677223689926,10.3769827337472,
2.25));
#107527=CARTESIAN_POINT('Ctrl Pts',(-10.6156263201293,10.4,2.25));
#107528=CARTESIAN_POINT('',(-10.7747185946659,10.4,2.34185196752971));
#107529=CARTESIAN_POINT('Ctrl Pts',(-10.7747185946659,10.4,2.34185196752971));
#107530=CARTESIAN_POINT('Ctrl Pts',(-10.7486705702342,10.3769827337472,
2.29673546577727));
#107531=CARTESIAN_POINT('Ctrl Pts',(-10.721687836487,10.35,2.25));
#107532=CARTESIAN_POINT('',(-11.3903449147952,10.4,3.4081480324703));
#107533=CARTESIAN_POINT('Origin',(-10.,10.4,3.5));
#107534=CARTESIAN_POINT('Ctrl Pts',(-11.4433756729741,10.35,3.5));
#107535=CARTESIAN_POINT('Ctrl Pts',(-11.4163929392269,10.3769827337472,
3.45326453422274));
#107536=CARTESIAN_POINT('Ctrl Pts',(-11.3903449147952,10.4,3.40814803247029));
#107537=CARTESIAN_POINT('',(-11.4933756729741,10.3,3.5));
#107538=CARTESIAN_POINT('Origin',(-10.,10.3,3.5));
#107539=CARTESIAN_POINT('',(-11.3903449147952,10.2,3.4081480324703));
#107540=CARTESIAN_POINT('',(-11.3903449147952,10.3,3.4081480324703));
#107541=CARTESIAN_POINT('',(-10.7747185946659,10.2,2.34185196752971));
#107542=CARTESIAN_POINT('',(-10.7747185946659,10.3,2.34185196752971));
#107543=CARTESIAN_POINT('Origin',(-10.,10.2,3.5));
#107544=CARTESIAN_POINT('Origin',(-10.,10.3,3.5));
#107545=CARTESIAN_POINT('',(-9.38437367987071,10.2,2.25));
#107546=CARTESIAN_POINT('',(-9.38437367987071,10.3,2.25));
#107547=CARTESIAN_POINT('',(-10.6156263201293,10.2,2.25));
#107548=CARTESIAN_POINT('Origin',(-10.,10.2,3.5));
#107549=CARTESIAN_POINT('',(-10.6156263201293,10.3,2.25));
#107550=CARTESIAN_POINT('Origin',(-10.,10.3,3.5));
#107551=CARTESIAN_POINT('',(-10.7747185946659,10.2,4.65814803247029));
#107552=CARTESIAN_POINT('',(-10.7747185946659,10.3,4.65814803247029));
#107553=CARTESIAN_POINT('',(-11.3903449147952,10.2,3.5918519675297));
#107554=CARTESIAN_POINT('',(-11.3903449147952,10.3,3.5918519675297));
#107555=CARTESIAN_POINT('Origin',(-10.,10.2,3.5));
#107556=CARTESIAN_POINT('Origin',(-10.,10.3,3.5));
#107557=CARTESIAN_POINT('',(-8.60965508520481,10.2,3.4081480324703));
#107558=CARTESIAN_POINT('',(-8.60965508520481,10.3,3.4081480324703));
#107559=CARTESIAN_POINT('',(-9.2252814053341,10.2,2.34185196752971));
#107560=CARTESIAN_POINT('Origin',(-10.,10.2,3.5));
#107561=CARTESIAN_POINT('',(-9.2252814053341,10.3,2.34185196752971));
#107562=CARTESIAN_POINT('Origin',(-10.,10.3,3.5));
#107563=CARTESIAN_POINT('',(-9.38437367987071,10.2,4.75));
#107564=CARTESIAN_POINT('',(-9.38437367987071,10.3,4.75));
#107565=CARTESIAN_POINT('',(-10.6156263201293,10.2,4.75));
#107566=CARTESIAN_POINT('',(-10.6156263201293,10.3,4.75));
#107567=CARTESIAN_POINT('Origin',(-10.,10.2,3.5));
#107568=CARTESIAN_POINT('Origin',(-10.,10.3,3.5));
#107569=CARTESIAN_POINT('',(-9.2252814053341,10.2,4.65814803247029));
#107570=CARTESIAN_POINT('',(-9.2252814053341,10.3,4.65814803247029));
#107571=CARTESIAN_POINT('',(-8.60965508520481,10.2,3.5918519675297));
#107572=CARTESIAN_POINT('Origin',(-10.,10.2,3.5));
#107573=CARTESIAN_POINT('',(-8.60965508520481,10.3,3.5918519675297));
#107574=CARTESIAN_POINT('Origin',(-10.721687836487,10.2,4.75));
#107575=CARTESIAN_POINT('',(-10.3608439182435,10.2,4.75));
#107576=CARTESIAN_POINT('',(-10.721687836487,11.5,4.75));
#107577=CARTESIAN_POINT('',(-10.721687836487,10.2,4.75));
#107578=CARTESIAN_POINT('',(-9.27831216351297,11.5,4.75));
#107579=CARTESIAN_POINT('',(-9.27831216351297,11.5,4.75));
#107580=CARTESIAN_POINT('',(-9.27831216351297,10.2,4.75));
#107581=CARTESIAN_POINT('Origin',(-11.4433756729741,10.2,3.5));
#107582=CARTESIAN_POINT('',(-11.2629537138523,10.2,3.8125));
#107583=CARTESIAN_POINT('',(-11.4433756729741,11.5,3.5));
#107584=CARTESIAN_POINT('',(-11.4433756729741,10.2,3.5));
#107585=CARTESIAN_POINT('',(-10.721687836487,11.5,4.75));
#107586=CARTESIAN_POINT('Origin',(-10.721687836487,10.2,2.25));
#107587=CARTESIAN_POINT('',(-10.9021097956088,10.2,2.5625));
#107588=CARTESIAN_POINT('',(-10.721687836487,11.5,2.25));
#107589=CARTESIAN_POINT('',(-10.721687836487,10.2,2.25));
#107590=CARTESIAN_POINT('',(-11.4433756729741,11.5,3.5));
#107591=CARTESIAN_POINT('Origin',(-10.,10.2,3.5));
#107592=CARTESIAN_POINT('Origin',(-10.,10.2,3.5));
#107593=CARTESIAN_POINT('Origin',(-10.,10.2,3.5));
#107594=CARTESIAN_POINT('',(-9.63915608175648,10.2,2.25));
#107595=CARTESIAN_POINT('Origin',(-10.,10.2,3.5));
#107596=CARTESIAN_POINT('Origin',(-10.,10.2,3.5));
#107597=CARTESIAN_POINT('',(-8.7370462861477,10.2,3.1875));
#107598=CARTESIAN_POINT('Origin',(-10.,10.2,3.5));
#107599=CARTESIAN_POINT('',(-9.09789020439121,10.2,4.4375));
#107600=CARTESIAN_POINT('Origin',(-10.,11.5,3.5));
#107601=CARTESIAN_POINT('',(-8.55662432702594,11.5,3.5));
#107602=CARTESIAN_POINT('',(-9.27831216351297,11.5,2.25));
#107603=CARTESIAN_POINT('',(-9.27831216351297,11.5,2.25));
#107604=CARTESIAN_POINT('Origin',(-10.,11.5,3.5));
#107605=CARTESIAN_POINT('Origin',(-10.,11.5,3.5));
#107606=CARTESIAN_POINT('',(-10.721687836487,11.5,2.25));
#107607=CARTESIAN_POINT('Origin',(-10.,11.5,3.5));
#107608=CARTESIAN_POINT('Origin',(-10.,11.5,3.5));
#107609=CARTESIAN_POINT('Origin',(-10.,11.5,3.5));
#107610=CARTESIAN_POINT('Origin',(-10.,11.5,3.5));
#107611=CARTESIAN_POINT('Origin',(-10.,11.5,3.5));
#107612=CARTESIAN_POINT('Origin',(-10.,11.5,3.5));
#107613=CARTESIAN_POINT('Origin',(-10.,11.5,3.5));
#107614=CARTESIAN_POINT('Origin',(-10.,11.5,3.5));
#107615=CARTESIAN_POINT('',(-8.55662432702594,11.5,3.5));
#107616=CARTESIAN_POINT('Origin',(-10.,11.5,3.5));
#107617=CARTESIAN_POINT('Origin',(-10.,11.9336338001763,3.5));
#107618=CARTESIAN_POINT('',(-10.,12.3672676003525,3.5));
#107619=CARTESIAN_POINT('',(-10.721687836487,11.9336338001763,3.5));
#107620=CARTESIAN_POINT('Origin',(-8.55662432702594,10.2,3.5));
#107621=CARTESIAN_POINT('',(-8.55662432702594,10.2,3.5));
#107622=CARTESIAN_POINT('',(-9.27831216351297,10.2,2.25));
#107623=CARTESIAN_POINT('Origin',(-9.27831216351297,10.2,4.75));
#107624=CARTESIAN_POINT('Origin',(-9.27831216351297,10.2,2.25));
#135264=UNCERTAINTY_MEASURE_WITH_UNIT(LENGTH_MEASURE(0.01),#135283,
'DISTANCE_ACCURACY_VALUE',
'Maximum model space distance between geometric entities at asserted c
onnectivities');
#135267=UNCERTAINTY_MEASURE_WITH_UNIT(LENGTH_MEASURE(0.01),#135283,
'DISTANCE_ACCURACY_VALUE',
'Maximum model space distance between geometric entities at asserted c
onnectivities');
#135279=(
GEOMETRIC_REPRESENTATION_CONTEXT(3)
GLOBAL_UNCERTAINTY_ASSIGNED_CONTEXT((#135264))
GLOBAL_UNIT_ASSIGNED_CONTEXT((#135283,#135285,#135286))
REPRESENTATION_CONTEXT('','3D')
);
#135282=(
GEOMETRIC_REPRESENTATION_CONTEXT(3)
GLOBAL_UNCERTAINTY_ASSIGNED_CONTEXT((#135267))
GLOBAL_UNIT_ASSIGNED_CONTEXT((#135283,#135285,#135286))
REPRESENTATION_CONTEXT('','3D')
);
#135283=(
LENGTH_UNIT()
NAMED_UNIT(*)
SI_UNIT(.MILLI.,.METRE.)
);
#135285=(
NAMED_UNIT(*)
PLANE_ANGLE_UNIT()
SI_UNIT($,.RADIAN.)
);
#135286=(
NAMED_UNIT(*)
SI_UNIT($,.STERADIAN.)
SOLID_ANGLE_UNIT()
);
#135298=SHAPE_DEFINITION_REPRESENTATION(#135312,#135347);
#135312=PRODUCT_DEFINITION_SHAPE('',$,#135362);
#135347=SHAPE_REPRESENTATION('',(#33555),#135279);
#135350=PRODUCT_DEFINITION_CONTEXT('part definition',#135394,'design');
#135362=PRODUCT_DEFINITION('2026-10-15-19-09-11-264',
'ISO 4762 - M3 x 12 - 12.9',#135376,#135350);
#135376=PRODUCT_DEFINITION_FORMATION('',$,#135407);
#135394=APPLICATION_CONTEXT(
'Core Data for Automotive Mechanical Design Process');
#135395=PRODUCT_CONTEXT('part definition',#135394,'mechanical');
#135407=PRODUCT('2026-10-15-19-09-11-264','ISO 4762 - M3 x 12 - 12.9',$,
(#135395));
#135421=PRESENTATION_STYLE_ASSIGNMENT((#135435));
#135435=SURFACE_STYLE_USAGE(.BOTH.,#135449);
#135449=SURFACE_SIDE_STYLE('',(#135463));
#135463=SURFACE_STYLE_FILL_AREA(#135477);
#135477=FILL_AREA_STYLE('Opaque(199,204,210)',(#135491));
#135491=FILL_AREA_STYLE_COLOUR('Opaque(199,204,210)',#135505);
#135505=COLOUR_RGB('Opaque(199,204,210)', 0.72549020, 0.75294118, 0.79215686);
ENDSEC;
END-ISO-10303-21;
